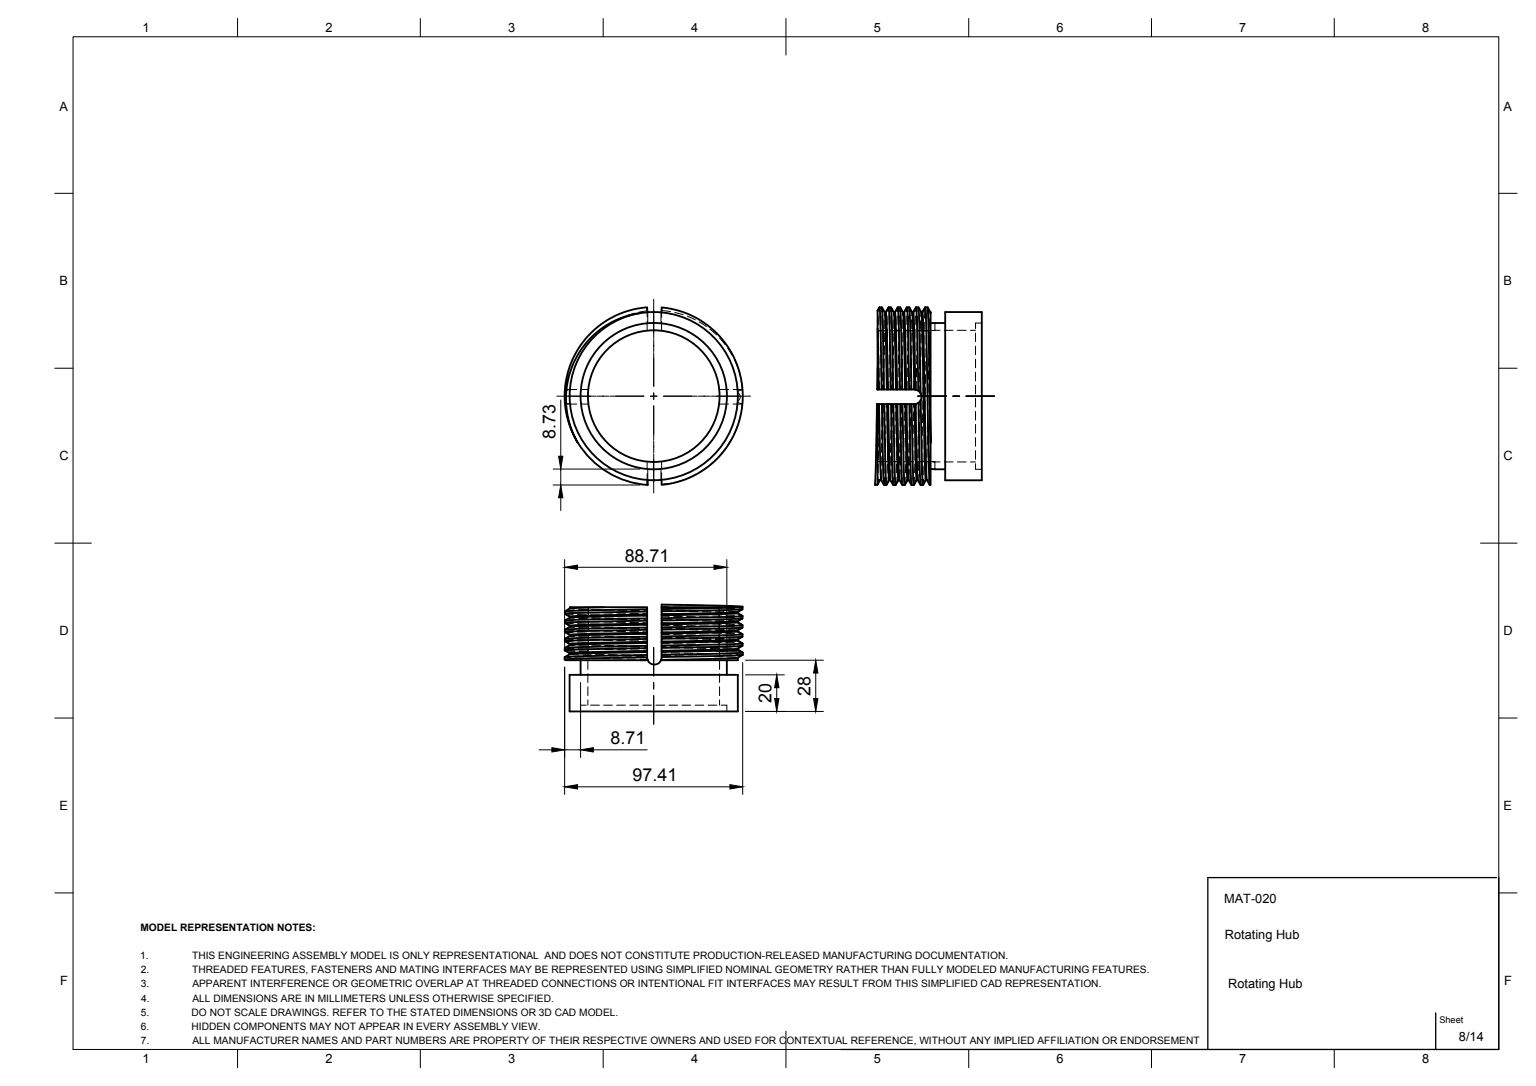
ISO-10303-21;
HEADER;
/* Generated by software containing ST-Developer
 * from STEP Tools, Inc. (www.steptools.com) 
 */

FILE_DESCRIPTION(
/* description */ ('STEP AP214'),
/* implementation_level */ '2;1');

FILE_NAME(
/* name */ 'Rotating Hub.step',
/* time_stamp */ '2026-11-14T06:20:50-08:00',
/* author */ (''),
/* organization */ (''),
/* preprocessor_version */ 'ST-DEVELOPER v20.2',
/* originating_system */ 'Autodesk Translation Framework v15.17.0.0',
/* authorisation */ '');

FILE_SCHEMA (('AUTOMOTIVE_DESIGN { 1 0 10303 214 3 1 1 }'));
ENDSEC;

DATA;
#10=MECHANICAL_DESIGN_GEOMETRIC_PRESENTATION_REPRESENTATION('',(#959),#20658);
#124=FACE_BOUND('',#1300,.T.);
#125=FACE_BOUND('',#1302,.T.);
#126=FACE_BOUND('',#1314,.T.);
#147=ELLIPSE('',#3911,3.97203818895926,3.95968922073708);
#152=(
BOUNDED_SURFACE()
B_SPLINE_SURFACE(1,2,((#5540,#5541,#5542,#5543,#5544,#5545,#5546,#5547,
#5548,#5549,#5550,#5551,#5552,#5553,#5554,#5555,#5556,#5557,#5558,#5559,
#5560,#5561,#5562,#5563,#5564,#5565,#5566,#5567,#5568,#5569,#5570,#5571,
#5572,#5573,#5574,#5575,#5576,#5577,#5578,#5579,#5580,#5581,#5582,#5583,
#5584,#5585,#5586,#5587,#5588,#5589,#5590,#5591,#5592,#5593,#5594,#5595,
#5596,#5597,#5598,#5599,#5600,#5601,#5602,#5603,#5604,#5605,#5606,#5607,
#5608,#5609,#5610,#5611,#5612,#5613,#5614,#5615,#5616,#5617,#5618,#5619,
#5620,#5621,#5622,#5623,#5624,#5625,#5626,#5627,#5628,#5629,#5630,#5631,
#5632,#5633,#5634,#5635,#5636,#5637,#5638,#5639,#5640,#5641,#5642,#5643,
#5644,#5645,#5646,#5647,#5648,#5649,#5650,#5651,#5652,#5653,#5654,#5655,
#5656,#5657,#5658,#5659,#5660,#5661,#5662,#5663,#5664,#5665,#5666,#5667,
#5668,#5669,#5670,#5671,#5672,#5673,#5674,#5675,#5676,#5677,#5678,#5679,
#5680,#5681,#5682,#5683,#5684),(#5685,#5686,#5687,#5688,#5689,#5690,#5691,
#5692,#5693,#5694,#5695,#5696,#5697,#5698,#5699,#5700,#5701,#5702,#5703,
#5704,#5705,#5706,#5707,#5708,#5709,#5710,#5711,#5712,#5713,#5714,#5715,
#5716,#5717,#5718,#5719,#5720,#5721,#5722,#5723,#5724,#5725,#5726,#5727,
#5728,#5729,#5730,#5731,#5732,#5733,#5734,#5735,#5736,#5737,#5738,#5739,
#5740,#5741,#5742,#5743,#5744,#5745,#5746,#5747,#5748,#5749,#5750,#5751,
#5752,#5753,#5754,#5755,#5756,#5757,#5758,#5759,#5760,#5761,#5762,#5763,
#5764,#5765,#5766,#5767,#5768,#5769,#5770,#5771,#5772,#5773,#5774,#5775,
#5776,#5777,#5778,#5779,#5780,#5781,#5782,#5783,#5784,#5785,#5786,#5787,
#5788,#5789,#5790,#5791,#5792,#5793,#5794,#5795,#5796,#5797,#5798,#5799,
#5800,#5801,#5802,#5803,#5804,#5805,#5806,#5807,#5808,#5809,#5810,#5811,
#5812,#5813,#5814,#5815,#5816,#5817,#5818,#5819,#5820,#5821,#5822,#5823,
#5824,#5825,#5826,#5827,#5828,#5829)),.UNSPECIFIED.,.F.,.F.,.F.)
B_SPLINE_SURFACE_WITH_KNOTS((2,2),(3,2,2,2,2,2,2,2,2,2,2,2,2,2,2,2,2,2,
2,2,2,2,2,2,2,2,2,2,2,2,2,2,2,2,2,2,2,2,2,2,2,2,2,2,2,2,2,2,2,2,2,2,2,2,
2,2,2,2,2,2,2,2,2,2,2,2,2,2,2,2,2,2,3),(0.,1.),(0.,0.0138888888888889,0.0277777777777778,
0.0416666666666667,0.0555555555555556,0.0694444444444444,0.0833333333333333,
0.0972222222222222,0.111111111111111,0.125,0.138888888888889,0.152777777777778,
0.166666666666667,0.180555555555556,0.194444444444444,0.208333333333333,
0.222222222222222,0.236111111111111,0.25,0.263888888888889,0.277777777777778,
0.291666666666667,0.305555555555556,0.319444444444444,0.333333333333333,
0.347222222222222,0.361111111111111,0.375,0.388888888888889,0.402777777777778,
0.416666666666667,0.430555555555556,0.444444444444444,0.458333333333333,
0.472222222222222,0.486111111111111,0.5,0.513888888888889,0.527777777777778,
0.541666666666667,0.555555555555556,0.569444444444444,0.583333333333333,
0.597222222222222,0.611111111111111,0.625,0.638888888888889,0.652777777777778,
0.666666666666667,0.680555555555556,0.694444444444444,0.708333333333333,
0.722222222222222,0.736111111111111,0.75,0.763888888888889,0.777777777777778,
0.791666666666667,0.805555555555556,0.819444444444444,0.833333333333333,
0.847222222222222,0.861111111111111,0.875,0.888888888888889,0.902777777777778,
0.916666666666667,0.930555555555556,0.944444444444444,0.958333333333333,
0.972222222222222,0.986111111111111,1.),.UNSPECIFIED.)
GEOMETRIC_REPRESENTATION_ITEM()
RATIONAL_B_SPLINE_SURFACE(((1.,0.965925826289068,1.,0.965925826289068,1.,
0.965925826289068,1.,0.965925826289068,1.,0.965925826289068,1.,0.965925826289068,
1.,0.965925826289068,1.,0.965925826289068,1.,0.965925826289068,1.,0.965925826289068,
1.,0.965925826289068,1.,0.965925826289068,1.,0.965925826289068,1.,0.965925826289068,
1.,0.965925826289068,1.,0.965925826289068,1.,0.965925826289068,1.,0.965925826289068,
1.,0.965925826289068,1.,0.965925826289068,1.,0.965925826289068,1.,0.965925826289068,
1.,0.965925826289068,1.,0.965925826289068,1.,0.965925826289068,1.,0.965925826289068,
1.,0.965925826289068,1.,0.965925826289068,1.,0.965925826289068,1.,0.965925826289068,
1.,0.965925826289068,1.,0.965925826289068,1.,0.965925826289068,1.,0.965925826289068,
1.,0.965925826289068,1.,0.965925826289068,1.,0.965925826289068,1.,0.965925826289068,
1.,0.965925826289068,1.,0.965925826289068,1.,0.965925826289068,1.,0.965925826289068,
1.,0.965925826289068,1.,0.965925826289068,1.,0.965925826289068,1.,0.965925826289068,
1.,0.965925826289068,1.,0.965925826289068,1.,0.965925826289068,1.,0.965925826289068,
1.,0.965925826289068,1.,0.965925826289068,1.,0.965925826289068,1.,0.965925826289068,
1.,0.965925826289068,1.,0.965925826289068,1.,0.965925826289068,1.,0.965925826289068,
1.,0.965925826289068,1.,0.965925826289068,1.,0.965925826289068,1.,0.965925826289068,
1.,0.965925826289068,1.,0.965925826289068,1.,0.965925826289068,1.,0.965925826289068,
1.,0.965925826289068,1.,0.965925826289068,1.,0.965925826289068,1.,0.965925826289068,
1.,0.965925826289068,1.,0.965925826289068,1.),(1.,0.965925826289068,1.,
0.965925826289068,1.,0.965925826289068,1.,0.965925826289068,1.,0.965925826289068,
1.,0.965925826289068,1.,0.965925826289068,1.,0.965925826289068,1.,0.965925826289068,
1.,0.965925826289068,1.,0.965925826289068,1.,0.965925826289068,1.,0.965925826289068,
1.,0.965925826289068,1.,0.965925826289068,1.,0.965925826289068,1.,0.965925826289068,
1.,0.965925826289068,1.,0.965925826289068,1.,0.965925826289068,1.,0.965925826289068,
1.,0.965925826289068,1.,0.965925826289068,1.,0.965925826289068,1.,0.965925826289068,
1.,0.965925826289068,1.,0.965925826289068,1.,0.965925826289068,1.,0.965925826289068,
1.,0.965925826289068,1.,0.965925826289068,1.,0.965925826289068,1.,0.965925826289068,
1.,0.965925826289068,1.,0.965925826289068,1.,0.965925826289068,1.,0.965925826289068,
1.,0.965925826289068,1.,0.965925826289068,1.,0.965925826289068,1.,0.965925826289068,
1.,0.965925826289068,1.,0.965925826289068,1.,0.965925826289068,1.,0.965925826289068,
1.,0.965925826289068,1.,0.965925826289068,1.,0.965925826289068,1.,0.965925826289068,
1.,0.965925826289068,1.,0.965925826289068,1.,0.965925826289068,1.,0.965925826289068,
1.,0.965925826289068,1.,0.965925826289068,1.,0.965925826289068,1.,0.965925826289068,
1.,0.965925826289068,1.,0.965925826289068,1.,0.965925826289068,1.,0.965925826289068,
1.,0.965925826289068,1.,0.965925826289068,1.,0.965925826289068,1.,0.965925826289068,
1.,0.965925826289068,1.,0.965925826289068,1.,0.965925826289068,1.,0.965925826289068,
1.,0.965925826289068,1.,0.965925826289068,1.,0.965925826289068,1.)))
REPRESENTATION_ITEM('')
SURFACE()
);
#153=(
BOUNDED_SURFACE()
B_SPLINE_SURFACE(1,2,((#5847,#5848,#5849,#5850,#5851,#5852,#5853,#5854,
#5855,#5856,#5857,#5858,#5859,#5860,#5861,#5862,#5863,#5864,#5865,#5866,
#5867,#5868,#5869,#5870,#5871,#5872,#5873,#5874,#5875,#5876,#5877,#5878,
#5879,#5880,#5881,#5882,#5883,#5884,#5885,#5886,#5887,#5888,#5889,#5890,
#5891,#5892,#5893,#5894,#5895,#5896,#5897,#5898,#5899,#5900,#5901,#5902,
#5903,#5904,#5905,#5906,#5907,#5908,#5909,#5910,#5911,#5912,#5913,#5914,
#5915,#5916,#5917,#5918,#5919,#5920,#5921,#5922,#5923,#5924,#5925,#5926,
#5927,#5928,#5929,#5930,#5931,#5932,#5933,#5934,#5935,#5936,#5937,#5938,
#5939,#5940,#5941,#5942,#5943,#5944,#5945,#5946,#5947,#5948,#5949,#5950,
#5951,#5952,#5953,#5954,#5955,#5956,#5957,#5958,#5959,#5960,#5961,#5962,
#5963,#5964,#5965,#5966,#5967,#5968,#5969,#5970,#5971,#5972,#5973,#5974,
#5975,#5976,#5977,#5978,#5979,#5980,#5981,#5982,#5983,#5984,#5985,#5986,
#5987,#5988,#5989,#5990,#5991),(#5992,#5993,#5994,#5995,#5996,#5997,#5998,
#5999,#6000,#6001,#6002,#6003,#6004,#6005,#6006,#6007,#6008,#6009,#6010,
#6011,#6012,#6013,#6014,#6015,#6016,#6017,#6018,#6019,#6020,#6021,#6022,
#6023,#6024,#6025,#6026,#6027,#6028,#6029,#6030,#6031,#6032,#6033,#6034,
#6035,#6036,#6037,#6038,#6039,#6040,#6041,#6042,#6043,#6044,#6045,#6046,
#6047,#6048,#6049,#6050,#6051,#6052,#6053,#6054,#6055,#6056,#6057,#6058,
#6059,#6060,#6061,#6062,#6063,#6064,#6065,#6066,#6067,#6068,#6069,#6070,
#6071,#6072,#6073,#6074,#6075,#6076,#6077,#6078,#6079,#6080,#6081,#6082,
#6083,#6084,#6085,#6086,#6087,#6088,#6089,#6090,#6091,#6092,#6093,#6094,
#6095,#6096,#6097,#6098,#6099,#6100,#6101,#6102,#6103,#6104,#6105,#6106,
#6107,#6108,#6109,#6110,#6111,#6112,#6113,#6114,#6115,#6116,#6117,#6118,
#6119,#6120,#6121,#6122,#6123,#6124,#6125,#6126,#6127,#6128,#6129,#6130,
#6131,#6132,#6133,#6134,#6135,#6136)),.UNSPECIFIED.,.F.,.F.,.F.)
B_SPLINE_SURFACE_WITH_KNOTS((2,2),(3,2,2,2,2,2,2,2,2,2,2,2,2,2,2,2,2,2,
2,2,2,2,2,2,2,2,2,2,2,2,2,2,2,2,2,2,2,2,2,2,2,2,2,2,2,2,2,2,2,2,2,2,2,2,
2,2,2,2,2,2,2,2,2,2,2,2,2,2,2,2,2,2,3),(0.,1.),(0.,0.0138888888888889,0.0277777777777778,
0.0416666666666667,0.0555555555555556,0.0694444444444444,0.0833333333333333,
0.0972222222222222,0.111111111111111,0.125,0.138888888888889,0.152777777777778,
0.166666666666667,0.180555555555556,0.194444444444444,0.208333333333333,
0.222222222222222,0.236111111111111,0.25,0.263888888888889,0.277777777777778,
0.291666666666667,0.305555555555556,0.319444444444444,0.333333333333333,
0.347222222222222,0.361111111111111,0.375,0.388888888888889,0.402777777777778,
0.416666666666667,0.430555555555556,0.444444444444444,0.458333333333333,
0.472222222222222,0.486111111111111,0.5,0.513888888888889,0.527777777777778,
0.541666666666667,0.555555555555556,0.569444444444444,0.583333333333333,
0.597222222222222,0.611111111111111,0.625,0.638888888888889,0.652777777777778,
0.666666666666667,0.680555555555556,0.694444444444444,0.708333333333333,
0.722222222222222,0.736111111111111,0.75,0.763888888888889,0.777777777777778,
0.791666666666667,0.805555555555556,0.819444444444444,0.833333333333333,
0.847222222222222,0.861111111111111,0.875,0.888888888888889,0.902777777777778,
0.916666666666667,0.930555555555556,0.944444444444444,0.958333333333333,
0.972222222222222,0.986111111111111,1.),.UNSPECIFIED.)
GEOMETRIC_REPRESENTATION_ITEM()
RATIONAL_B_SPLINE_SURFACE(((1.,0.965925826289068,1.,0.965925826289068,1.,
0.965925826289068,1.,0.965925826289068,1.,0.965925826289068,1.,0.965925826289068,
1.,0.965925826289068,1.,0.965925826289068,1.,0.965925826289068,1.,0.965925826289068,
1.,0.965925826289068,1.,0.965925826289068,1.,0.965925826289068,1.,0.965925826289068,
1.,0.965925826289068,1.,0.965925826289068,1.,0.965925826289068,1.,0.965925826289068,
1.,0.965925826289068,1.,0.965925826289068,1.,0.965925826289068,1.,0.965925826289068,
1.,0.965925826289068,1.,0.965925826289068,1.,0.965925826289068,1.,0.965925826289068,
1.,0.965925826289068,1.,0.965925826289068,1.,0.965925826289068,1.,0.965925826289068,
1.,0.965925826289068,1.,0.965925826289068,1.,0.965925826289068,1.,0.965925826289068,
1.,0.965925826289068,1.,0.965925826289068,1.,0.965925826289068,1.,0.965925826289068,
1.,0.965925826289068,1.,0.965925826289068,1.,0.965925826289068,1.,0.965925826289068,
1.,0.965925826289068,1.,0.965925826289068,1.,0.965925826289068,1.,0.965925826289068,
1.,0.965925826289068,1.,0.965925826289068,1.,0.965925826289068,1.,0.965925826289068,
1.,0.965925826289068,1.,0.965925826289068,1.,0.965925826289068,1.,0.965925826289068,
1.,0.965925826289068,1.,0.965925826289068,1.,0.965925826289068,1.,0.965925826289068,
1.,0.965925826289068,1.,0.965925826289068,1.,0.965925826289068,1.,0.965925826289068,
1.,0.965925826289068,1.,0.965925826289068,1.,0.965925826289068,1.,0.965925826289068,
1.,0.965925826289068,1.,0.965925826289068,1.,0.965925826289068,1.,0.965925826289068,
1.,0.965925826289068,1.,0.965925826289068,1.),(1.,0.965925826289068,1.,
0.965925826289068,1.,0.965925826289068,1.,0.965925826289068,1.,0.965925826289068,
1.,0.965925826289068,1.,0.965925826289068,1.,0.965925826289068,1.,0.965925826289068,
1.,0.965925826289068,1.,0.965925826289068,1.,0.965925826289068,1.,0.965925826289068,
1.,0.965925826289068,1.,0.965925826289068,1.,0.965925826289068,1.,0.965925826289068,
1.,0.965925826289068,1.,0.965925826289068,1.,0.965925826289068,1.,0.965925826289068,
1.,0.965925826289068,1.,0.965925826289068,1.,0.965925826289068,1.,0.965925826289068,
1.,0.965925826289068,1.,0.965925826289068,1.,0.965925826289068,1.,0.965925826289068,
1.,0.965925826289068,1.,0.965925826289068,1.,0.965925826289068,1.,0.965925826289068,
1.,0.965925826289068,1.,0.965925826289068,1.,0.965925826289068,1.,0.965925826289068,
1.,0.965925826289068,1.,0.965925826289068,1.,0.965925826289068,1.,0.965925826289068,
1.,0.965925826289068,1.,0.965925826289068,1.,0.965925826289068,1.,0.965925826289068,
1.,0.965925826289068,1.,0.965925826289068,1.,0.965925826289068,1.,0.965925826289068,
1.,0.965925826289068,1.,0.965925826289068,1.,0.965925826289068,1.,0.965925826289068,
1.,0.965925826289068,1.,0.965925826289068,1.,0.965925826289068,1.,0.965925826289068,
1.,0.965925826289068,1.,0.965925826289068,1.,0.965925826289068,1.,0.965925826289068,
1.,0.965925826289068,1.,0.965925826289068,1.,0.965925826289068,1.,0.965925826289068,
1.,0.965925826289068,1.,0.965925826289068,1.,0.965925826289068,1.,0.965925826289068,
1.,0.965925826289068,1.,0.965925826289068,1.,0.965925826289068,1.)))
REPRESENTATION_ITEM('')
SURFACE()
);
#154=(
BOUNDED_SURFACE()
B_SPLINE_SURFACE(1,2,((#6162,#6163,#6164,#6165,#6166,#6167,#6168,#6169,
#6170,#6171,#6172,#6173,#6174,#6175,#6176,#6177,#6178,#6179,#6180,#6181,
#6182,#6183,#6184,#6185,#6186,#6187,#6188,#6189,#6190,#6191,#6192,#6193,
#6194,#6195,#6196,#6197,#6198,#6199,#6200,#6201,#6202,#6203,#6204,#6205,
#6206,#6207,#6208,#6209,#6210,#6211,#6212,#6213,#6214,#6215,#6216,#6217,
#6218,#6219,#6220,#6221,#6222,#6223,#6224,#6225,#6226,#6227,#6228,#6229,
#6230,#6231,#6232,#6233,#6234,#6235,#6236,#6237,#6238,#6239,#6240,#6241,
#6242,#6243,#6244,#6245,#6246,#6247,#6248,#6249,#6250,#6251,#6252,#6253,
#6254,#6255,#6256,#6257,#6258,#6259,#6260,#6261,#6262,#6263,#6264,#6265,
#6266,#6267,#6268,#6269,#6270,#6271,#6272,#6273,#6274,#6275,#6276,#6277,
#6278,#6279,#6280,#6281,#6282,#6283,#6284,#6285,#6286,#6287,#6288,#6289,
#6290,#6291,#6292,#6293,#6294,#6295,#6296,#6297,#6298,#6299,#6300,#6301,
#6302,#6303,#6304,#6305,#6306),(#6307,#6308,#6309,#6310,#6311,#6312,#6313,
#6314,#6315,#6316,#6317,#6318,#6319,#6320,#6321,#6322,#6323,#6324,#6325,
#6326,#6327,#6328,#6329,#6330,#6331,#6332,#6333,#6334,#6335,#6336,#6337,
#6338,#6339,#6340,#6341,#6342,#6343,#6344,#6345,#6346,#6347,#6348,#6349,
#6350,#6351,#6352,#6353,#6354,#6355,#6356,#6357,#6358,#6359,#6360,#6361,
#6362,#6363,#6364,#6365,#6366,#6367,#6368,#6369,#6370,#6371,#6372,#6373,
#6374,#6375,#6376,#6377,#6378,#6379,#6380,#6381,#6382,#6383,#6384,#6385,
#6386,#6387,#6388,#6389,#6390,#6391,#6392,#6393,#6394,#6395,#6396,#6397,
#6398,#6399,#6400,#6401,#6402,#6403,#6404,#6405,#6406,#6407,#6408,#6409,
#6410,#6411,#6412,#6413,#6414,#6415,#6416,#6417,#6418,#6419,#6420,#6421,
#6422,#6423,#6424,#6425,#6426,#6427,#6428,#6429,#6430,#6431,#6432,#6433,
#6434,#6435,#6436,#6437,#6438,#6439,#6440,#6441,#6442,#6443,#6444,#6445,
#6446,#6447,#6448,#6449,#6450,#6451)),.UNSPECIFIED.,.F.,.F.,.F.)
B_SPLINE_SURFACE_WITH_KNOTS((2,2),(3,2,2,2,2,2,2,2,2,2,2,2,2,2,2,2,2,2,
2,2,2,2,2,2,2,2,2,2,2,2,2,2,2,2,2,2,2,2,2,2,2,2,2,2,2,2,2,2,2,2,2,2,2,2,
2,2,2,2,2,2,2,2,2,2,2,2,2,2,2,2,2,2,3),(0.,1.),(0.,0.0138888888888889,0.0277777777777778,
0.0416666666666667,0.0555555555555556,0.0694444444444444,0.0833333333333333,
0.0972222222222222,0.111111111111111,0.125,0.138888888888889,0.152777777777778,
0.166666666666667,0.180555555555556,0.194444444444444,0.208333333333333,
0.222222222222222,0.236111111111111,0.25,0.263888888888889,0.277777777777778,
0.291666666666667,0.305555555555556,0.319444444444444,0.333333333333333,
0.347222222222222,0.361111111111111,0.375,0.388888888888889,0.402777777777778,
0.416666666666667,0.430555555555556,0.444444444444444,0.458333333333333,
0.472222222222222,0.486111111111111,0.5,0.513888888888889,0.527777777777778,
0.541666666666667,0.555555555555556,0.569444444444444,0.583333333333333,
0.597222222222222,0.611111111111111,0.625,0.638888888888889,0.652777777777778,
0.666666666666667,0.680555555555556,0.694444444444444,0.708333333333333,
0.722222222222222,0.736111111111111,0.75,0.763888888888889,0.777777777777778,
0.791666666666667,0.805555555555556,0.819444444444444,0.833333333333333,
0.847222222222222,0.861111111111111,0.875,0.888888888888889,0.902777777777778,
0.916666666666667,0.930555555555556,0.944444444444444,0.958333333333333,
0.972222222222222,0.986111111111111,1.),.UNSPECIFIED.)
GEOMETRIC_REPRESENTATION_ITEM()
RATIONAL_B_SPLINE_SURFACE(((1.,0.965925826289068,1.,0.965925826289068,1.,
0.965925826289068,1.,0.965925826289068,1.,0.965925826289068,1.,0.965925826289068,
1.,0.965925826289068,1.,0.965925826289068,1.,0.965925826289068,1.,0.965925826289068,
1.,0.965925826289068,1.,0.965925826289068,1.,0.965925826289068,1.,0.965925826289068,
1.,0.965925826289068,1.,0.965925826289068,1.,0.965925826289068,1.,0.965925826289068,
1.,0.965925826289068,1.,0.965925826289068,1.,0.965925826289068,1.,0.965925826289068,
1.,0.965925826289068,1.,0.965925826289068,1.,0.965925826289068,1.,0.965925826289068,
1.,0.965925826289068,1.,0.965925826289068,1.,0.965925826289068,1.,0.965925826289068,
1.,0.965925826289068,1.,0.965925826289068,1.,0.965925826289068,1.,0.965925826289068,
1.,0.965925826289068,1.,0.965925826289068,1.,0.965925826289068,1.,0.965925826289068,
1.,0.965925826289068,1.,0.965925826289068,1.,0.965925826289068,1.,0.965925826289068,
1.,0.965925826289068,1.,0.965925826289068,1.,0.965925826289068,1.,0.965925826289068,
1.,0.965925826289068,1.,0.965925826289068,1.,0.965925826289068,1.,0.965925826289068,
1.,0.965925826289068,1.,0.965925826289068,1.,0.965925826289068,1.,0.965925826289068,
1.,0.965925826289068,1.,0.965925826289068,1.,0.965925826289068,1.,0.965925826289068,
1.,0.965925826289068,1.,0.965925826289068,1.,0.965925826289068,1.,0.965925826289068,
1.,0.965925826289068,1.,0.965925826289068,1.,0.965925826289068,1.,0.965925826289068,
1.,0.965925826289068,1.,0.965925826289068,1.,0.965925826289068,1.,0.965925826289068,
1.,0.965925826289068,1.,0.965925826289068,1.),(1.,0.965925826289068,1.,
0.965925826289068,1.,0.965925826289068,1.,0.965925826289068,1.,0.965925826289068,
1.,0.965925826289068,1.,0.965925826289068,1.,0.965925826289068,1.,0.965925826289068,
1.,0.965925826289068,1.,0.965925826289068,1.,0.965925826289068,1.,0.965925826289068,
1.,0.965925826289068,1.,0.965925826289068,1.,0.965925826289068,1.,0.965925826289068,
1.,0.965925826289068,1.,0.965925826289068,1.,0.965925826289068,1.,0.965925826289068,
1.,0.965925826289068,1.,0.965925826289068,1.,0.965925826289068,1.,0.965925826289068,
1.,0.965925826289068,1.,0.965925826289068,1.,0.965925826289068,1.,0.965925826289068,
1.,0.965925826289068,1.,0.965925826289068,1.,0.965925826289068,1.,0.965925826289068,
1.,0.965925826289068,1.,0.965925826289068,1.,0.965925826289068,1.,0.965925826289068,
1.,0.965925826289068,1.,0.965925826289068,1.,0.965925826289068,1.,0.965925826289068,
1.,0.965925826289068,1.,0.965925826289068,1.,0.965925826289068,1.,0.965925826289068,
1.,0.965925826289068,1.,0.965925826289068,1.,0.965925826289068,1.,0.965925826289068,
1.,0.965925826289068,1.,0.965925826289068,1.,0.965925826289068,1.,0.965925826289068,
1.,0.965925826289068,1.,0.965925826289068,1.,0.965925826289068,1.,0.965925826289068,
1.,0.965925826289068,1.,0.965925826289068,1.,0.965925826289068,1.,0.965925826289068,
1.,0.965925826289068,1.,0.965925826289068,1.,0.965925826289068,1.,0.965925826289068,
1.,0.965925826289068,1.,0.965925826289068,1.,0.965925826289068,1.,0.965925826289068,
1.,0.965925826289068,1.,0.965925826289068,1.,0.965925826289068,1.)))
REPRESENTATION_ITEM('')
SURFACE()
);
#155=(
BOUNDED_SURFACE()
B_SPLINE_SURFACE(1,2,((#6469,#6470,#6471,#6472,#6473,#6474,#6475,#6476,
#6477,#6478,#6479,#6480,#6481,#6482,#6483,#6484,#6485,#6486,#6487,#6488,
#6489,#6490,#6491,#6492,#6493,#6494,#6495,#6496,#6497,#6498,#6499,#6500,
#6501,#6502,#6503,#6504,#6505,#6506,#6507,#6508,#6509,#6510,#6511,#6512,
#6513,#6514,#6515,#6516,#6517,#6518,#6519,#6520,#6521,#6522,#6523,#6524,
#6525,#6526,#6527,#6528,#6529,#6530,#6531,#6532,#6533,#6534,#6535,#6536,
#6537,#6538,#6539,#6540,#6541,#6542,#6543,#6544,#6545,#6546,#6547,#6548,
#6549,#6550,#6551,#6552,#6553,#6554,#6555,#6556,#6557,#6558,#6559,#6560,
#6561,#6562,#6563,#6564,#6565,#6566,#6567,#6568,#6569,#6570,#6571,#6572,
#6573,#6574,#6575,#6576,#6577,#6578,#6579,#6580,#6581,#6582,#6583,#6584,
#6585,#6586,#6587,#6588,#6589,#6590,#6591,#6592,#6593,#6594,#6595,#6596,
#6597,#6598,#6599,#6600,#6601,#6602,#6603,#6604,#6605,#6606,#6607,#6608,
#6609,#6610,#6611,#6612,#6613),(#6614,#6615,#6616,#6617,#6618,#6619,#6620,
#6621,#6622,#6623,#6624,#6625,#6626,#6627,#6628,#6629,#6630,#6631,#6632,
#6633,#6634,#6635,#6636,#6637,#6638,#6639,#6640,#6641,#6642,#6643,#6644,
#6645,#6646,#6647,#6648,#6649,#6650,#6651,#6652,#6653,#6654,#6655,#6656,
#6657,#6658,#6659,#6660,#6661,#6662,#6663,#6664,#6665,#6666,#6667,#6668,
#6669,#6670,#6671,#6672,#6673,#6674,#6675,#6676,#6677,#6678,#6679,#6680,
#6681,#6682,#6683,#6684,#6685,#6686,#6687,#6688,#6689,#6690,#6691,#6692,
#6693,#6694,#6695,#6696,#6697,#6698,#6699,#6700,#6701,#6702,#6703,#6704,
#6705,#6706,#6707,#6708,#6709,#6710,#6711,#6712,#6713,#6714,#6715,#6716,
#6717,#6718,#6719,#6720,#6721,#6722,#6723,#6724,#6725,#6726,#6727,#6728,
#6729,#6730,#6731,#6732,#6733,#6734,#6735,#6736,#6737,#6738,#6739,#6740,
#6741,#6742,#6743,#6744,#6745,#6746,#6747,#6748,#6749,#6750,#6751,#6752,
#6753,#6754,#6755,#6756,#6757,#6758)),.UNSPECIFIED.,.F.,.F.,.F.)
B_SPLINE_SURFACE_WITH_KNOTS((2,2),(3,2,2,2,2,2,2,2,2,2,2,2,2,2,2,2,2,2,
2,2,2,2,2,2,2,2,2,2,2,2,2,2,2,2,2,2,2,2,2,2,2,2,2,2,2,2,2,2,2,2,2,2,2,2,
2,2,2,2,2,2,2,2,2,2,2,2,2,2,2,2,2,2,3),(0.,1.),(0.,0.0138888888888889,0.0277777777777778,
0.0416666666666667,0.0555555555555556,0.0694444444444444,0.0833333333333333,
0.0972222222222222,0.111111111111111,0.125,0.138888888888889,0.152777777777778,
0.166666666666667,0.180555555555556,0.194444444444444,0.208333333333333,
0.222222222222222,0.236111111111111,0.25,0.263888888888889,0.277777777777778,
0.291666666666667,0.305555555555556,0.319444444444444,0.333333333333333,
0.347222222222222,0.361111111111111,0.375,0.388888888888889,0.402777777777778,
0.416666666666667,0.430555555555556,0.444444444444444,0.458333333333333,
0.472222222222222,0.486111111111111,0.5,0.513888888888889,0.527777777777778,
0.541666666666667,0.555555555555556,0.569444444444444,0.583333333333333,
0.597222222222222,0.611111111111111,0.625,0.638888888888889,0.652777777777778,
0.666666666666667,0.680555555555556,0.694444444444444,0.708333333333333,
0.722222222222222,0.736111111111111,0.75,0.763888888888889,0.777777777777778,
0.791666666666667,0.805555555555556,0.819444444444444,0.833333333333333,
0.847222222222222,0.861111111111111,0.875,0.888888888888889,0.902777777777778,
0.916666666666667,0.930555555555556,0.944444444444444,0.958333333333333,
0.972222222222222,0.986111111111111,1.),.UNSPECIFIED.)
GEOMETRIC_REPRESENTATION_ITEM()
RATIONAL_B_SPLINE_SURFACE(((1.,0.965925826289068,1.,0.965925826289068,1.,
0.965925826289068,1.,0.965925826289068,1.,0.965925826289068,1.,0.965925826289068,
1.,0.965925826289068,1.,0.965925826289068,1.,0.965925826289068,1.,0.965925826289068,
1.,0.965925826289068,1.,0.965925826289068,1.,0.965925826289068,1.,0.965925826289068,
1.,0.965925826289068,1.,0.965925826289068,1.,0.965925826289068,1.,0.965925826289068,
1.,0.965925826289068,1.,0.965925826289068,1.,0.965925826289068,1.,0.965925826289068,
1.,0.965925826289068,1.,0.965925826289068,1.,0.965925826289068,1.,0.965925826289068,
1.,0.965925826289068,1.,0.965925826289068,1.,0.965925826289068,1.,0.965925826289068,
1.,0.965925826289068,1.,0.965925826289068,1.,0.965925826289068,1.,0.965925826289068,
1.,0.965925826289068,1.,0.965925826289068,1.,0.965925826289068,1.,0.965925826289068,
1.,0.965925826289068,1.,0.965925826289068,1.,0.965925826289068,1.,0.965925826289068,
1.,0.965925826289068,1.,0.965925826289068,1.,0.965925826289068,1.,0.965925826289068,
1.,0.965925826289068,1.,0.965925826289068,1.,0.965925826289068,1.,0.965925826289068,
1.,0.965925826289068,1.,0.965925826289068,1.,0.965925826289068,1.,0.965925826289068,
1.,0.965925826289068,1.,0.965925826289068,1.,0.965925826289068,1.,0.965925826289068,
1.,0.965925826289068,1.,0.965925826289068,1.,0.965925826289068,1.,0.965925826289068,
1.,0.965925826289068,1.,0.965925826289068,1.,0.965925826289068,1.,0.965925826289068,
1.,0.965925826289068,1.,0.965925826289068,1.,0.965925826289068,1.,0.965925826289068,
1.,0.965925826289068,1.,0.965925826289068,1.),(1.,0.965925826289068,1.,
0.965925826289068,1.,0.965925826289068,1.,0.965925826289068,1.,0.965925826289068,
1.,0.965925826289068,1.,0.965925826289068,1.,0.965925826289068,1.,0.965925826289068,
1.,0.965925826289068,1.,0.965925826289068,1.,0.965925826289068,1.,0.965925826289068,
1.,0.965925826289068,1.,0.965925826289068,1.,0.965925826289068,1.,0.965925826289068,
1.,0.965925826289068,1.,0.965925826289068,1.,0.965925826289068,1.,0.965925826289068,
1.,0.965925826289068,1.,0.965925826289068,1.,0.965925826289068,1.,0.965925826289068,
1.,0.965925826289068,1.,0.965925826289068,1.,0.965925826289068,1.,0.965925826289068,
1.,0.965925826289068,1.,0.965925826289068,1.,0.965925826289068,1.,0.965925826289068,
1.,0.965925826289068,1.,0.965925826289068,1.,0.965925826289068,1.,0.965925826289068,
1.,0.965925826289068,1.,0.965925826289068,1.,0.965925826289068,1.,0.965925826289068,
1.,0.965925826289068,1.,0.965925826289068,1.,0.965925826289068,1.,0.965925826289068,
1.,0.965925826289068,1.,0.965925826289068,1.,0.965925826289068,1.,0.965925826289068,
1.,0.965925826289068,1.,0.965925826289068,1.,0.965925826289068,1.,0.965925826289068,
1.,0.965925826289068,1.,0.965925826289068,1.,0.965925826289068,1.,0.965925826289068,
1.,0.965925826289068,1.,0.965925826289068,1.,0.965925826289068,1.,0.965925826289068,
1.,0.965925826289068,1.,0.965925826289068,1.,0.965925826289068,1.,0.965925826289068,
1.,0.965925826289068,1.,0.965925826289068,1.,0.965925826289068,1.,0.965925826289068,
1.,0.965925826289068,1.,0.965925826289068,1.,0.965925826289068,1.)))
REPRESENTATION_ITEM('')
SURFACE()
);
#156=(
BOUNDED_SURFACE()
B_SPLINE_SURFACE(1,2,((#6784,#6785,#6786,#6787,#6788,#6789,#6790,#6791,
#6792,#6793,#6794,#6795,#6796,#6797,#6798,#6799,#6800,#6801,#6802,#6803,
#6804,#6805,#6806,#6807,#6808,#6809,#6810,#6811,#6812,#6813,#6814,#6815,
#6816,#6817,#6818,#6819,#6820,#6821,#6822,#6823,#6824,#6825,#6826,#6827,
#6828,#6829,#6830,#6831,#6832,#6833,#6834,#6835,#6836,#6837,#6838,#6839,
#6840,#6841,#6842,#6843,#6844,#6845,#6846,#6847,#6848,#6849,#6850,#6851,
#6852,#6853,#6854,#6855,#6856,#6857,#6858,#6859,#6860,#6861,#6862,#6863,
#6864,#6865,#6866,#6867,#6868,#6869,#6870,#6871,#6872,#6873,#6874,#6875,
#6876,#6877,#6878,#6879,#6880,#6881,#6882,#6883,#6884,#6885,#6886,#6887,
#6888,#6889,#6890,#6891,#6892,#6893,#6894,#6895,#6896,#6897,#6898,#6899,
#6900,#6901,#6902,#6903,#6904,#6905,#6906,#6907,#6908,#6909,#6910,#6911,
#6912,#6913,#6914,#6915,#6916,#6917,#6918,#6919,#6920,#6921,#6922,#6923,
#6924,#6925,#6926,#6927,#6928),(#6929,#6930,#6931,#6932,#6933,#6934,#6935,
#6936,#6937,#6938,#6939,#6940,#6941,#6942,#6943,#6944,#6945,#6946,#6947,
#6948,#6949,#6950,#6951,#6952,#6953,#6954,#6955,#6956,#6957,#6958,#6959,
#6960,#6961,#6962,#6963,#6964,#6965,#6966,#6967,#6968,#6969,#6970,#6971,
#6972,#6973,#6974,#6975,#6976,#6977,#6978,#6979,#6980,#6981,#6982,#6983,
#6984,#6985,#6986,#6987,#6988,#6989,#6990,#6991,#6992,#6993,#6994,#6995,
#6996,#6997,#6998,#6999,#7000,#7001,#7002,#7003,#7004,#7005,#7006,#7007,
#7008,#7009,#7010,#7011,#7012,#7013,#7014,#7015,#7016,#7017,#7018,#7019,
#7020,#7021,#7022,#7023,#7024,#7025,#7026,#7027,#7028,#7029,#7030,#7031,
#7032,#7033,#7034,#7035,#7036,#7037,#7038,#7039,#7040,#7041,#7042,#7043,
#7044,#7045,#7046,#7047,#7048,#7049,#7050,#7051,#7052,#7053,#7054,#7055,
#7056,#7057,#7058,#7059,#7060,#7061,#7062,#7063,#7064,#7065,#7066,#7067,
#7068,#7069,#7070,#7071,#7072,#7073)),.UNSPECIFIED.,.F.,.F.,.F.)
B_SPLINE_SURFACE_WITH_KNOTS((2,2),(3,2,2,2,2,2,2,2,2,2,2,2,2,2,2,2,2,2,
2,2,2,2,2,2,2,2,2,2,2,2,2,2,2,2,2,2,2,2,2,2,2,2,2,2,2,2,2,2,2,2,2,2,2,2,
2,2,2,2,2,2,2,2,2,2,2,2,2,2,2,2,2,2,3),(0.,1.),(0.,0.0138888888888889,0.0277777777777778,
0.0416666666666667,0.0555555555555556,0.0694444444444444,0.0833333333333333,
0.0972222222222222,0.111111111111111,0.125,0.138888888888889,0.152777777777778,
0.166666666666667,0.180555555555556,0.194444444444444,0.208333333333333,
0.222222222222222,0.236111111111111,0.25,0.263888888888889,0.277777777777778,
0.291666666666667,0.305555555555556,0.319444444444444,0.333333333333333,
0.347222222222222,0.361111111111111,0.375,0.388888888888889,0.402777777777778,
0.416666666666667,0.430555555555556,0.444444444444444,0.458333333333333,
0.472222222222222,0.486111111111111,0.5,0.513888888888889,0.527777777777778,
0.541666666666667,0.555555555555556,0.569444444444444,0.583333333333333,
0.597222222222222,0.611111111111111,0.625,0.638888888888889,0.652777777777778,
0.666666666666667,0.680555555555556,0.694444444444444,0.708333333333333,
0.722222222222222,0.736111111111111,0.75,0.763888888888889,0.777777777777778,
0.791666666666667,0.805555555555556,0.819444444444444,0.833333333333333,
0.847222222222222,0.861111111111111,0.875,0.888888888888889,0.902777777777778,
0.916666666666667,0.930555555555556,0.944444444444444,0.958333333333333,
0.972222222222222,0.986111111111111,1.),.UNSPECIFIED.)
GEOMETRIC_REPRESENTATION_ITEM()
RATIONAL_B_SPLINE_SURFACE(((1.,0.965925826289068,1.,0.965925826289068,1.,
0.965925826289068,1.,0.965925826289068,1.,0.965925826289068,1.,0.965925826289068,
1.,0.965925826289068,1.,0.965925826289068,1.,0.965925826289068,1.,0.965925826289068,
1.,0.965925826289068,1.,0.965925826289068,1.,0.965925826289068,1.,0.965925826289068,
1.,0.965925826289068,1.,0.965925826289068,1.,0.965925826289068,1.,0.965925826289068,
1.,0.965925826289068,1.,0.965925826289068,1.,0.965925826289068,1.,0.965925826289068,
1.,0.965925826289068,1.,0.965925826289068,1.,0.965925826289068,1.,0.965925826289068,
1.,0.965925826289068,1.,0.965925826289068,1.,0.965925826289068,1.,0.965925826289068,
1.,0.965925826289068,1.,0.965925826289068,1.,0.965925826289068,1.,0.965925826289068,
1.,0.965925826289068,1.,0.965925826289068,1.,0.965925826289068,1.,0.965925826289068,
1.,0.965925826289068,1.,0.965925826289068,1.,0.965925826289068,1.,0.965925826289068,
1.,0.965925826289068,1.,0.965925826289068,1.,0.965925826289068,1.,0.965925826289068,
1.,0.965925826289068,1.,0.965925826289068,1.,0.965925826289068,1.,0.965925826289068,
1.,0.965925826289068,1.,0.965925826289068,1.,0.965925826289068,1.,0.965925826289068,
1.,0.965925826289068,1.,0.965925826289068,1.,0.965925826289068,1.,0.965925826289068,
1.,0.965925826289068,1.,0.965925826289068,1.,0.965925826289068,1.,0.965925826289068,
1.,0.965925826289068,1.,0.965925826289068,1.,0.965925826289068,1.,0.965925826289068,
1.,0.965925826289068,1.,0.965925826289068,1.,0.965925826289068,1.,0.965925826289068,
1.,0.965925826289068,1.,0.965925826289068,1.),(1.,0.965925826289068,1.,
0.965925826289068,1.,0.965925826289068,1.,0.965925826289068,1.,0.965925826289068,
1.,0.965925826289068,1.,0.965925826289068,1.,0.965925826289068,1.,0.965925826289068,
1.,0.965925826289068,1.,0.965925826289068,1.,0.965925826289068,1.,0.965925826289068,
1.,0.965925826289068,1.,0.965925826289068,1.,0.965925826289068,1.,0.965925826289068,
1.,0.965925826289068,1.,0.965925826289068,1.,0.965925826289068,1.,0.965925826289068,
1.,0.965925826289068,1.,0.965925826289068,1.,0.965925826289068,1.,0.965925826289068,
1.,0.965925826289068,1.,0.965925826289068,1.,0.965925826289068,1.,0.965925826289068,
1.,0.965925826289068,1.,0.965925826289068,1.,0.965925826289068,1.,0.965925826289068,
1.,0.965925826289068,1.,0.965925826289068,1.,0.965925826289068,1.,0.965925826289068,
1.,0.965925826289068,1.,0.965925826289068,1.,0.965925826289068,1.,0.965925826289068,
1.,0.965925826289068,1.,0.965925826289068,1.,0.965925826289068,1.,0.965925826289068,
1.,0.965925826289068,1.,0.965925826289068,1.,0.965925826289068,1.,0.965925826289068,
1.,0.965925826289068,1.,0.965925826289068,1.,0.965925826289068,1.,0.965925826289068,
1.,0.965925826289068,1.,0.965925826289068,1.,0.965925826289068,1.,0.965925826289068,
1.,0.965925826289068,1.,0.965925826289068,1.,0.965925826289068,1.,0.965925826289068,
1.,0.965925826289068,1.,0.965925826289068,1.,0.965925826289068,1.,0.965925826289068,
1.,0.965925826289068,1.,0.965925826289068,1.,0.965925826289068,1.,0.965925826289068,
1.,0.965925826289068,1.,0.965925826289068,1.,0.965925826289068,1.)))
REPRESENTATION_ITEM('')
SURFACE()
);
#157=(
BOUNDED_SURFACE()
B_SPLINE_SURFACE(1,2,((#7091,#7092,#7093,#7094,#7095,#7096,#7097,#7098,
#7099,#7100,#7101,#7102,#7103,#7104,#7105,#7106,#7107,#7108,#7109,#7110,
#7111,#7112,#7113,#7114,#7115,#7116,#7117,#7118,#7119,#7120,#7121,#7122,
#7123,#7124,#7125,#7126,#7127,#7128,#7129,#7130,#7131,#7132,#7133,#7134,
#7135,#7136,#7137,#7138,#7139,#7140,#7141,#7142,#7143,#7144,#7145,#7146,
#7147,#7148,#7149,#7150,#7151,#7152,#7153,#7154,#7155,#7156,#7157,#7158,
#7159,#7160,#7161,#7162,#7163,#7164,#7165,#7166,#7167,#7168,#7169,#7170,
#7171,#7172,#7173,#7174,#7175,#7176,#7177,#7178,#7179,#7180,#7181,#7182,
#7183,#7184,#7185,#7186,#7187,#7188,#7189,#7190,#7191,#7192,#7193,#7194,
#7195,#7196,#7197,#7198,#7199,#7200,#7201,#7202,#7203,#7204,#7205,#7206,
#7207,#7208,#7209,#7210,#7211,#7212,#7213,#7214,#7215,#7216,#7217,#7218,
#7219,#7220,#7221,#7222,#7223,#7224,#7225,#7226,#7227,#7228,#7229,#7230,
#7231,#7232,#7233,#7234,#7235),(#7236,#7237,#7238,#7239,#7240,#7241,#7242,
#7243,#7244,#7245,#7246,#7247,#7248,#7249,#7250,#7251,#7252,#7253,#7254,
#7255,#7256,#7257,#7258,#7259,#7260,#7261,#7262,#7263,#7264,#7265,#7266,
#7267,#7268,#7269,#7270,#7271,#7272,#7273,#7274,#7275,#7276,#7277,#7278,
#7279,#7280,#7281,#7282,#7283,#7284,#7285,#7286,#7287,#7288,#7289,#7290,
#7291,#7292,#7293,#7294,#7295,#7296,#7297,#7298,#7299,#7300,#7301,#7302,
#7303,#7304,#7305,#7306,#7307,#7308,#7309,#7310,#7311,#7312,#7313,#7314,
#7315,#7316,#7317,#7318,#7319,#7320,#7321,#7322,#7323,#7324,#7325,#7326,
#7327,#7328,#7329,#7330,#7331,#7332,#7333,#7334,#7335,#7336,#7337,#7338,
#7339,#7340,#7341,#7342,#7343,#7344,#7345,#7346,#7347,#7348,#7349,#7350,
#7351,#7352,#7353,#7354,#7355,#7356,#7357,#7358,#7359,#7360,#7361,#7362,
#7363,#7364,#7365,#7366,#7367,#7368,#7369,#7370,#7371,#7372,#7373,#7374,
#7375,#7376,#7377,#7378,#7379,#7380)),.UNSPECIFIED.,.F.,.F.,.F.)
B_SPLINE_SURFACE_WITH_KNOTS((2,2),(3,2,2,2,2,2,2,2,2,2,2,2,2,2,2,2,2,2,
2,2,2,2,2,2,2,2,2,2,2,2,2,2,2,2,2,2,2,2,2,2,2,2,2,2,2,2,2,2,2,2,2,2,2,2,
2,2,2,2,2,2,2,2,2,2,2,2,2,2,2,2,2,2,3),(0.,1.),(0.,0.0138888888888889,0.0277777777777778,
0.0416666666666667,0.0555555555555556,0.0694444444444444,0.0833333333333333,
0.0972222222222222,0.111111111111111,0.125,0.138888888888889,0.152777777777778,
0.166666666666667,0.180555555555556,0.194444444444444,0.208333333333333,
0.222222222222222,0.236111111111111,0.25,0.263888888888889,0.277777777777778,
0.291666666666667,0.305555555555556,0.319444444444444,0.333333333333333,
0.347222222222222,0.361111111111111,0.375,0.388888888888889,0.402777777777778,
0.416666666666667,0.430555555555556,0.444444444444444,0.458333333333333,
0.472222222222222,0.486111111111111,0.5,0.513888888888889,0.527777777777778,
0.541666666666667,0.555555555555556,0.569444444444444,0.583333333333333,
0.597222222222222,0.611111111111111,0.625,0.638888888888889,0.652777777777778,
0.666666666666667,0.680555555555556,0.694444444444444,0.708333333333333,
0.722222222222222,0.736111111111111,0.75,0.763888888888889,0.777777777777778,
0.791666666666667,0.805555555555556,0.819444444444444,0.833333333333333,
0.847222222222222,0.861111111111111,0.875,0.888888888888889,0.902777777777778,
0.916666666666667,0.930555555555556,0.944444444444444,0.958333333333333,
0.972222222222222,0.986111111111111,1.),.UNSPECIFIED.)
GEOMETRIC_REPRESENTATION_ITEM()
RATIONAL_B_SPLINE_SURFACE(((1.,0.965925826289068,1.,0.965925826289068,1.,
0.965925826289068,1.,0.965925826289068,1.,0.965925826289068,1.,0.965925826289068,
1.,0.965925826289068,1.,0.965925826289068,1.,0.965925826289068,1.,0.965925826289068,
1.,0.965925826289068,1.,0.965925826289068,1.,0.965925826289068,1.,0.965925826289068,
1.,0.965925826289068,1.,0.965925826289068,1.,0.965925826289068,1.,0.965925826289068,
1.,0.965925826289068,1.,0.965925826289068,1.,0.965925826289068,1.,0.965925826289068,
1.,0.965925826289068,1.,0.965925826289068,1.,0.965925826289068,1.,0.965925826289068,
1.,0.965925826289068,1.,0.965925826289068,1.,0.965925826289068,1.,0.965925826289068,
1.,0.965925826289068,1.,0.965925826289068,1.,0.965925826289068,1.,0.965925826289068,
1.,0.965925826289068,1.,0.965925826289068,1.,0.965925826289068,1.,0.965925826289068,
1.,0.965925826289068,1.,0.965925826289068,1.,0.965925826289068,1.,0.965925826289068,
1.,0.965925826289068,1.,0.965925826289068,1.,0.965925826289068,1.,0.965925826289068,
1.,0.965925826289068,1.,0.965925826289068,1.,0.965925826289068,1.,0.965925826289068,
1.,0.965925826289068,1.,0.965925826289068,1.,0.965925826289068,1.,0.965925826289068,
1.,0.965925826289068,1.,0.965925826289068,1.,0.965925826289068,1.,0.965925826289068,
1.,0.965925826289068,1.,0.965925826289068,1.,0.965925826289068,1.,0.965925826289068,
1.,0.965925826289068,1.,0.965925826289068,1.,0.965925826289068,1.,0.965925826289068,
1.,0.965925826289068,1.,0.965925826289068,1.,0.965925826289068,1.,0.965925826289068,
1.,0.965925826289068,1.,0.965925826289068,1.),(1.,0.965925826289068,1.,
0.965925826289068,1.,0.965925826289068,1.,0.965925826289068,1.,0.965925826289068,
1.,0.965925826289068,1.,0.965925826289068,1.,0.965925826289068,1.,0.965925826289068,
1.,0.965925826289068,1.,0.965925826289068,1.,0.965925826289068,1.,0.965925826289068,
1.,0.965925826289068,1.,0.965925826289068,1.,0.965925826289068,1.,0.965925826289068,
1.,0.965925826289068,1.,0.965925826289068,1.,0.965925826289068,1.,0.965925826289068,
1.,0.965925826289068,1.,0.965925826289068,1.,0.965925826289068,1.,0.965925826289068,
1.,0.965925826289068,1.,0.965925826289068,1.,0.965925826289068,1.,0.965925826289068,
1.,0.965925826289068,1.,0.965925826289068,1.,0.965925826289068,1.,0.965925826289068,
1.,0.965925826289068,1.,0.965925826289068,1.,0.965925826289068,1.,0.965925826289068,
1.,0.965925826289068,1.,0.965925826289068,1.,0.965925826289068,1.,0.965925826289068,
1.,0.965925826289068,1.,0.965925826289068,1.,0.965925826289068,1.,0.965925826289068,
1.,0.965925826289068,1.,0.965925826289068,1.,0.965925826289068,1.,0.965925826289068,
1.,0.965925826289068,1.,0.965925826289068,1.,0.965925826289068,1.,0.965925826289068,
1.,0.965925826289068,1.,0.965925826289068,1.,0.965925826289068,1.,0.965925826289068,
1.,0.965925826289068,1.,0.965925826289068,1.,0.965925826289068,1.,0.965925826289068,
1.,0.965925826289068,1.,0.965925826289068,1.,0.965925826289068,1.,0.965925826289068,
1.,0.965925826289068,1.,0.965925826289068,1.,0.965925826289068,1.,0.965925826289068,
1.,0.965925826289068,1.,0.965925826289068,1.,0.965925826289068,1.)))
REPRESENTATION_ITEM('')
SURFACE()
);
#158=(
BOUNDED_SURFACE()
B_SPLINE_SURFACE(1,2,((#7406,#7407,#7408,#7409,#7410,#7411,#7412,#7413,
#7414,#7415,#7416,#7417,#7418,#7419,#7420,#7421,#7422,#7423,#7424,#7425,
#7426,#7427,#7428,#7429,#7430,#7431,#7432,#7433,#7434,#7435,#7436,#7437,
#7438,#7439,#7440,#7441,#7442,#7443,#7444,#7445,#7446,#7447,#7448,#7449,
#7450,#7451,#7452,#7453,#7454,#7455,#7456,#7457,#7458,#7459,#7460,#7461,
#7462,#7463,#7464,#7465,#7466,#7467,#7468,#7469,#7470,#7471,#7472,#7473,
#7474,#7475,#7476,#7477,#7478,#7479,#7480,#7481,#7482,#7483,#7484,#7485,
#7486,#7487,#7488,#7489,#7490,#7491,#7492,#7493,#7494,#7495,#7496,#7497,
#7498,#7499,#7500,#7501,#7502,#7503,#7504,#7505,#7506,#7507,#7508,#7509,
#7510,#7511,#7512,#7513,#7514,#7515,#7516,#7517,#7518,#7519,#7520,#7521,
#7522,#7523,#7524,#7525,#7526,#7527,#7528,#7529,#7530,#7531,#7532,#7533,
#7534,#7535,#7536,#7537,#7538,#7539,#7540,#7541,#7542,#7543,#7544,#7545,
#7546,#7547,#7548,#7549,#7550),(#7551,#7552,#7553,#7554,#7555,#7556,#7557,
#7558,#7559,#7560,#7561,#7562,#7563,#7564,#7565,#7566,#7567,#7568,#7569,
#7570,#7571,#7572,#7573,#7574,#7575,#7576,#7577,#7578,#7579,#7580,#7581,
#7582,#7583,#7584,#7585,#7586,#7587,#7588,#7589,#7590,#7591,#7592,#7593,
#7594,#7595,#7596,#7597,#7598,#7599,#7600,#7601,#7602,#7603,#7604,#7605,
#7606,#7607,#7608,#7609,#7610,#7611,#7612,#7613,#7614,#7615,#7616,#7617,
#7618,#7619,#7620,#7621,#7622,#7623,#7624,#7625,#7626,#7627,#7628,#7629,
#7630,#7631,#7632,#7633,#7634,#7635,#7636,#7637,#7638,#7639,#7640,#7641,
#7642,#7643,#7644,#7645,#7646,#7647,#7648,#7649,#7650,#7651,#7652,#7653,
#7654,#7655,#7656,#7657,#7658,#7659,#7660,#7661,#7662,#7663,#7664,#7665,
#7666,#7667,#7668,#7669,#7670,#7671,#7672,#7673,#7674,#7675,#7676,#7677,
#7678,#7679,#7680,#7681,#7682,#7683,#7684,#7685,#7686,#7687,#7688,#7689,
#7690,#7691,#7692,#7693,#7694,#7695)),.UNSPECIFIED.,.F.,.F.,.F.)
B_SPLINE_SURFACE_WITH_KNOTS((2,2),(3,2,2,2,2,2,2,2,2,2,2,2,2,2,2,2,2,2,
2,2,2,2,2,2,2,2,2,2,2,2,2,2,2,2,2,2,2,2,2,2,2,2,2,2,2,2,2,2,2,2,2,2,2,2,
2,2,2,2,2,2,2,2,2,2,2,2,2,2,2,2,2,2,3),(0.,1.),(0.,0.0138888888888889,0.0277777777777778,
0.0416666666666667,0.0555555555555556,0.0694444444444444,0.0833333333333333,
0.0972222222222222,0.111111111111111,0.125,0.138888888888889,0.152777777777778,
0.166666666666667,0.180555555555556,0.194444444444444,0.208333333333333,
0.222222222222222,0.236111111111111,0.25,0.263888888888889,0.277777777777778,
0.291666666666667,0.305555555555556,0.319444444444444,0.333333333333333,
0.347222222222222,0.361111111111111,0.375,0.388888888888889,0.402777777777778,
0.416666666666667,0.430555555555556,0.444444444444444,0.458333333333333,
0.472222222222222,0.486111111111111,0.5,0.513888888888889,0.527777777777778,
0.541666666666667,0.555555555555556,0.569444444444444,0.583333333333333,
0.597222222222222,0.611111111111111,0.625,0.638888888888889,0.652777777777778,
0.666666666666667,0.680555555555556,0.694444444444444,0.708333333333333,
0.722222222222222,0.736111111111111,0.75,0.763888888888889,0.777777777777778,
0.791666666666667,0.805555555555556,0.819444444444444,0.833333333333333,
0.847222222222222,0.861111111111111,0.875,0.888888888888889,0.902777777777778,
0.916666666666667,0.930555555555556,0.944444444444444,0.958333333333333,
0.972222222222222,0.986111111111111,1.),.UNSPECIFIED.)
GEOMETRIC_REPRESENTATION_ITEM()
RATIONAL_B_SPLINE_SURFACE(((1.,0.965925826289068,1.,0.965925826289068,1.,
0.965925826289068,1.,0.965925826289068,1.,0.965925826289068,1.,0.965925826289068,
1.,0.965925826289068,1.,0.965925826289068,1.,0.965925826289068,1.,0.965925826289068,
1.,0.965925826289068,1.,0.965925826289068,1.,0.965925826289068,1.,0.965925826289068,
1.,0.965925826289068,1.,0.965925826289068,1.,0.965925826289068,1.,0.965925826289068,
1.,0.965925826289068,1.,0.965925826289068,1.,0.965925826289068,1.,0.965925826289068,
1.,0.965925826289068,1.,0.965925826289068,1.,0.965925826289068,1.,0.965925826289068,
1.,0.965925826289068,1.,0.965925826289068,1.,0.965925826289068,1.,0.965925826289068,
1.,0.965925826289068,1.,0.965925826289068,1.,0.965925826289068,1.,0.965925826289068,
1.,0.965925826289068,1.,0.965925826289068,1.,0.965925826289068,1.,0.965925826289068,
1.,0.965925826289068,1.,0.965925826289068,1.,0.965925826289068,1.,0.965925826289068,
1.,0.965925826289068,1.,0.965925826289068,1.,0.965925826289068,1.,0.965925826289068,
1.,0.965925826289068,1.,0.965925826289068,1.,0.965925826289068,1.,0.965925826289068,
1.,0.965925826289068,1.,0.965925826289068,1.,0.965925826289068,1.,0.965925826289068,
1.,0.965925826289068,1.,0.965925826289068,1.,0.965925826289068,1.,0.965925826289068,
1.,0.965925826289068,1.,0.965925826289068,1.,0.965925826289068,1.,0.965925826289068,
1.,0.965925826289068,1.,0.965925826289068,1.,0.965925826289068,1.,0.965925826289068,
1.,0.965925826289068,1.,0.965925826289068,1.,0.965925826289068,1.,0.965925826289068,
1.,0.965925826289068,1.,0.965925826289068,1.),(1.,0.965925826289068,1.,
0.965925826289068,1.,0.965925826289068,1.,0.965925826289068,1.,0.965925826289068,
1.,0.965925826289068,1.,0.965925826289068,1.,0.965925826289068,1.,0.965925826289068,
1.,0.965925826289068,1.,0.965925826289068,1.,0.965925826289068,1.,0.965925826289068,
1.,0.965925826289068,1.,0.965925826289068,1.,0.965925826289068,1.,0.965925826289068,
1.,0.965925826289068,1.,0.965925826289068,1.,0.965925826289068,1.,0.965925826289068,
1.,0.965925826289068,1.,0.965925826289068,1.,0.965925826289068,1.,0.965925826289068,
1.,0.965925826289068,1.,0.965925826289068,1.,0.965925826289068,1.,0.965925826289068,
1.,0.965925826289068,1.,0.965925826289068,1.,0.965925826289068,1.,0.965925826289068,
1.,0.965925826289068,1.,0.965925826289068,1.,0.965925826289068,1.,0.965925826289068,
1.,0.965925826289068,1.,0.965925826289068,1.,0.965925826289068,1.,0.965925826289068,
1.,0.965925826289068,1.,0.965925826289068,1.,0.965925826289068,1.,0.965925826289068,
1.,0.965925826289068,1.,0.965925826289068,1.,0.965925826289068,1.,0.965925826289068,
1.,0.965925826289068,1.,0.965925826289068,1.,0.965925826289068,1.,0.965925826289068,
1.,0.965925826289068,1.,0.965925826289068,1.,0.965925826289068,1.,0.965925826289068,
1.,0.965925826289068,1.,0.965925826289068,1.,0.965925826289068,1.,0.965925826289068,
1.,0.965925826289068,1.,0.965925826289068,1.,0.965925826289068,1.,0.965925826289068,
1.,0.965925826289068,1.,0.965925826289068,1.,0.965925826289068,1.,0.965925826289068,
1.,0.965925826289068,1.,0.965925826289068,1.,0.965925826289068,1.)))
REPRESENTATION_ITEM('')
SURFACE()
);
#159=(
BOUNDED_SURFACE()
B_SPLINE_SURFACE(1,2,((#7713,#7714,#7715,#7716,#7717,#7718,#7719,#7720,
#7721,#7722,#7723,#7724,#7725,#7726,#7727,#7728,#7729,#7730,#7731,#7732,
#7733,#7734,#7735,#7736,#7737,#7738,#7739,#7740,#7741,#7742,#7743,#7744,
#7745,#7746,#7747,#7748,#7749,#7750,#7751,#7752,#7753,#7754,#7755,#7756,
#7757,#7758,#7759,#7760,#7761,#7762,#7763,#7764,#7765,#7766,#7767,#7768,
#7769,#7770,#7771,#7772,#7773,#7774,#7775,#7776,#7777,#7778,#7779,#7780,
#7781,#7782,#7783,#7784,#7785,#7786,#7787,#7788,#7789,#7790,#7791,#7792,
#7793,#7794,#7795,#7796,#7797,#7798,#7799,#7800,#7801,#7802,#7803,#7804,
#7805,#7806,#7807,#7808,#7809,#7810,#7811,#7812,#7813,#7814,#7815,#7816,
#7817,#7818,#7819,#7820,#7821,#7822,#7823,#7824,#7825,#7826,#7827,#7828,
#7829,#7830,#7831,#7832,#7833,#7834,#7835,#7836,#7837,#7838,#7839,#7840,
#7841,#7842,#7843,#7844,#7845,#7846,#7847,#7848,#7849,#7850,#7851,#7852,
#7853,#7854,#7855,#7856,#7857),(#7858,#7859,#7860,#7861,#7862,#7863,#7864,
#7865,#7866,#7867,#7868,#7869,#7870,#7871,#7872,#7873,#7874,#7875,#7876,
#7877,#7878,#7879,#7880,#7881,#7882,#7883,#7884,#7885,#7886,#7887,#7888,
#7889,#7890,#7891,#7892,#7893,#7894,#7895,#7896,#7897,#7898,#7899,#7900,
#7901,#7902,#7903,#7904,#7905,#7906,#7907,#7908,#7909,#7910,#7911,#7912,
#7913,#7914,#7915,#7916,#7917,#7918,#7919,#7920,#7921,#7922,#7923,#7924,
#7925,#7926,#7927,#7928,#7929,#7930,#7931,#7932,#7933,#7934,#7935,#7936,
#7937,#7938,#7939,#7940,#7941,#7942,#7943,#7944,#7945,#7946,#7947,#7948,
#7949,#7950,#7951,#7952,#7953,#7954,#7955,#7956,#7957,#7958,#7959,#7960,
#7961,#7962,#7963,#7964,#7965,#7966,#7967,#7968,#7969,#7970,#7971,#7972,
#7973,#7974,#7975,#7976,#7977,#7978,#7979,#7980,#7981,#7982,#7983,#7984,
#7985,#7986,#7987,#7988,#7989,#7990,#7991,#7992,#7993,#7994,#7995,#7996,
#7997,#7998,#7999,#8000,#8001,#8002)),.UNSPECIFIED.,.F.,.F.,.F.)
B_SPLINE_SURFACE_WITH_KNOTS((2,2),(3,2,2,2,2,2,2,2,2,2,2,2,2,2,2,2,2,2,
2,2,2,2,2,2,2,2,2,2,2,2,2,2,2,2,2,2,2,2,2,2,2,2,2,2,2,2,2,2,2,2,2,2,2,2,
2,2,2,2,2,2,2,2,2,2,2,2,2,2,2,2,2,2,3),(0.,1.),(0.,0.0138888888888889,0.0277777777777778,
0.0416666666666667,0.0555555555555556,0.0694444444444444,0.0833333333333333,
0.0972222222222222,0.111111111111111,0.125,0.138888888888889,0.152777777777778,
0.166666666666667,0.180555555555556,0.194444444444444,0.208333333333333,
0.222222222222222,0.236111111111111,0.25,0.263888888888889,0.277777777777778,
0.291666666666667,0.305555555555556,0.319444444444444,0.333333333333333,
0.347222222222222,0.361111111111111,0.375,0.388888888888889,0.402777777777778,
0.416666666666667,0.430555555555556,0.444444444444444,0.458333333333333,
0.472222222222222,0.486111111111111,0.5,0.513888888888889,0.527777777777778,
0.541666666666667,0.555555555555556,0.569444444444444,0.583333333333333,
0.597222222222222,0.611111111111111,0.625,0.638888888888889,0.652777777777778,
0.666666666666667,0.680555555555556,0.694444444444444,0.708333333333333,
0.722222222222222,0.736111111111111,0.75,0.763888888888889,0.777777777777778,
0.791666666666667,0.805555555555556,0.819444444444444,0.833333333333333,
0.847222222222222,0.861111111111111,0.875,0.888888888888889,0.902777777777778,
0.916666666666667,0.930555555555556,0.944444444444444,0.958333333333333,
0.972222222222222,0.986111111111111,1.),.UNSPECIFIED.)
GEOMETRIC_REPRESENTATION_ITEM()
RATIONAL_B_SPLINE_SURFACE(((1.,0.965925826289068,1.,0.965925826289068,1.,
0.965925826289068,1.,0.965925826289068,1.,0.965925826289068,1.,0.965925826289068,
1.,0.965925826289068,1.,0.965925826289068,1.,0.965925826289068,1.,0.965925826289068,
1.,0.965925826289068,1.,0.965925826289068,1.,0.965925826289068,1.,0.965925826289068,
1.,0.965925826289068,1.,0.965925826289068,1.,0.965925826289068,1.,0.965925826289068,
1.,0.965925826289068,1.,0.965925826289068,1.,0.965925826289068,1.,0.965925826289068,
1.,0.965925826289068,1.,0.965925826289068,1.,0.965925826289068,1.,0.965925826289068,
1.,0.965925826289068,1.,0.965925826289068,1.,0.965925826289068,1.,0.965925826289068,
1.,0.965925826289068,1.,0.965925826289068,1.,0.965925826289068,1.,0.965925826289068,
1.,0.965925826289068,1.,0.965925826289068,1.,0.965925826289068,1.,0.965925826289068,
1.,0.965925826289068,1.,0.965925826289068,1.,0.965925826289068,1.,0.965925826289068,
1.,0.965925826289068,1.,0.965925826289068,1.,0.965925826289068,1.,0.965925826289068,
1.,0.965925826289068,1.,0.965925826289068,1.,0.965925826289068,1.,0.965925826289068,
1.,0.965925826289068,1.,0.965925826289068,1.,0.965925826289068,1.,0.965925826289068,
1.,0.965925826289068,1.,0.965925826289068,1.,0.965925826289068,1.,0.965925826289068,
1.,0.965925826289068,1.,0.965925826289068,1.,0.965925826289068,1.,0.965925826289068,
1.,0.965925826289068,1.,0.965925826289068,1.,0.965925826289068,1.,0.965925826289068,
1.,0.965925826289068,1.,0.965925826289068,1.,0.965925826289068,1.,0.965925826289068,
1.,0.965925826289068,1.,0.965925826289068,1.),(1.,0.965925826289068,1.,
0.965925826289068,1.,0.965925826289068,1.,0.965925826289068,1.,0.965925826289068,
1.,0.965925826289068,1.,0.965925826289068,1.,0.965925826289068,1.,0.965925826289068,
1.,0.965925826289068,1.,0.965925826289068,1.,0.965925826289068,1.,0.965925826289068,
1.,0.965925826289068,1.,0.965925826289068,1.,0.965925826289068,1.,0.965925826289068,
1.,0.965925826289068,1.,0.965925826289068,1.,0.965925826289068,1.,0.965925826289068,
1.,0.965925826289068,1.,0.965925826289068,1.,0.965925826289068,1.,0.965925826289068,
1.,0.965925826289068,1.,0.965925826289068,1.,0.965925826289068,1.,0.965925826289068,
1.,0.965925826289068,1.,0.965925826289068,1.,0.965925826289068,1.,0.965925826289068,
1.,0.965925826289068,1.,0.965925826289068,1.,0.965925826289068,1.,0.965925826289068,
1.,0.965925826289068,1.,0.965925826289068,1.,0.965925826289068,1.,0.965925826289068,
1.,0.965925826289068,1.,0.965925826289068,1.,0.965925826289068,1.,0.965925826289068,
1.,0.965925826289068,1.,0.965925826289068,1.,0.965925826289068,1.,0.965925826289068,
1.,0.965925826289068,1.,0.965925826289068,1.,0.965925826289068,1.,0.965925826289068,
1.,0.965925826289068,1.,0.965925826289068,1.,0.965925826289068,1.,0.965925826289068,
1.,0.965925826289068,1.,0.965925826289068,1.,0.965925826289068,1.,0.965925826289068,
1.,0.965925826289068,1.,0.965925826289068,1.,0.965925826289068,1.,0.965925826289068,
1.,0.965925826289068,1.,0.965925826289068,1.,0.965925826289068,1.,0.965925826289068,
1.,0.965925826289068,1.,0.965925826289068,1.,0.965925826289068,1.)))
REPRESENTATION_ITEM('')
SURFACE()
);
#160=(
BOUNDED_SURFACE()
B_SPLINE_SURFACE(1,2,((#8031,#8032,#8033,#8034,#8035,#8036,#8037,#8038,
#8039,#8040,#8041,#8042,#8043,#8044,#8045,#8046,#8047,#8048,#8049,#8050,
#8051,#8052,#8053,#8054,#8055,#8056,#8057,#8058,#8059,#8060,#8061,#8062,
#8063,#8064,#8065,#8066,#8067,#8068,#8069,#8070,#8071,#8072,#8073,#8074,
#8075,#8076,#8077,#8078,#8079,#8080,#8081,#8082,#8083,#8084,#8085,#8086,
#8087,#8088,#8089,#8090,#8091,#8092,#8093,#8094,#8095,#8096,#8097,#8098,
#8099,#8100,#8101,#8102,#8103,#8104,#8105,#8106,#8107,#8108,#8109,#8110,
#8111,#8112,#8113,#8114,#8115,#8116,#8117,#8118,#8119,#8120,#8121,#8122,
#8123,#8124,#8125,#8126,#8127,#8128,#8129,#8130,#8131,#8132,#8133,#8134,
#8135,#8136,#8137,#8138,#8139,#8140,#8141,#8142,#8143,#8144,#8145,#8146,
#8147,#8148,#8149,#8150,#8151,#8152,#8153,#8154,#8155,#8156,#8157,#8158,
#8159,#8160,#8161,#8162,#8163,#8164,#8165,#8166,#8167,#8168,#8169,#8170,
#8171,#8172,#8173,#8174,#8175),(#8176,#8177,#8178,#8179,#8180,#8181,#8182,
#8183,#8184,#8185,#8186,#8187,#8188,#8189,#8190,#8191,#8192,#8193,#8194,
#8195,#8196,#8197,#8198,#8199,#8200,#8201,#8202,#8203,#8204,#8205,#8206,
#8207,#8208,#8209,#8210,#8211,#8212,#8213,#8214,#8215,#8216,#8217,#8218,
#8219,#8220,#8221,#8222,#8223,#8224,#8225,#8226,#8227,#8228,#8229,#8230,
#8231,#8232,#8233,#8234,#8235,#8236,#8237,#8238,#8239,#8240,#8241,#8242,
#8243,#8244,#8245,#8246,#8247,#8248,#8249,#8250,#8251,#8252,#8253,#8254,
#8255,#8256,#8257,#8258,#8259,#8260,#8261,#8262,#8263,#8264,#8265,#8266,
#8267,#8268,#8269,#8270,#8271,#8272,#8273,#8274,#8275,#8276,#8277,#8278,
#8279,#8280,#8281,#8282,#8283,#8284,#8285,#8286,#8287,#8288,#8289,#8290,
#8291,#8292,#8293,#8294,#8295,#8296,#8297,#8298,#8299,#8300,#8301,#8302,
#8303,#8304,#8305,#8306,#8307,#8308,#8309,#8310,#8311,#8312,#8313,#8314,
#8315,#8316,#8317,#8318,#8319,#8320)),.UNSPECIFIED.,.F.,.F.,.F.)
B_SPLINE_SURFACE_WITH_KNOTS((2,2),(3,2,2,2,2,2,2,2,2,2,2,2,2,2,2,2,2,2,
2,2,2,2,2,2,2,2,2,2,2,2,2,2,2,2,2,2,2,2,2,2,2,2,2,2,2,2,2,2,2,2,2,2,2,2,
2,2,2,2,2,2,2,2,2,2,2,2,2,2,2,2,2,2,3),(0.,1.),(0.,0.0138888888888889,0.0277777777777778,
0.0416666666666667,0.0555555555555556,0.0694444444444444,0.0833333333333333,
0.0972222222222222,0.111111111111111,0.125,0.138888888888889,0.152777777777778,
0.166666666666667,0.180555555555556,0.194444444444444,0.208333333333333,
0.222222222222222,0.236111111111111,0.25,0.263888888888889,0.277777777777778,
0.291666666666667,0.305555555555556,0.319444444444444,0.333333333333333,
0.347222222222222,0.361111111111111,0.375,0.388888888888889,0.402777777777778,
0.416666666666667,0.430555555555556,0.444444444444444,0.458333333333333,
0.472222222222222,0.486111111111111,0.5,0.513888888888889,0.527777777777778,
0.541666666666667,0.555555555555556,0.569444444444444,0.583333333333333,
0.597222222222222,0.611111111111111,0.625,0.638888888888889,0.652777777777778,
0.666666666666667,0.680555555555556,0.694444444444444,0.708333333333333,
0.722222222222222,0.736111111111111,0.75,0.763888888888889,0.777777777777778,
0.791666666666667,0.805555555555556,0.819444444444444,0.833333333333333,
0.847222222222222,0.861111111111111,0.875,0.888888888888889,0.902777777777778,
0.916666666666667,0.930555555555556,0.944444444444444,0.958333333333333,
0.972222222222222,0.986111111111111,1.),.UNSPECIFIED.)
GEOMETRIC_REPRESENTATION_ITEM()
RATIONAL_B_SPLINE_SURFACE(((1.,0.965925826289068,1.,0.965925826289068,1.,
0.965925826289068,1.,0.965925826289068,1.,0.965925826289068,1.,0.965925826289068,
1.,0.965925826289068,1.,0.965925826289068,1.,0.965925826289068,1.,0.965925826289068,
1.,0.965925826289068,1.,0.965925826289068,1.,0.965925826289068,1.,0.965925826289068,
1.,0.965925826289068,1.,0.965925826289068,1.,0.965925826289068,1.,0.965925826289068,
1.,0.965925826289068,1.,0.965925826289068,1.,0.965925826289068,1.,0.965925826289068,
1.,0.965925826289068,1.,0.965925826289068,1.,0.965925826289068,1.,0.965925826289068,
1.,0.965925826289068,1.,0.965925826289068,1.,0.965925826289068,1.,0.965925826289068,
1.,0.965925826289068,1.,0.965925826289068,1.,0.965925826289068,1.,0.965925826289068,
1.,0.965925826289068,1.,0.965925826289068,1.,0.965925826289068,1.,0.965925826289068,
1.,0.965925826289068,1.,0.965925826289068,1.,0.965925826289068,1.,0.965925826289068,
1.,0.965925826289068,1.,0.965925826289068,1.,0.965925826289068,1.,0.965925826289068,
1.,0.965925826289068,1.,0.965925826289068,1.,0.965925826289068,1.,0.965925826289068,
1.,0.965925826289068,1.,0.965925826289068,1.,0.965925826289068,1.,0.965925826289068,
1.,0.965925826289068,1.,0.965925826289068,1.,0.965925826289068,1.,0.965925826289068,
1.,0.965925826289068,1.,0.965925826289068,1.,0.965925826289068,1.,0.965925826289068,
1.,0.965925826289068,1.,0.965925826289068,1.,0.965925826289068,1.,0.965925826289068,
1.,0.965925826289068,1.,0.965925826289068,1.,0.965925826289068,1.,0.965925826289068,
1.,0.965925826289068,1.,0.965925826289068,1.),(1.,0.965925826289068,1.,
0.965925826289068,1.,0.965925826289068,1.,0.965925826289068,1.,0.965925826289068,
1.,0.965925826289068,1.,0.965925826289068,1.,0.965925826289068,1.,0.965925826289068,
1.,0.965925826289068,1.,0.965925826289068,1.,0.965925826289068,1.,0.965925826289068,
1.,0.965925826289068,1.,0.965925826289068,1.,0.965925826289068,1.,0.965925826289068,
1.,0.965925826289068,1.,0.965925826289068,1.,0.965925826289068,1.,0.965925826289068,
1.,0.965925826289068,1.,0.965925826289068,1.,0.965925826289068,1.,0.965925826289068,
1.,0.965925826289068,1.,0.965925826289068,1.,0.965925826289068,1.,0.965925826289068,
1.,0.965925826289068,1.,0.965925826289068,1.,0.965925826289068,1.,0.965925826289068,
1.,0.965925826289068,1.,0.965925826289068,1.,0.965925826289068,1.,0.965925826289068,
1.,0.965925826289068,1.,0.965925826289068,1.,0.965925826289068,1.,0.965925826289068,
1.,0.965925826289068,1.,0.965925826289068,1.,0.965925826289068,1.,0.965925826289068,
1.,0.965925826289068,1.,0.965925826289068,1.,0.965925826289068,1.,0.965925826289068,
1.,0.965925826289068,1.,0.965925826289068,1.,0.965925826289068,1.,0.965925826289068,
1.,0.965925826289068,1.,0.965925826289068,1.,0.965925826289068,1.,0.965925826289068,
1.,0.965925826289068,1.,0.965925826289068,1.,0.965925826289068,1.,0.965925826289068,
1.,0.965925826289068,1.,0.965925826289068,1.,0.965925826289068,1.,0.965925826289068,
1.,0.965925826289068,1.,0.965925826289068,1.,0.965925826289068,1.,0.965925826289068,
1.,0.965925826289068,1.,0.965925826289068,1.,0.965925826289068,1.)))
REPRESENTATION_ITEM('')
SURFACE()
);
#161=(
BOUNDED_SURFACE()
B_SPLINE_SURFACE(1,2,((#8344,#8345,#8346,#8347,#8348,#8349,#8350,#8351,
#8352,#8353,#8354,#8355,#8356,#8357,#8358,#8359,#8360,#8361,#8362,#8363,
#8364,#8365,#8366,#8367,#8368,#8369,#8370,#8371,#8372,#8373,#8374,#8375,
#8376,#8377,#8378,#8379,#8380,#8381,#8382,#8383,#8384,#8385,#8386,#8387,
#8388,#8389,#8390,#8391,#8392,#8393,#8394,#8395,#8396,#8397,#8398,#8399,
#8400,#8401,#8402,#8403,#8404,#8405,#8406,#8407,#8408,#8409,#8410,#8411,
#8412,#8413,#8414,#8415,#8416,#8417,#8418,#8419,#8420,#8421,#8422,#8423,
#8424,#8425,#8426,#8427,#8428,#8429,#8430,#8431,#8432,#8433,#8434,#8435,
#8436,#8437,#8438,#8439,#8440,#8441,#8442,#8443,#8444,#8445,#8446,#8447,
#8448,#8449,#8450,#8451,#8452,#8453,#8454,#8455,#8456,#8457,#8458,#8459,
#8460,#8461,#8462,#8463,#8464,#8465,#8466,#8467,#8468,#8469,#8470,#8471,
#8472,#8473,#8474,#8475,#8476,#8477,#8478,#8479,#8480,#8481,#8482,#8483,
#8484,#8485,#8486,#8487,#8488),(#8489,#8490,#8491,#8492,#8493,#8494,#8495,
#8496,#8497,#8498,#8499,#8500,#8501,#8502,#8503,#8504,#8505,#8506,#8507,
#8508,#8509,#8510,#8511,#8512,#8513,#8514,#8515,#8516,#8517,#8518,#8519,
#8520,#8521,#8522,#8523,#8524,#8525,#8526,#8527,#8528,#8529,#8530,#8531,
#8532,#8533,#8534,#8535,#8536,#8537,#8538,#8539,#8540,#8541,#8542,#8543,
#8544,#8545,#8546,#8547,#8548,#8549,#8550,#8551,#8552,#8553,#8554,#8555,
#8556,#8557,#8558,#8559,#8560,#8561,#8562,#8563,#8564,#8565,#8566,#8567,
#8568,#8569,#8570,#8571,#8572,#8573,#8574,#8575,#8576,#8577,#8578,#8579,
#8580,#8581,#8582,#8583,#8584,#8585,#8586,#8587,#8588,#8589,#8590,#8591,
#8592,#8593,#8594,#8595,#8596,#8597,#8598,#8599,#8600,#8601,#8602,#8603,
#8604,#8605,#8606,#8607,#8608,#8609,#8610,#8611,#8612,#8613,#8614,#8615,
#8616,#8617,#8618,#8619,#8620,#8621,#8622,#8623,#8624,#8625,#8626,#8627,
#8628,#8629,#8630,#8631,#8632,#8633)),.UNSPECIFIED.,.F.,.F.,.F.)
B_SPLINE_SURFACE_WITH_KNOTS((2,2),(3,2,2,2,2,2,2,2,2,2,2,2,2,2,2,2,2,2,
2,2,2,2,2,2,2,2,2,2,2,2,2,2,2,2,2,2,2,2,2,2,2,2,2,2,2,2,2,2,2,2,2,2,2,2,
2,2,2,2,2,2,2,2,2,2,2,2,2,2,2,2,2,2,3),(0.,1.),(0.,0.0138888888888889,0.0277777777777778,
0.0416666666666667,0.0555555555555556,0.0694444444444444,0.0833333333333333,
0.0972222222222222,0.111111111111111,0.125,0.138888888888889,0.152777777777778,
0.166666666666667,0.180555555555556,0.194444444444444,0.208333333333333,
0.222222222222222,0.236111111111111,0.25,0.263888888888889,0.277777777777778,
0.291666666666667,0.305555555555556,0.319444444444444,0.333333333333333,
0.347222222222222,0.361111111111111,0.375,0.388888888888889,0.402777777777778,
0.416666666666667,0.430555555555556,0.444444444444444,0.458333333333333,
0.472222222222222,0.486111111111111,0.5,0.513888888888889,0.527777777777778,
0.541666666666667,0.555555555555556,0.569444444444444,0.583333333333333,
0.597222222222222,0.611111111111111,0.625,0.638888888888889,0.652777777777778,
0.666666666666667,0.680555555555556,0.694444444444444,0.708333333333333,
0.722222222222222,0.736111111111111,0.75,0.763888888888889,0.777777777777778,
0.791666666666667,0.805555555555556,0.819444444444444,0.833333333333333,
0.847222222222222,0.861111111111111,0.875,0.888888888888889,0.902777777777778,
0.916666666666667,0.930555555555556,0.944444444444444,0.958333333333333,
0.972222222222222,0.986111111111111,1.),.UNSPECIFIED.)
GEOMETRIC_REPRESENTATION_ITEM()
RATIONAL_B_SPLINE_SURFACE(((1.,0.965925826289068,1.,0.965925826289068,1.,
0.965925826289068,1.,0.965925826289068,1.,0.965925826289068,1.,0.965925826289068,
1.,0.965925826289068,1.,0.965925826289068,1.,0.965925826289068,1.,0.965925826289068,
1.,0.965925826289068,1.,0.965925826289068,1.,0.965925826289068,1.,0.965925826289068,
1.,0.965925826289068,1.,0.965925826289068,1.,0.965925826289068,1.,0.965925826289068,
1.,0.965925826289068,1.,0.965925826289068,1.,0.965925826289068,1.,0.965925826289068,
1.,0.965925826289068,1.,0.965925826289068,1.,0.965925826289068,1.,0.965925826289068,
1.,0.965925826289068,1.,0.965925826289068,1.,0.965925826289068,1.,0.965925826289068,
1.,0.965925826289068,1.,0.965925826289068,1.,0.965925826289068,1.,0.965925826289068,
1.,0.965925826289068,1.,0.965925826289068,1.,0.965925826289068,1.,0.965925826289068,
1.,0.965925826289068,1.,0.965925826289068,1.,0.965925826289068,1.,0.965925826289068,
1.,0.965925826289068,1.,0.965925826289068,1.,0.965925826289068,1.,0.965925826289068,
1.,0.965925826289068,1.,0.965925826289068,1.,0.965925826289068,1.,0.965925826289068,
1.,0.965925826289068,1.,0.965925826289068,1.,0.965925826289068,1.,0.965925826289068,
1.,0.965925826289068,1.,0.965925826289068,1.,0.965925826289068,1.,0.965925826289068,
1.,0.965925826289068,1.,0.965925826289068,1.,0.965925826289068,1.,0.965925826289068,
1.,0.965925826289068,1.,0.965925826289068,1.,0.965925826289068,1.,0.965925826289068,
1.,0.965925826289068,1.,0.965925826289068,1.,0.965925826289068,1.,0.965925826289068,
1.,0.965925826289068,1.,0.965925826289068,1.),(1.,0.965925826289068,1.,
0.965925826289068,1.,0.965925826289068,1.,0.965925826289068,1.,0.965925826289068,
1.,0.965925826289068,1.,0.965925826289068,1.,0.965925826289068,1.,0.965925826289068,
1.,0.965925826289068,1.,0.965925826289068,1.,0.965925826289068,1.,0.965925826289068,
1.,0.965925826289068,1.,0.965925826289068,1.,0.965925826289068,1.,0.965925826289068,
1.,0.965925826289068,1.,0.965925826289068,1.,0.965925826289068,1.,0.965925826289068,
1.,0.965925826289068,1.,0.965925826289068,1.,0.965925826289068,1.,0.965925826289068,
1.,0.965925826289068,1.,0.965925826289068,1.,0.965925826289068,1.,0.965925826289068,
1.,0.965925826289068,1.,0.965925826289068,1.,0.965925826289068,1.,0.965925826289068,
1.,0.965925826289068,1.,0.965925826289068,1.,0.965925826289068,1.,0.965925826289068,
1.,0.965925826289068,1.,0.965925826289068,1.,0.965925826289068,1.,0.965925826289068,
1.,0.965925826289068,1.,0.965925826289068,1.,0.965925826289068,1.,0.965925826289068,
1.,0.965925826289068,1.,0.965925826289068,1.,0.965925826289068,1.,0.965925826289068,
1.,0.965925826289068,1.,0.965925826289068,1.,0.965925826289068,1.,0.965925826289068,
1.,0.965925826289068,1.,0.965925826289068,1.,0.965925826289068,1.,0.965925826289068,
1.,0.965925826289068,1.,0.965925826289068,1.,0.965925826289068,1.,0.965925826289068,
1.,0.965925826289068,1.,0.965925826289068,1.,0.965925826289068,1.,0.965925826289068,
1.,0.965925826289068,1.,0.965925826289068,1.,0.965925826289068,1.,0.965925826289068,
1.,0.965925826289068,1.,0.965925826289068,1.,0.965925826289068,1.)))
REPRESENTATION_ITEM('')
SURFACE()
);
#162=(
BOUNDED_SURFACE()
B_SPLINE_SURFACE(1,2,((#8651,#8652,#8653,#8654,#8655,#8656,#8657,#8658,
#8659,#8660,#8661,#8662,#8663,#8664,#8665,#8666,#8667,#8668,#8669,#8670,
#8671,#8672,#8673,#8674,#8675,#8676,#8677,#8678,#8679,#8680,#8681,#8682,
#8683,#8684,#8685,#8686,#8687,#8688,#8689,#8690,#8691,#8692,#8693,#8694,
#8695,#8696,#8697,#8698,#8699,#8700,#8701,#8702,#8703,#8704,#8705,#8706,
#8707,#8708,#8709,#8710,#8711,#8712,#8713,#8714,#8715,#8716,#8717,#8718,
#8719,#8720,#8721,#8722,#8723,#8724,#8725,#8726,#8727,#8728,#8729,#8730,
#8731,#8732,#8733,#8734,#8735,#8736,#8737,#8738,#8739,#8740,#8741,#8742,
#8743,#8744,#8745,#8746,#8747,#8748,#8749,#8750,#8751,#8752,#8753,#8754,
#8755,#8756,#8757,#8758,#8759,#8760,#8761,#8762,#8763,#8764,#8765,#8766,
#8767,#8768,#8769,#8770,#8771,#8772,#8773,#8774,#8775,#8776,#8777,#8778,
#8779,#8780,#8781,#8782,#8783,#8784,#8785,#8786,#8787,#8788,#8789,#8790,
#8791,#8792,#8793,#8794,#8795),(#8796,#8797,#8798,#8799,#8800,#8801,#8802,
#8803,#8804,#8805,#8806,#8807,#8808,#8809,#8810,#8811,#8812,#8813,#8814,
#8815,#8816,#8817,#8818,#8819,#8820,#8821,#8822,#8823,#8824,#8825,#8826,
#8827,#8828,#8829,#8830,#8831,#8832,#8833,#8834,#8835,#8836,#8837,#8838,
#8839,#8840,#8841,#8842,#8843,#8844,#8845,#8846,#8847,#8848,#8849,#8850,
#8851,#8852,#8853,#8854,#8855,#8856,#8857,#8858,#8859,#8860,#8861,#8862,
#8863,#8864,#8865,#8866,#8867,#8868,#8869,#8870,#8871,#8872,#8873,#8874,
#8875,#8876,#8877,#8878,#8879,#8880,#8881,#8882,#8883,#8884,#8885,#8886,
#8887,#8888,#8889,#8890,#8891,#8892,#8893,#8894,#8895,#8896,#8897,#8898,
#8899,#8900,#8901,#8902,#8903,#8904,#8905,#8906,#8907,#8908,#8909,#8910,
#8911,#8912,#8913,#8914,#8915,#8916,#8917,#8918,#8919,#8920,#8921,#8922,
#8923,#8924,#8925,#8926,#8927,#8928,#8929,#8930,#8931,#8932,#8933,#8934,
#8935,#8936,#8937,#8938,#8939,#8940)),.UNSPECIFIED.,.F.,.F.,.F.)
B_SPLINE_SURFACE_WITH_KNOTS((2,2),(3,2,2,2,2,2,2,2,2,2,2,2,2,2,2,2,2,2,
2,2,2,2,2,2,2,2,2,2,2,2,2,2,2,2,2,2,2,2,2,2,2,2,2,2,2,2,2,2,2,2,2,2,2,2,
2,2,2,2,2,2,2,2,2,2,2,2,2,2,2,2,2,2,3),(0.,1.),(0.,0.0138888888888889,0.0277777777777778,
0.0416666666666667,0.0555555555555556,0.0694444444444444,0.0833333333333333,
0.0972222222222222,0.111111111111111,0.125,0.138888888888889,0.152777777777778,
0.166666666666667,0.180555555555556,0.194444444444444,0.208333333333333,
0.222222222222222,0.236111111111111,0.25,0.263888888888889,0.277777777777778,
0.291666666666667,0.305555555555556,0.319444444444444,0.333333333333333,
0.347222222222222,0.361111111111111,0.375,0.388888888888889,0.402777777777778,
0.416666666666667,0.430555555555556,0.444444444444444,0.458333333333333,
0.472222222222222,0.486111111111111,0.5,0.513888888888889,0.527777777777778,
0.541666666666667,0.555555555555556,0.569444444444444,0.583333333333333,
0.597222222222222,0.611111111111111,0.625,0.638888888888889,0.652777777777778,
0.666666666666667,0.680555555555556,0.694444444444444,0.708333333333333,
0.722222222222222,0.736111111111111,0.75,0.763888888888889,0.777777777777778,
0.791666666666667,0.805555555555556,0.819444444444444,0.833333333333333,
0.847222222222222,0.861111111111111,0.875,0.888888888888889,0.902777777777778,
0.916666666666667,0.930555555555556,0.944444444444444,0.958333333333333,
0.972222222222222,0.986111111111111,1.),.UNSPECIFIED.)
GEOMETRIC_REPRESENTATION_ITEM()
RATIONAL_B_SPLINE_SURFACE(((1.,0.965925826289068,1.,0.965925826289068,1.,
0.965925826289068,1.,0.965925826289068,1.,0.965925826289068,1.,0.965925826289068,
1.,0.965925826289068,1.,0.965925826289068,1.,0.965925826289068,1.,0.965925826289068,
1.,0.965925826289068,1.,0.965925826289068,1.,0.965925826289068,1.,0.965925826289068,
1.,0.965925826289068,1.,0.965925826289068,1.,0.965925826289068,1.,0.965925826289068,
1.,0.965925826289068,1.,0.965925826289068,1.,0.965925826289068,1.,0.965925826289068,
1.,0.965925826289068,1.,0.965925826289068,1.,0.965925826289068,1.,0.965925826289068,
1.,0.965925826289068,1.,0.965925826289068,1.,0.965925826289068,1.,0.965925826289068,
1.,0.965925826289068,1.,0.965925826289068,1.,0.965925826289068,1.,0.965925826289068,
1.,0.965925826289068,1.,0.965925826289068,1.,0.965925826289068,1.,0.965925826289068,
1.,0.965925826289068,1.,0.965925826289068,1.,0.965925826289068,1.,0.965925826289068,
1.,0.965925826289068,1.,0.965925826289068,1.,0.965925826289068,1.,0.965925826289068,
1.,0.965925826289068,1.,0.965925826289068,1.,0.965925826289068,1.,0.965925826289068,
1.,0.965925826289068,1.,0.965925826289068,1.,0.965925826289068,1.,0.965925826289068,
1.,0.965925826289068,1.,0.965925826289068,1.,0.965925826289068,1.,0.965925826289068,
1.,0.965925826289068,1.,0.965925826289068,1.,0.965925826289068,1.,0.965925826289068,
1.,0.965925826289068,1.,0.965925826289068,1.,0.965925826289068,1.,0.965925826289068,
1.,0.965925826289068,1.,0.965925826289068,1.,0.965925826289068,1.,0.965925826289068,
1.,0.965925826289068,1.,0.965925826289068,1.),(1.,0.965925826289068,1.,
0.965925826289068,1.,0.965925826289068,1.,0.965925826289068,1.,0.965925826289068,
1.,0.965925826289068,1.,0.965925826289068,1.,0.965925826289068,1.,0.965925826289068,
1.,0.965925826289068,1.,0.965925826289068,1.,0.965925826289068,1.,0.965925826289068,
1.,0.965925826289068,1.,0.965925826289068,1.,0.965925826289068,1.,0.965925826289068,
1.,0.965925826289068,1.,0.965925826289068,1.,0.965925826289068,1.,0.965925826289068,
1.,0.965925826289068,1.,0.965925826289068,1.,0.965925826289068,1.,0.965925826289068,
1.,0.965925826289068,1.,0.965925826289068,1.,0.965925826289068,1.,0.965925826289068,
1.,0.965925826289068,1.,0.965925826289068,1.,0.965925826289068,1.,0.965925826289068,
1.,0.965925826289068,1.,0.965925826289068,1.,0.965925826289068,1.,0.965925826289068,
1.,0.965925826289068,1.,0.965925826289068,1.,0.965925826289068,1.,0.965925826289068,
1.,0.965925826289068,1.,0.965925826289068,1.,0.965925826289068,1.,0.965925826289068,
1.,0.965925826289068,1.,0.965925826289068,1.,0.965925826289068,1.,0.965925826289068,
1.,0.965925826289068,1.,0.965925826289068,1.,0.965925826289068,1.,0.965925826289068,
1.,0.965925826289068,1.,0.965925826289068,1.,0.965925826289068,1.,0.965925826289068,
1.,0.965925826289068,1.,0.965925826289068,1.,0.965925826289068,1.,0.965925826289068,
1.,0.965925826289068,1.,0.965925826289068,1.,0.965925826289068,1.,0.965925826289068,
1.,0.965925826289068,1.,0.965925826289068,1.,0.965925826289068,1.,0.965925826289068,
1.,0.965925826289068,1.,0.965925826289068,1.,0.965925826289068,1.)))
REPRESENTATION_ITEM('')
SURFACE()
);
#163=(
BOUNDED_SURFACE()
B_SPLINE_SURFACE(1,2,((#8966,#8967,#8968,#8969,#8970,#8971,#8972,#8973,
#8974,#8975,#8976,#8977,#8978,#8979,#8980,#8981,#8982,#8983,#8984,#8985,
#8986,#8987,#8988,#8989,#8990,#8991,#8992,#8993,#8994,#8995,#8996,#8997,
#8998,#8999,#9000,#9001,#9002,#9003,#9004,#9005,#9006,#9007,#9008,#9009,
#9010,#9011,#9012,#9013,#9014,#9015,#9016,#9017,#9018,#9019,#9020,#9021,
#9022,#9023,#9024,#9025,#9026,#9027,#9028,#9029,#9030,#9031,#9032,#9033,
#9034,#9035,#9036,#9037,#9038,#9039,#9040,#9041,#9042,#9043,#9044,#9045,
#9046,#9047,#9048,#9049,#9050,#9051,#9052,#9053,#9054,#9055,#9056,#9057,
#9058,#9059,#9060,#9061,#9062,#9063,#9064,#9065,#9066,#9067,#9068,#9069,
#9070,#9071,#9072,#9073,#9074,#9075,#9076,#9077,#9078,#9079,#9080,#9081,
#9082,#9083,#9084,#9085,#9086,#9087,#9088,#9089,#9090,#9091,#9092,#9093,
#9094,#9095,#9096,#9097,#9098,#9099,#9100,#9101,#9102,#9103,#9104,#9105,
#9106,#9107,#9108,#9109,#9110),(#9111,#9112,#9113,#9114,#9115,#9116,#9117,
#9118,#9119,#9120,#9121,#9122,#9123,#9124,#9125,#9126,#9127,#9128,#9129,
#9130,#9131,#9132,#9133,#9134,#9135,#9136,#9137,#9138,#9139,#9140,#9141,
#9142,#9143,#9144,#9145,#9146,#9147,#9148,#9149,#9150,#9151,#9152,#9153,
#9154,#9155,#9156,#9157,#9158,#9159,#9160,#9161,#9162,#9163,#9164,#9165,
#9166,#9167,#9168,#9169,#9170,#9171,#9172,#9173,#9174,#9175,#9176,#9177,
#9178,#9179,#9180,#9181,#9182,#9183,#9184,#9185,#9186,#9187,#9188,#9189,
#9190,#9191,#9192,#9193,#9194,#9195,#9196,#9197,#9198,#9199,#9200,#9201,
#9202,#9203,#9204,#9205,#9206,#9207,#9208,#9209,#9210,#9211,#9212,#9213,
#9214,#9215,#9216,#9217,#9218,#9219,#9220,#9221,#9222,#9223,#9224,#9225,
#9226,#9227,#9228,#9229,#9230,#9231,#9232,#9233,#9234,#9235,#9236,#9237,
#9238,#9239,#9240,#9241,#9242,#9243,#9244,#9245,#9246,#9247,#9248,#9249,
#9250,#9251,#9252,#9253,#9254,#9255)),.UNSPECIFIED.,.F.,.F.,.F.)
B_SPLINE_SURFACE_WITH_KNOTS((2,2),(3,2,2,2,2,2,2,2,2,2,2,2,2,2,2,2,2,2,
2,2,2,2,2,2,2,2,2,2,2,2,2,2,2,2,2,2,2,2,2,2,2,2,2,2,2,2,2,2,2,2,2,2,2,2,
2,2,2,2,2,2,2,2,2,2,2,2,2,2,2,2,2,2,3),(0.,1.),(0.,0.0138888888888889,0.0277777777777778,
0.0416666666666667,0.0555555555555556,0.0694444444444444,0.0833333333333333,
0.0972222222222222,0.111111111111111,0.125,0.138888888888889,0.152777777777778,
0.166666666666667,0.180555555555556,0.194444444444444,0.208333333333333,
0.222222222222222,0.236111111111111,0.25,0.263888888888889,0.277777777777778,
0.291666666666667,0.305555555555556,0.319444444444444,0.333333333333333,
0.347222222222222,0.361111111111111,0.375,0.388888888888889,0.402777777777778,
0.416666666666667,0.430555555555556,0.444444444444444,0.458333333333333,
0.472222222222222,0.486111111111111,0.5,0.513888888888889,0.527777777777778,
0.541666666666667,0.555555555555556,0.569444444444444,0.583333333333333,
0.597222222222222,0.611111111111111,0.625,0.638888888888889,0.652777777777778,
0.666666666666667,0.680555555555556,0.694444444444444,0.708333333333333,
0.722222222222222,0.736111111111111,0.75,0.763888888888889,0.777777777777778,
0.791666666666667,0.805555555555556,0.819444444444444,0.833333333333333,
0.847222222222222,0.861111111111111,0.875,0.888888888888889,0.902777777777778,
0.916666666666667,0.930555555555556,0.944444444444444,0.958333333333333,
0.972222222222222,0.986111111111111,1.),.UNSPECIFIED.)
GEOMETRIC_REPRESENTATION_ITEM()
RATIONAL_B_SPLINE_SURFACE(((1.,0.965925826289068,1.,0.965925826289068,1.,
0.965925826289068,1.,0.965925826289068,1.,0.965925826289068,1.,0.965925826289068,
1.,0.965925826289068,1.,0.965925826289068,1.,0.965925826289068,1.,0.965925826289068,
1.,0.965925826289068,1.,0.965925826289068,1.,0.965925826289068,1.,0.965925826289068,
1.,0.965925826289068,1.,0.965925826289068,1.,0.965925826289068,1.,0.965925826289068,
1.,0.965925826289068,1.,0.965925826289068,1.,0.965925826289068,1.,0.965925826289068,
1.,0.965925826289068,1.,0.965925826289068,1.,0.965925826289068,1.,0.965925826289068,
1.,0.965925826289068,1.,0.965925826289068,1.,0.965925826289068,1.,0.965925826289068,
1.,0.965925826289068,1.,0.965925826289068,1.,0.965925826289068,1.,0.965925826289068,
1.,0.965925826289068,1.,0.965925826289068,1.,0.965925826289068,1.,0.965925826289068,
1.,0.965925826289068,1.,0.965925826289068,1.,0.965925826289068,1.,0.965925826289068,
1.,0.965925826289068,1.,0.965925826289068,1.,0.965925826289068,1.,0.965925826289068,
1.,0.965925826289068,1.,0.965925826289068,1.,0.965925826289068,1.,0.965925826289068,
1.,0.965925826289068,1.,0.965925826289068,1.,0.965925826289068,1.,0.965925826289068,
1.,0.965925826289068,1.,0.965925826289068,1.,0.965925826289068,1.,0.965925826289068,
1.,0.965925826289068,1.,0.965925826289068,1.,0.965925826289068,1.,0.965925826289068,
1.,0.965925826289068,1.,0.965925826289068,1.,0.965925826289068,1.,0.965925826289068,
1.,0.965925826289068,1.,0.965925826289068,1.,0.965925826289068,1.,0.965925826289068,
1.,0.965925826289068,1.,0.965925826289068,1.),(1.,0.965925826289068,1.,
0.965925826289068,1.,0.965925826289068,1.,0.965925826289068,1.,0.965925826289068,
1.,0.965925826289068,1.,0.965925826289068,1.,0.965925826289068,1.,0.965925826289068,
1.,0.965925826289068,1.,0.965925826289068,1.,0.965925826289068,1.,0.965925826289068,
1.,0.965925826289068,1.,0.965925826289068,1.,0.965925826289068,1.,0.965925826289068,
1.,0.965925826289068,1.,0.965925826289068,1.,0.965925826289068,1.,0.965925826289068,
1.,0.965925826289068,1.,0.965925826289068,1.,0.965925826289068,1.,0.965925826289068,
1.,0.965925826289068,1.,0.965925826289068,1.,0.965925826289068,1.,0.965925826289068,
1.,0.965925826289068,1.,0.965925826289068,1.,0.965925826289068,1.,0.965925826289068,
1.,0.965925826289068,1.,0.965925826289068,1.,0.965925826289068,1.,0.965925826289068,
1.,0.965925826289068,1.,0.965925826289068,1.,0.965925826289068,1.,0.965925826289068,
1.,0.965925826289068,1.,0.965925826289068,1.,0.965925826289068,1.,0.965925826289068,
1.,0.965925826289068,1.,0.965925826289068,1.,0.965925826289068,1.,0.965925826289068,
1.,0.965925826289068,1.,0.965925826289068,1.,0.965925826289068,1.,0.965925826289068,
1.,0.965925826289068,1.,0.965925826289068,1.,0.965925826289068,1.,0.965925826289068,
1.,0.965925826289068,1.,0.965925826289068,1.,0.965925826289068,1.,0.965925826289068,
1.,0.965925826289068,1.,0.965925826289068,1.,0.965925826289068,1.,0.965925826289068,
1.,0.965925826289068,1.,0.965925826289068,1.,0.965925826289068,1.,0.965925826289068,
1.,0.965925826289068,1.,0.965925826289068,1.,0.965925826289068,1.)))
REPRESENTATION_ITEM('')
SURFACE()
);
#164=(
BOUNDED_SURFACE()
B_SPLINE_SURFACE(1,2,((#9273,#9274,#9275,#9276,#9277,#9278,#9279,#9280,
#9281,#9282,#9283,#9284,#9285,#9286,#9287,#9288,#9289,#9290,#9291,#9292,
#9293,#9294,#9295,#9296,#9297,#9298,#9299,#9300,#9301,#9302,#9303,#9304,
#9305,#9306,#9307,#9308,#9309,#9310,#9311,#9312,#9313,#9314,#9315,#9316,
#9317,#9318,#9319,#9320,#9321,#9322,#9323,#9324,#9325,#9326,#9327,#9328,
#9329,#9330,#9331,#9332,#9333,#9334,#9335,#9336,#9337,#9338,#9339,#9340,
#9341,#9342,#9343,#9344,#9345,#9346,#9347,#9348,#9349,#9350,#9351,#9352,
#9353,#9354,#9355,#9356,#9357,#9358,#9359,#9360,#9361,#9362,#9363,#9364,
#9365,#9366,#9367,#9368,#9369,#9370,#9371,#9372,#9373,#9374,#9375,#9376,
#9377,#9378,#9379,#9380,#9381,#9382,#9383,#9384,#9385,#9386,#9387,#9388,
#9389,#9390,#9391,#9392,#9393,#9394,#9395,#9396,#9397,#9398,#9399,#9400,
#9401,#9402,#9403,#9404,#9405,#9406,#9407,#9408,#9409,#9410,#9411,#9412,
#9413,#9414,#9415,#9416,#9417),(#9418,#9419,#9420,#9421,#9422,#9423,#9424,
#9425,#9426,#9427,#9428,#9429,#9430,#9431,#9432,#9433,#9434,#9435,#9436,
#9437,#9438,#9439,#9440,#9441,#9442,#9443,#9444,#9445,#9446,#9447,#9448,
#9449,#9450,#9451,#9452,#9453,#9454,#9455,#9456,#9457,#9458,#9459,#9460,
#9461,#9462,#9463,#9464,#9465,#9466,#9467,#9468,#9469,#9470,#9471,#9472,
#9473,#9474,#9475,#9476,#9477,#9478,#9479,#9480,#9481,#9482,#9483,#9484,
#9485,#9486,#9487,#9488,#9489,#9490,#9491,#9492,#9493,#9494,#9495,#9496,
#9497,#9498,#9499,#9500,#9501,#9502,#9503,#9504,#9505,#9506,#9507,#9508,
#9509,#9510,#9511,#9512,#9513,#9514,#9515,#9516,#9517,#9518,#9519,#9520,
#9521,#9522,#9523,#9524,#9525,#9526,#9527,#9528,#9529,#9530,#9531,#9532,
#9533,#9534,#9535,#9536,#9537,#9538,#9539,#9540,#9541,#9542,#9543,#9544,
#9545,#9546,#9547,#9548,#9549,#9550,#9551,#9552,#9553,#9554,#9555,#9556,
#9557,#9558,#9559,#9560,#9561,#9562)),.UNSPECIFIED.,.F.,.F.,.F.)
B_SPLINE_SURFACE_WITH_KNOTS((2,2),(3,2,2,2,2,2,2,2,2,2,2,2,2,2,2,2,2,2,
2,2,2,2,2,2,2,2,2,2,2,2,2,2,2,2,2,2,2,2,2,2,2,2,2,2,2,2,2,2,2,2,2,2,2,2,
2,2,2,2,2,2,2,2,2,2,2,2,2,2,2,2,2,2,3),(0.,1.),(0.,0.0138888888888889,0.0277777777777778,
0.0416666666666667,0.0555555555555556,0.0694444444444444,0.0833333333333333,
0.0972222222222222,0.111111111111111,0.125,0.138888888888889,0.152777777777778,
0.166666666666667,0.180555555555556,0.194444444444444,0.208333333333333,
0.222222222222222,0.236111111111111,0.25,0.263888888888889,0.277777777777778,
0.291666666666667,0.305555555555556,0.319444444444444,0.333333333333333,
0.347222222222222,0.361111111111111,0.375,0.388888888888889,0.402777777777778,
0.416666666666667,0.430555555555556,0.444444444444444,0.458333333333333,
0.472222222222222,0.486111111111111,0.5,0.513888888888889,0.527777777777778,
0.541666666666667,0.555555555555556,0.569444444444444,0.583333333333333,
0.597222222222222,0.611111111111111,0.625,0.638888888888889,0.652777777777778,
0.666666666666667,0.680555555555556,0.694444444444444,0.708333333333333,
0.722222222222222,0.736111111111111,0.75,0.763888888888889,0.777777777777778,
0.791666666666667,0.805555555555556,0.819444444444444,0.833333333333333,
0.847222222222222,0.861111111111111,0.875,0.888888888888889,0.902777777777778,
0.916666666666667,0.930555555555556,0.944444444444444,0.958333333333333,
0.972222222222222,0.986111111111111,1.),.UNSPECIFIED.)
GEOMETRIC_REPRESENTATION_ITEM()
RATIONAL_B_SPLINE_SURFACE(((1.,0.965925826289068,1.,0.965925826289068,1.,
0.965925826289068,1.,0.965925826289068,1.,0.965925826289068,1.,0.965925826289068,
1.,0.965925826289068,1.,0.965925826289068,1.,0.965925826289068,1.,0.965925826289068,
1.,0.965925826289068,1.,0.965925826289068,1.,0.965925826289068,1.,0.965925826289068,
1.,0.965925826289068,1.,0.965925826289068,1.,0.965925826289068,1.,0.965925826289068,
1.,0.965925826289068,1.,0.965925826289068,1.,0.965925826289068,1.,0.965925826289068,
1.,0.965925826289068,1.,0.965925826289068,1.,0.965925826289068,1.,0.965925826289068,
1.,0.965925826289068,1.,0.965925826289068,1.,0.965925826289068,1.,0.965925826289068,
1.,0.965925826289068,1.,0.965925826289068,1.,0.965925826289068,1.,0.965925826289068,
1.,0.965925826289068,1.,0.965925826289068,1.,0.965925826289068,1.,0.965925826289068,
1.,0.965925826289068,1.,0.965925826289068,1.,0.965925826289068,1.,0.965925826289068,
1.,0.965925826289068,1.,0.965925826289068,1.,0.965925826289068,1.,0.965925826289068,
1.,0.965925826289068,1.,0.965925826289068,1.,0.965925826289068,1.,0.965925826289068,
1.,0.965925826289068,1.,0.965925826289068,1.,0.965925826289068,1.,0.965925826289068,
1.,0.965925826289068,1.,0.965925826289068,1.,0.965925826289068,1.,0.965925826289068,
1.,0.965925826289068,1.,0.965925826289068,1.,0.965925826289068,1.,0.965925826289068,
1.,0.965925826289068,1.,0.965925826289068,1.,0.965925826289068,1.,0.965925826289068,
1.,0.965925826289068,1.,0.965925826289068,1.,0.965925826289068,1.,0.965925826289068,
1.,0.965925826289068,1.,0.965925826289068,1.),(1.,0.965925826289068,1.,
0.965925826289068,1.,0.965925826289068,1.,0.965925826289068,1.,0.965925826289068,
1.,0.965925826289068,1.,0.965925826289068,1.,0.965925826289068,1.,0.965925826289068,
1.,0.965925826289068,1.,0.965925826289068,1.,0.965925826289068,1.,0.965925826289068,
1.,0.965925826289068,1.,0.965925826289068,1.,0.965925826289068,1.,0.965925826289068,
1.,0.965925826289068,1.,0.965925826289068,1.,0.965925826289068,1.,0.965925826289068,
1.,0.965925826289068,1.,0.965925826289068,1.,0.965925826289068,1.,0.965925826289068,
1.,0.965925826289068,1.,0.965925826289068,1.,0.965925826289068,1.,0.965925826289068,
1.,0.965925826289068,1.,0.965925826289068,1.,0.965925826289068,1.,0.965925826289068,
1.,0.965925826289068,1.,0.965925826289068,1.,0.965925826289068,1.,0.965925826289068,
1.,0.965925826289068,1.,0.965925826289068,1.,0.965925826289068,1.,0.965925826289068,
1.,0.965925826289068,1.,0.965925826289068,1.,0.965925826289068,1.,0.965925826289068,
1.,0.965925826289068,1.,0.965925826289068,1.,0.965925826289068,1.,0.965925826289068,
1.,0.965925826289068,1.,0.965925826289068,1.,0.965925826289068,1.,0.965925826289068,
1.,0.965925826289068,1.,0.965925826289068,1.,0.965925826289068,1.,0.965925826289068,
1.,0.965925826289068,1.,0.965925826289068,1.,0.965925826289068,1.,0.965925826289068,
1.,0.965925826289068,1.,0.965925826289068,1.,0.965925826289068,1.,0.965925826289068,
1.,0.965925826289068,1.,0.965925826289068,1.,0.965925826289068,1.,0.965925826289068,
1.,0.965925826289068,1.,0.965925826289068,1.,0.965925826289068,1.)))
REPRESENTATION_ITEM('')
SURFACE()
);
#165=(
BOUNDED_SURFACE()
B_SPLINE_SURFACE(1,2,((#9588,#9589,#9590,#9591,#9592,#9593,#9594,#9595,
#9596,#9597,#9598,#9599,#9600,#9601,#9602,#9603,#9604,#9605,#9606,#9607,
#9608,#9609,#9610,#9611,#9612,#9613,#9614,#9615,#9616,#9617,#9618,#9619,
#9620,#9621,#9622,#9623,#9624,#9625,#9626,#9627,#9628,#9629,#9630,#9631,
#9632,#9633,#9634,#9635,#9636,#9637,#9638,#9639,#9640,#9641,#9642,#9643,
#9644,#9645,#9646,#9647,#9648,#9649,#9650,#9651,#9652,#9653,#9654,#9655,
#9656,#9657,#9658,#9659,#9660,#9661,#9662,#9663,#9664,#9665,#9666,#9667,
#9668,#9669,#9670,#9671,#9672,#9673,#9674,#9675,#9676,#9677,#9678,#9679,
#9680,#9681,#9682,#9683,#9684,#9685,#9686,#9687,#9688,#9689,#9690,#9691,
#9692,#9693,#9694,#9695,#9696,#9697,#9698,#9699,#9700,#9701,#9702,#9703,
#9704,#9705,#9706,#9707,#9708,#9709,#9710,#9711,#9712,#9713,#9714,#9715,
#9716,#9717,#9718,#9719,#9720,#9721,#9722,#9723,#9724,#9725,#9726,#9727,
#9728,#9729,#9730,#9731,#9732),(#9733,#9734,#9735,#9736,#9737,#9738,#9739,
#9740,#9741,#9742,#9743,#9744,#9745,#9746,#9747,#9748,#9749,#9750,#9751,
#9752,#9753,#9754,#9755,#9756,#9757,#9758,#9759,#9760,#9761,#9762,#9763,
#9764,#9765,#9766,#9767,#9768,#9769,#9770,#9771,#9772,#9773,#9774,#9775,
#9776,#9777,#9778,#9779,#9780,#9781,#9782,#9783,#9784,#9785,#9786,#9787,
#9788,#9789,#9790,#9791,#9792,#9793,#9794,#9795,#9796,#9797,#9798,#9799,
#9800,#9801,#9802,#9803,#9804,#9805,#9806,#9807,#9808,#9809,#9810,#9811,
#9812,#9813,#9814,#9815,#9816,#9817,#9818,#9819,#9820,#9821,#9822,#9823,
#9824,#9825,#9826,#9827,#9828,#9829,#9830,#9831,#9832,#9833,#9834,#9835,
#9836,#9837,#9838,#9839,#9840,#9841,#9842,#9843,#9844,#9845,#9846,#9847,
#9848,#9849,#9850,#9851,#9852,#9853,#9854,#9855,#9856,#9857,#9858,#9859,
#9860,#9861,#9862,#9863,#9864,#9865,#9866,#9867,#9868,#9869,#9870,#9871,
#9872,#9873,#9874,#9875,#9876,#9877)),.UNSPECIFIED.,.F.,.F.,.F.)
B_SPLINE_SURFACE_WITH_KNOTS((2,2),(3,2,2,2,2,2,2,2,2,2,2,2,2,2,2,2,2,2,
2,2,2,2,2,2,2,2,2,2,2,2,2,2,2,2,2,2,2,2,2,2,2,2,2,2,2,2,2,2,2,2,2,2,2,2,
2,2,2,2,2,2,2,2,2,2,2,2,2,2,2,2,2,2,3),(0.,1.),(0.,0.0138888888888889,0.0277777777777778,
0.0416666666666667,0.0555555555555556,0.0694444444444444,0.0833333333333333,
0.0972222222222222,0.111111111111111,0.125,0.138888888888889,0.152777777777778,
0.166666666666667,0.180555555555556,0.194444444444444,0.208333333333333,
0.222222222222222,0.236111111111111,0.25,0.263888888888889,0.277777777777778,
0.291666666666667,0.305555555555556,0.319444444444444,0.333333333333333,
0.347222222222222,0.361111111111111,0.375,0.388888888888889,0.402777777777778,
0.416666666666667,0.430555555555556,0.444444444444444,0.458333333333333,
0.472222222222222,0.486111111111111,0.5,0.513888888888889,0.527777777777778,
0.541666666666667,0.555555555555556,0.569444444444444,0.583333333333333,
0.597222222222222,0.611111111111111,0.625,0.638888888888889,0.652777777777778,
0.666666666666667,0.680555555555556,0.694444444444444,0.708333333333333,
0.722222222222222,0.736111111111111,0.75,0.763888888888889,0.777777777777778,
0.791666666666667,0.805555555555556,0.819444444444444,0.833333333333333,
0.847222222222222,0.861111111111111,0.875,0.888888888888889,0.902777777777778,
0.916666666666667,0.930555555555556,0.944444444444444,0.958333333333333,
0.972222222222222,0.986111111111111,1.),.UNSPECIFIED.)
GEOMETRIC_REPRESENTATION_ITEM()
RATIONAL_B_SPLINE_SURFACE(((1.,0.965925826289068,1.,0.965925826289068,1.,
0.965925826289068,1.,0.965925826289068,1.,0.965925826289068,1.,0.965925826289068,
1.,0.965925826289068,1.,0.965925826289068,1.,0.965925826289068,1.,0.965925826289068,
1.,0.965925826289068,1.,0.965925826289068,1.,0.965925826289068,1.,0.965925826289068,
1.,0.965925826289068,1.,0.965925826289068,1.,0.965925826289068,1.,0.965925826289068,
1.,0.965925826289068,1.,0.965925826289068,1.,0.965925826289068,1.,0.965925826289068,
1.,0.965925826289068,1.,0.965925826289068,1.,0.965925826289068,1.,0.965925826289068,
1.,0.965925826289068,1.,0.965925826289068,1.,0.965925826289068,1.,0.965925826289068,
1.,0.965925826289068,1.,0.965925826289068,1.,0.965925826289068,1.,0.965925826289068,
1.,0.965925826289068,1.,0.965925826289068,1.,0.965925826289068,1.,0.965925826289068,
1.,0.965925826289068,1.,0.965925826289068,1.,0.965925826289068,1.,0.965925826289068,
1.,0.965925826289068,1.,0.965925826289068,1.,0.965925826289068,1.,0.965925826289068,
1.,0.965925826289068,1.,0.965925826289068,1.,0.965925826289068,1.,0.965925826289068,
1.,0.965925826289068,1.,0.965925826289068,1.,0.965925826289068,1.,0.965925826289068,
1.,0.965925826289068,1.,0.965925826289068,1.,0.965925826289068,1.,0.965925826289068,
1.,0.965925826289068,1.,0.965925826289068,1.,0.965925826289068,1.,0.965925826289068,
1.,0.965925826289068,1.,0.965925826289068,1.,0.965925826289068,1.,0.965925826289068,
1.,0.965925826289068,1.,0.965925826289068,1.,0.965925826289068,1.,0.965925826289068,
1.,0.965925826289068,1.,0.965925826289068,1.),(1.,0.965925826289068,1.,
0.965925826289068,1.,0.965925826289068,1.,0.965925826289068,1.,0.965925826289068,
1.,0.965925826289068,1.,0.965925826289068,1.,0.965925826289068,1.,0.965925826289068,
1.,0.965925826289068,1.,0.965925826289068,1.,0.965925826289068,1.,0.965925826289068,
1.,0.965925826289068,1.,0.965925826289068,1.,0.965925826289068,1.,0.965925826289068,
1.,0.965925826289068,1.,0.965925826289068,1.,0.965925826289068,1.,0.965925826289068,
1.,0.965925826289068,1.,0.965925826289068,1.,0.965925826289068,1.,0.965925826289068,
1.,0.965925826289068,1.,0.965925826289068,1.,0.965925826289068,1.,0.965925826289068,
1.,0.965925826289068,1.,0.965925826289068,1.,0.965925826289068,1.,0.965925826289068,
1.,0.965925826289068,1.,0.965925826289068,1.,0.965925826289068,1.,0.965925826289068,
1.,0.965925826289068,1.,0.965925826289068,1.,0.965925826289068,1.,0.965925826289068,
1.,0.965925826289068,1.,0.965925826289068,1.,0.965925826289068,1.,0.965925826289068,
1.,0.965925826289068,1.,0.965925826289068,1.,0.965925826289068,1.,0.965925826289068,
1.,0.965925826289068,1.,0.965925826289068,1.,0.965925826289068,1.,0.965925826289068,
1.,0.965925826289068,1.,0.965925826289068,1.,0.965925826289068,1.,0.965925826289068,
1.,0.965925826289068,1.,0.965925826289068,1.,0.965925826289068,1.,0.965925826289068,
1.,0.965925826289068,1.,0.965925826289068,1.,0.965925826289068,1.,0.965925826289068,
1.,0.965925826289068,1.,0.965925826289068,1.,0.965925826289068,1.,0.965925826289068,
1.,0.965925826289068,1.,0.965925826289068,1.,0.965925826289068,1.)))
REPRESENTATION_ITEM('')
SURFACE()
);
#166=(
BOUNDED_SURFACE()
B_SPLINE_SURFACE(1,2,((#9895,#9896,#9897,#9898,#9899,#9900,#9901,#9902,
#9903,#9904,#9905,#9906,#9907,#9908,#9909,#9910,#9911,#9912,#9913,#9914,
#9915,#9916,#9917,#9918,#9919,#9920,#9921,#9922,#9923,#9924,#9925,#9926,
#9927,#9928,#9929,#9930,#9931,#9932,#9933,#9934,#9935,#9936,#9937,#9938,
#9939,#9940,#9941,#9942,#9943,#9944,#9945,#9946,#9947,#9948,#9949,#9950,
#9951,#9952,#9953,#9954,#9955,#9956,#9957,#9958,#9959,#9960,#9961,#9962,
#9963,#9964,#9965,#9966,#9967,#9968,#9969,#9970,#9971,#9972,#9973,#9974,
#9975,#9976,#9977,#9978,#9979,#9980,#9981,#9982,#9983,#9984,#9985,#9986,
#9987,#9988,#9989,#9990,#9991,#9992,#9993,#9994,#9995,#9996,#9997,#9998,
#9999,#10000,#10001,#10002,#10003,#10004,#10005,#10006,#10007,#10008,#10009,
#10010,#10011,#10012,#10013,#10014,#10015,#10016,#10017,#10018,#10019,#10020,
#10021,#10022,#10023,#10024,#10025,#10026,#10027,#10028,#10029,#10030,#10031,
#10032,#10033,#10034,#10035,#10036,#10037,#10038,#10039),(#10040,#10041,
#10042,#10043,#10044,#10045,#10046,#10047,#10048,#10049,#10050,#10051,#10052,
#10053,#10054,#10055,#10056,#10057,#10058,#10059,#10060,#10061,#10062,#10063,
#10064,#10065,#10066,#10067,#10068,#10069,#10070,#10071,#10072,#10073,#10074,
#10075,#10076,#10077,#10078,#10079,#10080,#10081,#10082,#10083,#10084,#10085,
#10086,#10087,#10088,#10089,#10090,#10091,#10092,#10093,#10094,#10095,#10096,
#10097,#10098,#10099,#10100,#10101,#10102,#10103,#10104,#10105,#10106,#10107,
#10108,#10109,#10110,#10111,#10112,#10113,#10114,#10115,#10116,#10117,#10118,
#10119,#10120,#10121,#10122,#10123,#10124,#10125,#10126,#10127,#10128,#10129,
#10130,#10131,#10132,#10133,#10134,#10135,#10136,#10137,#10138,#10139,#10140,
#10141,#10142,#10143,#10144,#10145,#10146,#10147,#10148,#10149,#10150,#10151,
#10152,#10153,#10154,#10155,#10156,#10157,#10158,#10159,#10160,#10161,#10162,
#10163,#10164,#10165,#10166,#10167,#10168,#10169,#10170,#10171,#10172,#10173,
#10174,#10175,#10176,#10177,#10178,#10179,#10180,#10181,#10182,#10183,#10184)),
 .UNSPECIFIED.,.F.,.F.,.F.)
B_SPLINE_SURFACE_WITH_KNOTS((2,2),(3,2,2,2,2,2,2,2,2,2,2,2,2,2,2,2,2,2,
2,2,2,2,2,2,2,2,2,2,2,2,2,2,2,2,2,2,2,2,2,2,2,2,2,2,2,2,2,2,2,2,2,2,2,2,
2,2,2,2,2,2,2,2,2,2,2,2,2,2,2,2,2,2,3),(0.,1.),(0.,0.0138888888888889,0.0277777777777778,
0.0416666666666667,0.0555555555555556,0.0694444444444444,0.0833333333333333,
0.0972222222222222,0.111111111111111,0.125,0.138888888888889,0.152777777777778,
0.166666666666667,0.180555555555556,0.194444444444444,0.208333333333333,
0.222222222222222,0.236111111111111,0.25,0.263888888888889,0.277777777777778,
0.291666666666667,0.305555555555556,0.319444444444444,0.333333333333333,
0.347222222222222,0.361111111111111,0.375,0.388888888888889,0.402777777777778,
0.416666666666667,0.430555555555556,0.444444444444444,0.458333333333333,
0.472222222222222,0.486111111111111,0.5,0.513888888888889,0.527777777777778,
0.541666666666667,0.555555555555556,0.569444444444444,0.583333333333333,
0.597222222222222,0.611111111111111,0.625,0.638888888888889,0.652777777777778,
0.666666666666667,0.680555555555556,0.694444444444444,0.708333333333333,
0.722222222222222,0.736111111111111,0.75,0.763888888888889,0.777777777777778,
0.791666666666667,0.805555555555556,0.819444444444444,0.833333333333333,
0.847222222222222,0.861111111111111,0.875,0.888888888888889,0.902777777777778,
0.916666666666667,0.930555555555556,0.944444444444444,0.958333333333333,
0.972222222222222,0.986111111111111,1.),.UNSPECIFIED.)
GEOMETRIC_REPRESENTATION_ITEM()
RATIONAL_B_SPLINE_SURFACE(((1.,0.965925826289068,1.,0.965925826289068,1.,
0.965925826289068,1.,0.965925826289068,1.,0.965925826289068,1.,0.965925826289068,
1.,0.965925826289068,1.,0.965925826289068,1.,0.965925826289068,1.,0.965925826289068,
1.,0.965925826289068,1.,0.965925826289068,1.,0.965925826289068,1.,0.965925826289068,
1.,0.965925826289068,1.,0.965925826289068,1.,0.965925826289068,1.,0.965925826289068,
1.,0.965925826289068,1.,0.965925826289068,1.,0.965925826289068,1.,0.965925826289068,
1.,0.965925826289068,1.,0.965925826289068,1.,0.965925826289068,1.,0.965925826289068,
1.,0.965925826289068,1.,0.965925826289068,1.,0.965925826289068,1.,0.965925826289068,
1.,0.965925826289068,1.,0.965925826289068,1.,0.965925826289068,1.,0.965925826289068,
1.,0.965925826289068,1.,0.965925826289068,1.,0.965925826289068,1.,0.965925826289068,
1.,0.965925826289068,1.,0.965925826289068,1.,0.965925826289068,1.,0.965925826289068,
1.,0.965925826289068,1.,0.965925826289068,1.,0.965925826289068,1.,0.965925826289068,
1.,0.965925826289068,1.,0.965925826289068,1.,0.965925826289068,1.,0.965925826289068,
1.,0.965925826289068,1.,0.965925826289068,1.,0.965925826289068,1.,0.965925826289068,
1.,0.965925826289068,1.,0.965925826289068,1.,0.965925826289068,1.,0.965925826289068,
1.,0.965925826289068,1.,0.965925826289068,1.,0.965925826289068,1.,0.965925826289068,
1.,0.965925826289068,1.,0.965925826289068,1.,0.965925826289068,1.,0.965925826289068,
1.,0.965925826289068,1.,0.965925826289068,1.,0.965925826289068,1.,0.965925826289068,
1.,0.965925826289068,1.,0.965925826289068,1.),(1.,0.965925826289068,1.,
0.965925826289068,1.,0.965925826289068,1.,0.965925826289068,1.,0.965925826289068,
1.,0.965925826289068,1.,0.965925826289068,1.,0.965925826289068,1.,0.965925826289068,
1.,0.965925826289068,1.,0.965925826289068,1.,0.965925826289068,1.,0.965925826289068,
1.,0.965925826289068,1.,0.965925826289068,1.,0.965925826289068,1.,0.965925826289068,
1.,0.965925826289068,1.,0.965925826289068,1.,0.965925826289068,1.,0.965925826289068,
1.,0.965925826289068,1.,0.965925826289068,1.,0.965925826289068,1.,0.965925826289068,
1.,0.965925826289068,1.,0.965925826289068,1.,0.965925826289068,1.,0.965925826289068,
1.,0.965925826289068,1.,0.965925826289068,1.,0.965925826289068,1.,0.965925826289068,
1.,0.965925826289068,1.,0.965925826289068,1.,0.965925826289068,1.,0.965925826289068,
1.,0.965925826289068,1.,0.965925826289068,1.,0.965925826289068,1.,0.965925826289068,
1.,0.965925826289068,1.,0.965925826289068,1.,0.965925826289068,1.,0.965925826289068,
1.,0.965925826289068,1.,0.965925826289068,1.,0.965925826289068,1.,0.965925826289068,
1.,0.965925826289068,1.,0.965925826289068,1.,0.965925826289068,1.,0.965925826289068,
1.,0.965925826289068,1.,0.965925826289068,1.,0.965925826289068,1.,0.965925826289068,
1.,0.965925826289068,1.,0.965925826289068,1.,0.965925826289068,1.,0.965925826289068,
1.,0.965925826289068,1.,0.965925826289068,1.,0.965925826289068,1.,0.965925826289068,
1.,0.965925826289068,1.,0.965925826289068,1.,0.965925826289068,1.,0.965925826289068,
1.,0.965925826289068,1.,0.965925826289068,1.,0.965925826289068,1.)))
REPRESENTATION_ITEM('')
SURFACE()
);
#167=(
BOUNDED_SURFACE()
B_SPLINE_SURFACE(1,2,((#10210,#10211,#10212,#10213,#10214,#10215,#10216,
#10217,#10218,#10219,#10220,#10221,#10222,#10223,#10224,#10225,#10226,#10227,
#10228,#10229,#10230,#10231,#10232,#10233,#10234,#10235,#10236,#10237,#10238,
#10239,#10240,#10241,#10242,#10243,#10244,#10245,#10246,#10247,#10248,#10249,
#10250,#10251,#10252,#10253,#10254,#10255,#10256,#10257,#10258,#10259,#10260,
#10261,#10262,#10263,#10264,#10265,#10266,#10267,#10268,#10269,#10270,#10271,
#10272,#10273,#10274,#10275,#10276,#10277,#10278,#10279,#10280,#10281,#10282,
#10283,#10284,#10285,#10286,#10287,#10288,#10289,#10290,#10291,#10292,#10293,
#10294,#10295,#10296,#10297,#10298,#10299,#10300,#10301,#10302,#10303,#10304,
#10305,#10306,#10307,#10308,#10309,#10310,#10311,#10312,#10313,#10314,#10315,
#10316,#10317,#10318,#10319,#10320,#10321,#10322,#10323,#10324,#10325,#10326,
#10327,#10328,#10329,#10330,#10331,#10332,#10333,#10334,#10335,#10336,#10337,
#10338,#10339,#10340,#10341,#10342,#10343,#10344,#10345,#10346,#10347,#10348,
#10349,#10350,#10351,#10352,#10353,#10354),(#10355,#10356,#10357,#10358,
#10359,#10360,#10361,#10362,#10363,#10364,#10365,#10366,#10367,#10368,#10369,
#10370,#10371,#10372,#10373,#10374,#10375,#10376,#10377,#10378,#10379,#10380,
#10381,#10382,#10383,#10384,#10385,#10386,#10387,#10388,#10389,#10390,#10391,
#10392,#10393,#10394,#10395,#10396,#10397,#10398,#10399,#10400,#10401,#10402,
#10403,#10404,#10405,#10406,#10407,#10408,#10409,#10410,#10411,#10412,#10413,
#10414,#10415,#10416,#10417,#10418,#10419,#10420,#10421,#10422,#10423,#10424,
#10425,#10426,#10427,#10428,#10429,#10430,#10431,#10432,#10433,#10434,#10435,
#10436,#10437,#10438,#10439,#10440,#10441,#10442,#10443,#10444,#10445,#10446,
#10447,#10448,#10449,#10450,#10451,#10452,#10453,#10454,#10455,#10456,#10457,
#10458,#10459,#10460,#10461,#10462,#10463,#10464,#10465,#10466,#10467,#10468,
#10469,#10470,#10471,#10472,#10473,#10474,#10475,#10476,#10477,#10478,#10479,
#10480,#10481,#10482,#10483,#10484,#10485,#10486,#10487,#10488,#10489,#10490,
#10491,#10492,#10493,#10494,#10495,#10496,#10497,#10498,#10499)),
 .UNSPECIFIED.,.F.,.F.,.F.)
B_SPLINE_SURFACE_WITH_KNOTS((2,2),(3,2,2,2,2,2,2,2,2,2,2,2,2,2,2,2,2,2,
2,2,2,2,2,2,2,2,2,2,2,2,2,2,2,2,2,2,2,2,2,2,2,2,2,2,2,2,2,2,2,2,2,2,2,2,
2,2,2,2,2,2,2,2,2,2,2,2,2,2,2,2,2,2,3),(0.,1.),(0.,0.0138888888888889,0.0277777777777778,
0.0416666666666667,0.0555555555555556,0.0694444444444444,0.0833333333333333,
0.0972222222222222,0.111111111111111,0.125,0.138888888888889,0.152777777777778,
0.166666666666667,0.180555555555556,0.194444444444444,0.208333333333333,
0.222222222222222,0.236111111111111,0.25,0.263888888888889,0.277777777777778,
0.291666666666667,0.305555555555556,0.319444444444444,0.333333333333333,
0.347222222222222,0.361111111111111,0.375,0.388888888888889,0.402777777777778,
0.416666666666667,0.430555555555556,0.444444444444444,0.458333333333333,
0.472222222222222,0.486111111111111,0.5,0.513888888888889,0.527777777777778,
0.541666666666667,0.555555555555556,0.569444444444444,0.583333333333333,
0.597222222222222,0.611111111111111,0.625,0.638888888888889,0.652777777777778,
0.666666666666667,0.680555555555556,0.694444444444444,0.708333333333333,
0.722222222222222,0.736111111111111,0.75,0.763888888888889,0.777777777777778,
0.791666666666667,0.805555555555556,0.819444444444444,0.833333333333333,
0.847222222222222,0.861111111111111,0.875,0.888888888888889,0.902777777777778,
0.916666666666667,0.930555555555556,0.944444444444444,0.958333333333333,
0.972222222222222,0.986111111111111,1.),.UNSPECIFIED.)
GEOMETRIC_REPRESENTATION_ITEM()
RATIONAL_B_SPLINE_SURFACE(((1.,0.965925826289068,1.,0.965925826289068,1.,
0.965925826289068,1.,0.965925826289068,1.,0.965925826289068,1.,0.965925826289068,
1.,0.965925826289068,1.,0.965925826289068,1.,0.965925826289068,1.,0.965925826289068,
1.,0.965925826289068,1.,0.965925826289068,1.,0.965925826289068,1.,0.965925826289068,
1.,0.965925826289068,1.,0.965925826289068,1.,0.965925826289068,1.,0.965925826289068,
1.,0.965925826289068,1.,0.965925826289068,1.,0.965925826289068,1.,0.965925826289068,
1.,0.965925826289068,1.,0.965925826289068,1.,0.965925826289068,1.,0.965925826289068,
1.,0.965925826289068,1.,0.965925826289068,1.,0.965925826289068,1.,0.965925826289068,
1.,0.965925826289068,1.,0.965925826289068,1.,0.965925826289068,1.,0.965925826289068,
1.,0.965925826289068,1.,0.965925826289068,1.,0.965925826289068,1.,0.965925826289068,
1.,0.965925826289068,1.,0.965925826289068,1.,0.965925826289068,1.,0.965925826289068,
1.,0.965925826289068,1.,0.965925826289068,1.,0.965925826289068,1.,0.965925826289068,
1.,0.965925826289068,1.,0.965925826289068,1.,0.965925826289068,1.,0.965925826289068,
1.,0.965925826289068,1.,0.965925826289068,1.,0.965925826289068,1.,0.965925826289068,
1.,0.965925826289068,1.,0.965925826289068,1.,0.965925826289068,1.,0.965925826289068,
1.,0.965925826289068,1.,0.965925826289068,1.,0.965925826289068,1.,0.965925826289068,
1.,0.965925826289068,1.,0.965925826289068,1.,0.965925826289068,1.,0.965925826289068,
1.,0.965925826289068,1.,0.965925826289068,1.,0.965925826289068,1.,0.965925826289068,
1.,0.965925826289068,1.,0.965925826289068,1.),(1.,0.965925826289068,1.,
0.965925826289068,1.,0.965925826289068,1.,0.965925826289068,1.,0.965925826289068,
1.,0.965925826289068,1.,0.965925826289068,1.,0.965925826289068,1.,0.965925826289068,
1.,0.965925826289068,1.,0.965925826289068,1.,0.965925826289068,1.,0.965925826289068,
1.,0.965925826289068,1.,0.965925826289068,1.,0.965925826289068,1.,0.965925826289068,
1.,0.965925826289068,1.,0.965925826289068,1.,0.965925826289068,1.,0.965925826289068,
1.,0.965925826289068,1.,0.965925826289068,1.,0.965925826289068,1.,0.965925826289068,
1.,0.965925826289068,1.,0.965925826289068,1.,0.965925826289068,1.,0.965925826289068,
1.,0.965925826289068,1.,0.965925826289068,1.,0.965925826289068,1.,0.965925826289068,
1.,0.965925826289068,1.,0.965925826289068,1.,0.965925826289068,1.,0.965925826289068,
1.,0.965925826289068,1.,0.965925826289068,1.,0.965925826289068,1.,0.965925826289068,
1.,0.965925826289068,1.,0.965925826289068,1.,0.965925826289068,1.,0.965925826289068,
1.,0.965925826289068,1.,0.965925826289068,1.,0.965925826289068,1.,0.965925826289068,
1.,0.965925826289068,1.,0.965925826289068,1.,0.965925826289068,1.,0.965925826289068,
1.,0.965925826289068,1.,0.965925826289068,1.,0.965925826289068,1.,0.965925826289068,
1.,0.965925826289068,1.,0.965925826289068,1.,0.965925826289068,1.,0.965925826289068,
1.,0.965925826289068,1.,0.965925826289068,1.,0.965925826289068,1.,0.965925826289068,
1.,0.965925826289068,1.,0.965925826289068,1.,0.965925826289068,1.,0.965925826289068,
1.,0.965925826289068,1.,0.965925826289068,1.,0.965925826289068,1.)))
REPRESENTATION_ITEM('')
SURFACE()
);
#168=(
BOUNDED_SURFACE()
B_SPLINE_SURFACE(1,2,((#10531,#10532,#10533,#10534,#10535,#10536,#10537,
#10538,#10539,#10540,#10541,#10542,#10543,#10544,#10545,#10546,#10547,#10548,
#10549,#10550,#10551,#10552,#10553,#10554,#10555,#10556,#10557,#10558,#10559,
#10560,#10561,#10562,#10563,#10564,#10565,#10566,#10567,#10568,#10569,#10570,
#10571,#10572,#10573,#10574,#10575,#10576,#10577,#10578,#10579,#10580,#10581,
#10582,#10583,#10584,#10585,#10586,#10587,#10588,#10589,#10590,#10591,#10592,
#10593,#10594,#10595,#10596,#10597,#10598,#10599,#10600,#10601,#10602,#10603,
#10604,#10605,#10606,#10607,#10608,#10609,#10610,#10611,#10612,#10613,#10614,
#10615,#10616,#10617,#10618,#10619,#10620,#10621,#10622,#10623,#10624,#10625,
#10626,#10627,#10628,#10629,#10630,#10631,#10632,#10633,#10634,#10635,#10636,
#10637,#10638,#10639,#10640,#10641,#10642,#10643,#10644,#10645,#10646,#10647,
#10648,#10649,#10650,#10651,#10652,#10653,#10654,#10655,#10656,#10657,#10658,
#10659,#10660,#10661,#10662,#10663,#10664,#10665,#10666,#10667,#10668,#10669,
#10670,#10671,#10672,#10673,#10674,#10675),(#10676,#10677,#10678,#10679,
#10680,#10681,#10682,#10683,#10684,#10685,#10686,#10687,#10688,#10689,#10690,
#10691,#10692,#10693,#10694,#10695,#10696,#10697,#10698,#10699,#10700,#10701,
#10702,#10703,#10704,#10705,#10706,#10707,#10708,#10709,#10710,#10711,#10712,
#10713,#10714,#10715,#10716,#10717,#10718,#10719,#10720,#10721,#10722,#10723,
#10724,#10725,#10726,#10727,#10728,#10729,#10730,#10731,#10732,#10733,#10734,
#10735,#10736,#10737,#10738,#10739,#10740,#10741,#10742,#10743,#10744,#10745,
#10746,#10747,#10748,#10749,#10750,#10751,#10752,#10753,#10754,#10755,#10756,
#10757,#10758,#10759,#10760,#10761,#10762,#10763,#10764,#10765,#10766,#10767,
#10768,#10769,#10770,#10771,#10772,#10773,#10774,#10775,#10776,#10777,#10778,
#10779,#10780,#10781,#10782,#10783,#10784,#10785,#10786,#10787,#10788,#10789,
#10790,#10791,#10792,#10793,#10794,#10795,#10796,#10797,#10798,#10799,#10800,
#10801,#10802,#10803,#10804,#10805,#10806,#10807,#10808,#10809,#10810,#10811,
#10812,#10813,#10814,#10815,#10816,#10817,#10818,#10819,#10820)),
 .UNSPECIFIED.,.F.,.F.,.F.)
B_SPLINE_SURFACE_WITH_KNOTS((2,2),(3,2,2,2,2,2,2,2,2,2,2,2,2,2,2,2,2,2,
2,2,2,2,2,2,2,2,2,2,2,2,2,2,2,2,2,2,2,2,2,2,2,2,2,2,2,2,2,2,2,2,2,2,2,2,
2,2,2,2,2,2,2,2,2,2,2,2,2,2,2,2,2,2,3),(0.,1.),(0.,0.0138888888888889,0.0277777777777778,
0.0416666666666667,0.0555555555555556,0.0694444444444444,0.0833333333333333,
0.0972222222222222,0.111111111111111,0.125,0.138888888888889,0.152777777777778,
0.166666666666667,0.180555555555556,0.194444444444444,0.208333333333333,
0.222222222222222,0.236111111111111,0.25,0.263888888888889,0.277777777777778,
0.291666666666667,0.305555555555556,0.319444444444444,0.333333333333333,
0.347222222222222,0.361111111111111,0.375,0.388888888888889,0.402777777777778,
0.416666666666667,0.430555555555556,0.444444444444444,0.458333333333333,
0.472222222222222,0.486111111111111,0.5,0.513888888888889,0.527777777777778,
0.541666666666667,0.555555555555556,0.569444444444444,0.583333333333333,
0.597222222222222,0.611111111111111,0.625,0.638888888888889,0.652777777777778,
0.666666666666667,0.680555555555556,0.694444444444444,0.708333333333333,
0.722222222222222,0.736111111111111,0.75,0.763888888888889,0.777777777777778,
0.791666666666667,0.805555555555556,0.819444444444444,0.833333333333333,
0.847222222222222,0.861111111111111,0.875,0.888888888888889,0.902777777777778,
0.916666666666667,0.930555555555556,0.944444444444444,0.958333333333333,
0.972222222222222,0.986111111111111,1.),.UNSPECIFIED.)
GEOMETRIC_REPRESENTATION_ITEM()
RATIONAL_B_SPLINE_SURFACE(((1.,0.965925826289068,1.,0.965925826289068,1.,
0.965925826289068,1.,0.965925826289068,1.,0.965925826289068,1.,0.965925826289068,
1.,0.965925826289068,1.,0.965925826289068,1.,0.965925826289068,1.,0.965925826289068,
1.,0.965925826289068,1.,0.965925826289068,1.,0.965925826289068,1.,0.965925826289068,
1.,0.965925826289068,1.,0.965925826289068,1.,0.965925826289068,1.,0.965925826289068,
1.,0.965925826289068,1.,0.965925826289068,1.,0.965925826289068,1.,0.965925826289068,
1.,0.965925826289068,1.,0.965925826289068,1.,0.965925826289068,1.,0.965925826289068,
1.,0.965925826289068,1.,0.965925826289068,1.,0.965925826289068,1.,0.965925826289068,
1.,0.965925826289068,1.,0.965925826289068,1.,0.965925826289068,1.,0.965925826289068,
1.,0.965925826289068,1.,0.965925826289068,1.,0.965925826289068,1.,0.965925826289068,
1.,0.965925826289068,1.,0.965925826289068,1.,0.965925826289068,1.,0.965925826289068,
1.,0.965925826289068,1.,0.965925826289068,1.,0.965925826289068,1.,0.965925826289068,
1.,0.965925826289068,1.,0.965925826289068,1.,0.965925826289068,1.,0.965925826289068,
1.,0.965925826289068,1.,0.965925826289068,1.,0.965925826289068,1.,0.965925826289068,
1.,0.965925826289068,1.,0.965925826289068,1.,0.965925826289068,1.,0.965925826289068,
1.,0.965925826289068,1.,0.965925826289068,1.,0.965925826289068,1.,0.965925826289068,
1.,0.965925826289068,1.,0.965925826289068,1.,0.965925826289068,1.,0.965925826289068,
1.,0.965925826289068,1.,0.965925826289068,1.,0.965925826289068,1.,0.965925826289068,
1.,0.965925826289068,1.,0.965925826289068,1.),(1.,0.965925826289068,1.,
0.965925826289068,1.,0.965925826289068,1.,0.965925826289068,1.,0.965925826289068,
1.,0.965925826289068,1.,0.965925826289068,1.,0.965925826289068,1.,0.965925826289068,
1.,0.965925826289068,1.,0.965925826289068,1.,0.965925826289068,1.,0.965925826289068,
1.,0.965925826289068,1.,0.965925826289068,1.,0.965925826289068,1.,0.965925826289068,
1.,0.965925826289068,1.,0.965925826289068,1.,0.965925826289068,1.,0.965925826289068,
1.,0.965925826289068,1.,0.965925826289068,1.,0.965925826289068,1.,0.965925826289068,
1.,0.965925826289068,1.,0.965925826289068,1.,0.965925826289068,1.,0.965925826289068,
1.,0.965925826289068,1.,0.965925826289068,1.,0.965925826289068,1.,0.965925826289068,
1.,0.965925826289068,1.,0.965925826289068,1.,0.965925826289068,1.,0.965925826289068,
1.,0.965925826289068,1.,0.965925826289068,1.,0.965925826289068,1.,0.965925826289068,
1.,0.965925826289068,1.,0.965925826289068,1.,0.965925826289068,1.,0.965925826289068,
1.,0.965925826289068,1.,0.965925826289068,1.,0.965925826289068,1.,0.965925826289068,
1.,0.965925826289068,1.,0.965925826289068,1.,0.965925826289068,1.,0.965925826289068,
1.,0.965925826289068,1.,0.965925826289068,1.,0.965925826289068,1.,0.965925826289068,
1.,0.965925826289068,1.,0.965925826289068,1.,0.965925826289068,1.,0.965925826289068,
1.,0.965925826289068,1.,0.965925826289068,1.,0.965925826289068,1.,0.965925826289068,
1.,0.965925826289068,1.,0.965925826289068,1.,0.965925826289068,1.,0.965925826289068,
1.,0.965925826289068,1.,0.965925826289068,1.,0.965925826289068,1.)))
REPRESENTATION_ITEM('')
SURFACE()
);
#169=(
BOUNDED_SURFACE()
B_SPLINE_SURFACE(1,2,((#11117,#11118,#11119,#11120,#11121,#11122,#11123,
#11124,#11125,#11126,#11127,#11128,#11129,#11130,#11131,#11132,#11133,#11134,
#11135,#11136,#11137,#11138,#11139,#11140,#11141,#11142,#11143,#11144,#11145,
#11146,#11147,#11148,#11149,#11150,#11151,#11152,#11153,#11154,#11155,#11156,
#11157,#11158,#11159,#11160,#11161,#11162,#11163,#11164,#11165,#11166,#11167,
#11168,#11169,#11170,#11171,#11172,#11173,#11174,#11175,#11176,#11177,#11178,
#11179,#11180,#11181,#11182,#11183,#11184,#11185,#11186,#11187,#11188,#11189,
#11190,#11191,#11192,#11193,#11194,#11195,#11196,#11197,#11198,#11199,#11200,
#11201,#11202,#11203,#11204,#11205,#11206,#11207,#11208,#11209,#11210,#11211,
#11212,#11213,#11214,#11215,#11216,#11217,#11218,#11219,#11220,#11221,#11222,
#11223,#11224,#11225,#11226,#11227,#11228,#11229,#11230,#11231,#11232,#11233,
#11234,#11235,#11236,#11237,#11238,#11239,#11240,#11241,#11242,#11243,#11244,
#11245,#11246,#11247,#11248,#11249,#11250,#11251,#11252,#11253,#11254,#11255,
#11256,#11257,#11258,#11259,#11260,#11261),(#11262,#11263,#11264,#11265,
#11266,#11267,#11268,#11269,#11270,#11271,#11272,#11273,#11274,#11275,#11276,
#11277,#11278,#11279,#11280,#11281,#11282,#11283,#11284,#11285,#11286,#11287,
#11288,#11289,#11290,#11291,#11292,#11293,#11294,#11295,#11296,#11297,#11298,
#11299,#11300,#11301,#11302,#11303,#11304,#11305,#11306,#11307,#11308,#11309,
#11310,#11311,#11312,#11313,#11314,#11315,#11316,#11317,#11318,#11319,#11320,
#11321,#11322,#11323,#11324,#11325,#11326,#11327,#11328,#11329,#11330,#11331,
#11332,#11333,#11334,#11335,#11336,#11337,#11338,#11339,#11340,#11341,#11342,
#11343,#11344,#11345,#11346,#11347,#11348,#11349,#11350,#11351,#11352,#11353,
#11354,#11355,#11356,#11357,#11358,#11359,#11360,#11361,#11362,#11363,#11364,
#11365,#11366,#11367,#11368,#11369,#11370,#11371,#11372,#11373,#11374,#11375,
#11376,#11377,#11378,#11379,#11380,#11381,#11382,#11383,#11384,#11385,#11386,
#11387,#11388,#11389,#11390,#11391,#11392,#11393,#11394,#11395,#11396,#11397,
#11398,#11399,#11400,#11401,#11402,#11403,#11404,#11405,#11406)),
 .UNSPECIFIED.,.F.,.F.,.F.)
B_SPLINE_SURFACE_WITH_KNOTS((2,2),(3,2,2,2,2,2,2,2,2,2,2,2,2,2,2,2,2,2,
2,2,2,2,2,2,2,2,2,2,2,2,2,2,2,2,2,2,2,2,2,2,2,2,2,2,2,2,2,2,2,2,2,2,2,2,
2,2,2,2,2,2,2,2,2,2,2,2,2,2,2,2,2,2,3),(0.,1.),(0.,0.0138888888888889,0.0277777777777778,
0.0416666666666667,0.0555555555555556,0.0694444444444444,0.0833333333333333,
0.0972222222222222,0.111111111111111,0.125,0.138888888888889,0.152777777777778,
0.166666666666667,0.180555555555556,0.194444444444444,0.208333333333333,
0.222222222222222,0.236111111111111,0.25,0.263888888888889,0.277777777777778,
0.291666666666667,0.305555555555556,0.319444444444444,0.333333333333333,
0.347222222222222,0.361111111111111,0.375,0.388888888888889,0.402777777777778,
0.416666666666667,0.430555555555556,0.444444444444444,0.458333333333333,
0.472222222222222,0.486111111111111,0.5,0.513888888888889,0.527777777777778,
0.541666666666667,0.555555555555556,0.569444444444444,0.583333333333333,
0.597222222222222,0.611111111111111,0.625,0.638888888888889,0.652777777777778,
0.666666666666667,0.680555555555556,0.694444444444444,0.708333333333333,
0.722222222222222,0.736111111111111,0.75,0.763888888888889,0.777777777777778,
0.791666666666667,0.805555555555556,0.819444444444444,0.833333333333333,
0.847222222222222,0.861111111111111,0.875,0.888888888888889,0.902777777777778,
0.916666666666667,0.930555555555556,0.944444444444444,0.958333333333333,
0.972222222222222,0.986111111111111,1.),.UNSPECIFIED.)
GEOMETRIC_REPRESENTATION_ITEM()
RATIONAL_B_SPLINE_SURFACE(((1.,0.965925826289068,1.,0.965925826289068,1.,
0.965925826289068,1.,0.965925826289068,1.,0.965925826289068,1.,0.965925826289068,
1.,0.965925826289068,1.,0.965925826289068,1.,0.965925826289068,1.,0.965925826289068,
1.,0.965925826289068,1.,0.965925826289068,1.,0.965925826289068,1.,0.965925826289068,
1.,0.965925826289068,1.,0.965925826289068,1.,0.965925826289068,1.,0.965925826289068,
1.,0.965925826289068,1.,0.965925826289068,1.,0.965925826289068,1.,0.965925826289068,
1.,0.965925826289068,1.,0.965925826289068,1.,0.965925826289068,1.,0.965925826289068,
1.,0.965925826289068,1.,0.965925826289068,1.,0.965925826289068,1.,0.965925826289068,
1.,0.965925826289068,1.,0.965925826289068,1.,0.965925826289068,1.,0.965925826289068,
1.,0.965925826289068,1.,0.965925826289068,1.,0.965925826289068,1.,0.965925826289068,
1.,0.965925826289068,1.,0.965925826289068,1.,0.965925826289068,1.,0.965925826289068,
1.,0.965925826289068,1.,0.965925826289068,1.,0.965925826289068,1.,0.965925826289068,
1.,0.965925826289068,1.,0.965925826289068,1.,0.965925826289068,1.,0.965925826289068,
1.,0.965925826289068,1.,0.965925826289068,1.,0.965925826289068,1.,0.965925826289068,
1.,0.965925826289068,1.,0.965925826289068,1.,0.965925826289068,1.,0.965925826289068,
1.,0.965925826289068,1.,0.965925826289068,1.,0.965925826289068,1.,0.965925826289068,
1.,0.965925826289068,1.,0.965925826289068,1.,0.965925826289068,1.,0.965925826289068,
1.,0.965925826289068,1.,0.965925826289068,1.,0.965925826289068,1.,0.965925826289068,
1.,0.965925826289068,1.,0.965925826289068,1.),(1.,0.965925826289068,1.,
0.965925826289068,1.,0.965925826289068,1.,0.965925826289068,1.,0.965925826289068,
1.,0.965925826289068,1.,0.965925826289068,1.,0.965925826289068,1.,0.965925826289068,
1.,0.965925826289068,1.,0.965925826289068,1.,0.965925826289068,1.,0.965925826289068,
1.,0.965925826289068,1.,0.965925826289068,1.,0.965925826289068,1.,0.965925826289068,
1.,0.965925826289068,1.,0.965925826289068,1.,0.965925826289068,1.,0.965925826289068,
1.,0.965925826289068,1.,0.965925826289068,1.,0.965925826289068,1.,0.965925826289068,
1.,0.965925826289068,1.,0.965925826289068,1.,0.965925826289068,1.,0.965925826289068,
1.,0.965925826289068,1.,0.965925826289068,1.,0.965925826289068,1.,0.965925826289068,
1.,0.965925826289068,1.,0.965925826289068,1.,0.965925826289068,1.,0.965925826289068,
1.,0.965925826289068,1.,0.965925826289068,1.,0.965925826289068,1.,0.965925826289068,
1.,0.965925826289068,1.,0.965925826289068,1.,0.965925826289068,1.,0.965925826289068,
1.,0.965925826289068,1.,0.965925826289068,1.,0.965925826289068,1.,0.965925826289068,
1.,0.965925826289068,1.,0.965925826289068,1.,0.965925826289068,1.,0.965925826289068,
1.,0.965925826289068,1.,0.965925826289068,1.,0.965925826289068,1.,0.965925826289068,
1.,0.965925826289068,1.,0.965925826289068,1.,0.965925826289068,1.,0.965925826289068,
1.,0.965925826289068,1.,0.965925826289068,1.,0.965925826289068,1.,0.965925826289068,
1.,0.965925826289068,1.,0.965925826289068,1.,0.965925826289068,1.,0.965925826289068,
1.,0.965925826289068,1.,0.965925826289068,1.,0.965925826289068,1.)))
REPRESENTATION_ITEM('')
SURFACE()
);
#170=(
BOUNDED_SURFACE()
B_SPLINE_SURFACE(1,2,((#11430,#11431,#11432,#11433,#11434,#11435,#11436,
#11437,#11438,#11439,#11440,#11441,#11442,#11443,#11444,#11445,#11446,#11447,
#11448,#11449,#11450,#11451,#11452,#11453,#11454,#11455,#11456,#11457,#11458,
#11459,#11460,#11461,#11462,#11463,#11464,#11465,#11466,#11467,#11468,#11469,
#11470,#11471,#11472,#11473,#11474,#11475,#11476,#11477,#11478,#11479,#11480,
#11481,#11482,#11483,#11484,#11485,#11486,#11487,#11488,#11489,#11490,#11491,
#11492,#11493,#11494,#11495,#11496,#11497,#11498,#11499,#11500,#11501,#11502,
#11503,#11504,#11505,#11506,#11507,#11508,#11509,#11510,#11511,#11512,#11513,
#11514,#11515,#11516,#11517,#11518,#11519,#11520,#11521,#11522,#11523,#11524,
#11525,#11526,#11527,#11528,#11529,#11530,#11531,#11532,#11533,#11534,#11535,
#11536,#11537,#11538,#11539,#11540,#11541,#11542,#11543,#11544,#11545,#11546,
#11547,#11548,#11549,#11550,#11551,#11552,#11553,#11554,#11555,#11556,#11557,
#11558,#11559,#11560,#11561,#11562,#11563,#11564,#11565,#11566,#11567,#11568,
#11569,#11570,#11571,#11572,#11573,#11574),(#11575,#11576,#11577,#11578,
#11579,#11580,#11581,#11582,#11583,#11584,#11585,#11586,#11587,#11588,#11589,
#11590,#11591,#11592,#11593,#11594,#11595,#11596,#11597,#11598,#11599,#11600,
#11601,#11602,#11603,#11604,#11605,#11606,#11607,#11608,#11609,#11610,#11611,
#11612,#11613,#11614,#11615,#11616,#11617,#11618,#11619,#11620,#11621,#11622,
#11623,#11624,#11625,#11626,#11627,#11628,#11629,#11630,#11631,#11632,#11633,
#11634,#11635,#11636,#11637,#11638,#11639,#11640,#11641,#11642,#11643,#11644,
#11645,#11646,#11647,#11648,#11649,#11650,#11651,#11652,#11653,#11654,#11655,
#11656,#11657,#11658,#11659,#11660,#11661,#11662,#11663,#11664,#11665,#11666,
#11667,#11668,#11669,#11670,#11671,#11672,#11673,#11674,#11675,#11676,#11677,
#11678,#11679,#11680,#11681,#11682,#11683,#11684,#11685,#11686,#11687,#11688,
#11689,#11690,#11691,#11692,#11693,#11694,#11695,#11696,#11697,#11698,#11699,
#11700,#11701,#11702,#11703,#11704,#11705,#11706,#11707,#11708,#11709,#11710,
#11711,#11712,#11713,#11714,#11715,#11716,#11717,#11718,#11719)),
 .UNSPECIFIED.,.F.,.F.,.F.)
B_SPLINE_SURFACE_WITH_KNOTS((2,2),(3,2,2,2,2,2,2,2,2,2,2,2,2,2,2,2,2,2,
2,2,2,2,2,2,2,2,2,2,2,2,2,2,2,2,2,2,2,2,2,2,2,2,2,2,2,2,2,2,2,2,2,2,2,2,
2,2,2,2,2,2,2,2,2,2,2,2,2,2,2,2,2,2,3),(0.,1.),(0.,0.0138888888888889,0.0277777777777778,
0.0416666666666667,0.0555555555555556,0.0694444444444444,0.0833333333333333,
0.0972222222222222,0.111111111111111,0.125,0.138888888888889,0.152777777777778,
0.166666666666667,0.180555555555556,0.194444444444444,0.208333333333333,
0.222222222222222,0.236111111111111,0.25,0.263888888888889,0.277777777777778,
0.291666666666667,0.305555555555556,0.319444444444444,0.333333333333333,
0.347222222222222,0.361111111111111,0.375,0.388888888888889,0.402777777777778,
0.416666666666667,0.430555555555556,0.444444444444444,0.458333333333333,
0.472222222222222,0.486111111111111,0.5,0.513888888888889,0.527777777777778,
0.541666666666667,0.555555555555556,0.569444444444444,0.583333333333333,
0.597222222222222,0.611111111111111,0.625,0.638888888888889,0.652777777777778,
0.666666666666667,0.680555555555556,0.694444444444444,0.708333333333333,
0.722222222222222,0.736111111111111,0.75,0.763888888888889,0.777777777777778,
0.791666666666667,0.805555555555556,0.819444444444444,0.833333333333333,
0.847222222222222,0.861111111111111,0.875,0.888888888888889,0.902777777777778,
0.916666666666667,0.930555555555556,0.944444444444444,0.958333333333333,
0.972222222222222,0.986111111111111,1.),.UNSPECIFIED.)
GEOMETRIC_REPRESENTATION_ITEM()
RATIONAL_B_SPLINE_SURFACE(((1.,0.965925826289068,1.,0.965925826289068,1.,
0.965925826289068,1.,0.965925826289068,1.,0.965925826289068,1.,0.965925826289068,
1.,0.965925826289068,1.,0.965925826289068,1.,0.965925826289068,1.,0.965925826289068,
1.,0.965925826289068,1.,0.965925826289068,1.,0.965925826289068,1.,0.965925826289068,
1.,0.965925826289068,1.,0.965925826289068,1.,0.965925826289068,1.,0.965925826289068,
1.,0.965925826289068,1.,0.965925826289068,1.,0.965925826289068,1.,0.965925826289068,
1.,0.965925826289068,1.,0.965925826289068,1.,0.965925826289068,1.,0.965925826289068,
1.,0.965925826289068,1.,0.965925826289068,1.,0.965925826289068,1.,0.965925826289068,
1.,0.965925826289068,1.,0.965925826289068,1.,0.965925826289068,1.,0.965925826289068,
1.,0.965925826289068,1.,0.965925826289068,1.,0.965925826289068,1.,0.965925826289068,
1.,0.965925826289068,1.,0.965925826289068,1.,0.965925826289068,1.,0.965925826289068,
1.,0.965925826289068,1.,0.965925826289068,1.,0.965925826289068,1.,0.965925826289068,
1.,0.965925826289068,1.,0.965925826289068,1.,0.965925826289068,1.,0.965925826289068,
1.,0.965925826289068,1.,0.965925826289068,1.,0.965925826289068,1.,0.965925826289068,
1.,0.965925826289068,1.,0.965925826289068,1.,0.965925826289068,1.,0.965925826289068,
1.,0.965925826289068,1.,0.965925826289068,1.,0.965925826289068,1.,0.965925826289068,
1.,0.965925826289068,1.,0.965925826289068,1.,0.965925826289068,1.,0.965925826289068,
1.,0.965925826289068,1.,0.965925826289068,1.,0.965925826289068,1.,0.965925826289068,
1.,0.965925826289068,1.,0.965925826289068,1.),(1.,0.965925826289068,1.,
0.965925826289068,1.,0.965925826289068,1.,0.965925826289068,1.,0.965925826289068,
1.,0.965925826289068,1.,0.965925826289068,1.,0.965925826289068,1.,0.965925826289068,
1.,0.965925826289068,1.,0.965925826289068,1.,0.965925826289068,1.,0.965925826289068,
1.,0.965925826289068,1.,0.965925826289068,1.,0.965925826289068,1.,0.965925826289068,
1.,0.965925826289068,1.,0.965925826289068,1.,0.965925826289068,1.,0.965925826289068,
1.,0.965925826289068,1.,0.965925826289068,1.,0.965925826289068,1.,0.965925826289068,
1.,0.965925826289068,1.,0.965925826289068,1.,0.965925826289068,1.,0.965925826289068,
1.,0.965925826289068,1.,0.965925826289068,1.,0.965925826289068,1.,0.965925826289068,
1.,0.965925826289068,1.,0.965925826289068,1.,0.965925826289068,1.,0.965925826289068,
1.,0.965925826289068,1.,0.965925826289068,1.,0.965925826289068,1.,0.965925826289068,
1.,0.965925826289068,1.,0.965925826289068,1.,0.965925826289068,1.,0.965925826289068,
1.,0.965925826289068,1.,0.965925826289068,1.,0.965925826289068,1.,0.965925826289068,
1.,0.965925826289068,1.,0.965925826289068,1.,0.965925826289068,1.,0.965925826289068,
1.,0.965925826289068,1.,0.965925826289068,1.,0.965925826289068,1.,0.965925826289068,
1.,0.965925826289068,1.,0.965925826289068,1.,0.965925826289068,1.,0.965925826289068,
1.,0.965925826289068,1.,0.965925826289068,1.,0.965925826289068,1.,0.965925826289068,
1.,0.965925826289068,1.,0.965925826289068,1.,0.965925826289068,1.,0.965925826289068,
1.,0.965925826289068,1.,0.965925826289068,1.,0.965925826289068,1.)))
REPRESENTATION_ITEM('')
SURFACE()
);
#171=(
BOUNDED_SURFACE()
B_SPLINE_SURFACE(1,2,((#11750,#11751,#11752,#11753,#11754,#11755,#11756,
#11757,#11758,#11759,#11760,#11761,#11762,#11763,#11764,#11765,#11766,#11767,
#11768,#11769,#11770,#11771,#11772,#11773,#11774,#11775,#11776,#11777,#11778,
#11779,#11780,#11781,#11782,#11783,#11784,#11785,#11786,#11787,#11788,#11789,
#11790,#11791,#11792,#11793,#11794,#11795,#11796,#11797,#11798,#11799,#11800,
#11801,#11802,#11803,#11804,#11805,#11806,#11807,#11808,#11809,#11810,#11811,
#11812,#11813,#11814,#11815,#11816,#11817,#11818,#11819,#11820,#11821,#11822,
#11823,#11824,#11825,#11826,#11827,#11828,#11829,#11830,#11831,#11832,#11833,
#11834,#11835,#11836,#11837,#11838,#11839,#11840,#11841,#11842,#11843,#11844,
#11845,#11846,#11847,#11848,#11849,#11850,#11851,#11852,#11853,#11854,#11855,
#11856,#11857,#11858,#11859,#11860,#11861,#11862,#11863,#11864,#11865,#11866,
#11867,#11868,#11869,#11870,#11871,#11872,#11873,#11874,#11875,#11876,#11877,
#11878,#11879,#11880,#11881,#11882,#11883,#11884,#11885,#11886,#11887,#11888,
#11889,#11890,#11891,#11892,#11893,#11894),(#11895,#11896,#11897,#11898,
#11899,#11900,#11901,#11902,#11903,#11904,#11905,#11906,#11907,#11908,#11909,
#11910,#11911,#11912,#11913,#11914,#11915,#11916,#11917,#11918,#11919,#11920,
#11921,#11922,#11923,#11924,#11925,#11926,#11927,#11928,#11929,#11930,#11931,
#11932,#11933,#11934,#11935,#11936,#11937,#11938,#11939,#11940,#11941,#11942,
#11943,#11944,#11945,#11946,#11947,#11948,#11949,#11950,#11951,#11952,#11953,
#11954,#11955,#11956,#11957,#11958,#11959,#11960,#11961,#11962,#11963,#11964,
#11965,#11966,#11967,#11968,#11969,#11970,#11971,#11972,#11973,#11974,#11975,
#11976,#11977,#11978,#11979,#11980,#11981,#11982,#11983,#11984,#11985,#11986,
#11987,#11988,#11989,#11990,#11991,#11992,#11993,#11994,#11995,#11996,#11997,
#11998,#11999,#12000,#12001,#12002,#12003,#12004,#12005,#12006,#12007,#12008,
#12009,#12010,#12011,#12012,#12013,#12014,#12015,#12016,#12017,#12018,#12019,
#12020,#12021,#12022,#12023,#12024,#12025,#12026,#12027,#12028,#12029,#12030,
#12031,#12032,#12033,#12034,#12035,#12036,#12037,#12038,#12039)),
 .UNSPECIFIED.,.F.,.F.,.F.)
B_SPLINE_SURFACE_WITH_KNOTS((2,2),(3,2,2,2,2,2,2,2,2,2,2,2,2,2,2,2,2,2,
2,2,2,2,2,2,2,2,2,2,2,2,2,2,2,2,2,2,2,2,2,2,2,2,2,2,2,2,2,2,2,2,2,2,2,2,
2,2,2,2,2,2,2,2,2,2,2,2,2,2,2,2,2,2,3),(0.,1.),(0.,0.0138888888888889,0.0277777777777778,
0.0416666666666667,0.0555555555555556,0.0694444444444444,0.0833333333333333,
0.0972222222222222,0.111111111111111,0.125,0.138888888888889,0.152777777777778,
0.166666666666667,0.180555555555556,0.194444444444444,0.208333333333333,
0.222222222222222,0.236111111111111,0.25,0.263888888888889,0.277777777777778,
0.291666666666667,0.305555555555556,0.319444444444444,0.333333333333333,
0.347222222222222,0.361111111111111,0.375,0.388888888888889,0.402777777777778,
0.416666666666667,0.430555555555556,0.444444444444444,0.458333333333333,
0.472222222222222,0.486111111111111,0.5,0.513888888888889,0.527777777777778,
0.541666666666667,0.555555555555556,0.569444444444444,0.583333333333333,
0.597222222222222,0.611111111111111,0.625,0.638888888888889,0.652777777777778,
0.666666666666667,0.680555555555556,0.694444444444444,0.708333333333333,
0.722222222222222,0.736111111111111,0.75,0.763888888888889,0.777777777777778,
0.791666666666667,0.805555555555556,0.819444444444444,0.833333333333333,
0.847222222222222,0.861111111111111,0.875,0.888888888888889,0.902777777777778,
0.916666666666667,0.930555555555556,0.944444444444444,0.958333333333333,
0.972222222222222,0.986111111111111,1.),.UNSPECIFIED.)
GEOMETRIC_REPRESENTATION_ITEM()
RATIONAL_B_SPLINE_SURFACE(((1.,0.965925826289068,1.,0.965925826289068,1.,
0.965925826289068,1.,0.965925826289068,1.,0.965925826289068,1.,0.965925826289068,
1.,0.965925826289068,1.,0.965925826289068,1.,0.965925826289068,1.,0.965925826289068,
1.,0.965925826289068,1.,0.965925826289068,1.,0.965925826289068,1.,0.965925826289068,
1.,0.965925826289068,1.,0.965925826289068,1.,0.965925826289068,1.,0.965925826289068,
1.,0.965925826289068,1.,0.965925826289068,1.,0.965925826289068,1.,0.965925826289068,
1.,0.965925826289068,1.,0.965925826289068,1.,0.965925826289068,1.,0.965925826289068,
1.,0.965925826289068,1.,0.965925826289068,1.,0.965925826289068,1.,0.965925826289068,
1.,0.965925826289068,1.,0.965925826289068,1.,0.965925826289068,1.,0.965925826289068,
1.,0.965925826289068,1.,0.965925826289068,1.,0.965925826289068,1.,0.965925826289068,
1.,0.965925826289068,1.,0.965925826289068,1.,0.965925826289068,1.,0.965925826289068,
1.,0.965925826289068,1.,0.965925826289068,1.,0.965925826289068,1.,0.965925826289068,
1.,0.965925826289068,1.,0.965925826289068,1.,0.965925826289068,1.,0.965925826289068,
1.,0.965925826289068,1.,0.965925826289068,1.,0.965925826289068,1.,0.965925826289068,
1.,0.965925826289068,1.,0.965925826289068,1.,0.965925826289068,1.,0.965925826289068,
1.,0.965925826289068,1.,0.965925826289068,1.,0.965925826289068,1.,0.965925826289068,
1.,0.965925826289068,1.,0.965925826289068,1.,0.965925826289068,1.,0.965925826289068,
1.,0.965925826289068,1.,0.965925826289068,1.,0.965925826289068,1.,0.965925826289068,
1.,0.965925826289068,1.,0.965925826289068,1.),(1.,0.965925826289068,1.,
0.965925826289068,1.,0.965925826289068,1.,0.965925826289068,1.,0.965925826289068,
1.,0.965925826289068,1.,0.965925826289068,1.,0.965925826289068,1.,0.965925826289068,
1.,0.965925826289068,1.,0.965925826289068,1.,0.965925826289068,1.,0.965925826289068,
1.,0.965925826289068,1.,0.965925826289068,1.,0.965925826289068,1.,0.965925826289068,
1.,0.965925826289068,1.,0.965925826289068,1.,0.965925826289068,1.,0.965925826289068,
1.,0.965925826289068,1.,0.965925826289068,1.,0.965925826289068,1.,0.965925826289068,
1.,0.965925826289068,1.,0.965925826289068,1.,0.965925826289068,1.,0.965925826289068,
1.,0.965925826289068,1.,0.965925826289068,1.,0.965925826289068,1.,0.965925826289068,
1.,0.965925826289068,1.,0.965925826289068,1.,0.965925826289068,1.,0.965925826289068,
1.,0.965925826289068,1.,0.965925826289068,1.,0.965925826289068,1.,0.965925826289068,
1.,0.965925826289068,1.,0.965925826289068,1.,0.965925826289068,1.,0.965925826289068,
1.,0.965925826289068,1.,0.965925826289068,1.,0.965925826289068,1.,0.965925826289068,
1.,0.965925826289068,1.,0.965925826289068,1.,0.965925826289068,1.,0.965925826289068,
1.,0.965925826289068,1.,0.965925826289068,1.,0.965925826289068,1.,0.965925826289068,
1.,0.965925826289068,1.,0.965925826289068,1.,0.965925826289068,1.,0.965925826289068,
1.,0.965925826289068,1.,0.965925826289068,1.,0.965925826289068,1.,0.965925826289068,
1.,0.965925826289068,1.,0.965925826289068,1.,0.965925826289068,1.,0.965925826289068,
1.,0.965925826289068,1.,0.965925826289068,1.,0.965925826289068,1.)))
REPRESENTATION_ITEM('')
SURFACE()
);
#172=(
BOUNDED_SURFACE()
B_SPLINE_SURFACE(1,2,((#12056,#12057,#12058,#12059,#12060,#12061,#12062,
#12063,#12064,#12065,#12066,#12067,#12068,#12069,#12070,#12071,#12072,#12073,
#12074,#12075,#12076,#12077,#12078,#12079,#12080,#12081,#12082,#12083,#12084,
#12085,#12086,#12087,#12088,#12089,#12090,#12091,#12092,#12093,#12094,#12095,
#12096,#12097,#12098,#12099,#12100,#12101,#12102,#12103,#12104,#12105,#12106,
#12107,#12108,#12109,#12110,#12111,#12112,#12113,#12114,#12115,#12116,#12117,
#12118,#12119,#12120,#12121,#12122,#12123,#12124,#12125,#12126,#12127,#12128,
#12129,#12130,#12131,#12132,#12133,#12134,#12135,#12136,#12137,#12138,#12139,
#12140,#12141,#12142,#12143,#12144,#12145,#12146,#12147,#12148,#12149,#12150,
#12151,#12152,#12153,#12154,#12155,#12156,#12157,#12158,#12159,#12160,#12161,
#12162,#12163,#12164,#12165,#12166,#12167,#12168,#12169,#12170,#12171,#12172,
#12173,#12174,#12175,#12176,#12177,#12178,#12179,#12180,#12181,#12182,#12183,
#12184,#12185,#12186,#12187,#12188,#12189,#12190,#12191,#12192,#12193,#12194,
#12195,#12196,#12197,#12198,#12199,#12200),(#12201,#12202,#12203,#12204,
#12205,#12206,#12207,#12208,#12209,#12210,#12211,#12212,#12213,#12214,#12215,
#12216,#12217,#12218,#12219,#12220,#12221,#12222,#12223,#12224,#12225,#12226,
#12227,#12228,#12229,#12230,#12231,#12232,#12233,#12234,#12235,#12236,#12237,
#12238,#12239,#12240,#12241,#12242,#12243,#12244,#12245,#12246,#12247,#12248,
#12249,#12250,#12251,#12252,#12253,#12254,#12255,#12256,#12257,#12258,#12259,
#12260,#12261,#12262,#12263,#12264,#12265,#12266,#12267,#12268,#12269,#12270,
#12271,#12272,#12273,#12274,#12275,#12276,#12277,#12278,#12279,#12280,#12281,
#12282,#12283,#12284,#12285,#12286,#12287,#12288,#12289,#12290,#12291,#12292,
#12293,#12294,#12295,#12296,#12297,#12298,#12299,#12300,#12301,#12302,#12303,
#12304,#12305,#12306,#12307,#12308,#12309,#12310,#12311,#12312,#12313,#12314,
#12315,#12316,#12317,#12318,#12319,#12320,#12321,#12322,#12323,#12324,#12325,
#12326,#12327,#12328,#12329,#12330,#12331,#12332,#12333,#12334,#12335,#12336,
#12337,#12338,#12339,#12340,#12341,#12342,#12343,#12344,#12345)),
 .UNSPECIFIED.,.F.,.F.,.F.)
B_SPLINE_SURFACE_WITH_KNOTS((2,2),(3,2,2,2,2,2,2,2,2,2,2,2,2,2,2,2,2,2,
2,2,2,2,2,2,2,2,2,2,2,2,2,2,2,2,2,2,2,2,2,2,2,2,2,2,2,2,2,2,2,2,2,2,2,2,
2,2,2,2,2,2,2,2,2,2,2,2,2,2,2,2,2,2,3),(0.,1.),(0.,0.0138888888888889,0.0277777777777778,
0.0416666666666667,0.0555555555555556,0.0694444444444444,0.0833333333333333,
0.0972222222222222,0.111111111111111,0.125,0.138888888888889,0.152777777777778,
0.166666666666667,0.180555555555556,0.194444444444444,0.208333333333333,
0.222222222222222,0.236111111111111,0.25,0.263888888888889,0.277777777777778,
0.291666666666667,0.305555555555556,0.319444444444444,0.333333333333333,
0.347222222222222,0.361111111111111,0.375,0.388888888888889,0.402777777777778,
0.416666666666667,0.430555555555556,0.444444444444444,0.458333333333333,
0.472222222222222,0.486111111111111,0.5,0.513888888888889,0.527777777777778,
0.541666666666667,0.555555555555556,0.569444444444444,0.583333333333333,
0.597222222222222,0.611111111111111,0.625,0.638888888888889,0.652777777777778,
0.666666666666667,0.680555555555556,0.694444444444444,0.708333333333333,
0.722222222222222,0.736111111111111,0.75,0.763888888888889,0.777777777777778,
0.791666666666667,0.805555555555556,0.819444444444444,0.833333333333333,
0.847222222222222,0.861111111111111,0.875,0.888888888888889,0.902777777777778,
0.916666666666667,0.930555555555556,0.944444444444444,0.958333333333333,
0.972222222222222,0.986111111111111,1.),.UNSPECIFIED.)
GEOMETRIC_REPRESENTATION_ITEM()
RATIONAL_B_SPLINE_SURFACE(((1.,0.965925826289068,1.,0.965925826289068,1.,
0.965925826289068,1.,0.965925826289068,1.,0.965925826289068,1.,0.965925826289068,
1.,0.965925826289068,1.,0.965925826289068,1.,0.965925826289068,1.,0.965925826289068,
1.,0.965925826289068,1.,0.965925826289068,1.,0.965925826289068,1.,0.965925826289068,
1.,0.965925826289068,1.,0.965925826289068,1.,0.965925826289068,1.,0.965925826289068,
1.,0.965925826289068,1.,0.965925826289068,1.,0.965925826289068,1.,0.965925826289068,
1.,0.965925826289068,1.,0.965925826289068,1.,0.965925826289068,1.,0.965925826289068,
1.,0.965925826289068,1.,0.965925826289068,1.,0.965925826289068,1.,0.965925826289068,
1.,0.965925826289068,1.,0.965925826289068,1.,0.965925826289068,1.,0.965925826289068,
1.,0.965925826289068,1.,0.965925826289068,1.,0.965925826289068,1.,0.965925826289068,
1.,0.965925826289068,1.,0.965925826289068,1.,0.965925826289068,1.,0.965925826289068,
1.,0.965925826289068,1.,0.965925826289068,1.,0.965925826289068,1.,0.965925826289068,
1.,0.965925826289068,1.,0.965925826289068,1.,0.965925826289068,1.,0.965925826289068,
1.,0.965925826289068,1.,0.965925826289068,1.,0.965925826289068,1.,0.965925826289068,
1.,0.965925826289068,1.,0.965925826289068,1.,0.965925826289068,1.,0.965925826289068,
1.,0.965925826289068,1.,0.965925826289068,1.,0.965925826289068,1.,0.965925826289068,
1.,0.965925826289068,1.,0.965925826289068,1.,0.965925826289068,1.,0.965925826289068,
1.,0.965925826289068,1.,0.965925826289068,1.,0.965925826289068,1.,0.965925826289068,
1.,0.965925826289068,1.,0.965925826289068,1.),(1.,0.965925826289068,1.,
0.965925826289068,1.,0.965925826289068,1.,0.965925826289068,1.,0.965925826289068,
1.,0.965925826289068,1.,0.965925826289068,1.,0.965925826289068,1.,0.965925826289068,
1.,0.965925826289068,1.,0.965925826289068,1.,0.965925826289068,1.,0.965925826289068,
1.,0.965925826289068,1.,0.965925826289068,1.,0.965925826289068,1.,0.965925826289068,
1.,0.965925826289068,1.,0.965925826289068,1.,0.965925826289068,1.,0.965925826289068,
1.,0.965925826289068,1.,0.965925826289068,1.,0.965925826289068,1.,0.965925826289068,
1.,0.965925826289068,1.,0.965925826289068,1.,0.965925826289068,1.,0.965925826289068,
1.,0.965925826289068,1.,0.965925826289068,1.,0.965925826289068,1.,0.965925826289068,
1.,0.965925826289068,1.,0.965925826289068,1.,0.965925826289068,1.,0.965925826289068,
1.,0.965925826289068,1.,0.965925826289068,1.,0.965925826289068,1.,0.965925826289068,
1.,0.965925826289068,1.,0.965925826289068,1.,0.965925826289068,1.,0.965925826289068,
1.,0.965925826289068,1.,0.965925826289068,1.,0.965925826289068,1.,0.965925826289068,
1.,0.965925826289068,1.,0.965925826289068,1.,0.965925826289068,1.,0.965925826289068,
1.,0.965925826289068,1.,0.965925826289068,1.,0.965925826289068,1.,0.965925826289068,
1.,0.965925826289068,1.,0.965925826289068,1.,0.965925826289068,1.,0.965925826289068,
1.,0.965925826289068,1.,0.965925826289068,1.,0.965925826289068,1.,0.965925826289068,
1.,0.965925826289068,1.,0.965925826289068,1.,0.965925826289068,1.,0.965925826289068,
1.,0.965925826289068,1.,0.965925826289068,1.,0.965925826289068,1.)))
REPRESENTATION_ITEM('')
SURFACE()
);
#173=(
BOUNDED_SURFACE()
B_SPLINE_SURFACE(1,2,((#12362,#12363,#12364,#12365,#12366,#12367,#12368,
#12369,#12370,#12371,#12372,#12373,#12374,#12375,#12376,#12377,#12378,#12379,
#12380,#12381,#12382,#12383,#12384,#12385,#12386,#12387,#12388,#12389,#12390,
#12391,#12392,#12393,#12394,#12395,#12396,#12397,#12398,#12399,#12400,#12401,
#12402,#12403,#12404,#12405,#12406,#12407,#12408,#12409,#12410,#12411,#12412,
#12413,#12414,#12415,#12416,#12417,#12418,#12419,#12420,#12421,#12422,#12423,
#12424,#12425,#12426,#12427,#12428,#12429,#12430,#12431,#12432,#12433,#12434,
#12435,#12436,#12437,#12438,#12439,#12440,#12441,#12442,#12443,#12444,#12445,
#12446,#12447,#12448,#12449,#12450,#12451,#12452,#12453,#12454,#12455,#12456,
#12457,#12458,#12459,#12460,#12461,#12462,#12463,#12464,#12465,#12466,#12467,
#12468,#12469,#12470,#12471,#12472,#12473,#12474,#12475,#12476,#12477,#12478,
#12479,#12480,#12481,#12482,#12483,#12484,#12485,#12486,#12487,#12488,#12489,
#12490,#12491,#12492,#12493,#12494,#12495,#12496,#12497,#12498,#12499,#12500,
#12501,#12502,#12503,#12504,#12505,#12506),(#12507,#12508,#12509,#12510,
#12511,#12512,#12513,#12514,#12515,#12516,#12517,#12518,#12519,#12520,#12521,
#12522,#12523,#12524,#12525,#12526,#12527,#12528,#12529,#12530,#12531,#12532,
#12533,#12534,#12535,#12536,#12537,#12538,#12539,#12540,#12541,#12542,#12543,
#12544,#12545,#12546,#12547,#12548,#12549,#12550,#12551,#12552,#12553,#12554,
#12555,#12556,#12557,#12558,#12559,#12560,#12561,#12562,#12563,#12564,#12565,
#12566,#12567,#12568,#12569,#12570,#12571,#12572,#12573,#12574,#12575,#12576,
#12577,#12578,#12579,#12580,#12581,#12582,#12583,#12584,#12585,#12586,#12587,
#12588,#12589,#12590,#12591,#12592,#12593,#12594,#12595,#12596,#12597,#12598,
#12599,#12600,#12601,#12602,#12603,#12604,#12605,#12606,#12607,#12608,#12609,
#12610,#12611,#12612,#12613,#12614,#12615,#12616,#12617,#12618,#12619,#12620,
#12621,#12622,#12623,#12624,#12625,#12626,#12627,#12628,#12629,#12630,#12631,
#12632,#12633,#12634,#12635,#12636,#12637,#12638,#12639,#12640,#12641,#12642,
#12643,#12644,#12645,#12646,#12647,#12648,#12649,#12650,#12651)),
 .UNSPECIFIED.,.F.,.F.,.F.)
B_SPLINE_SURFACE_WITH_KNOTS((2,2),(3,2,2,2,2,2,2,2,2,2,2,2,2,2,2,2,2,2,
2,2,2,2,2,2,2,2,2,2,2,2,2,2,2,2,2,2,2,2,2,2,2,2,2,2,2,2,2,2,2,2,2,2,2,2,
2,2,2,2,2,2,2,2,2,2,2,2,2,2,2,2,2,2,3),(0.,1.),(0.,0.0138888888888889,0.0277777777777778,
0.0416666666666667,0.0555555555555556,0.0694444444444444,0.0833333333333333,
0.0972222222222222,0.111111111111111,0.125,0.138888888888889,0.152777777777778,
0.166666666666667,0.180555555555556,0.194444444444444,0.208333333333333,
0.222222222222222,0.236111111111111,0.25,0.263888888888889,0.277777777777778,
0.291666666666667,0.305555555555556,0.319444444444444,0.333333333333333,
0.347222222222222,0.361111111111111,0.375,0.388888888888889,0.402777777777778,
0.416666666666667,0.430555555555556,0.444444444444444,0.458333333333333,
0.472222222222222,0.486111111111111,0.5,0.513888888888889,0.527777777777778,
0.541666666666667,0.555555555555556,0.569444444444444,0.583333333333333,
0.597222222222222,0.611111111111111,0.625,0.638888888888889,0.652777777777778,
0.666666666666667,0.680555555555556,0.694444444444444,0.708333333333333,
0.722222222222222,0.736111111111111,0.75,0.763888888888889,0.777777777777778,
0.791666666666667,0.805555555555556,0.819444444444444,0.833333333333333,
0.847222222222222,0.861111111111111,0.875,0.888888888888889,0.902777777777778,
0.916666666666667,0.930555555555556,0.944444444444444,0.958333333333333,
0.972222222222222,0.986111111111111,1.),.UNSPECIFIED.)
GEOMETRIC_REPRESENTATION_ITEM()
RATIONAL_B_SPLINE_SURFACE(((1.,0.965925826289068,1.,0.965925826289068,1.,
0.965925826289068,1.,0.965925826289068,1.,0.965925826289068,1.,0.965925826289068,
1.,0.965925826289068,1.,0.965925826289068,1.,0.965925826289068,1.,0.965925826289068,
1.,0.965925826289068,1.,0.965925826289068,1.,0.965925826289068,1.,0.965925826289068,
1.,0.965925826289068,1.,0.965925826289068,1.,0.965925826289068,1.,0.965925826289068,
1.,0.965925826289068,1.,0.965925826289068,1.,0.965925826289068,1.,0.965925826289068,
1.,0.965925826289068,1.,0.965925826289068,1.,0.965925826289068,1.,0.965925826289068,
1.,0.965925826289068,1.,0.965925826289068,1.,0.965925826289068,1.,0.965925826289068,
1.,0.965925826289068,1.,0.965925826289068,1.,0.965925826289068,1.,0.965925826289068,
1.,0.965925826289068,1.,0.965925826289068,1.,0.965925826289068,1.,0.965925826289068,
1.,0.965925826289068,1.,0.965925826289068,1.,0.965925826289068,1.,0.965925826289068,
1.,0.965925826289068,1.,0.965925826289068,1.,0.965925826289068,1.,0.965925826289068,
1.,0.965925826289068,1.,0.965925826289068,1.,0.965925826289068,1.,0.965925826289068,
1.,0.965925826289068,1.,0.965925826289068,1.,0.965925826289068,1.,0.965925826289068,
1.,0.965925826289068,1.,0.965925826289068,1.,0.965925826289068,1.,0.965925826289068,
1.,0.965925826289068,1.,0.965925826289068,1.,0.965925826289068,1.,0.965925826289068,
1.,0.965925826289068,1.,0.965925826289068,1.,0.965925826289068,1.,0.965925826289068,
1.,0.965925826289068,1.,0.965925826289068,1.,0.965925826289068,1.,0.965925826289068,
1.,0.965925826289068,1.,0.965925826289068,1.),(1.,0.965925826289068,1.,
0.965925826289068,1.,0.965925826289068,1.,0.965925826289068,1.,0.965925826289068,
1.,0.965925826289068,1.,0.965925826289068,1.,0.965925826289068,1.,0.965925826289068,
1.,0.965925826289068,1.,0.965925826289068,1.,0.965925826289068,1.,0.965925826289068,
1.,0.965925826289068,1.,0.965925826289068,1.,0.965925826289068,1.,0.965925826289068,
1.,0.965925826289068,1.,0.965925826289068,1.,0.965925826289068,1.,0.965925826289068,
1.,0.965925826289068,1.,0.965925826289068,1.,0.965925826289068,1.,0.965925826289068,
1.,0.965925826289068,1.,0.965925826289068,1.,0.965925826289068,1.,0.965925826289068,
1.,0.965925826289068,1.,0.965925826289068,1.,0.965925826289068,1.,0.965925826289068,
1.,0.965925826289068,1.,0.965925826289068,1.,0.965925826289068,1.,0.965925826289068,
1.,0.965925826289068,1.,0.965925826289068,1.,0.965925826289068,1.,0.965925826289068,
1.,0.965925826289068,1.,0.965925826289068,1.,0.965925826289068,1.,0.965925826289068,
1.,0.965925826289068,1.,0.965925826289068,1.,0.965925826289068,1.,0.965925826289068,
1.,0.965925826289068,1.,0.965925826289068,1.,0.965925826289068,1.,0.965925826289068,
1.,0.965925826289068,1.,0.965925826289068,1.,0.965925826289068,1.,0.965925826289068,
1.,0.965925826289068,1.,0.965925826289068,1.,0.965925826289068,1.,0.965925826289068,
1.,0.965925826289068,1.,0.965925826289068,1.,0.965925826289068,1.,0.965925826289068,
1.,0.965925826289068,1.,0.965925826289068,1.,0.965925826289068,1.,0.965925826289068,
1.,0.965925826289068,1.,0.965925826289068,1.,0.965925826289068,1.)))
REPRESENTATION_ITEM('')
SURFACE()
);
#174=(
BOUNDED_SURFACE()
B_SPLINE_SURFACE(1,2,((#12668,#12669,#12670,#12671,#12672,#12673,#12674,
#12675,#12676,#12677,#12678,#12679,#12680,#12681,#12682,#12683,#12684,#12685,
#12686,#12687,#12688,#12689,#12690,#12691,#12692,#12693,#12694,#12695,#12696,
#12697,#12698,#12699,#12700,#12701,#12702,#12703,#12704,#12705,#12706,#12707,
#12708,#12709,#12710,#12711,#12712,#12713,#12714,#12715,#12716,#12717,#12718,
#12719,#12720,#12721,#12722,#12723,#12724,#12725,#12726,#12727,#12728,#12729,
#12730,#12731,#12732,#12733,#12734,#12735,#12736,#12737,#12738,#12739,#12740,
#12741,#12742,#12743,#12744,#12745,#12746,#12747,#12748,#12749,#12750,#12751,
#12752,#12753,#12754,#12755,#12756,#12757,#12758,#12759,#12760,#12761,#12762,
#12763,#12764,#12765,#12766,#12767,#12768,#12769,#12770,#12771,#12772,#12773,
#12774,#12775,#12776,#12777,#12778,#12779,#12780,#12781,#12782,#12783,#12784,
#12785,#12786,#12787,#12788,#12789,#12790,#12791,#12792,#12793,#12794,#12795,
#12796,#12797,#12798,#12799,#12800,#12801,#12802,#12803,#12804,#12805,#12806,
#12807,#12808,#12809,#12810,#12811,#12812),(#12813,#12814,#12815,#12816,
#12817,#12818,#12819,#12820,#12821,#12822,#12823,#12824,#12825,#12826,#12827,
#12828,#12829,#12830,#12831,#12832,#12833,#12834,#12835,#12836,#12837,#12838,
#12839,#12840,#12841,#12842,#12843,#12844,#12845,#12846,#12847,#12848,#12849,
#12850,#12851,#12852,#12853,#12854,#12855,#12856,#12857,#12858,#12859,#12860,
#12861,#12862,#12863,#12864,#12865,#12866,#12867,#12868,#12869,#12870,#12871,
#12872,#12873,#12874,#12875,#12876,#12877,#12878,#12879,#12880,#12881,#12882,
#12883,#12884,#12885,#12886,#12887,#12888,#12889,#12890,#12891,#12892,#12893,
#12894,#12895,#12896,#12897,#12898,#12899,#12900,#12901,#12902,#12903,#12904,
#12905,#12906,#12907,#12908,#12909,#12910,#12911,#12912,#12913,#12914,#12915,
#12916,#12917,#12918,#12919,#12920,#12921,#12922,#12923,#12924,#12925,#12926,
#12927,#12928,#12929,#12930,#12931,#12932,#12933,#12934,#12935,#12936,#12937,
#12938,#12939,#12940,#12941,#12942,#12943,#12944,#12945,#12946,#12947,#12948,
#12949,#12950,#12951,#12952,#12953,#12954,#12955,#12956,#12957)),
 .UNSPECIFIED.,.F.,.F.,.F.)
B_SPLINE_SURFACE_WITH_KNOTS((2,2),(3,2,2,2,2,2,2,2,2,2,2,2,2,2,2,2,2,2,
2,2,2,2,2,2,2,2,2,2,2,2,2,2,2,2,2,2,2,2,2,2,2,2,2,2,2,2,2,2,2,2,2,2,2,2,
2,2,2,2,2,2,2,2,2,2,2,2,2,2,2,2,2,2,3),(0.,1.),(0.,0.0138888888888889,0.0277777777777778,
0.0416666666666667,0.0555555555555556,0.0694444444444444,0.0833333333333333,
0.0972222222222222,0.111111111111111,0.125,0.138888888888889,0.152777777777778,
0.166666666666667,0.180555555555556,0.194444444444444,0.208333333333333,
0.222222222222222,0.236111111111111,0.25,0.263888888888889,0.277777777777778,
0.291666666666667,0.305555555555556,0.319444444444444,0.333333333333333,
0.347222222222222,0.361111111111111,0.375,0.388888888888889,0.402777777777778,
0.416666666666667,0.430555555555556,0.444444444444444,0.458333333333333,
0.472222222222222,0.486111111111111,0.5,0.513888888888889,0.527777777777778,
0.541666666666667,0.555555555555556,0.569444444444444,0.583333333333333,
0.597222222222222,0.611111111111111,0.625,0.638888888888889,0.652777777777778,
0.666666666666667,0.680555555555556,0.694444444444444,0.708333333333333,
0.722222222222222,0.736111111111111,0.75,0.763888888888889,0.777777777777778,
0.791666666666667,0.805555555555556,0.819444444444444,0.833333333333333,
0.847222222222222,0.861111111111111,0.875,0.888888888888889,0.902777777777778,
0.916666666666667,0.930555555555556,0.944444444444444,0.958333333333333,
0.972222222222222,0.986111111111111,1.),.UNSPECIFIED.)
GEOMETRIC_REPRESENTATION_ITEM()
RATIONAL_B_SPLINE_SURFACE(((1.,0.965925826289068,1.,0.965925826289068,1.,
0.965925826289068,1.,0.965925826289068,1.,0.965925826289068,1.,0.965925826289068,
1.,0.965925826289068,1.,0.965925826289068,1.,0.965925826289068,1.,0.965925826289068,
1.,0.965925826289068,1.,0.965925826289068,1.,0.965925826289068,1.,0.965925826289068,
1.,0.965925826289068,1.,0.965925826289068,1.,0.965925826289068,1.,0.965925826289068,
1.,0.965925826289068,1.,0.965925826289068,1.,0.965925826289068,1.,0.965925826289068,
1.,0.965925826289068,1.,0.965925826289068,1.,0.965925826289068,1.,0.965925826289068,
1.,0.965925826289068,1.,0.965925826289068,1.,0.965925826289068,1.,0.965925826289068,
1.,0.965925826289068,1.,0.965925826289068,1.,0.965925826289068,1.,0.965925826289068,
1.,0.965925826289068,1.,0.965925826289068,1.,0.965925826289068,1.,0.965925826289068,
1.,0.965925826289068,1.,0.965925826289068,1.,0.965925826289068,1.,0.965925826289068,
1.,0.965925826289068,1.,0.965925826289068,1.,0.965925826289068,1.,0.965925826289068,
1.,0.965925826289068,1.,0.965925826289068,1.,0.965925826289068,1.,0.965925826289068,
1.,0.965925826289068,1.,0.965925826289068,1.,0.965925826289068,1.,0.965925826289068,
1.,0.965925826289068,1.,0.965925826289068,1.,0.965925826289068,1.,0.965925826289068,
1.,0.965925826289068,1.,0.965925826289068,1.,0.965925826289068,1.,0.965925826289068,
1.,0.965925826289068,1.,0.965925826289068,1.,0.965925826289068,1.,0.965925826289068,
1.,0.965925826289068,1.,0.965925826289068,1.,0.965925826289068,1.,0.965925826289068,
1.,0.965925826289068,1.,0.965925826289068,1.),(1.,0.965925826289068,1.,
0.965925826289068,1.,0.965925826289068,1.,0.965925826289068,1.,0.965925826289068,
1.,0.965925826289068,1.,0.965925826289068,1.,0.965925826289068,1.,0.965925826289068,
1.,0.965925826289068,1.,0.965925826289068,1.,0.965925826289068,1.,0.965925826289068,
1.,0.965925826289068,1.,0.965925826289068,1.,0.965925826289068,1.,0.965925826289068,
1.,0.965925826289068,1.,0.965925826289068,1.,0.965925826289068,1.,0.965925826289068,
1.,0.965925826289068,1.,0.965925826289068,1.,0.965925826289068,1.,0.965925826289068,
1.,0.965925826289068,1.,0.965925826289068,1.,0.965925826289068,1.,0.965925826289068,
1.,0.965925826289068,1.,0.965925826289068,1.,0.965925826289068,1.,0.965925826289068,
1.,0.965925826289068,1.,0.965925826289068,1.,0.965925826289068,1.,0.965925826289068,
1.,0.965925826289068,1.,0.965925826289068,1.,0.965925826289068,1.,0.965925826289068,
1.,0.965925826289068,1.,0.965925826289068,1.,0.965925826289068,1.,0.965925826289068,
1.,0.965925826289068,1.,0.965925826289068,1.,0.965925826289068,1.,0.965925826289068,
1.,0.965925826289068,1.,0.965925826289068,1.,0.965925826289068,1.,0.965925826289068,
1.,0.965925826289068,1.,0.965925826289068,1.,0.965925826289068,1.,0.965925826289068,
1.,0.965925826289068,1.,0.965925826289068,1.,0.965925826289068,1.,0.965925826289068,
1.,0.965925826289068,1.,0.965925826289068,1.,0.965925826289068,1.,0.965925826289068,
1.,0.965925826289068,1.,0.965925826289068,1.,0.965925826289068,1.,0.965925826289068,
1.,0.965925826289068,1.,0.965925826289068,1.,0.965925826289068,1.)))
REPRESENTATION_ITEM('')
SURFACE()
);
#175=(
BOUNDED_SURFACE()
B_SPLINE_SURFACE(1,2,((#12974,#12975,#12976,#12977,#12978,#12979,#12980,
#12981,#12982,#12983,#12984,#12985,#12986,#12987,#12988,#12989,#12990,#12991,
#12992,#12993,#12994,#12995,#12996,#12997,#12998,#12999,#13000,#13001,#13002,
#13003,#13004,#13005,#13006,#13007,#13008,#13009,#13010,#13011,#13012,#13013,
#13014,#13015,#13016,#13017,#13018,#13019,#13020,#13021,#13022,#13023,#13024,
#13025,#13026,#13027,#13028,#13029,#13030,#13031,#13032,#13033,#13034,#13035,
#13036,#13037,#13038,#13039,#13040,#13041,#13042,#13043,#13044,#13045,#13046,
#13047,#13048,#13049,#13050,#13051,#13052,#13053,#13054,#13055,#13056,#13057,
#13058,#13059,#13060,#13061,#13062,#13063,#13064,#13065,#13066,#13067,#13068,
#13069,#13070,#13071,#13072,#13073,#13074,#13075,#13076,#13077,#13078,#13079,
#13080,#13081,#13082,#13083,#13084,#13085,#13086,#13087,#13088,#13089,#13090,
#13091,#13092,#13093,#13094,#13095,#13096,#13097,#13098,#13099,#13100,#13101,
#13102,#13103,#13104,#13105,#13106,#13107,#13108,#13109,#13110,#13111,#13112,
#13113,#13114,#13115,#13116,#13117,#13118),(#13119,#13120,#13121,#13122,
#13123,#13124,#13125,#13126,#13127,#13128,#13129,#13130,#13131,#13132,#13133,
#13134,#13135,#13136,#13137,#13138,#13139,#13140,#13141,#13142,#13143,#13144,
#13145,#13146,#13147,#13148,#13149,#13150,#13151,#13152,#13153,#13154,#13155,
#13156,#13157,#13158,#13159,#13160,#13161,#13162,#13163,#13164,#13165,#13166,
#13167,#13168,#13169,#13170,#13171,#13172,#13173,#13174,#13175,#13176,#13177,
#13178,#13179,#13180,#13181,#13182,#13183,#13184,#13185,#13186,#13187,#13188,
#13189,#13190,#13191,#13192,#13193,#13194,#13195,#13196,#13197,#13198,#13199,
#13200,#13201,#13202,#13203,#13204,#13205,#13206,#13207,#13208,#13209,#13210,
#13211,#13212,#13213,#13214,#13215,#13216,#13217,#13218,#13219,#13220,#13221,
#13222,#13223,#13224,#13225,#13226,#13227,#13228,#13229,#13230,#13231,#13232,
#13233,#13234,#13235,#13236,#13237,#13238,#13239,#13240,#13241,#13242,#13243,
#13244,#13245,#13246,#13247,#13248,#13249,#13250,#13251,#13252,#13253,#13254,
#13255,#13256,#13257,#13258,#13259,#13260,#13261,#13262,#13263)),
 .UNSPECIFIED.,.F.,.F.,.F.)
B_SPLINE_SURFACE_WITH_KNOTS((2,2),(3,2,2,2,2,2,2,2,2,2,2,2,2,2,2,2,2,2,
2,2,2,2,2,2,2,2,2,2,2,2,2,2,2,2,2,2,2,2,2,2,2,2,2,2,2,2,2,2,2,2,2,2,2,2,
2,2,2,2,2,2,2,2,2,2,2,2,2,2,2,2,2,2,3),(0.,1.),(0.,0.0138888888888889,0.0277777777777778,
0.0416666666666667,0.0555555555555556,0.0694444444444444,0.0833333333333333,
0.0972222222222222,0.111111111111111,0.125,0.138888888888889,0.152777777777778,
0.166666666666667,0.180555555555556,0.194444444444444,0.208333333333333,
0.222222222222222,0.236111111111111,0.25,0.263888888888889,0.277777777777778,
0.291666666666667,0.305555555555556,0.319444444444444,0.333333333333333,
0.347222222222222,0.361111111111111,0.375,0.388888888888889,0.402777777777778,
0.416666666666667,0.430555555555556,0.444444444444444,0.458333333333333,
0.472222222222222,0.486111111111111,0.5,0.513888888888889,0.527777777777778,
0.541666666666667,0.555555555555556,0.569444444444444,0.583333333333333,
0.597222222222222,0.611111111111111,0.625,0.638888888888889,0.652777777777778,
0.666666666666667,0.680555555555556,0.694444444444444,0.708333333333333,
0.722222222222222,0.736111111111111,0.75,0.763888888888889,0.777777777777778,
0.791666666666667,0.805555555555556,0.819444444444444,0.833333333333333,
0.847222222222222,0.861111111111111,0.875,0.888888888888889,0.902777777777778,
0.916666666666667,0.930555555555556,0.944444444444444,0.958333333333333,
0.972222222222222,0.986111111111111,1.),.UNSPECIFIED.)
GEOMETRIC_REPRESENTATION_ITEM()
RATIONAL_B_SPLINE_SURFACE(((1.,0.965925826289068,1.,0.965925826289068,1.,
0.965925826289068,1.,0.965925826289068,1.,0.965925826289068,1.,0.965925826289068,
1.,0.965925826289068,1.,0.965925826289068,1.,0.965925826289068,1.,0.965925826289068,
1.,0.965925826289068,1.,0.965925826289068,1.,0.965925826289068,1.,0.965925826289068,
1.,0.965925826289068,1.,0.965925826289068,1.,0.965925826289068,1.,0.965925826289068,
1.,0.965925826289068,1.,0.965925826289068,1.,0.965925826289068,1.,0.965925826289068,
1.,0.965925826289068,1.,0.965925826289068,1.,0.965925826289068,1.,0.965925826289068,
1.,0.965925826289068,1.,0.965925826289068,1.,0.965925826289068,1.,0.965925826289068,
1.,0.965925826289068,1.,0.965925826289068,1.,0.965925826289068,1.,0.965925826289068,
1.,0.965925826289068,1.,0.965925826289068,1.,0.965925826289068,1.,0.965925826289068,
1.,0.965925826289068,1.,0.965925826289068,1.,0.965925826289068,1.,0.965925826289068,
1.,0.965925826289068,1.,0.965925826289068,1.,0.965925826289068,1.,0.965925826289068,
1.,0.965925826289068,1.,0.965925826289068,1.,0.965925826289068,1.,0.965925826289068,
1.,0.965925826289068,1.,0.965925826289068,1.,0.965925826289068,1.,0.965925826289068,
1.,0.965925826289068,1.,0.965925826289068,1.,0.965925826289068,1.,0.965925826289068,
1.,0.965925826289068,1.,0.965925826289068,1.,0.965925826289068,1.,0.965925826289068,
1.,0.965925826289068,1.,0.965925826289068,1.,0.965925826289068,1.,0.965925826289068,
1.,0.965925826289068,1.,0.965925826289068,1.,0.965925826289068,1.,0.965925826289068,
1.,0.965925826289068,1.,0.965925826289068,1.),(1.,0.965925826289068,1.,
0.965925826289068,1.,0.965925826289068,1.,0.965925826289068,1.,0.965925826289068,
1.,0.965925826289068,1.,0.965925826289068,1.,0.965925826289068,1.,0.965925826289068,
1.,0.965925826289068,1.,0.965925826289068,1.,0.965925826289068,1.,0.965925826289068,
1.,0.965925826289068,1.,0.965925826289068,1.,0.965925826289068,1.,0.965925826289068,
1.,0.965925826289068,1.,0.965925826289068,1.,0.965925826289068,1.,0.965925826289068,
1.,0.965925826289068,1.,0.965925826289068,1.,0.965925826289068,1.,0.965925826289068,
1.,0.965925826289068,1.,0.965925826289068,1.,0.965925826289068,1.,0.965925826289068,
1.,0.965925826289068,1.,0.965925826289068,1.,0.965925826289068,1.,0.965925826289068,
1.,0.965925826289068,1.,0.965925826289068,1.,0.965925826289068,1.,0.965925826289068,
1.,0.965925826289068,1.,0.965925826289068,1.,0.965925826289068,1.,0.965925826289068,
1.,0.965925826289068,1.,0.965925826289068,1.,0.965925826289068,1.,0.965925826289068,
1.,0.965925826289068,1.,0.965925826289068,1.,0.965925826289068,1.,0.965925826289068,
1.,0.965925826289068,1.,0.965925826289068,1.,0.965925826289068,1.,0.965925826289068,
1.,0.965925826289068,1.,0.965925826289068,1.,0.965925826289068,1.,0.965925826289068,
1.,0.965925826289068,1.,0.965925826289068,1.,0.965925826289068,1.,0.965925826289068,
1.,0.965925826289068,1.,0.965925826289068,1.,0.965925826289068,1.,0.965925826289068,
1.,0.965925826289068,1.,0.965925826289068,1.,0.965925826289068,1.,0.965925826289068,
1.,0.965925826289068,1.,0.965925826289068,1.,0.965925826289068,1.)))
REPRESENTATION_ITEM('')
SURFACE()
);
#176=(
BOUNDED_SURFACE()
B_SPLINE_SURFACE(1,2,((#13280,#13281,#13282,#13283,#13284,#13285,#13286,
#13287,#13288,#13289,#13290,#13291,#13292,#13293,#13294,#13295,#13296,#13297,
#13298,#13299,#13300,#13301,#13302,#13303,#13304,#13305,#13306,#13307,#13308,
#13309,#13310,#13311,#13312,#13313,#13314,#13315,#13316,#13317,#13318,#13319,
#13320,#13321,#13322,#13323,#13324,#13325,#13326,#13327,#13328,#13329,#13330,
#13331,#13332,#13333,#13334,#13335,#13336,#13337,#13338,#13339,#13340,#13341,
#13342,#13343,#13344,#13345,#13346,#13347,#13348,#13349,#13350,#13351,#13352,
#13353,#13354,#13355,#13356,#13357,#13358,#13359,#13360,#13361,#13362,#13363,
#13364,#13365,#13366,#13367,#13368,#13369,#13370,#13371,#13372,#13373,#13374,
#13375,#13376,#13377,#13378,#13379,#13380,#13381,#13382,#13383,#13384,#13385,
#13386,#13387,#13388,#13389,#13390,#13391,#13392,#13393,#13394,#13395,#13396,
#13397,#13398,#13399,#13400,#13401,#13402,#13403,#13404,#13405,#13406,#13407,
#13408,#13409,#13410,#13411,#13412,#13413,#13414,#13415,#13416,#13417,#13418,
#13419,#13420,#13421,#13422,#13423,#13424),(#13425,#13426,#13427,#13428,
#13429,#13430,#13431,#13432,#13433,#13434,#13435,#13436,#13437,#13438,#13439,
#13440,#13441,#13442,#13443,#13444,#13445,#13446,#13447,#13448,#13449,#13450,
#13451,#13452,#13453,#13454,#13455,#13456,#13457,#13458,#13459,#13460,#13461,
#13462,#13463,#13464,#13465,#13466,#13467,#13468,#13469,#13470,#13471,#13472,
#13473,#13474,#13475,#13476,#13477,#13478,#13479,#13480,#13481,#13482,#13483,
#13484,#13485,#13486,#13487,#13488,#13489,#13490,#13491,#13492,#13493,#13494,
#13495,#13496,#13497,#13498,#13499,#13500,#13501,#13502,#13503,#13504,#13505,
#13506,#13507,#13508,#13509,#13510,#13511,#13512,#13513,#13514,#13515,#13516,
#13517,#13518,#13519,#13520,#13521,#13522,#13523,#13524,#13525,#13526,#13527,
#13528,#13529,#13530,#13531,#13532,#13533,#13534,#13535,#13536,#13537,#13538,
#13539,#13540,#13541,#13542,#13543,#13544,#13545,#13546,#13547,#13548,#13549,
#13550,#13551,#13552,#13553,#13554,#13555,#13556,#13557,#13558,#13559,#13560,
#13561,#13562,#13563,#13564,#13565,#13566,#13567,#13568,#13569)),
 .UNSPECIFIED.,.F.,.F.,.F.)
B_SPLINE_SURFACE_WITH_KNOTS((2,2),(3,2,2,2,2,2,2,2,2,2,2,2,2,2,2,2,2,2,
2,2,2,2,2,2,2,2,2,2,2,2,2,2,2,2,2,2,2,2,2,2,2,2,2,2,2,2,2,2,2,2,2,2,2,2,
2,2,2,2,2,2,2,2,2,2,2,2,2,2,2,2,2,2,3),(0.,1.),(0.,0.0138888888888889,0.0277777777777778,
0.0416666666666667,0.0555555555555556,0.0694444444444444,0.0833333333333333,
0.0972222222222222,0.111111111111111,0.125,0.138888888888889,0.152777777777778,
0.166666666666667,0.180555555555556,0.194444444444444,0.208333333333333,
0.222222222222222,0.236111111111111,0.25,0.263888888888889,0.277777777777778,
0.291666666666667,0.305555555555556,0.319444444444444,0.333333333333333,
0.347222222222222,0.361111111111111,0.375,0.388888888888889,0.402777777777778,
0.416666666666667,0.430555555555556,0.444444444444444,0.458333333333333,
0.472222222222222,0.486111111111111,0.5,0.513888888888889,0.527777777777778,
0.541666666666667,0.555555555555556,0.569444444444444,0.583333333333333,
0.597222222222222,0.611111111111111,0.625,0.638888888888889,0.652777777777778,
0.666666666666667,0.680555555555556,0.694444444444444,0.708333333333333,
0.722222222222222,0.736111111111111,0.75,0.763888888888889,0.777777777777778,
0.791666666666667,0.805555555555556,0.819444444444444,0.833333333333333,
0.847222222222222,0.861111111111111,0.875,0.888888888888889,0.902777777777778,
0.916666666666667,0.930555555555556,0.944444444444444,0.958333333333333,
0.972222222222222,0.986111111111111,1.),.UNSPECIFIED.)
GEOMETRIC_REPRESENTATION_ITEM()
RATIONAL_B_SPLINE_SURFACE(((1.,0.965925826289068,1.,0.965925826289068,1.,
0.965925826289068,1.,0.965925826289068,1.,0.965925826289068,1.,0.965925826289068,
1.,0.965925826289068,1.,0.965925826289068,1.,0.965925826289068,1.,0.965925826289068,
1.,0.965925826289068,1.,0.965925826289068,1.,0.965925826289068,1.,0.965925826289068,
1.,0.965925826289068,1.,0.965925826289068,1.,0.965925826289068,1.,0.965925826289068,
1.,0.965925826289068,1.,0.965925826289068,1.,0.965925826289068,1.,0.965925826289068,
1.,0.965925826289068,1.,0.965925826289068,1.,0.965925826289068,1.,0.965925826289068,
1.,0.965925826289068,1.,0.965925826289068,1.,0.965925826289068,1.,0.965925826289068,
1.,0.965925826289068,1.,0.965925826289068,1.,0.965925826289068,1.,0.965925826289068,
1.,0.965925826289068,1.,0.965925826289068,1.,0.965925826289068,1.,0.965925826289068,
1.,0.965925826289068,1.,0.965925826289068,1.,0.965925826289068,1.,0.965925826289068,
1.,0.965925826289068,1.,0.965925826289068,1.,0.965925826289068,1.,0.965925826289068,
1.,0.965925826289068,1.,0.965925826289068,1.,0.965925826289068,1.,0.965925826289068,
1.,0.965925826289068,1.,0.965925826289068,1.,0.965925826289068,1.,0.965925826289068,
1.,0.965925826289068,1.,0.965925826289068,1.,0.965925826289068,1.,0.965925826289068,
1.,0.965925826289068,1.,0.965925826289068,1.,0.965925826289068,1.,0.965925826289068,
1.,0.965925826289068,1.,0.965925826289068,1.,0.965925826289068,1.,0.965925826289068,
1.,0.965925826289068,1.,0.965925826289068,1.,0.965925826289068,1.,0.965925826289068,
1.,0.965925826289068,1.,0.965925826289068,1.),(1.,0.965925826289068,1.,
0.965925826289068,1.,0.965925826289068,1.,0.965925826289068,1.,0.965925826289068,
1.,0.965925826289068,1.,0.965925826289068,1.,0.965925826289068,1.,0.965925826289068,
1.,0.965925826289068,1.,0.965925826289068,1.,0.965925826289068,1.,0.965925826289068,
1.,0.965925826289068,1.,0.965925826289068,1.,0.965925826289068,1.,0.965925826289068,
1.,0.965925826289068,1.,0.965925826289068,1.,0.965925826289068,1.,0.965925826289068,
1.,0.965925826289068,1.,0.965925826289068,1.,0.965925826289068,1.,0.965925826289068,
1.,0.965925826289068,1.,0.965925826289068,1.,0.965925826289068,1.,0.965925826289068,
1.,0.965925826289068,1.,0.965925826289068,1.,0.965925826289068,1.,0.965925826289068,
1.,0.965925826289068,1.,0.965925826289068,1.,0.965925826289068,1.,0.965925826289068,
1.,0.965925826289068,1.,0.965925826289068,1.,0.965925826289068,1.,0.965925826289068,
1.,0.965925826289068,1.,0.965925826289068,1.,0.965925826289068,1.,0.965925826289068,
1.,0.965925826289068,1.,0.965925826289068,1.,0.965925826289068,1.,0.965925826289068,
1.,0.965925826289068,1.,0.965925826289068,1.,0.965925826289068,1.,0.965925826289068,
1.,0.965925826289068,1.,0.965925826289068,1.,0.965925826289068,1.,0.965925826289068,
1.,0.965925826289068,1.,0.965925826289068,1.,0.965925826289068,1.,0.965925826289068,
1.,0.965925826289068,1.,0.965925826289068,1.,0.965925826289068,1.,0.965925826289068,
1.,0.965925826289068,1.,0.965925826289068,1.,0.965925826289068,1.,0.965925826289068,
1.,0.965925826289068,1.,0.965925826289068,1.,0.965925826289068,1.)))
REPRESENTATION_ITEM('')
SURFACE()
);
#177=(
BOUNDED_SURFACE()
B_SPLINE_SURFACE(1,2,((#13586,#13587,#13588,#13589,#13590,#13591,#13592,
#13593,#13594,#13595,#13596,#13597,#13598,#13599,#13600,#13601,#13602,#13603,
#13604,#13605,#13606,#13607,#13608,#13609,#13610,#13611,#13612,#13613,#13614,
#13615,#13616,#13617,#13618,#13619,#13620,#13621,#13622,#13623,#13624,#13625,
#13626,#13627,#13628,#13629,#13630,#13631,#13632,#13633,#13634,#13635,#13636,
#13637,#13638,#13639,#13640,#13641,#13642,#13643,#13644,#13645,#13646,#13647,
#13648,#13649,#13650,#13651,#13652,#13653,#13654,#13655,#13656,#13657,#13658,
#13659,#13660,#13661,#13662,#13663,#13664,#13665,#13666,#13667,#13668,#13669,
#13670,#13671,#13672,#13673,#13674,#13675,#13676,#13677,#13678,#13679,#13680,
#13681,#13682,#13683,#13684,#13685,#13686,#13687,#13688,#13689,#13690,#13691,
#13692,#13693,#13694,#13695,#13696,#13697,#13698,#13699,#13700,#13701,#13702,
#13703,#13704,#13705,#13706,#13707,#13708,#13709,#13710,#13711,#13712,#13713,
#13714,#13715,#13716,#13717,#13718,#13719,#13720,#13721,#13722,#13723,#13724,
#13725,#13726,#13727,#13728,#13729,#13730),(#13731,#13732,#13733,#13734,
#13735,#13736,#13737,#13738,#13739,#13740,#13741,#13742,#13743,#13744,#13745,
#13746,#13747,#13748,#13749,#13750,#13751,#13752,#13753,#13754,#13755,#13756,
#13757,#13758,#13759,#13760,#13761,#13762,#13763,#13764,#13765,#13766,#13767,
#13768,#13769,#13770,#13771,#13772,#13773,#13774,#13775,#13776,#13777,#13778,
#13779,#13780,#13781,#13782,#13783,#13784,#13785,#13786,#13787,#13788,#13789,
#13790,#13791,#13792,#13793,#13794,#13795,#13796,#13797,#13798,#13799,#13800,
#13801,#13802,#13803,#13804,#13805,#13806,#13807,#13808,#13809,#13810,#13811,
#13812,#13813,#13814,#13815,#13816,#13817,#13818,#13819,#13820,#13821,#13822,
#13823,#13824,#13825,#13826,#13827,#13828,#13829,#13830,#13831,#13832,#13833,
#13834,#13835,#13836,#13837,#13838,#13839,#13840,#13841,#13842,#13843,#13844,
#13845,#13846,#13847,#13848,#13849,#13850,#13851,#13852,#13853,#13854,#13855,
#13856,#13857,#13858,#13859,#13860,#13861,#13862,#13863,#13864,#13865,#13866,
#13867,#13868,#13869,#13870,#13871,#13872,#13873,#13874,#13875)),
 .UNSPECIFIED.,.F.,.F.,.F.)
B_SPLINE_SURFACE_WITH_KNOTS((2,2),(3,2,2,2,2,2,2,2,2,2,2,2,2,2,2,2,2,2,
2,2,2,2,2,2,2,2,2,2,2,2,2,2,2,2,2,2,2,2,2,2,2,2,2,2,2,2,2,2,2,2,2,2,2,2,
2,2,2,2,2,2,2,2,2,2,2,2,2,2,2,2,2,2,3),(0.,1.),(0.,0.0138888888888889,0.0277777777777778,
0.0416666666666667,0.0555555555555556,0.0694444444444444,0.0833333333333333,
0.0972222222222222,0.111111111111111,0.125,0.138888888888889,0.152777777777778,
0.166666666666667,0.180555555555556,0.194444444444444,0.208333333333333,
0.222222222222222,0.236111111111111,0.25,0.263888888888889,0.277777777777778,
0.291666666666667,0.305555555555556,0.319444444444444,0.333333333333333,
0.347222222222222,0.361111111111111,0.375,0.388888888888889,0.402777777777778,
0.416666666666667,0.430555555555556,0.444444444444444,0.458333333333333,
0.472222222222222,0.486111111111111,0.5,0.513888888888889,0.527777777777778,
0.541666666666667,0.555555555555556,0.569444444444444,0.583333333333333,
0.597222222222222,0.611111111111111,0.625,0.638888888888889,0.652777777777778,
0.666666666666667,0.680555555555556,0.694444444444444,0.708333333333333,
0.722222222222222,0.736111111111111,0.75,0.763888888888889,0.777777777777778,
0.791666666666667,0.805555555555556,0.819444444444444,0.833333333333333,
0.847222222222222,0.861111111111111,0.875,0.888888888888889,0.902777777777778,
0.916666666666667,0.930555555555556,0.944444444444444,0.958333333333333,
0.972222222222222,0.986111111111111,1.),.UNSPECIFIED.)
GEOMETRIC_REPRESENTATION_ITEM()
RATIONAL_B_SPLINE_SURFACE(((1.,0.965925826289068,1.,0.965925826289068,1.,
0.965925826289068,1.,0.965925826289068,1.,0.965925826289068,1.,0.965925826289068,
1.,0.965925826289068,1.,0.965925826289068,1.,0.965925826289068,1.,0.965925826289068,
1.,0.965925826289068,1.,0.965925826289068,1.,0.965925826289068,1.,0.965925826289068,
1.,0.965925826289068,1.,0.965925826289068,1.,0.965925826289068,1.,0.965925826289068,
1.,0.965925826289068,1.,0.965925826289068,1.,0.965925826289068,1.,0.965925826289068,
1.,0.965925826289068,1.,0.965925826289068,1.,0.965925826289068,1.,0.965925826289068,
1.,0.965925826289068,1.,0.965925826289068,1.,0.965925826289068,1.,0.965925826289068,
1.,0.965925826289068,1.,0.965925826289068,1.,0.965925826289068,1.,0.965925826289068,
1.,0.965925826289068,1.,0.965925826289068,1.,0.965925826289068,1.,0.965925826289068,
1.,0.965925826289068,1.,0.965925826289068,1.,0.965925826289068,1.,0.965925826289068,
1.,0.965925826289068,1.,0.965925826289068,1.,0.965925826289068,1.,0.965925826289068,
1.,0.965925826289068,1.,0.965925826289068,1.,0.965925826289068,1.,0.965925826289068,
1.,0.965925826289068,1.,0.965925826289068,1.,0.965925826289068,1.,0.965925826289068,
1.,0.965925826289068,1.,0.965925826289068,1.,0.965925826289068,1.,0.965925826289068,
1.,0.965925826289068,1.,0.965925826289068,1.,0.965925826289068,1.,0.965925826289068,
1.,0.965925826289068,1.,0.965925826289068,1.,0.965925826289068,1.,0.965925826289068,
1.,0.965925826289068,1.,0.965925826289068,1.,0.965925826289068,1.,0.965925826289068,
1.,0.965925826289068,1.,0.965925826289068,1.),(1.,0.965925826289068,1.,
0.965925826289068,1.,0.965925826289068,1.,0.965925826289068,1.,0.965925826289068,
1.,0.965925826289068,1.,0.965925826289068,1.,0.965925826289068,1.,0.965925826289068,
1.,0.965925826289068,1.,0.965925826289068,1.,0.965925826289068,1.,0.965925826289068,
1.,0.965925826289068,1.,0.965925826289068,1.,0.965925826289068,1.,0.965925826289068,
1.,0.965925826289068,1.,0.965925826289068,1.,0.965925826289068,1.,0.965925826289068,
1.,0.965925826289068,1.,0.965925826289068,1.,0.965925826289068,1.,0.965925826289068,
1.,0.965925826289068,1.,0.965925826289068,1.,0.965925826289068,1.,0.965925826289068,
1.,0.965925826289068,1.,0.965925826289068,1.,0.965925826289068,1.,0.965925826289068,
1.,0.965925826289068,1.,0.965925826289068,1.,0.965925826289068,1.,0.965925826289068,
1.,0.965925826289068,1.,0.965925826289068,1.,0.965925826289068,1.,0.965925826289068,
1.,0.965925826289068,1.,0.965925826289068,1.,0.965925826289068,1.,0.965925826289068,
1.,0.965925826289068,1.,0.965925826289068,1.,0.965925826289068,1.,0.965925826289068,
1.,0.965925826289068,1.,0.965925826289068,1.,0.965925826289068,1.,0.965925826289068,
1.,0.965925826289068,1.,0.965925826289068,1.,0.965925826289068,1.,0.965925826289068,
1.,0.965925826289068,1.,0.965925826289068,1.,0.965925826289068,1.,0.965925826289068,
1.,0.965925826289068,1.,0.965925826289068,1.,0.965925826289068,1.,0.965925826289068,
1.,0.965925826289068,1.,0.965925826289068,1.,0.965925826289068,1.,0.965925826289068,
1.,0.965925826289068,1.,0.965925826289068,1.,0.965925826289068,1.)))
REPRESENTATION_ITEM('')
SURFACE()
);
#178=(
BOUNDED_SURFACE()
B_SPLINE_SURFACE(1,2,((#13887,#13888,#13889,#13890,#13891,#13892,#13893,
#13894,#13895,#13896,#13897,#13898,#13899,#13900,#13901,#13902,#13903,#13904,
#13905,#13906,#13907,#13908,#13909,#13910,#13911,#13912,#13913,#13914,#13915,
#13916,#13917,#13918,#13919,#13920,#13921,#13922,#13923,#13924,#13925,#13926,
#13927,#13928,#13929,#13930,#13931,#13932,#13933,#13934,#13935,#13936,#13937,
#13938,#13939,#13940,#13941,#13942,#13943,#13944,#13945,#13946,#13947,#13948,
#13949,#13950,#13951,#13952,#13953,#13954,#13955,#13956,#13957,#13958,#13959,
#13960,#13961,#13962,#13963,#13964,#13965,#13966,#13967,#13968,#13969,#13970,
#13971,#13972,#13973,#13974,#13975,#13976,#13977,#13978,#13979,#13980,#13981,
#13982,#13983,#13984,#13985,#13986,#13987,#13988,#13989,#13990,#13991,#13992,
#13993,#13994,#13995,#13996,#13997,#13998,#13999,#14000,#14001,#14002,#14003,
#14004,#14005,#14006,#14007,#14008,#14009,#14010,#14011,#14012,#14013,#14014,
#14015,#14016,#14017,#14018,#14019,#14020,#14021,#14022,#14023,#14024,#14025,
#14026,#14027,#14028,#14029,#14030,#14031),(#14032,#14033,#14034,#14035,
#14036,#14037,#14038,#14039,#14040,#14041,#14042,#14043,#14044,#14045,#14046,
#14047,#14048,#14049,#14050,#14051,#14052,#14053,#14054,#14055,#14056,#14057,
#14058,#14059,#14060,#14061,#14062,#14063,#14064,#14065,#14066,#14067,#14068,
#14069,#14070,#14071,#14072,#14073,#14074,#14075,#14076,#14077,#14078,#14079,
#14080,#14081,#14082,#14083,#14084,#14085,#14086,#14087,#14088,#14089,#14090,
#14091,#14092,#14093,#14094,#14095,#14096,#14097,#14098,#14099,#14100,#14101,
#14102,#14103,#14104,#14105,#14106,#14107,#14108,#14109,#14110,#14111,#14112,
#14113,#14114,#14115,#14116,#14117,#14118,#14119,#14120,#14121,#14122,#14123,
#14124,#14125,#14126,#14127,#14128,#14129,#14130,#14131,#14132,#14133,#14134,
#14135,#14136,#14137,#14138,#14139,#14140,#14141,#14142,#14143,#14144,#14145,
#14146,#14147,#14148,#14149,#14150,#14151,#14152,#14153,#14154,#14155,#14156,
#14157,#14158,#14159,#14160,#14161,#14162,#14163,#14164,#14165,#14166,#14167,
#14168,#14169,#14170,#14171,#14172,#14173,#14174,#14175,#14176)),
 .UNSPECIFIED.,.F.,.F.,.F.)
B_SPLINE_SURFACE_WITH_KNOTS((2,2),(3,2,2,2,2,2,2,2,2,2,2,2,2,2,2,2,2,2,
2,2,2,2,2,2,2,2,2,2,2,2,2,2,2,2,2,2,2,2,2,2,2,2,2,2,2,2,2,2,2,2,2,2,2,2,
2,2,2,2,2,2,2,2,2,2,2,2,2,2,2,2,2,2,3),(0.,1.),(0.,0.0138888888888889,0.0277777777777778,
0.0416666666666667,0.0555555555555556,0.0694444444444444,0.0833333333333333,
0.0972222222222222,0.111111111111111,0.125,0.138888888888889,0.152777777777778,
0.166666666666667,0.180555555555556,0.194444444444444,0.208333333333333,
0.222222222222222,0.236111111111111,0.25,0.263888888888889,0.277777777777778,
0.291666666666667,0.305555555555556,0.319444444444444,0.333333333333333,
0.347222222222222,0.361111111111111,0.375,0.388888888888889,0.402777777777778,
0.416666666666667,0.430555555555556,0.444444444444444,0.458333333333333,
0.472222222222222,0.486111111111111,0.5,0.513888888888889,0.527777777777778,
0.541666666666667,0.555555555555556,0.569444444444444,0.583333333333333,
0.597222222222222,0.611111111111111,0.625,0.638888888888889,0.652777777777778,
0.666666666666667,0.680555555555556,0.694444444444444,0.708333333333333,
0.722222222222222,0.736111111111111,0.75,0.763888888888889,0.777777777777778,
0.791666666666667,0.805555555555556,0.819444444444444,0.833333333333333,
0.847222222222222,0.861111111111111,0.875,0.888888888888889,0.902777777777778,
0.916666666666667,0.930555555555556,0.944444444444444,0.958333333333333,
0.972222222222222,0.986111111111111,1.),.UNSPECIFIED.)
GEOMETRIC_REPRESENTATION_ITEM()
RATIONAL_B_SPLINE_SURFACE(((1.,0.965925826289068,1.,0.965925826289068,1.,
0.965925826289068,1.,0.965925826289068,1.,0.965925826289068,1.,0.965925826289068,
1.,0.965925826289068,1.,0.965925826289068,1.,0.965925826289068,1.,0.965925826289068,
1.,0.965925826289068,1.,0.965925826289068,1.,0.965925826289068,1.,0.965925826289068,
1.,0.965925826289068,1.,0.965925826289068,1.,0.965925826289068,1.,0.965925826289068,
1.,0.965925826289068,1.,0.965925826289068,1.,0.965925826289068,1.,0.965925826289068,
1.,0.965925826289068,1.,0.965925826289068,1.,0.965925826289068,1.,0.965925826289068,
1.,0.965925826289068,1.,0.965925826289068,1.,0.965925826289068,1.,0.965925826289068,
1.,0.965925826289068,1.,0.965925826289068,1.,0.965925826289068,1.,0.965925826289068,
1.,0.965925826289068,1.,0.965925826289068,1.,0.965925826289068,1.,0.965925826289068,
1.,0.965925826289068,1.,0.965925826289068,1.,0.965925826289068,1.,0.965925826289068,
1.,0.965925826289068,1.,0.965925826289068,1.,0.965925826289068,1.,0.965925826289068,
1.,0.965925826289068,1.,0.965925826289068,1.,0.965925826289068,1.,0.965925826289068,
1.,0.965925826289068,1.,0.965925826289068,1.,0.965925826289068,1.,0.965925826289068,
1.,0.965925826289068,1.,0.965925826289068,1.,0.965925826289068,1.,0.965925826289068,
1.,0.965925826289068,1.,0.965925826289068,1.,0.965925826289068,1.,0.965925826289068,
1.,0.965925826289068,1.,0.965925826289068,1.,0.965925826289068,1.,0.965925826289068,
1.,0.965925826289068,1.,0.965925826289068,1.,0.965925826289068,1.,0.965925826289068,
1.,0.965925826289068,1.,0.965925826289068,1.),(1.,0.965925826289068,1.,
0.965925826289068,1.,0.965925826289068,1.,0.965925826289068,1.,0.965925826289068,
1.,0.965925826289068,1.,0.965925826289068,1.,0.965925826289068,1.,0.965925826289068,
1.,0.965925826289068,1.,0.965925826289068,1.,0.965925826289068,1.,0.965925826289068,
1.,0.965925826289068,1.,0.965925826289068,1.,0.965925826289068,1.,0.965925826289068,
1.,0.965925826289068,1.,0.965925826289068,1.,0.965925826289068,1.,0.965925826289068,
1.,0.965925826289068,1.,0.965925826289068,1.,0.965925826289068,1.,0.965925826289068,
1.,0.965925826289068,1.,0.965925826289068,1.,0.965925826289068,1.,0.965925826289068,
1.,0.965925826289068,1.,0.965925826289068,1.,0.965925826289068,1.,0.965925826289068,
1.,0.965925826289068,1.,0.965925826289068,1.,0.965925826289068,1.,0.965925826289068,
1.,0.965925826289068,1.,0.965925826289068,1.,0.965925826289068,1.,0.965925826289068,
1.,0.965925826289068,1.,0.965925826289068,1.,0.965925826289068,1.,0.965925826289068,
1.,0.965925826289068,1.,0.965925826289068,1.,0.965925826289068,1.,0.965925826289068,
1.,0.965925826289068,1.,0.965925826289068,1.,0.965925826289068,1.,0.965925826289068,
1.,0.965925826289068,1.,0.965925826289068,1.,0.965925826289068,1.,0.965925826289068,
1.,0.965925826289068,1.,0.965925826289068,1.,0.965925826289068,1.,0.965925826289068,
1.,0.965925826289068,1.,0.965925826289068,1.,0.965925826289068,1.,0.965925826289068,
1.,0.965925826289068,1.,0.965925826289068,1.,0.965925826289068,1.,0.965925826289068,
1.,0.965925826289068,1.,0.965925826289068,1.,0.965925826289068,1.)))
REPRESENTATION_ITEM('')
SURFACE()
);
#179=(
BOUNDED_SURFACE()
B_SPLINE_SURFACE(1,2,((#14185,#14186,#14187,#14188,#14189,#14190,#14191,
#14192,#14193,#14194,#14195,#14196,#14197,#14198,#14199,#14200,#14201,#14202,
#14203,#14204,#14205,#14206,#14207,#14208,#14209,#14210,#14211,#14212,#14213,
#14214,#14215,#14216,#14217,#14218,#14219,#14220,#14221,#14222,#14223,#14224,
#14225,#14226,#14227,#14228,#14229,#14230,#14231,#14232,#14233,#14234,#14235,
#14236,#14237,#14238,#14239,#14240,#14241,#14242,#14243,#14244,#14245,#14246,
#14247,#14248,#14249,#14250,#14251,#14252,#14253,#14254,#14255,#14256,#14257,
#14258,#14259,#14260,#14261,#14262,#14263,#14264,#14265,#14266,#14267,#14268,
#14269,#14270,#14271,#14272,#14273,#14274,#14275,#14276,#14277,#14278,#14279,
#14280,#14281,#14282,#14283,#14284,#14285,#14286,#14287,#14288,#14289,#14290,
#14291,#14292,#14293,#14294,#14295,#14296,#14297,#14298,#14299,#14300,#14301,
#14302,#14303,#14304,#14305,#14306,#14307,#14308,#14309,#14310,#14311,#14312,
#14313,#14314,#14315,#14316,#14317,#14318,#14319,#14320,#14321,#14322,#14323,
#14324,#14325,#14326,#14327,#14328,#14329),(#14330,#14331,#14332,#14333,
#14334,#14335,#14336,#14337,#14338,#14339,#14340,#14341,#14342,#14343,#14344,
#14345,#14346,#14347,#14348,#14349,#14350,#14351,#14352,#14353,#14354,#14355,
#14356,#14357,#14358,#14359,#14360,#14361,#14362,#14363,#14364,#14365,#14366,
#14367,#14368,#14369,#14370,#14371,#14372,#14373,#14374,#14375,#14376,#14377,
#14378,#14379,#14380,#14381,#14382,#14383,#14384,#14385,#14386,#14387,#14388,
#14389,#14390,#14391,#14392,#14393,#14394,#14395,#14396,#14397,#14398,#14399,
#14400,#14401,#14402,#14403,#14404,#14405,#14406,#14407,#14408,#14409,#14410,
#14411,#14412,#14413,#14414,#14415,#14416,#14417,#14418,#14419,#14420,#14421,
#14422,#14423,#14424,#14425,#14426,#14427,#14428,#14429,#14430,#14431,#14432,
#14433,#14434,#14435,#14436,#14437,#14438,#14439,#14440,#14441,#14442,#14443,
#14444,#14445,#14446,#14447,#14448,#14449,#14450,#14451,#14452,#14453,#14454,
#14455,#14456,#14457,#14458,#14459,#14460,#14461,#14462,#14463,#14464,#14465,
#14466,#14467,#14468,#14469,#14470,#14471,#14472,#14473,#14474)),
 .UNSPECIFIED.,.F.,.F.,.F.)
B_SPLINE_SURFACE_WITH_KNOTS((2,2),(3,2,2,2,2,2,2,2,2,2,2,2,2,2,2,2,2,2,
2,2,2,2,2,2,2,2,2,2,2,2,2,2,2,2,2,2,2,2,2,2,2,2,2,2,2,2,2,2,2,2,2,2,2,2,
2,2,2,2,2,2,2,2,2,2,2,2,2,2,2,2,2,2,3),(0.,1.),(0.,0.0138888888888889,0.0277777777777778,
0.0416666666666667,0.0555555555555556,0.0694444444444444,0.0833333333333333,
0.0972222222222222,0.111111111111111,0.125,0.138888888888889,0.152777777777778,
0.166666666666667,0.180555555555556,0.194444444444444,0.208333333333333,
0.222222222222222,0.236111111111111,0.25,0.263888888888889,0.277777777777778,
0.291666666666667,0.305555555555556,0.319444444444444,0.333333333333333,
0.347222222222222,0.361111111111111,0.375,0.388888888888889,0.402777777777778,
0.416666666666667,0.430555555555556,0.444444444444444,0.458333333333333,
0.472222222222222,0.486111111111111,0.5,0.513888888888889,0.527777777777778,
0.541666666666667,0.555555555555556,0.569444444444444,0.583333333333333,
0.597222222222222,0.611111111111111,0.625,0.638888888888889,0.652777777777778,
0.666666666666667,0.680555555555556,0.694444444444444,0.708333333333333,
0.722222222222222,0.736111111111111,0.75,0.763888888888889,0.777777777777778,
0.791666666666667,0.805555555555556,0.819444444444444,0.833333333333333,
0.847222222222222,0.861111111111111,0.875,0.888888888888889,0.902777777777778,
0.916666666666667,0.930555555555556,0.944444444444444,0.958333333333333,
0.972222222222222,0.986111111111111,1.),.UNSPECIFIED.)
GEOMETRIC_REPRESENTATION_ITEM()
RATIONAL_B_SPLINE_SURFACE(((1.,0.965925826289068,1.,0.965925826289068,1.,
0.965925826289068,1.,0.965925826289068,1.,0.965925826289068,1.,0.965925826289068,
1.,0.965925826289068,1.,0.965925826289068,1.,0.965925826289068,1.,0.965925826289068,
1.,0.965925826289068,1.,0.965925826289068,1.,0.965925826289068,1.,0.965925826289068,
1.,0.965925826289068,1.,0.965925826289068,1.,0.965925826289068,1.,0.965925826289068,
1.,0.965925826289068,1.,0.965925826289068,1.,0.965925826289068,1.,0.965925826289068,
1.,0.965925826289068,1.,0.965925826289068,1.,0.965925826289068,1.,0.965925826289068,
1.,0.965925826289068,1.,0.965925826289068,1.,0.965925826289068,1.,0.965925826289068,
1.,0.965925826289068,1.,0.965925826289068,1.,0.965925826289068,1.,0.965925826289068,
1.,0.965925826289068,1.,0.965925826289068,1.,0.965925826289068,1.,0.965925826289068,
1.,0.965925826289068,1.,0.965925826289068,1.,0.965925826289068,1.,0.965925826289068,
1.,0.965925826289068,1.,0.965925826289068,1.,0.965925826289068,1.,0.965925826289068,
1.,0.965925826289068,1.,0.965925826289068,1.,0.965925826289068,1.,0.965925826289068,
1.,0.965925826289068,1.,0.965925826289068,1.,0.965925826289068,1.,0.965925826289068,
1.,0.965925826289068,1.,0.965925826289068,1.,0.965925826289068,1.,0.965925826289068,
1.,0.965925826289068,1.,0.965925826289068,1.,0.965925826289068,1.,0.965925826289068,
1.,0.965925826289068,1.,0.965925826289068,1.,0.965925826289068,1.,0.965925826289068,
1.,0.965925826289068,1.,0.965925826289068,1.,0.965925826289068,1.,0.965925826289068,
1.,0.965925826289068,1.,0.965925826289068,1.),(1.,0.965925826289068,1.,
0.965925826289068,1.,0.965925826289068,1.,0.965925826289068,1.,0.965925826289068,
1.,0.965925826289068,1.,0.965925826289068,1.,0.965925826289068,1.,0.965925826289068,
1.,0.965925826289068,1.,0.965925826289068,1.,0.965925826289068,1.,0.965925826289068,
1.,0.965925826289068,1.,0.965925826289068,1.,0.965925826289068,1.,0.965925826289068,
1.,0.965925826289068,1.,0.965925826289068,1.,0.965925826289068,1.,0.965925826289068,
1.,0.965925826289068,1.,0.965925826289068,1.,0.965925826289068,1.,0.965925826289068,
1.,0.965925826289068,1.,0.965925826289068,1.,0.965925826289068,1.,0.965925826289068,
1.,0.965925826289068,1.,0.965925826289068,1.,0.965925826289068,1.,0.965925826289068,
1.,0.965925826289068,1.,0.965925826289068,1.,0.965925826289068,1.,0.965925826289068,
1.,0.965925826289068,1.,0.965925826289068,1.,0.965925826289068,1.,0.965925826289068,
1.,0.965925826289068,1.,0.965925826289068,1.,0.965925826289068,1.,0.965925826289068,
1.,0.965925826289068,1.,0.965925826289068,1.,0.965925826289068,1.,0.965925826289068,
1.,0.965925826289068,1.,0.965925826289068,1.,0.965925826289068,1.,0.965925826289068,
1.,0.965925826289068,1.,0.965925826289068,1.,0.965925826289068,1.,0.965925826289068,
1.,0.965925826289068,1.,0.965925826289068,1.,0.965925826289068,1.,0.965925826289068,
1.,0.965925826289068,1.,0.965925826289068,1.,0.965925826289068,1.,0.965925826289068,
1.,0.965925826289068,1.,0.965925826289068,1.,0.965925826289068,1.,0.965925826289068,
1.,0.965925826289068,1.,0.965925826289068,1.,0.965925826289068,1.)))
REPRESENTATION_ITEM('')
SURFACE()
);
#180=(
BOUNDED_SURFACE()
B_SPLINE_SURFACE(1,2,((#14483,#14484,#14485,#14486,#14487,#14488,#14489,
#14490,#14491,#14492,#14493,#14494,#14495,#14496,#14497,#14498,#14499,#14500,
#14501,#14502,#14503,#14504,#14505,#14506,#14507,#14508,#14509,#14510,#14511,
#14512,#14513,#14514,#14515,#14516,#14517,#14518,#14519,#14520,#14521,#14522,
#14523,#14524,#14525,#14526,#14527,#14528,#14529,#14530,#14531,#14532,#14533,
#14534,#14535,#14536,#14537,#14538,#14539,#14540,#14541,#14542,#14543,#14544,
#14545,#14546,#14547,#14548,#14549,#14550,#14551,#14552,#14553,#14554,#14555,
#14556,#14557,#14558,#14559,#14560,#14561,#14562,#14563,#14564,#14565,#14566,
#14567,#14568,#14569,#14570,#14571,#14572,#14573,#14574,#14575,#14576,#14577,
#14578,#14579,#14580,#14581,#14582,#14583,#14584,#14585,#14586,#14587,#14588,
#14589,#14590,#14591,#14592,#14593,#14594,#14595,#14596,#14597,#14598,#14599,
#14600,#14601,#14602,#14603,#14604,#14605,#14606,#14607,#14608,#14609,#14610,
#14611,#14612,#14613,#14614,#14615,#14616,#14617,#14618,#14619,#14620,#14621,
#14622,#14623,#14624,#14625,#14626,#14627),(#14628,#14629,#14630,#14631,
#14632,#14633,#14634,#14635,#14636,#14637,#14638,#14639,#14640,#14641,#14642,
#14643,#14644,#14645,#14646,#14647,#14648,#14649,#14650,#14651,#14652,#14653,
#14654,#14655,#14656,#14657,#14658,#14659,#14660,#14661,#14662,#14663,#14664,
#14665,#14666,#14667,#14668,#14669,#14670,#14671,#14672,#14673,#14674,#14675,
#14676,#14677,#14678,#14679,#14680,#14681,#14682,#14683,#14684,#14685,#14686,
#14687,#14688,#14689,#14690,#14691,#14692,#14693,#14694,#14695,#14696,#14697,
#14698,#14699,#14700,#14701,#14702,#14703,#14704,#14705,#14706,#14707,#14708,
#14709,#14710,#14711,#14712,#14713,#14714,#14715,#14716,#14717,#14718,#14719,
#14720,#14721,#14722,#14723,#14724,#14725,#14726,#14727,#14728,#14729,#14730,
#14731,#14732,#14733,#14734,#14735,#14736,#14737,#14738,#14739,#14740,#14741,
#14742,#14743,#14744,#14745,#14746,#14747,#14748,#14749,#14750,#14751,#14752,
#14753,#14754,#14755,#14756,#14757,#14758,#14759,#14760,#14761,#14762,#14763,
#14764,#14765,#14766,#14767,#14768,#14769,#14770,#14771,#14772)),
 .UNSPECIFIED.,.F.,.F.,.F.)
B_SPLINE_SURFACE_WITH_KNOTS((2,2),(3,2,2,2,2,2,2,2,2,2,2,2,2,2,2,2,2,2,
2,2,2,2,2,2,2,2,2,2,2,2,2,2,2,2,2,2,2,2,2,2,2,2,2,2,2,2,2,2,2,2,2,2,2,2,
2,2,2,2,2,2,2,2,2,2,2,2,2,2,2,2,2,2,3),(0.,1.),(0.,0.0138888888888889,0.0277777777777778,
0.0416666666666667,0.0555555555555556,0.0694444444444444,0.0833333333333333,
0.0972222222222222,0.111111111111111,0.125,0.138888888888889,0.152777777777778,
0.166666666666667,0.180555555555556,0.194444444444444,0.208333333333333,
0.222222222222222,0.236111111111111,0.25,0.263888888888889,0.277777777777778,
0.291666666666667,0.305555555555556,0.319444444444444,0.333333333333333,
0.347222222222222,0.361111111111111,0.375,0.388888888888889,0.402777777777778,
0.416666666666667,0.430555555555556,0.444444444444444,0.458333333333333,
0.472222222222222,0.486111111111111,0.5,0.513888888888889,0.527777777777778,
0.541666666666667,0.555555555555556,0.569444444444444,0.583333333333333,
0.597222222222222,0.611111111111111,0.625,0.638888888888889,0.652777777777778,
0.666666666666667,0.680555555555556,0.694444444444444,0.708333333333333,
0.722222222222222,0.736111111111111,0.75,0.763888888888889,0.777777777777778,
0.791666666666667,0.805555555555556,0.819444444444444,0.833333333333333,
0.847222222222222,0.861111111111111,0.875,0.888888888888889,0.902777777777778,
0.916666666666667,0.930555555555556,0.944444444444444,0.958333333333333,
0.972222222222222,0.986111111111111,1.),.UNSPECIFIED.)
GEOMETRIC_REPRESENTATION_ITEM()
RATIONAL_B_SPLINE_SURFACE(((1.,0.965925826289068,1.,0.965925826289068,1.,
0.965925826289068,1.,0.965925826289068,1.,0.965925826289068,1.,0.965925826289068,
1.,0.965925826289068,1.,0.965925826289068,1.,0.965925826289068,1.,0.965925826289068,
1.,0.965925826289068,1.,0.965925826289068,1.,0.965925826289068,1.,0.965925826289068,
1.,0.965925826289068,1.,0.965925826289068,1.,0.965925826289068,1.,0.965925826289068,
1.,0.965925826289068,1.,0.965925826289068,1.,0.965925826289068,1.,0.965925826289068,
1.,0.965925826289068,1.,0.965925826289068,1.,0.965925826289068,1.,0.965925826289068,
1.,0.965925826289068,1.,0.965925826289068,1.,0.965925826289068,1.,0.965925826289068,
1.,0.965925826289068,1.,0.965925826289068,1.,0.965925826289068,1.,0.965925826289068,
1.,0.965925826289068,1.,0.965925826289068,1.,0.965925826289068,1.,0.965925826289068,
1.,0.965925826289068,1.,0.965925826289068,1.,0.965925826289068,1.,0.965925826289068,
1.,0.965925826289068,1.,0.965925826289068,1.,0.965925826289068,1.,0.965925826289068,
1.,0.965925826289068,1.,0.965925826289068,1.,0.965925826289068,1.,0.965925826289068,
1.,0.965925826289068,1.,0.965925826289068,1.,0.965925826289068,1.,0.965925826289068,
1.,0.965925826289068,1.,0.965925826289068,1.,0.965925826289068,1.,0.965925826289068,
1.,0.965925826289068,1.,0.965925826289068,1.,0.965925826289068,1.,0.965925826289068,
1.,0.965925826289068,1.,0.965925826289068,1.,0.965925826289068,1.,0.965925826289068,
1.,0.965925826289068,1.,0.965925826289068,1.,0.965925826289068,1.,0.965925826289068,
1.,0.965925826289068,1.,0.965925826289068,1.),(1.,0.965925826289068,1.,
0.965925826289068,1.,0.965925826289068,1.,0.965925826289068,1.,0.965925826289068,
1.,0.965925826289068,1.,0.965925826289068,1.,0.965925826289068,1.,0.965925826289068,
1.,0.965925826289068,1.,0.965925826289068,1.,0.965925826289068,1.,0.965925826289068,
1.,0.965925826289068,1.,0.965925826289068,1.,0.965925826289068,1.,0.965925826289068,
1.,0.965925826289068,1.,0.965925826289068,1.,0.965925826289068,1.,0.965925826289068,
1.,0.965925826289068,1.,0.965925826289068,1.,0.965925826289068,1.,0.965925826289068,
1.,0.965925826289068,1.,0.965925826289068,1.,0.965925826289068,1.,0.965925826289068,
1.,0.965925826289068,1.,0.965925826289068,1.,0.965925826289068,1.,0.965925826289068,
1.,0.965925826289068,1.,0.965925826289068,1.,0.965925826289068,1.,0.965925826289068,
1.,0.965925826289068,1.,0.965925826289068,1.,0.965925826289068,1.,0.965925826289068,
1.,0.965925826289068,1.,0.965925826289068,1.,0.965925826289068,1.,0.965925826289068,
1.,0.965925826289068,1.,0.965925826289068,1.,0.965925826289068,1.,0.965925826289068,
1.,0.965925826289068,1.,0.965925826289068,1.,0.965925826289068,1.,0.965925826289068,
1.,0.965925826289068,1.,0.965925826289068,1.,0.965925826289068,1.,0.965925826289068,
1.,0.965925826289068,1.,0.965925826289068,1.,0.965925826289068,1.,0.965925826289068,
1.,0.965925826289068,1.,0.965925826289068,1.,0.965925826289068,1.,0.965925826289068,
1.,0.965925826289068,1.,0.965925826289068,1.,0.965925826289068,1.,0.965925826289068,
1.,0.965925826289068,1.,0.965925826289068,1.,0.965925826289068,1.)))
REPRESENTATION_ITEM('')
SURFACE()
);
#181=(
BOUNDED_SURFACE()
B_SPLINE_SURFACE(1,2,((#14781,#14782,#14783,#14784,#14785,#14786,#14787,
#14788,#14789,#14790,#14791,#14792,#14793,#14794,#14795,#14796,#14797,#14798,
#14799,#14800,#14801,#14802,#14803,#14804,#14805,#14806,#14807,#14808,#14809,
#14810,#14811,#14812,#14813,#14814,#14815,#14816,#14817,#14818,#14819,#14820,
#14821,#14822,#14823,#14824,#14825,#14826,#14827,#14828,#14829,#14830,#14831,
#14832,#14833,#14834,#14835,#14836,#14837,#14838,#14839,#14840,#14841,#14842,
#14843,#14844,#14845,#14846,#14847,#14848,#14849,#14850,#14851,#14852,#14853,
#14854,#14855,#14856,#14857,#14858,#14859,#14860,#14861,#14862,#14863,#14864,
#14865,#14866,#14867,#14868,#14869,#14870,#14871,#14872,#14873,#14874,#14875,
#14876,#14877,#14878,#14879,#14880,#14881,#14882,#14883,#14884,#14885,#14886,
#14887,#14888,#14889,#14890,#14891,#14892,#14893,#14894,#14895,#14896,#14897,
#14898,#14899,#14900,#14901,#14902,#14903,#14904,#14905,#14906,#14907,#14908,
#14909,#14910,#14911,#14912,#14913,#14914,#14915,#14916,#14917,#14918,#14919,
#14920,#14921,#14922,#14923,#14924,#14925),(#14926,#14927,#14928,#14929,
#14930,#14931,#14932,#14933,#14934,#14935,#14936,#14937,#14938,#14939,#14940,
#14941,#14942,#14943,#14944,#14945,#14946,#14947,#14948,#14949,#14950,#14951,
#14952,#14953,#14954,#14955,#14956,#14957,#14958,#14959,#14960,#14961,#14962,
#14963,#14964,#14965,#14966,#14967,#14968,#14969,#14970,#14971,#14972,#14973,
#14974,#14975,#14976,#14977,#14978,#14979,#14980,#14981,#14982,#14983,#14984,
#14985,#14986,#14987,#14988,#14989,#14990,#14991,#14992,#14993,#14994,#14995,
#14996,#14997,#14998,#14999,#15000,#15001,#15002,#15003,#15004,#15005,#15006,
#15007,#15008,#15009,#15010,#15011,#15012,#15013,#15014,#15015,#15016,#15017,
#15018,#15019,#15020,#15021,#15022,#15023,#15024,#15025,#15026,#15027,#15028,
#15029,#15030,#15031,#15032,#15033,#15034,#15035,#15036,#15037,#15038,#15039,
#15040,#15041,#15042,#15043,#15044,#15045,#15046,#15047,#15048,#15049,#15050,
#15051,#15052,#15053,#15054,#15055,#15056,#15057,#15058,#15059,#15060,#15061,
#15062,#15063,#15064,#15065,#15066,#15067,#15068,#15069,#15070)),
 .UNSPECIFIED.,.F.,.F.,.F.)
B_SPLINE_SURFACE_WITH_KNOTS((2,2),(3,2,2,2,2,2,2,2,2,2,2,2,2,2,2,2,2,2,
2,2,2,2,2,2,2,2,2,2,2,2,2,2,2,2,2,2,2,2,2,2,2,2,2,2,2,2,2,2,2,2,2,2,2,2,
2,2,2,2,2,2,2,2,2,2,2,2,2,2,2,2,2,2,3),(0.,1.),(0.,0.0138888888888889,0.0277777777777778,
0.0416666666666667,0.0555555555555556,0.0694444444444444,0.0833333333333333,
0.0972222222222222,0.111111111111111,0.125,0.138888888888889,0.152777777777778,
0.166666666666667,0.180555555555556,0.194444444444444,0.208333333333333,
0.222222222222222,0.236111111111111,0.25,0.263888888888889,0.277777777777778,
0.291666666666667,0.305555555555556,0.319444444444444,0.333333333333333,
0.347222222222222,0.361111111111111,0.375,0.388888888888889,0.402777777777778,
0.416666666666667,0.430555555555556,0.444444444444444,0.458333333333333,
0.472222222222222,0.486111111111111,0.5,0.513888888888889,0.527777777777778,
0.541666666666667,0.555555555555556,0.569444444444444,0.583333333333333,
0.597222222222222,0.611111111111111,0.625,0.638888888888889,0.652777777777778,
0.666666666666667,0.680555555555556,0.694444444444444,0.708333333333333,
0.722222222222222,0.736111111111111,0.75,0.763888888888889,0.777777777777778,
0.791666666666667,0.805555555555556,0.819444444444444,0.833333333333333,
0.847222222222222,0.861111111111111,0.875,0.888888888888889,0.902777777777778,
0.916666666666667,0.930555555555556,0.944444444444444,0.958333333333333,
0.972222222222222,0.986111111111111,1.),.UNSPECIFIED.)
GEOMETRIC_REPRESENTATION_ITEM()
RATIONAL_B_SPLINE_SURFACE(((1.,0.965925826289068,1.,0.965925826289068,1.,
0.965925826289068,1.,0.965925826289068,1.,0.965925826289068,1.,0.965925826289068,
1.,0.965925826289068,1.,0.965925826289068,1.,0.965925826289068,1.,0.965925826289068,
1.,0.965925826289068,1.,0.965925826289068,1.,0.965925826289068,1.,0.965925826289068,
1.,0.965925826289068,1.,0.965925826289068,1.,0.965925826289068,1.,0.965925826289068,
1.,0.965925826289068,1.,0.965925826289068,1.,0.965925826289068,1.,0.965925826289068,
1.,0.965925826289068,1.,0.965925826289068,1.,0.965925826289068,1.,0.965925826289068,
1.,0.965925826289068,1.,0.965925826289068,1.,0.965925826289068,1.,0.965925826289068,
1.,0.965925826289068,1.,0.965925826289068,1.,0.965925826289068,1.,0.965925826289068,
1.,0.965925826289068,1.,0.965925826289068,1.,0.965925826289068,1.,0.965925826289068,
1.,0.965925826289068,1.,0.965925826289068,1.,0.965925826289068,1.,0.965925826289068,
1.,0.965925826289068,1.,0.965925826289068,1.,0.965925826289068,1.,0.965925826289068,
1.,0.965925826289068,1.,0.965925826289068,1.,0.965925826289068,1.,0.965925826289068,
1.,0.965925826289068,1.,0.965925826289068,1.,0.965925826289068,1.,0.965925826289068,
1.,0.965925826289068,1.,0.965925826289068,1.,0.965925826289068,1.,0.965925826289068,
1.,0.965925826289068,1.,0.965925826289068,1.,0.965925826289068,1.,0.965925826289068,
1.,0.965925826289068,1.,0.965925826289068,1.,0.965925826289068,1.,0.965925826289068,
1.,0.965925826289068,1.,0.965925826289068,1.,0.965925826289068,1.,0.965925826289068,
1.,0.965925826289068,1.,0.965925826289068,1.),(1.,0.965925826289068,1.,
0.965925826289068,1.,0.965925826289068,1.,0.965925826289068,1.,0.965925826289068,
1.,0.965925826289068,1.,0.965925826289068,1.,0.965925826289068,1.,0.965925826289068,
1.,0.965925826289068,1.,0.965925826289068,1.,0.965925826289068,1.,0.965925826289068,
1.,0.965925826289068,1.,0.965925826289068,1.,0.965925826289068,1.,0.965925826289068,
1.,0.965925826289068,1.,0.965925826289068,1.,0.965925826289068,1.,0.965925826289068,
1.,0.965925826289068,1.,0.965925826289068,1.,0.965925826289068,1.,0.965925826289068,
1.,0.965925826289068,1.,0.965925826289068,1.,0.965925826289068,1.,0.965925826289068,
1.,0.965925826289068,1.,0.965925826289068,1.,0.965925826289068,1.,0.965925826289068,
1.,0.965925826289068,1.,0.965925826289068,1.,0.965925826289068,1.,0.965925826289068,
1.,0.965925826289068,1.,0.965925826289068,1.,0.965925826289068,1.,0.965925826289068,
1.,0.965925826289068,1.,0.965925826289068,1.,0.965925826289068,1.,0.965925826289068,
1.,0.965925826289068,1.,0.965925826289068,1.,0.965925826289068,1.,0.965925826289068,
1.,0.965925826289068,1.,0.965925826289068,1.,0.965925826289068,1.,0.965925826289068,
1.,0.965925826289068,1.,0.965925826289068,1.,0.965925826289068,1.,0.965925826289068,
1.,0.965925826289068,1.,0.965925826289068,1.,0.965925826289068,1.,0.965925826289068,
1.,0.965925826289068,1.,0.965925826289068,1.,0.965925826289068,1.,0.965925826289068,
1.,0.965925826289068,1.,0.965925826289068,1.,0.965925826289068,1.,0.965925826289068,
1.,0.965925826289068,1.,0.965925826289068,1.,0.965925826289068,1.)))
REPRESENTATION_ITEM('')
SURFACE()
);
#182=(
BOUNDED_SURFACE()
B_SPLINE_SURFACE(1,2,((#15079,#15080,#15081,#15082,#15083,#15084,#15085,
#15086,#15087,#15088,#15089,#15090,#15091,#15092,#15093,#15094,#15095,#15096,
#15097,#15098,#15099,#15100,#15101,#15102,#15103,#15104,#15105,#15106,#15107,
#15108,#15109,#15110,#15111,#15112,#15113,#15114,#15115,#15116,#15117,#15118,
#15119,#15120,#15121,#15122,#15123,#15124,#15125,#15126,#15127,#15128,#15129,
#15130,#15131,#15132,#15133,#15134,#15135,#15136,#15137,#15138,#15139,#15140,
#15141,#15142,#15143,#15144,#15145,#15146,#15147,#15148,#15149,#15150,#15151,
#15152,#15153,#15154,#15155,#15156,#15157,#15158,#15159,#15160,#15161,#15162,
#15163,#15164,#15165,#15166,#15167,#15168,#15169,#15170,#15171,#15172,#15173,
#15174,#15175,#15176,#15177,#15178,#15179,#15180,#15181,#15182,#15183,#15184,
#15185,#15186,#15187,#15188,#15189,#15190,#15191,#15192,#15193,#15194,#15195,
#15196,#15197,#15198,#15199,#15200,#15201,#15202,#15203,#15204,#15205,#15206,
#15207,#15208,#15209,#15210,#15211,#15212,#15213,#15214,#15215,#15216,#15217,
#15218,#15219,#15220,#15221,#15222,#15223),(#15224,#15225,#15226,#15227,
#15228,#15229,#15230,#15231,#15232,#15233,#15234,#15235,#15236,#15237,#15238,
#15239,#15240,#15241,#15242,#15243,#15244,#15245,#15246,#15247,#15248,#15249,
#15250,#15251,#15252,#15253,#15254,#15255,#15256,#15257,#15258,#15259,#15260,
#15261,#15262,#15263,#15264,#15265,#15266,#15267,#15268,#15269,#15270,#15271,
#15272,#15273,#15274,#15275,#15276,#15277,#15278,#15279,#15280,#15281,#15282,
#15283,#15284,#15285,#15286,#15287,#15288,#15289,#15290,#15291,#15292,#15293,
#15294,#15295,#15296,#15297,#15298,#15299,#15300,#15301,#15302,#15303,#15304,
#15305,#15306,#15307,#15308,#15309,#15310,#15311,#15312,#15313,#15314,#15315,
#15316,#15317,#15318,#15319,#15320,#15321,#15322,#15323,#15324,#15325,#15326,
#15327,#15328,#15329,#15330,#15331,#15332,#15333,#15334,#15335,#15336,#15337,
#15338,#15339,#15340,#15341,#15342,#15343,#15344,#15345,#15346,#15347,#15348,
#15349,#15350,#15351,#15352,#15353,#15354,#15355,#15356,#15357,#15358,#15359,
#15360,#15361,#15362,#15363,#15364,#15365,#15366,#15367,#15368)),
 .UNSPECIFIED.,.F.,.F.,.F.)
B_SPLINE_SURFACE_WITH_KNOTS((2,2),(3,2,2,2,2,2,2,2,2,2,2,2,2,2,2,2,2,2,
2,2,2,2,2,2,2,2,2,2,2,2,2,2,2,2,2,2,2,2,2,2,2,2,2,2,2,2,2,2,2,2,2,2,2,2,
2,2,2,2,2,2,2,2,2,2,2,2,2,2,2,2,2,2,3),(0.,1.),(0.,0.0138888888888889,0.0277777777777778,
0.0416666666666667,0.0555555555555556,0.0694444444444444,0.0833333333333333,
0.0972222222222222,0.111111111111111,0.125,0.138888888888889,0.152777777777778,
0.166666666666667,0.180555555555556,0.194444444444444,0.208333333333333,
0.222222222222222,0.236111111111111,0.25,0.263888888888889,0.277777777777778,
0.291666666666667,0.305555555555556,0.319444444444444,0.333333333333333,
0.347222222222222,0.361111111111111,0.375,0.388888888888889,0.402777777777778,
0.416666666666667,0.430555555555556,0.444444444444444,0.458333333333333,
0.472222222222222,0.486111111111111,0.5,0.513888888888889,0.527777777777778,
0.541666666666667,0.555555555555556,0.569444444444444,0.583333333333333,
0.597222222222222,0.611111111111111,0.625,0.638888888888889,0.652777777777778,
0.666666666666667,0.680555555555556,0.694444444444444,0.708333333333333,
0.722222222222222,0.736111111111111,0.75,0.763888888888889,0.777777777777778,
0.791666666666667,0.805555555555556,0.819444444444444,0.833333333333333,
0.847222222222222,0.861111111111111,0.875,0.888888888888889,0.902777777777778,
0.916666666666667,0.930555555555556,0.944444444444444,0.958333333333333,
0.972222222222222,0.986111111111111,1.),.UNSPECIFIED.)
GEOMETRIC_REPRESENTATION_ITEM()
RATIONAL_B_SPLINE_SURFACE(((1.,0.965925826289068,1.,0.965925826289068,1.,
0.965925826289068,1.,0.965925826289068,1.,0.965925826289068,1.,0.965925826289068,
1.,0.965925826289068,1.,0.965925826289068,1.,0.965925826289068,1.,0.965925826289068,
1.,0.965925826289068,1.,0.965925826289068,1.,0.965925826289068,1.,0.965925826289068,
1.,0.965925826289068,1.,0.965925826289068,1.,0.965925826289068,1.,0.965925826289068,
1.,0.965925826289068,1.,0.965925826289068,1.,0.965925826289068,1.,0.965925826289068,
1.,0.965925826289068,1.,0.965925826289068,1.,0.965925826289068,1.,0.965925826289068,
1.,0.965925826289068,1.,0.965925826289068,1.,0.965925826289068,1.,0.965925826289068,
1.,0.965925826289068,1.,0.965925826289068,1.,0.965925826289068,1.,0.965925826289068,
1.,0.965925826289068,1.,0.965925826289068,1.,0.965925826289068,1.,0.965925826289068,
1.,0.965925826289068,1.,0.965925826289068,1.,0.965925826289068,1.,0.965925826289068,
1.,0.965925826289068,1.,0.965925826289068,1.,0.965925826289068,1.,0.965925826289068,
1.,0.965925826289068,1.,0.965925826289068,1.,0.965925826289068,1.,0.965925826289068,
1.,0.965925826289068,1.,0.965925826289068,1.,0.965925826289068,1.,0.965925826289068,
1.,0.965925826289068,1.,0.965925826289068,1.,0.965925826289068,1.,0.965925826289068,
1.,0.965925826289068,1.,0.965925826289068,1.,0.965925826289068,1.,0.965925826289068,
1.,0.965925826289068,1.,0.965925826289068,1.,0.965925826289068,1.,0.965925826289068,
1.,0.965925826289068,1.,0.965925826289068,1.,0.965925826289068,1.,0.965925826289068,
1.,0.965925826289068,1.,0.965925826289068,1.),(1.,0.965925826289068,1.,
0.965925826289068,1.,0.965925826289068,1.,0.965925826289068,1.,0.965925826289068,
1.,0.965925826289068,1.,0.965925826289068,1.,0.965925826289068,1.,0.965925826289068,
1.,0.965925826289068,1.,0.965925826289068,1.,0.965925826289068,1.,0.965925826289068,
1.,0.965925826289068,1.,0.965925826289068,1.,0.965925826289068,1.,0.965925826289068,
1.,0.965925826289068,1.,0.965925826289068,1.,0.965925826289068,1.,0.965925826289068,
1.,0.965925826289068,1.,0.965925826289068,1.,0.965925826289068,1.,0.965925826289068,
1.,0.965925826289068,1.,0.965925826289068,1.,0.965925826289068,1.,0.965925826289068,
1.,0.965925826289068,1.,0.965925826289068,1.,0.965925826289068,1.,0.965925826289068,
1.,0.965925826289068,1.,0.965925826289068,1.,0.965925826289068,1.,0.965925826289068,
1.,0.965925826289068,1.,0.965925826289068,1.,0.965925826289068,1.,0.965925826289068,
1.,0.965925826289068,1.,0.965925826289068,1.,0.965925826289068,1.,0.965925826289068,
1.,0.965925826289068,1.,0.965925826289068,1.,0.965925826289068,1.,0.965925826289068,
1.,0.965925826289068,1.,0.965925826289068,1.,0.965925826289068,1.,0.965925826289068,
1.,0.965925826289068,1.,0.965925826289068,1.,0.965925826289068,1.,0.965925826289068,
1.,0.965925826289068,1.,0.965925826289068,1.,0.965925826289068,1.,0.965925826289068,
1.,0.965925826289068,1.,0.965925826289068,1.,0.965925826289068,1.,0.965925826289068,
1.,0.965925826289068,1.,0.965925826289068,1.,0.965925826289068,1.,0.965925826289068,
1.,0.965925826289068,1.,0.965925826289068,1.,0.965925826289068,1.)))
REPRESENTATION_ITEM('')
SURFACE()
);
#183=(
BOUNDED_SURFACE()
B_SPLINE_SURFACE(1,2,((#15377,#15378,#15379,#15380,#15381,#15382,#15383,
#15384,#15385,#15386,#15387,#15388,#15389,#15390,#15391,#15392,#15393,#15394,
#15395,#15396,#15397,#15398,#15399,#15400,#15401,#15402,#15403,#15404,#15405,
#15406,#15407,#15408,#15409,#15410,#15411,#15412,#15413,#15414,#15415,#15416,
#15417,#15418,#15419,#15420,#15421,#15422,#15423,#15424,#15425,#15426,#15427,
#15428,#15429,#15430,#15431,#15432,#15433,#15434,#15435,#15436,#15437,#15438,
#15439,#15440,#15441,#15442,#15443,#15444,#15445,#15446,#15447,#15448,#15449,
#15450,#15451,#15452,#15453,#15454,#15455,#15456,#15457,#15458,#15459,#15460,
#15461,#15462,#15463,#15464,#15465,#15466,#15467,#15468,#15469,#15470,#15471,
#15472,#15473,#15474,#15475,#15476,#15477,#15478,#15479,#15480,#15481,#15482,
#15483,#15484,#15485,#15486,#15487,#15488,#15489,#15490,#15491,#15492,#15493,
#15494,#15495,#15496,#15497,#15498,#15499,#15500,#15501,#15502,#15503,#15504,
#15505,#15506,#15507,#15508,#15509,#15510,#15511,#15512,#15513,#15514,#15515,
#15516,#15517,#15518,#15519,#15520,#15521),(#15522,#15523,#15524,#15525,
#15526,#15527,#15528,#15529,#15530,#15531,#15532,#15533,#15534,#15535,#15536,
#15537,#15538,#15539,#15540,#15541,#15542,#15543,#15544,#15545,#15546,#15547,
#15548,#15549,#15550,#15551,#15552,#15553,#15554,#15555,#15556,#15557,#15558,
#15559,#15560,#15561,#15562,#15563,#15564,#15565,#15566,#15567,#15568,#15569,
#15570,#15571,#15572,#15573,#15574,#15575,#15576,#15577,#15578,#15579,#15580,
#15581,#15582,#15583,#15584,#15585,#15586,#15587,#15588,#15589,#15590,#15591,
#15592,#15593,#15594,#15595,#15596,#15597,#15598,#15599,#15600,#15601,#15602,
#15603,#15604,#15605,#15606,#15607,#15608,#15609,#15610,#15611,#15612,#15613,
#15614,#15615,#15616,#15617,#15618,#15619,#15620,#15621,#15622,#15623,#15624,
#15625,#15626,#15627,#15628,#15629,#15630,#15631,#15632,#15633,#15634,#15635,
#15636,#15637,#15638,#15639,#15640,#15641,#15642,#15643,#15644,#15645,#15646,
#15647,#15648,#15649,#15650,#15651,#15652,#15653,#15654,#15655,#15656,#15657,
#15658,#15659,#15660,#15661,#15662,#15663,#15664,#15665,#15666)),
 .UNSPECIFIED.,.F.,.F.,.F.)
B_SPLINE_SURFACE_WITH_KNOTS((2,2),(3,2,2,2,2,2,2,2,2,2,2,2,2,2,2,2,2,2,
2,2,2,2,2,2,2,2,2,2,2,2,2,2,2,2,2,2,2,2,2,2,2,2,2,2,2,2,2,2,2,2,2,2,2,2,
2,2,2,2,2,2,2,2,2,2,2,2,2,2,2,2,2,2,3),(0.,1.),(0.,0.0138888888888889,0.0277777777777778,
0.0416666666666667,0.0555555555555556,0.0694444444444444,0.0833333333333333,
0.0972222222222222,0.111111111111111,0.125,0.138888888888889,0.152777777777778,
0.166666666666667,0.180555555555556,0.194444444444444,0.208333333333333,
0.222222222222222,0.236111111111111,0.25,0.263888888888889,0.277777777777778,
0.291666666666667,0.305555555555556,0.319444444444444,0.333333333333333,
0.347222222222222,0.361111111111111,0.375,0.388888888888889,0.402777777777778,
0.416666666666667,0.430555555555556,0.444444444444444,0.458333333333333,
0.472222222222222,0.486111111111111,0.5,0.513888888888889,0.527777777777778,
0.541666666666667,0.555555555555556,0.569444444444444,0.583333333333333,
0.597222222222222,0.611111111111111,0.625,0.638888888888889,0.652777777777778,
0.666666666666667,0.680555555555556,0.694444444444444,0.708333333333333,
0.722222222222222,0.736111111111111,0.75,0.763888888888889,0.777777777777778,
0.791666666666667,0.805555555555556,0.819444444444444,0.833333333333333,
0.847222222222222,0.861111111111111,0.875,0.888888888888889,0.902777777777778,
0.916666666666667,0.930555555555556,0.944444444444444,0.958333333333333,
0.972222222222222,0.986111111111111,1.),.UNSPECIFIED.)
GEOMETRIC_REPRESENTATION_ITEM()
RATIONAL_B_SPLINE_SURFACE(((1.,0.965925826289068,1.,0.965925826289068,1.,
0.965925826289068,1.,0.965925826289068,1.,0.965925826289068,1.,0.965925826289068,
1.,0.965925826289068,1.,0.965925826289068,1.,0.965925826289068,1.,0.965925826289068,
1.,0.965925826289068,1.,0.965925826289068,1.,0.965925826289068,1.,0.965925826289068,
1.,0.965925826289068,1.,0.965925826289068,1.,0.965925826289068,1.,0.965925826289068,
1.,0.965925826289068,1.,0.965925826289068,1.,0.965925826289068,1.,0.965925826289068,
1.,0.965925826289068,1.,0.965925826289068,1.,0.965925826289068,1.,0.965925826289068,
1.,0.965925826289068,1.,0.965925826289068,1.,0.965925826289068,1.,0.965925826289068,
1.,0.965925826289068,1.,0.965925826289068,1.,0.965925826289068,1.,0.965925826289068,
1.,0.965925826289068,1.,0.965925826289068,1.,0.965925826289068,1.,0.965925826289068,
1.,0.965925826289068,1.,0.965925826289068,1.,0.965925826289068,1.,0.965925826289068,
1.,0.965925826289068,1.,0.965925826289068,1.,0.965925826289068,1.,0.965925826289068,
1.,0.965925826289068,1.,0.965925826289068,1.,0.965925826289068,1.,0.965925826289068,
1.,0.965925826289068,1.,0.965925826289068,1.,0.965925826289068,1.,0.965925826289068,
1.,0.965925826289068,1.,0.965925826289068,1.,0.965925826289068,1.,0.965925826289068,
1.,0.965925826289068,1.,0.965925826289068,1.,0.965925826289068,1.,0.965925826289068,
1.,0.965925826289068,1.,0.965925826289068,1.,0.965925826289068,1.,0.965925826289068,
1.,0.965925826289068,1.,0.965925826289068,1.,0.965925826289068,1.,0.965925826289068,
1.,0.965925826289068,1.,0.965925826289068,1.),(1.,0.965925826289068,1.,
0.965925826289068,1.,0.965925826289068,1.,0.965925826289068,1.,0.965925826289068,
1.,0.965925826289068,1.,0.965925826289068,1.,0.965925826289068,1.,0.965925826289068,
1.,0.965925826289068,1.,0.965925826289068,1.,0.965925826289068,1.,0.965925826289068,
1.,0.965925826289068,1.,0.965925826289068,1.,0.965925826289068,1.,0.965925826289068,
1.,0.965925826289068,1.,0.965925826289068,1.,0.965925826289068,1.,0.965925826289068,
1.,0.965925826289068,1.,0.965925826289068,1.,0.965925826289068,1.,0.965925826289068,
1.,0.965925826289068,1.,0.965925826289068,1.,0.965925826289068,1.,0.965925826289068,
1.,0.965925826289068,1.,0.965925826289068,1.,0.965925826289068,1.,0.965925826289068,
1.,0.965925826289068,1.,0.965925826289068,1.,0.965925826289068,1.,0.965925826289068,
1.,0.965925826289068,1.,0.965925826289068,1.,0.965925826289068,1.,0.965925826289068,
1.,0.965925826289068,1.,0.965925826289068,1.,0.965925826289068,1.,0.965925826289068,
1.,0.965925826289068,1.,0.965925826289068,1.,0.965925826289068,1.,0.965925826289068,
1.,0.965925826289068,1.,0.965925826289068,1.,0.965925826289068,1.,0.965925826289068,
1.,0.965925826289068,1.,0.965925826289068,1.,0.965925826289068,1.,0.965925826289068,
1.,0.965925826289068,1.,0.965925826289068,1.,0.965925826289068,1.,0.965925826289068,
1.,0.965925826289068,1.,0.965925826289068,1.,0.965925826289068,1.,0.965925826289068,
1.,0.965925826289068,1.,0.965925826289068,1.,0.965925826289068,1.,0.965925826289068,
1.,0.965925826289068,1.,0.965925826289068,1.,0.965925826289068,1.)))
REPRESENTATION_ITEM('')
SURFACE()
);
#184=(
BOUNDED_SURFACE()
B_SPLINE_SURFACE(1,2,((#15675,#15676,#15677,#15678,#15679,#15680,#15681,
#15682,#15683,#15684,#15685,#15686,#15687,#15688,#15689,#15690,#15691,#15692,
#15693,#15694,#15695,#15696,#15697,#15698,#15699,#15700,#15701,#15702,#15703,
#15704,#15705,#15706,#15707,#15708,#15709,#15710,#15711,#15712,#15713,#15714,
#15715,#15716,#15717,#15718,#15719,#15720,#15721,#15722,#15723,#15724,#15725,
#15726,#15727,#15728,#15729,#15730,#15731,#15732,#15733,#15734,#15735,#15736,
#15737,#15738,#15739,#15740,#15741,#15742,#15743,#15744,#15745,#15746,#15747,
#15748,#15749,#15750,#15751,#15752,#15753,#15754,#15755,#15756,#15757,#15758,
#15759,#15760,#15761,#15762,#15763,#15764,#15765,#15766,#15767,#15768,#15769,
#15770,#15771,#15772,#15773,#15774,#15775,#15776,#15777,#15778,#15779,#15780,
#15781,#15782,#15783,#15784,#15785,#15786,#15787,#15788,#15789,#15790,#15791,
#15792,#15793,#15794,#15795,#15796,#15797,#15798,#15799,#15800,#15801,#15802,
#15803,#15804,#15805,#15806,#15807,#15808,#15809,#15810,#15811,#15812,#15813,
#15814,#15815,#15816,#15817,#15818,#15819),(#15820,#15821,#15822,#15823,
#15824,#15825,#15826,#15827,#15828,#15829,#15830,#15831,#15832,#15833,#15834,
#15835,#15836,#15837,#15838,#15839,#15840,#15841,#15842,#15843,#15844,#15845,
#15846,#15847,#15848,#15849,#15850,#15851,#15852,#15853,#15854,#15855,#15856,
#15857,#15858,#15859,#15860,#15861,#15862,#15863,#15864,#15865,#15866,#15867,
#15868,#15869,#15870,#15871,#15872,#15873,#15874,#15875,#15876,#15877,#15878,
#15879,#15880,#15881,#15882,#15883,#15884,#15885,#15886,#15887,#15888,#15889,
#15890,#15891,#15892,#15893,#15894,#15895,#15896,#15897,#15898,#15899,#15900,
#15901,#15902,#15903,#15904,#15905,#15906,#15907,#15908,#15909,#15910,#15911,
#15912,#15913,#15914,#15915,#15916,#15917,#15918,#15919,#15920,#15921,#15922,
#15923,#15924,#15925,#15926,#15927,#15928,#15929,#15930,#15931,#15932,#15933,
#15934,#15935,#15936,#15937,#15938,#15939,#15940,#15941,#15942,#15943,#15944,
#15945,#15946,#15947,#15948,#15949,#15950,#15951,#15952,#15953,#15954,#15955,
#15956,#15957,#15958,#15959,#15960,#15961,#15962,#15963,#15964)),
 .UNSPECIFIED.,.F.,.F.,.F.)
B_SPLINE_SURFACE_WITH_KNOTS((2,2),(3,2,2,2,2,2,2,2,2,2,2,2,2,2,2,2,2,2,
2,2,2,2,2,2,2,2,2,2,2,2,2,2,2,2,2,2,2,2,2,2,2,2,2,2,2,2,2,2,2,2,2,2,2,2,
2,2,2,2,2,2,2,2,2,2,2,2,2,2,2,2,2,2,3),(0.,1.),(0.,0.0138888888888889,0.0277777777777778,
0.0416666666666667,0.0555555555555556,0.0694444444444444,0.0833333333333333,
0.0972222222222222,0.111111111111111,0.125,0.138888888888889,0.152777777777778,
0.166666666666667,0.180555555555556,0.194444444444444,0.208333333333333,
0.222222222222222,0.236111111111111,0.25,0.263888888888889,0.277777777777778,
0.291666666666667,0.305555555555556,0.319444444444444,0.333333333333333,
0.347222222222222,0.361111111111111,0.375,0.388888888888889,0.402777777777778,
0.416666666666667,0.430555555555556,0.444444444444444,0.458333333333333,
0.472222222222222,0.486111111111111,0.5,0.513888888888889,0.527777777777778,
0.541666666666667,0.555555555555556,0.569444444444444,0.583333333333333,
0.597222222222222,0.611111111111111,0.625,0.638888888888889,0.652777777777778,
0.666666666666667,0.680555555555556,0.694444444444444,0.708333333333333,
0.722222222222222,0.736111111111111,0.75,0.763888888888889,0.777777777777778,
0.791666666666667,0.805555555555556,0.819444444444444,0.833333333333333,
0.847222222222222,0.861111111111111,0.875,0.888888888888889,0.902777777777778,
0.916666666666667,0.930555555555556,0.944444444444444,0.958333333333333,
0.972222222222222,0.986111111111111,1.),.UNSPECIFIED.)
GEOMETRIC_REPRESENTATION_ITEM()
RATIONAL_B_SPLINE_SURFACE(((1.,0.965925826289068,1.,0.965925826289068,1.,
0.965925826289068,1.,0.965925826289068,1.,0.965925826289068,1.,0.965925826289068,
1.,0.965925826289068,1.,0.965925826289068,1.,0.965925826289068,1.,0.965925826289068,
1.,0.965925826289068,1.,0.965925826289068,1.,0.965925826289068,1.,0.965925826289068,
1.,0.965925826289068,1.,0.965925826289068,1.,0.965925826289068,1.,0.965925826289068,
1.,0.965925826289068,1.,0.965925826289068,1.,0.965925826289068,1.,0.965925826289068,
1.,0.965925826289068,1.,0.965925826289068,1.,0.965925826289068,1.,0.965925826289068,
1.,0.965925826289068,1.,0.965925826289068,1.,0.965925826289068,1.,0.965925826289068,
1.,0.965925826289068,1.,0.965925826289068,1.,0.965925826289068,1.,0.965925826289068,
1.,0.965925826289068,1.,0.965925826289068,1.,0.965925826289068,1.,0.965925826289068,
1.,0.965925826289068,1.,0.965925826289068,1.,0.965925826289068,1.,0.965925826289068,
1.,0.965925826289068,1.,0.965925826289068,1.,0.965925826289068,1.,0.965925826289068,
1.,0.965925826289068,1.,0.965925826289068,1.,0.965925826289068,1.,0.965925826289068,
1.,0.965925826289068,1.,0.965925826289068,1.,0.965925826289068,1.,0.965925826289068,
1.,0.965925826289068,1.,0.965925826289068,1.,0.965925826289068,1.,0.965925826289068,
1.,0.965925826289068,1.,0.965925826289068,1.,0.965925826289068,1.,0.965925826289068,
1.,0.965925826289068,1.,0.965925826289068,1.,0.965925826289068,1.,0.965925826289068,
1.,0.965925826289068,1.,0.965925826289068,1.,0.965925826289068,1.,0.965925826289068,
1.,0.965925826289068,1.,0.965925826289068,1.),(1.,0.965925826289068,1.,
0.965925826289068,1.,0.965925826289068,1.,0.965925826289068,1.,0.965925826289068,
1.,0.965925826289068,1.,0.965925826289068,1.,0.965925826289068,1.,0.965925826289068,
1.,0.965925826289068,1.,0.965925826289068,1.,0.965925826289068,1.,0.965925826289068,
1.,0.965925826289068,1.,0.965925826289068,1.,0.965925826289068,1.,0.965925826289068,
1.,0.965925826289068,1.,0.965925826289068,1.,0.965925826289068,1.,0.965925826289068,
1.,0.965925826289068,1.,0.965925826289068,1.,0.965925826289068,1.,0.965925826289068,
1.,0.965925826289068,1.,0.965925826289068,1.,0.965925826289068,1.,0.965925826289068,
1.,0.965925826289068,1.,0.965925826289068,1.,0.965925826289068,1.,0.965925826289068,
1.,0.965925826289068,1.,0.965925826289068,1.,0.965925826289068,1.,0.965925826289068,
1.,0.965925826289068,1.,0.965925826289068,1.,0.965925826289068,1.,0.965925826289068,
1.,0.965925826289068,1.,0.965925826289068,1.,0.965925826289068,1.,0.965925826289068,
1.,0.965925826289068,1.,0.965925826289068,1.,0.965925826289068,1.,0.965925826289068,
1.,0.965925826289068,1.,0.965925826289068,1.,0.965925826289068,1.,0.965925826289068,
1.,0.965925826289068,1.,0.965925826289068,1.,0.965925826289068,1.,0.965925826289068,
1.,0.965925826289068,1.,0.965925826289068,1.,0.965925826289068,1.,0.965925826289068,
1.,0.965925826289068,1.,0.965925826289068,1.,0.965925826289068,1.,0.965925826289068,
1.,0.965925826289068,1.,0.965925826289068,1.,0.965925826289068,1.,0.965925826289068,
1.,0.965925826289068,1.,0.965925826289068,1.,0.965925826289068,1.)))
REPRESENTATION_ITEM('')
SURFACE()
);
#185=(
BOUNDED_SURFACE()
B_SPLINE_SURFACE(1,2,((#15973,#15974,#15975,#15976,#15977,#15978,#15979,
#15980,#15981,#15982,#15983,#15984,#15985,#15986,#15987,#15988,#15989,#15990,
#15991,#15992,#15993,#15994,#15995,#15996,#15997,#15998,#15999,#16000,#16001,
#16002,#16003,#16004,#16005,#16006,#16007,#16008,#16009,#16010,#16011,#16012,
#16013,#16014,#16015,#16016,#16017,#16018,#16019,#16020,#16021,#16022,#16023,
#16024,#16025,#16026,#16027,#16028,#16029,#16030,#16031,#16032,#16033,#16034,
#16035,#16036,#16037,#16038,#16039,#16040,#16041,#16042,#16043,#16044,#16045,
#16046,#16047,#16048,#16049,#16050,#16051,#16052,#16053,#16054,#16055,#16056,
#16057,#16058,#16059,#16060,#16061,#16062,#16063,#16064,#16065,#16066,#16067,
#16068,#16069,#16070,#16071,#16072,#16073,#16074,#16075,#16076,#16077,#16078,
#16079,#16080,#16081,#16082,#16083,#16084,#16085,#16086,#16087,#16088,#16089,
#16090,#16091,#16092,#16093,#16094,#16095,#16096,#16097,#16098,#16099,#16100,
#16101,#16102,#16103,#16104,#16105,#16106,#16107,#16108,#16109,#16110,#16111,
#16112,#16113,#16114,#16115,#16116,#16117),(#16118,#16119,#16120,#16121,
#16122,#16123,#16124,#16125,#16126,#16127,#16128,#16129,#16130,#16131,#16132,
#16133,#16134,#16135,#16136,#16137,#16138,#16139,#16140,#16141,#16142,#16143,
#16144,#16145,#16146,#16147,#16148,#16149,#16150,#16151,#16152,#16153,#16154,
#16155,#16156,#16157,#16158,#16159,#16160,#16161,#16162,#16163,#16164,#16165,
#16166,#16167,#16168,#16169,#16170,#16171,#16172,#16173,#16174,#16175,#16176,
#16177,#16178,#16179,#16180,#16181,#16182,#16183,#16184,#16185,#16186,#16187,
#16188,#16189,#16190,#16191,#16192,#16193,#16194,#16195,#16196,#16197,#16198,
#16199,#16200,#16201,#16202,#16203,#16204,#16205,#16206,#16207,#16208,#16209,
#16210,#16211,#16212,#16213,#16214,#16215,#16216,#16217,#16218,#16219,#16220,
#16221,#16222,#16223,#16224,#16225,#16226,#16227,#16228,#16229,#16230,#16231,
#16232,#16233,#16234,#16235,#16236,#16237,#16238,#16239,#16240,#16241,#16242,
#16243,#16244,#16245,#16246,#16247,#16248,#16249,#16250,#16251,#16252,#16253,
#16254,#16255,#16256,#16257,#16258,#16259,#16260,#16261,#16262)),
 .UNSPECIFIED.,.F.,.F.,.F.)
B_SPLINE_SURFACE_WITH_KNOTS((2,2),(3,2,2,2,2,2,2,2,2,2,2,2,2,2,2,2,2,2,
2,2,2,2,2,2,2,2,2,2,2,2,2,2,2,2,2,2,2,2,2,2,2,2,2,2,2,2,2,2,2,2,2,2,2,2,
2,2,2,2,2,2,2,2,2,2,2,2,2,2,2,2,2,2,3),(0.,1.),(0.,0.0138888888888889,0.0277777777777778,
0.0416666666666667,0.0555555555555556,0.0694444444444444,0.0833333333333333,
0.0972222222222222,0.111111111111111,0.125,0.138888888888889,0.152777777777778,
0.166666666666667,0.180555555555556,0.194444444444444,0.208333333333333,
0.222222222222222,0.236111111111111,0.25,0.263888888888889,0.277777777777778,
0.291666666666667,0.305555555555556,0.319444444444444,0.333333333333333,
0.347222222222222,0.361111111111111,0.375,0.388888888888889,0.402777777777778,
0.416666666666667,0.430555555555556,0.444444444444444,0.458333333333333,
0.472222222222222,0.486111111111111,0.5,0.513888888888889,0.527777777777778,
0.541666666666667,0.555555555555556,0.569444444444444,0.583333333333333,
0.597222222222222,0.611111111111111,0.625,0.638888888888889,0.652777777777778,
0.666666666666667,0.680555555555556,0.694444444444444,0.708333333333333,
0.722222222222222,0.736111111111111,0.75,0.763888888888889,0.777777777777778,
0.791666666666667,0.805555555555556,0.819444444444444,0.833333333333333,
0.847222222222222,0.861111111111111,0.875,0.888888888888889,0.902777777777778,
0.916666666666667,0.930555555555556,0.944444444444444,0.958333333333333,
0.972222222222222,0.986111111111111,1.),.UNSPECIFIED.)
GEOMETRIC_REPRESENTATION_ITEM()
RATIONAL_B_SPLINE_SURFACE(((1.,0.965925826289068,1.,0.965925826289068,1.,
0.965925826289068,1.,0.965925826289068,1.,0.965925826289068,1.,0.965925826289068,
1.,0.965925826289068,1.,0.965925826289068,1.,0.965925826289068,1.,0.965925826289068,
1.,0.965925826289068,1.,0.965925826289068,1.,0.965925826289068,1.,0.965925826289068,
1.,0.965925826289068,1.,0.965925826289068,1.,0.965925826289068,1.,0.965925826289068,
1.,0.965925826289068,1.,0.965925826289068,1.,0.965925826289068,1.,0.965925826289068,
1.,0.965925826289068,1.,0.965925826289068,1.,0.965925826289068,1.,0.965925826289068,
1.,0.965925826289068,1.,0.965925826289068,1.,0.965925826289068,1.,0.965925826289068,
1.,0.965925826289068,1.,0.965925826289068,1.,0.965925826289068,1.,0.965925826289068,
1.,0.965925826289068,1.,0.965925826289068,1.,0.965925826289068,1.,0.965925826289068,
1.,0.965925826289068,1.,0.965925826289068,1.,0.965925826289068,1.,0.965925826289068,
1.,0.965925826289068,1.,0.965925826289068,1.,0.965925826289068,1.,0.965925826289068,
1.,0.965925826289068,1.,0.965925826289068,1.,0.965925826289068,1.,0.965925826289068,
1.,0.965925826289068,1.,0.965925826289068,1.,0.965925826289068,1.,0.965925826289068,
1.,0.965925826289068,1.,0.965925826289068,1.,0.965925826289068,1.,0.965925826289068,
1.,0.965925826289068,1.,0.965925826289068,1.,0.965925826289068,1.,0.965925826289068,
1.,0.965925826289068,1.,0.965925826289068,1.,0.965925826289068,1.,0.965925826289068,
1.,0.965925826289068,1.,0.965925826289068,1.,0.965925826289068,1.,0.965925826289068,
1.,0.965925826289068,1.,0.965925826289068,1.),(1.,0.965925826289068,1.,
0.965925826289068,1.,0.965925826289068,1.,0.965925826289068,1.,0.965925826289068,
1.,0.965925826289068,1.,0.965925826289068,1.,0.965925826289068,1.,0.965925826289068,
1.,0.965925826289068,1.,0.965925826289068,1.,0.965925826289068,1.,0.965925826289068,
1.,0.965925826289068,1.,0.965925826289068,1.,0.965925826289068,1.,0.965925826289068,
1.,0.965925826289068,1.,0.965925826289068,1.,0.965925826289068,1.,0.965925826289068,
1.,0.965925826289068,1.,0.965925826289068,1.,0.965925826289068,1.,0.965925826289068,
1.,0.965925826289068,1.,0.965925826289068,1.,0.965925826289068,1.,0.965925826289068,
1.,0.965925826289068,1.,0.965925826289068,1.,0.965925826289068,1.,0.965925826289068,
1.,0.965925826289068,1.,0.965925826289068,1.,0.965925826289068,1.,0.965925826289068,
1.,0.965925826289068,1.,0.965925826289068,1.,0.965925826289068,1.,0.965925826289068,
1.,0.965925826289068,1.,0.965925826289068,1.,0.965925826289068,1.,0.965925826289068,
1.,0.965925826289068,1.,0.965925826289068,1.,0.965925826289068,1.,0.965925826289068,
1.,0.965925826289068,1.,0.965925826289068,1.,0.965925826289068,1.,0.965925826289068,
1.,0.965925826289068,1.,0.965925826289068,1.,0.965925826289068,1.,0.965925826289068,
1.,0.965925826289068,1.,0.965925826289068,1.,0.965925826289068,1.,0.965925826289068,
1.,0.965925826289068,1.,0.965925826289068,1.,0.965925826289068,1.,0.965925826289068,
1.,0.965925826289068,1.,0.965925826289068,1.,0.965925826289068,1.,0.965925826289068,
1.,0.965925826289068,1.,0.965925826289068,1.,0.965925826289068,1.)))
REPRESENTATION_ITEM('')
SURFACE()
);
#186=(
BOUNDED_SURFACE()
B_SPLINE_SURFACE(1,2,((#16271,#16272,#16273,#16274,#16275,#16276,#16277,
#16278,#16279,#16280,#16281,#16282,#16283,#16284,#16285,#16286,#16287,#16288,
#16289,#16290,#16291,#16292,#16293,#16294,#16295,#16296,#16297,#16298,#16299,
#16300,#16301,#16302,#16303,#16304,#16305,#16306,#16307,#16308,#16309,#16310,
#16311,#16312,#16313,#16314,#16315,#16316,#16317,#16318,#16319,#16320,#16321,
#16322,#16323,#16324,#16325,#16326,#16327,#16328,#16329,#16330,#16331,#16332,
#16333,#16334,#16335,#16336,#16337,#16338,#16339,#16340,#16341,#16342,#16343,
#16344,#16345,#16346,#16347,#16348,#16349,#16350,#16351,#16352,#16353,#16354,
#16355,#16356,#16357,#16358,#16359,#16360,#16361,#16362,#16363,#16364,#16365,
#16366,#16367,#16368,#16369,#16370,#16371,#16372,#16373,#16374,#16375,#16376,
#16377,#16378,#16379,#16380,#16381,#16382,#16383,#16384,#16385,#16386,#16387,
#16388,#16389,#16390,#16391,#16392,#16393,#16394,#16395,#16396,#16397,#16398,
#16399,#16400,#16401,#16402,#16403,#16404,#16405,#16406,#16407,#16408,#16409,
#16410,#16411,#16412,#16413,#16414,#16415),(#16416,#16417,#16418,#16419,
#16420,#16421,#16422,#16423,#16424,#16425,#16426,#16427,#16428,#16429,#16430,
#16431,#16432,#16433,#16434,#16435,#16436,#16437,#16438,#16439,#16440,#16441,
#16442,#16443,#16444,#16445,#16446,#16447,#16448,#16449,#16450,#16451,#16452,
#16453,#16454,#16455,#16456,#16457,#16458,#16459,#16460,#16461,#16462,#16463,
#16464,#16465,#16466,#16467,#16468,#16469,#16470,#16471,#16472,#16473,#16474,
#16475,#16476,#16477,#16478,#16479,#16480,#16481,#16482,#16483,#16484,#16485,
#16486,#16487,#16488,#16489,#16490,#16491,#16492,#16493,#16494,#16495,#16496,
#16497,#16498,#16499,#16500,#16501,#16502,#16503,#16504,#16505,#16506,#16507,
#16508,#16509,#16510,#16511,#16512,#16513,#16514,#16515,#16516,#16517,#16518,
#16519,#16520,#16521,#16522,#16523,#16524,#16525,#16526,#16527,#16528,#16529,
#16530,#16531,#16532,#16533,#16534,#16535,#16536,#16537,#16538,#16539,#16540,
#16541,#16542,#16543,#16544,#16545,#16546,#16547,#16548,#16549,#16550,#16551,
#16552,#16553,#16554,#16555,#16556,#16557,#16558,#16559,#16560)),
 .UNSPECIFIED.,.F.,.F.,.F.)
B_SPLINE_SURFACE_WITH_KNOTS((2,2),(3,2,2,2,2,2,2,2,2,2,2,2,2,2,2,2,2,2,
2,2,2,2,2,2,2,2,2,2,2,2,2,2,2,2,2,2,2,2,2,2,2,2,2,2,2,2,2,2,2,2,2,2,2,2,
2,2,2,2,2,2,2,2,2,2,2,2,2,2,2,2,2,2,3),(0.,1.),(0.,0.0138888888888889,0.0277777777777778,
0.0416666666666667,0.0555555555555556,0.0694444444444444,0.0833333333333333,
0.0972222222222222,0.111111111111111,0.125,0.138888888888889,0.152777777777778,
0.166666666666667,0.180555555555556,0.194444444444444,0.208333333333333,
0.222222222222222,0.236111111111111,0.25,0.263888888888889,0.277777777777778,
0.291666666666667,0.305555555555556,0.319444444444444,0.333333333333333,
0.347222222222222,0.361111111111111,0.375,0.388888888888889,0.402777777777778,
0.416666666666667,0.430555555555556,0.444444444444444,0.458333333333333,
0.472222222222222,0.486111111111111,0.5,0.513888888888889,0.527777777777778,
0.541666666666667,0.555555555555556,0.569444444444444,0.583333333333333,
0.597222222222222,0.611111111111111,0.625,0.638888888888889,0.652777777777778,
0.666666666666667,0.680555555555556,0.694444444444444,0.708333333333333,
0.722222222222222,0.736111111111111,0.75,0.763888888888889,0.777777777777778,
0.791666666666667,0.805555555555556,0.819444444444444,0.833333333333333,
0.847222222222222,0.861111111111111,0.875,0.888888888888889,0.902777777777778,
0.916666666666667,0.930555555555556,0.944444444444444,0.958333333333333,
0.972222222222222,0.986111111111111,1.),.UNSPECIFIED.)
GEOMETRIC_REPRESENTATION_ITEM()
RATIONAL_B_SPLINE_SURFACE(((1.,0.965925826289068,1.,0.965925826289068,1.,
0.965925826289068,1.,0.965925826289068,1.,0.965925826289068,1.,0.965925826289068,
1.,0.965925826289068,1.,0.965925826289068,1.,0.965925826289068,1.,0.965925826289068,
1.,0.965925826289068,1.,0.965925826289068,1.,0.965925826289068,1.,0.965925826289068,
1.,0.965925826289068,1.,0.965925826289068,1.,0.965925826289068,1.,0.965925826289068,
1.,0.965925826289068,1.,0.965925826289068,1.,0.965925826289068,1.,0.965925826289068,
1.,0.965925826289068,1.,0.965925826289068,1.,0.965925826289068,1.,0.965925826289068,
1.,0.965925826289068,1.,0.965925826289068,1.,0.965925826289068,1.,0.965925826289068,
1.,0.965925826289068,1.,0.965925826289068,1.,0.965925826289068,1.,0.965925826289068,
1.,0.965925826289068,1.,0.965925826289068,1.,0.965925826289068,1.,0.965925826289068,
1.,0.965925826289068,1.,0.965925826289068,1.,0.965925826289068,1.,0.965925826289068,
1.,0.965925826289068,1.,0.965925826289068,1.,0.965925826289068,1.,0.965925826289068,
1.,0.965925826289068,1.,0.965925826289068,1.,0.965925826289068,1.,0.965925826289068,
1.,0.965925826289068,1.,0.965925826289068,1.,0.965925826289068,1.,0.965925826289068,
1.,0.965925826289068,1.,0.965925826289068,1.,0.965925826289068,1.,0.965925826289068,
1.,0.965925826289068,1.,0.965925826289068,1.,0.965925826289068,1.,0.965925826289068,
1.,0.965925826289068,1.,0.965925826289068,1.,0.965925826289068,1.,0.965925826289068,
1.,0.965925826289068,1.,0.965925826289068,1.,0.965925826289068,1.,0.965925826289068,
1.,0.965925826289068,1.,0.965925826289068,1.),(1.,0.965925826289068,1.,
0.965925826289068,1.,0.965925826289068,1.,0.965925826289068,1.,0.965925826289068,
1.,0.965925826289068,1.,0.965925826289068,1.,0.965925826289068,1.,0.965925826289068,
1.,0.965925826289068,1.,0.965925826289068,1.,0.965925826289068,1.,0.965925826289068,
1.,0.965925826289068,1.,0.965925826289068,1.,0.965925826289068,1.,0.965925826289068,
1.,0.965925826289068,1.,0.965925826289068,1.,0.965925826289068,1.,0.965925826289068,
1.,0.965925826289068,1.,0.965925826289068,1.,0.965925826289068,1.,0.965925826289068,
1.,0.965925826289068,1.,0.965925826289068,1.,0.965925826289068,1.,0.965925826289068,
1.,0.965925826289068,1.,0.965925826289068,1.,0.965925826289068,1.,0.965925826289068,
1.,0.965925826289068,1.,0.965925826289068,1.,0.965925826289068,1.,0.965925826289068,
1.,0.965925826289068,1.,0.965925826289068,1.,0.965925826289068,1.,0.965925826289068,
1.,0.965925826289068,1.,0.965925826289068,1.,0.965925826289068,1.,0.965925826289068,
1.,0.965925826289068,1.,0.965925826289068,1.,0.965925826289068,1.,0.965925826289068,
1.,0.965925826289068,1.,0.965925826289068,1.,0.965925826289068,1.,0.965925826289068,
1.,0.965925826289068,1.,0.965925826289068,1.,0.965925826289068,1.,0.965925826289068,
1.,0.965925826289068,1.,0.965925826289068,1.,0.965925826289068,1.,0.965925826289068,
1.,0.965925826289068,1.,0.965925826289068,1.,0.965925826289068,1.,0.965925826289068,
1.,0.965925826289068,1.,0.965925826289068,1.,0.965925826289068,1.,0.965925826289068,
1.,0.965925826289068,1.,0.965925826289068,1.,0.965925826289068,1.)))
REPRESENTATION_ITEM('')
SURFACE()
);
#187=(
BOUNDED_SURFACE()
B_SPLINE_SURFACE(1,2,((#16577,#16578,#16579,#16580,#16581,#16582,#16583,
#16584,#16585,#16586,#16587,#16588,#16589,#16590,#16591,#16592,#16593,#16594,
#16595,#16596,#16597,#16598,#16599,#16600,#16601,#16602,#16603,#16604,#16605,
#16606,#16607,#16608,#16609,#16610,#16611,#16612,#16613,#16614,#16615,#16616,
#16617,#16618,#16619,#16620,#16621,#16622,#16623,#16624,#16625,#16626,#16627,
#16628,#16629,#16630,#16631,#16632,#16633,#16634,#16635,#16636,#16637,#16638,
#16639,#16640,#16641,#16642,#16643,#16644,#16645,#16646,#16647,#16648,#16649,
#16650,#16651,#16652,#16653,#16654,#16655,#16656,#16657,#16658,#16659,#16660,
#16661,#16662,#16663,#16664,#16665,#16666,#16667,#16668,#16669,#16670,#16671,
#16672,#16673,#16674,#16675,#16676,#16677,#16678,#16679,#16680,#16681,#16682,
#16683,#16684,#16685,#16686,#16687,#16688,#16689,#16690,#16691,#16692,#16693,
#16694,#16695,#16696,#16697,#16698,#16699,#16700,#16701,#16702,#16703,#16704,
#16705,#16706,#16707,#16708,#16709,#16710,#16711,#16712,#16713,#16714,#16715,
#16716,#16717,#16718,#16719,#16720,#16721),(#16722,#16723,#16724,#16725,
#16726,#16727,#16728,#16729,#16730,#16731,#16732,#16733,#16734,#16735,#16736,
#16737,#16738,#16739,#16740,#16741,#16742,#16743,#16744,#16745,#16746,#16747,
#16748,#16749,#16750,#16751,#16752,#16753,#16754,#16755,#16756,#16757,#16758,
#16759,#16760,#16761,#16762,#16763,#16764,#16765,#16766,#16767,#16768,#16769,
#16770,#16771,#16772,#16773,#16774,#16775,#16776,#16777,#16778,#16779,#16780,
#16781,#16782,#16783,#16784,#16785,#16786,#16787,#16788,#16789,#16790,#16791,
#16792,#16793,#16794,#16795,#16796,#16797,#16798,#16799,#16800,#16801,#16802,
#16803,#16804,#16805,#16806,#16807,#16808,#16809,#16810,#16811,#16812,#16813,
#16814,#16815,#16816,#16817,#16818,#16819,#16820,#16821,#16822,#16823,#16824,
#16825,#16826,#16827,#16828,#16829,#16830,#16831,#16832,#16833,#16834,#16835,
#16836,#16837,#16838,#16839,#16840,#16841,#16842,#16843,#16844,#16845,#16846,
#16847,#16848,#16849,#16850,#16851,#16852,#16853,#16854,#16855,#16856,#16857,
#16858,#16859,#16860,#16861,#16862,#16863,#16864,#16865,#16866)),
 .UNSPECIFIED.,.F.,.F.,.F.)
B_SPLINE_SURFACE_WITH_KNOTS((2,2),(3,2,2,2,2,2,2,2,2,2,2,2,2,2,2,2,2,2,
2,2,2,2,2,2,2,2,2,2,2,2,2,2,2,2,2,2,2,2,2,2,2,2,2,2,2,2,2,2,2,2,2,2,2,2,
2,2,2,2,2,2,2,2,2,2,2,2,2,2,2,2,2,2,3),(0.,1.),(0.,0.0138888888888889,0.0277777777777778,
0.0416666666666667,0.0555555555555556,0.0694444444444444,0.0833333333333333,
0.0972222222222222,0.111111111111111,0.125,0.138888888888889,0.152777777777778,
0.166666666666667,0.180555555555556,0.194444444444444,0.208333333333333,
0.222222222222222,0.236111111111111,0.25,0.263888888888889,0.277777777777778,
0.291666666666667,0.305555555555556,0.319444444444444,0.333333333333333,
0.347222222222222,0.361111111111111,0.375,0.388888888888889,0.402777777777778,
0.416666666666667,0.430555555555556,0.444444444444444,0.458333333333333,
0.472222222222222,0.486111111111111,0.5,0.513888888888889,0.527777777777778,
0.541666666666667,0.555555555555556,0.569444444444444,0.583333333333333,
0.597222222222222,0.611111111111111,0.625,0.638888888888889,0.652777777777778,
0.666666666666667,0.680555555555556,0.694444444444444,0.708333333333333,
0.722222222222222,0.736111111111111,0.75,0.763888888888889,0.777777777777778,
0.791666666666667,0.805555555555556,0.819444444444444,0.833333333333333,
0.847222222222222,0.861111111111111,0.875,0.888888888888889,0.902777777777778,
0.916666666666667,0.930555555555556,0.944444444444444,0.958333333333333,
0.972222222222222,0.986111111111111,1.),.UNSPECIFIED.)
GEOMETRIC_REPRESENTATION_ITEM()
RATIONAL_B_SPLINE_SURFACE(((1.,0.965925826289068,1.,0.965925826289068,1.,
0.965925826289068,1.,0.965925826289068,1.,0.965925826289068,1.,0.965925826289068,
1.,0.965925826289068,1.,0.965925826289068,1.,0.965925826289068,1.,0.965925826289068,
1.,0.965925826289068,1.,0.965925826289068,1.,0.965925826289068,1.,0.965925826289068,
1.,0.965925826289068,1.,0.965925826289068,1.,0.965925826289068,1.,0.965925826289068,
1.,0.965925826289068,1.,0.965925826289068,1.,0.965925826289068,1.,0.965925826289068,
1.,0.965925826289068,1.,0.965925826289068,1.,0.965925826289068,1.,0.965925826289068,
1.,0.965925826289068,1.,0.965925826289068,1.,0.965925826289068,1.,0.965925826289068,
1.,0.965925826289068,1.,0.965925826289068,1.,0.965925826289068,1.,0.965925826289068,
1.,0.965925826289068,1.,0.965925826289068,1.,0.965925826289068,1.,0.965925826289068,
1.,0.965925826289068,1.,0.965925826289068,1.,0.965925826289068,1.,0.965925826289068,
1.,0.965925826289068,1.,0.965925826289068,1.,0.965925826289068,1.,0.965925826289068,
1.,0.965925826289068,1.,0.965925826289068,1.,0.965925826289068,1.,0.965925826289068,
1.,0.965925826289068,1.,0.965925826289068,1.,0.965925826289068,1.,0.965925826289068,
1.,0.965925826289068,1.,0.965925826289068,1.,0.965925826289068,1.,0.965925826289068,
1.,0.965925826289068,1.,0.965925826289068,1.,0.965925826289068,1.,0.965925826289068,
1.,0.965925826289068,1.,0.965925826289068,1.,0.965925826289068,1.,0.965925826289068,
1.,0.965925826289068,1.,0.965925826289068,1.,0.965925826289068,1.,0.965925826289068,
1.,0.965925826289068,1.,0.965925826289068,1.),(1.,0.965925826289068,1.,
0.965925826289068,1.,0.965925826289068,1.,0.965925826289068,1.,0.965925826289068,
1.,0.965925826289068,1.,0.965925826289068,1.,0.965925826289068,1.,0.965925826289068,
1.,0.965925826289068,1.,0.965925826289068,1.,0.965925826289068,1.,0.965925826289068,
1.,0.965925826289068,1.,0.965925826289068,1.,0.965925826289068,1.,0.965925826289068,
1.,0.965925826289068,1.,0.965925826289068,1.,0.965925826289068,1.,0.965925826289068,
1.,0.965925826289068,1.,0.965925826289068,1.,0.965925826289068,1.,0.965925826289068,
1.,0.965925826289068,1.,0.965925826289068,1.,0.965925826289068,1.,0.965925826289068,
1.,0.965925826289068,1.,0.965925826289068,1.,0.965925826289068,1.,0.965925826289068,
1.,0.965925826289068,1.,0.965925826289068,1.,0.965925826289068,1.,0.965925826289068,
1.,0.965925826289068,1.,0.965925826289068,1.,0.965925826289068,1.,0.965925826289068,
1.,0.965925826289068,1.,0.965925826289068,1.,0.965925826289068,1.,0.965925826289068,
1.,0.965925826289068,1.,0.965925826289068,1.,0.965925826289068,1.,0.965925826289068,
1.,0.965925826289068,1.,0.965925826289068,1.,0.965925826289068,1.,0.965925826289068,
1.,0.965925826289068,1.,0.965925826289068,1.,0.965925826289068,1.,0.965925826289068,
1.,0.965925826289068,1.,0.965925826289068,1.,0.965925826289068,1.,0.965925826289068,
1.,0.965925826289068,1.,0.965925826289068,1.,0.965925826289068,1.,0.965925826289068,
1.,0.965925826289068,1.,0.965925826289068,1.,0.965925826289068,1.,0.965925826289068,
1.,0.965925826289068,1.,0.965925826289068,1.,0.965925826289068,1.)))
REPRESENTATION_ITEM('')
SURFACE()
);
#188=(
BOUNDED_SURFACE()
B_SPLINE_SURFACE(1,2,((#17011,#17012,#17013,#17014,#17015,#17016,#17017,
#17018,#17019,#17020,#17021,#17022,#17023,#17024,#17025,#17026,#17027,#17028,
#17029,#17030,#17031,#17032,#17033,#17034,#17035,#17036,#17037,#17038,#17039,
#17040,#17041,#17042,#17043,#17044,#17045,#17046,#17047,#17048,#17049,#17050,
#17051,#17052,#17053,#17054,#17055,#17056,#17057,#17058,#17059,#17060,#17061,
#17062,#17063,#17064,#17065,#17066,#17067,#17068,#17069,#17070,#17071,#17072,
#17073,#17074,#17075,#17076,#17077,#17078,#17079,#17080,#17081,#17082,#17083,
#17084,#17085,#17086,#17087,#17088,#17089,#17090,#17091,#17092,#17093,#17094,
#17095,#17096,#17097,#17098,#17099,#17100,#17101,#17102,#17103,#17104,#17105,
#17106,#17107,#17108,#17109,#17110,#17111,#17112,#17113,#17114,#17115,#17116,
#17117,#17118,#17119,#17120,#17121,#17122,#17123,#17124,#17125,#17126,#17127,
#17128,#17129,#17130,#17131,#17132,#17133,#17134,#17135,#17136,#17137,#17138,
#17139,#17140,#17141,#17142,#17143,#17144,#17145,#17146,#17147,#17148,#17149,
#17150,#17151,#17152,#17153,#17154,#17155),(#17156,#17157,#17158,#17159,
#17160,#17161,#17162,#17163,#17164,#17165,#17166,#17167,#17168,#17169,#17170,
#17171,#17172,#17173,#17174,#17175,#17176,#17177,#17178,#17179,#17180,#17181,
#17182,#17183,#17184,#17185,#17186,#17187,#17188,#17189,#17190,#17191,#17192,
#17193,#17194,#17195,#17196,#17197,#17198,#17199,#17200,#17201,#17202,#17203,
#17204,#17205,#17206,#17207,#17208,#17209,#17210,#17211,#17212,#17213,#17214,
#17215,#17216,#17217,#17218,#17219,#17220,#17221,#17222,#17223,#17224,#17225,
#17226,#17227,#17228,#17229,#17230,#17231,#17232,#17233,#17234,#17235,#17236,
#17237,#17238,#17239,#17240,#17241,#17242,#17243,#17244,#17245,#17246,#17247,
#17248,#17249,#17250,#17251,#17252,#17253,#17254,#17255,#17256,#17257,#17258,
#17259,#17260,#17261,#17262,#17263,#17264,#17265,#17266,#17267,#17268,#17269,
#17270,#17271,#17272,#17273,#17274,#17275,#17276,#17277,#17278,#17279,#17280,
#17281,#17282,#17283,#17284,#17285,#17286,#17287,#17288,#17289,#17290,#17291,
#17292,#17293,#17294,#17295,#17296,#17297,#17298,#17299,#17300)),
 .UNSPECIFIED.,.F.,.F.,.F.)
B_SPLINE_SURFACE_WITH_KNOTS((2,2),(3,2,2,2,2,2,2,2,2,2,2,2,2,2,2,2,2,2,
2,2,2,2,2,2,2,2,2,2,2,2,2,2,2,2,2,2,2,2,2,2,2,2,2,2,2,2,2,2,2,2,2,2,2,2,
2,2,2,2,2,2,2,2,2,2,2,2,2,2,2,2,2,2,3),(0.,1.),(0.,0.0138888888888889,0.0277777777777778,
0.0416666666666667,0.0555555555555556,0.0694444444444444,0.0833333333333333,
0.0972222222222222,0.111111111111111,0.125,0.138888888888889,0.152777777777778,
0.166666666666667,0.180555555555556,0.194444444444444,0.208333333333333,
0.222222222222222,0.236111111111111,0.25,0.263888888888889,0.277777777777778,
0.291666666666667,0.305555555555556,0.319444444444444,0.333333333333333,
0.347222222222222,0.361111111111111,0.375,0.388888888888889,0.402777777777778,
0.416666666666667,0.430555555555556,0.444444444444444,0.458333333333333,
0.472222222222222,0.486111111111111,0.5,0.513888888888889,0.527777777777778,
0.541666666666667,0.555555555555556,0.569444444444444,0.583333333333333,
0.597222222222222,0.611111111111111,0.625,0.638888888888889,0.652777777777778,
0.666666666666667,0.680555555555556,0.694444444444444,0.708333333333333,
0.722222222222222,0.736111111111111,0.75,0.763888888888889,0.777777777777778,
0.791666666666667,0.805555555555556,0.819444444444444,0.833333333333333,
0.847222222222222,0.861111111111111,0.875,0.888888888888889,0.902777777777778,
0.916666666666667,0.930555555555556,0.944444444444444,0.958333333333333,
0.972222222222222,0.986111111111111,1.),.UNSPECIFIED.)
GEOMETRIC_REPRESENTATION_ITEM()
RATIONAL_B_SPLINE_SURFACE(((1.,0.965925826289068,1.,0.965925826289068,1.,
0.965925826289068,1.,0.965925826289068,1.,0.965925826289068,1.,0.965925826289068,
1.,0.965925826289068,1.,0.965925826289068,1.,0.965925826289068,1.,0.965925826289068,
1.,0.965925826289068,1.,0.965925826289068,1.,0.965925826289068,1.,0.965925826289068,
1.,0.965925826289068,1.,0.965925826289068,1.,0.965925826289068,1.,0.965925826289068,
1.,0.965925826289068,1.,0.965925826289068,1.,0.965925826289068,1.,0.965925826289068,
1.,0.965925826289068,1.,0.965925826289068,1.,0.965925826289068,1.,0.965925826289068,
1.,0.965925826289068,1.,0.965925826289068,1.,0.965925826289068,1.,0.965925826289068,
1.,0.965925826289068,1.,0.965925826289068,1.,0.965925826289068,1.,0.965925826289068,
1.,0.965925826289068,1.,0.965925826289068,1.,0.965925826289068,1.,0.965925826289068,
1.,0.965925826289068,1.,0.965925826289068,1.,0.965925826289068,1.,0.965925826289068,
1.,0.965925826289068,1.,0.965925826289068,1.,0.965925826289068,1.,0.965925826289068,
1.,0.965925826289068,1.,0.965925826289068,1.,0.965925826289068,1.,0.965925826289068,
1.,0.965925826289068,1.,0.965925826289068,1.,0.965925826289068,1.,0.965925826289068,
1.,0.965925826289068,1.,0.965925826289068,1.,0.965925826289068,1.,0.965925826289068,
1.,0.965925826289068,1.,0.965925826289068,1.,0.965925826289068,1.,0.965925826289068,
1.,0.965925826289068,1.,0.965925826289068,1.,0.965925826289068,1.,0.965925826289068,
1.,0.965925826289068,1.,0.965925826289068,1.,0.965925826289068,1.,0.965925826289068,
1.,0.965925826289068,1.,0.965925826289068,1.),(1.,0.965925826289068,1.,
0.965925826289068,1.,0.965925826289068,1.,0.965925826289068,1.,0.965925826289068,
1.,0.965925826289068,1.,0.965925826289068,1.,0.965925826289068,1.,0.965925826289068,
1.,0.965925826289068,1.,0.965925826289068,1.,0.965925826289068,1.,0.965925826289068,
1.,0.965925826289068,1.,0.965925826289068,1.,0.965925826289068,1.,0.965925826289068,
1.,0.965925826289068,1.,0.965925826289068,1.,0.965925826289068,1.,0.965925826289068,
1.,0.965925826289068,1.,0.965925826289068,1.,0.965925826289068,1.,0.965925826289068,
1.,0.965925826289068,1.,0.965925826289068,1.,0.965925826289068,1.,0.965925826289068,
1.,0.965925826289068,1.,0.965925826289068,1.,0.965925826289068,1.,0.965925826289068,
1.,0.965925826289068,1.,0.965925826289068,1.,0.965925826289068,1.,0.965925826289068,
1.,0.965925826289068,1.,0.965925826289068,1.,0.965925826289068,1.,0.965925826289068,
1.,0.965925826289068,1.,0.965925826289068,1.,0.965925826289068,1.,0.965925826289068,
1.,0.965925826289068,1.,0.965925826289068,1.,0.965925826289068,1.,0.965925826289068,
1.,0.965925826289068,1.,0.965925826289068,1.,0.965925826289068,1.,0.965925826289068,
1.,0.965925826289068,1.,0.965925826289068,1.,0.965925826289068,1.,0.965925826289068,
1.,0.965925826289068,1.,0.965925826289068,1.,0.965925826289068,1.,0.965925826289068,
1.,0.965925826289068,1.,0.965925826289068,1.,0.965925826289068,1.,0.965925826289068,
1.,0.965925826289068,1.,0.965925826289068,1.,0.965925826289068,1.,0.965925826289068,
1.,0.965925826289068,1.,0.965925826289068,1.,0.965925826289068,1.)))
REPRESENTATION_ITEM('')
SURFACE()
);
#189=(
BOUNDED_SURFACE()
B_SPLINE_SURFACE(1,2,((#17308,#17309,#17310,#17311,#17312,#17313,#17314,
#17315,#17316,#17317,#17318,#17319,#17320,#17321,#17322,#17323,#17324,#17325,
#17326,#17327,#17328,#17329,#17330,#17331,#17332,#17333,#17334,#17335,#17336,
#17337,#17338,#17339,#17340,#17341,#17342,#17343,#17344,#17345,#17346,#17347,
#17348,#17349,#17350,#17351,#17352,#17353,#17354,#17355,#17356,#17357,#17358,
#17359,#17360,#17361,#17362,#17363,#17364,#17365,#17366,#17367,#17368,#17369,
#17370,#17371,#17372,#17373,#17374,#17375,#17376,#17377,#17378,#17379,#17380,
#17381,#17382,#17383,#17384,#17385,#17386,#17387,#17388,#17389,#17390,#17391,
#17392,#17393,#17394,#17395,#17396,#17397,#17398,#17399,#17400,#17401,#17402,
#17403,#17404,#17405,#17406,#17407,#17408,#17409,#17410,#17411,#17412,#17413,
#17414,#17415,#17416,#17417,#17418,#17419,#17420,#17421,#17422,#17423,#17424,
#17425,#17426,#17427,#17428,#17429,#17430,#17431,#17432,#17433,#17434,#17435,
#17436,#17437,#17438,#17439,#17440,#17441,#17442,#17443,#17444,#17445,#17446,
#17447,#17448,#17449,#17450,#17451,#17452),(#17453,#17454,#17455,#17456,
#17457,#17458,#17459,#17460,#17461,#17462,#17463,#17464,#17465,#17466,#17467,
#17468,#17469,#17470,#17471,#17472,#17473,#17474,#17475,#17476,#17477,#17478,
#17479,#17480,#17481,#17482,#17483,#17484,#17485,#17486,#17487,#17488,#17489,
#17490,#17491,#17492,#17493,#17494,#17495,#17496,#17497,#17498,#17499,#17500,
#17501,#17502,#17503,#17504,#17505,#17506,#17507,#17508,#17509,#17510,#17511,
#17512,#17513,#17514,#17515,#17516,#17517,#17518,#17519,#17520,#17521,#17522,
#17523,#17524,#17525,#17526,#17527,#17528,#17529,#17530,#17531,#17532,#17533,
#17534,#17535,#17536,#17537,#17538,#17539,#17540,#17541,#17542,#17543,#17544,
#17545,#17546,#17547,#17548,#17549,#17550,#17551,#17552,#17553,#17554,#17555,
#17556,#17557,#17558,#17559,#17560,#17561,#17562,#17563,#17564,#17565,#17566,
#17567,#17568,#17569,#17570,#17571,#17572,#17573,#17574,#17575,#17576,#17577,
#17578,#17579,#17580,#17581,#17582,#17583,#17584,#17585,#17586,#17587,#17588,
#17589,#17590,#17591,#17592,#17593,#17594,#17595,#17596,#17597)),
 .UNSPECIFIED.,.F.,.F.,.F.)
B_SPLINE_SURFACE_WITH_KNOTS((2,2),(3,2,2,2,2,2,2,2,2,2,2,2,2,2,2,2,2,2,
2,2,2,2,2,2,2,2,2,2,2,2,2,2,2,2,2,2,2,2,2,2,2,2,2,2,2,2,2,2,2,2,2,2,2,2,
2,2,2,2,2,2,2,2,2,2,2,2,2,2,2,2,2,2,3),(0.,1.),(0.,0.0138888888888889,0.0277777777777778,
0.0416666666666667,0.0555555555555556,0.0694444444444444,0.0833333333333333,
0.0972222222222222,0.111111111111111,0.125,0.138888888888889,0.152777777777778,
0.166666666666667,0.180555555555556,0.194444444444444,0.208333333333333,
0.222222222222222,0.236111111111111,0.25,0.263888888888889,0.277777777777778,
0.291666666666667,0.305555555555556,0.319444444444444,0.333333333333333,
0.347222222222222,0.361111111111111,0.375,0.388888888888889,0.402777777777778,
0.416666666666667,0.430555555555556,0.444444444444444,0.458333333333333,
0.472222222222222,0.486111111111111,0.5,0.513888888888889,0.527777777777778,
0.541666666666667,0.555555555555556,0.569444444444444,0.583333333333333,
0.597222222222222,0.611111111111111,0.625,0.638888888888889,0.652777777777778,
0.666666666666667,0.680555555555556,0.694444444444444,0.708333333333333,
0.722222222222222,0.736111111111111,0.75,0.763888888888889,0.777777777777778,
0.791666666666667,0.805555555555556,0.819444444444444,0.833333333333333,
0.847222222222222,0.861111111111111,0.875,0.888888888888889,0.902777777777778,
0.916666666666667,0.930555555555556,0.944444444444444,0.958333333333333,
0.972222222222222,0.986111111111111,1.),.UNSPECIFIED.)
GEOMETRIC_REPRESENTATION_ITEM()
RATIONAL_B_SPLINE_SURFACE(((1.,0.965925826289068,1.,0.965925826289068,1.,
0.965925826289068,1.,0.965925826289068,1.,0.965925826289068,1.,0.965925826289068,
1.,0.965925826289068,1.,0.965925826289068,1.,0.965925826289068,1.,0.965925826289068,
1.,0.965925826289068,1.,0.965925826289068,1.,0.965925826289068,1.,0.965925826289068,
1.,0.965925826289068,1.,0.965925826289068,1.,0.965925826289068,1.,0.965925826289068,
1.,0.965925826289068,1.,0.965925826289068,1.,0.965925826289068,1.,0.965925826289068,
1.,0.965925826289068,1.,0.965925826289068,1.,0.965925826289068,1.,0.965925826289068,
1.,0.965925826289068,1.,0.965925826289068,1.,0.965925826289068,1.,0.965925826289068,
1.,0.965925826289068,1.,0.965925826289068,1.,0.965925826289068,1.,0.965925826289068,
1.,0.965925826289068,1.,0.965925826289068,1.,0.965925826289068,1.,0.965925826289068,
1.,0.965925826289068,1.,0.965925826289068,1.,0.965925826289068,1.,0.965925826289068,
1.,0.965925826289068,1.,0.965925826289068,1.,0.965925826289068,1.,0.965925826289068,
1.,0.965925826289068,1.,0.965925826289068,1.,0.965925826289068,1.,0.965925826289068,
1.,0.965925826289068,1.,0.965925826289068,1.,0.965925826289068,1.,0.965925826289068,
1.,0.965925826289068,1.,0.965925826289068,1.,0.965925826289068,1.,0.965925826289068,
1.,0.965925826289068,1.,0.965925826289068,1.,0.965925826289068,1.,0.965925826289068,
1.,0.965925826289068,1.,0.965925826289068,1.,0.965925826289068,1.,0.965925826289068,
1.,0.965925826289068,1.,0.965925826289068,1.,0.965925826289068,1.,0.965925826289068,
1.,0.965925826289068,1.,0.965925826289068,1.),(1.,0.965925826289068,1.,
0.965925826289068,1.,0.965925826289068,1.,0.965925826289068,1.,0.965925826289068,
1.,0.965925826289068,1.,0.965925826289068,1.,0.965925826289068,1.,0.965925826289068,
1.,0.965925826289068,1.,0.965925826289068,1.,0.965925826289068,1.,0.965925826289068,
1.,0.965925826289068,1.,0.965925826289068,1.,0.965925826289068,1.,0.965925826289068,
1.,0.965925826289068,1.,0.965925826289068,1.,0.965925826289068,1.,0.965925826289068,
1.,0.965925826289068,1.,0.965925826289068,1.,0.965925826289068,1.,0.965925826289068,
1.,0.965925826289068,1.,0.965925826289068,1.,0.965925826289068,1.,0.965925826289068,
1.,0.965925826289068,1.,0.965925826289068,1.,0.965925826289068,1.,0.965925826289068,
1.,0.965925826289068,1.,0.965925826289068,1.,0.965925826289068,1.,0.965925826289068,
1.,0.965925826289068,1.,0.965925826289068,1.,0.965925826289068,1.,0.965925826289068,
1.,0.965925826289068,1.,0.965925826289068,1.,0.965925826289068,1.,0.965925826289068,
1.,0.965925826289068,1.,0.965925826289068,1.,0.965925826289068,1.,0.965925826289068,
1.,0.965925826289068,1.,0.965925826289068,1.,0.965925826289068,1.,0.965925826289068,
1.,0.965925826289068,1.,0.965925826289068,1.,0.965925826289068,1.,0.965925826289068,
1.,0.965925826289068,1.,0.965925826289068,1.,0.965925826289068,1.,0.965925826289068,
1.,0.965925826289068,1.,0.965925826289068,1.,0.965925826289068,1.,0.965925826289068,
1.,0.965925826289068,1.,0.965925826289068,1.,0.965925826289068,1.,0.965925826289068,
1.,0.965925826289068,1.,0.965925826289068,1.,0.965925826289068,1.)))
REPRESENTATION_ITEM('')
SURFACE()
);
#190=(
BOUNDED_SURFACE()
B_SPLINE_SURFACE(1,2,((#17653,#17654,#17655,#17656,#17657,#17658,#17659,
#17660,#17661,#17662,#17663,#17664,#17665,#17666,#17667,#17668,#17669,#17670,
#17671,#17672,#17673,#17674,#17675,#17676,#17677,#17678,#17679,#17680,#17681,
#17682,#17683,#17684,#17685,#17686,#17687,#17688,#17689,#17690,#17691,#17692,
#17693,#17694,#17695,#17696,#17697,#17698,#17699,#17700,#17701,#17702,#17703,
#17704,#17705,#17706,#17707,#17708,#17709,#17710,#17711,#17712,#17713,#17714,
#17715,#17716,#17717,#17718,#17719,#17720,#17721,#17722,#17723,#17724,#17725,
#17726,#17727,#17728,#17729,#17730,#17731,#17732,#17733,#17734,#17735,#17736,
#17737,#17738,#17739,#17740,#17741,#17742,#17743,#17744,#17745,#17746,#17747,
#17748,#17749,#17750,#17751,#17752,#17753,#17754,#17755,#17756,#17757,#17758,
#17759,#17760,#17761,#17762,#17763,#17764,#17765,#17766,#17767,#17768,#17769,
#17770,#17771,#17772,#17773,#17774,#17775,#17776,#17777,#17778,#17779,#17780,
#17781,#17782,#17783,#17784,#17785,#17786,#17787,#17788,#17789,#17790,#17791,
#17792,#17793,#17794,#17795,#17796,#17797),(#17798,#17799,#17800,#17801,
#17802,#17803,#17804,#17805,#17806,#17807,#17808,#17809,#17810,#17811,#17812,
#17813,#17814,#17815,#17816,#17817,#17818,#17819,#17820,#17821,#17822,#17823,
#17824,#17825,#17826,#17827,#17828,#17829,#17830,#17831,#17832,#17833,#17834,
#17835,#17836,#17837,#17838,#17839,#17840,#17841,#17842,#17843,#17844,#17845,
#17846,#17847,#17848,#17849,#17850,#17851,#17852,#17853,#17854,#17855,#17856,
#17857,#17858,#17859,#17860,#17861,#17862,#17863,#17864,#17865,#17866,#17867,
#17868,#17869,#17870,#17871,#17872,#17873,#17874,#17875,#17876,#17877,#17878,
#17879,#17880,#17881,#17882,#17883,#17884,#17885,#17886,#17887,#17888,#17889,
#17890,#17891,#17892,#17893,#17894,#17895,#17896,#17897,#17898,#17899,#17900,
#17901,#17902,#17903,#17904,#17905,#17906,#17907,#17908,#17909,#17910,#17911,
#17912,#17913,#17914,#17915,#17916,#17917,#17918,#17919,#17920,#17921,#17922,
#17923,#17924,#17925,#17926,#17927,#17928,#17929,#17930,#17931,#17932,#17933,
#17934,#17935,#17936,#17937,#17938,#17939,#17940,#17941,#17942)),
 .UNSPECIFIED.,.F.,.F.,.F.)
B_SPLINE_SURFACE_WITH_KNOTS((2,2),(3,2,2,2,2,2,2,2,2,2,2,2,2,2,2,2,2,2,
2,2,2,2,2,2,2,2,2,2,2,2,2,2,2,2,2,2,2,2,2,2,2,2,2,2,2,2,2,2,2,2,2,2,2,2,
2,2,2,2,2,2,2,2,2,2,2,2,2,2,2,2,2,2,3),(0.,1.),(0.,0.0138888888888889,0.0277777777777778,
0.0416666666666667,0.0555555555555556,0.0694444444444444,0.0833333333333333,
0.0972222222222222,0.111111111111111,0.125,0.138888888888889,0.152777777777778,
0.166666666666667,0.180555555555556,0.194444444444444,0.208333333333333,
0.222222222222222,0.236111111111111,0.25,0.263888888888889,0.277777777777778,
0.291666666666667,0.305555555555556,0.319444444444444,0.333333333333333,
0.347222222222222,0.361111111111111,0.375,0.388888888888889,0.402777777777778,
0.416666666666667,0.430555555555556,0.444444444444444,0.458333333333333,
0.472222222222222,0.486111111111111,0.5,0.513888888888889,0.527777777777778,
0.541666666666667,0.555555555555556,0.569444444444444,0.583333333333333,
0.597222222222222,0.611111111111111,0.625,0.638888888888889,0.652777777777778,
0.666666666666667,0.680555555555556,0.694444444444444,0.708333333333333,
0.722222222222222,0.736111111111111,0.75,0.763888888888889,0.777777777777778,
0.791666666666667,0.805555555555556,0.819444444444444,0.833333333333333,
0.847222222222222,0.861111111111111,0.875,0.888888888888889,0.902777777777778,
0.916666666666667,0.930555555555556,0.944444444444444,0.958333333333333,
0.972222222222222,0.986111111111111,1.),.UNSPECIFIED.)
GEOMETRIC_REPRESENTATION_ITEM()
RATIONAL_B_SPLINE_SURFACE(((1.,0.965925826289068,1.,0.965925826289068,1.,
0.965925826289068,1.,0.965925826289068,1.,0.965925826289068,1.,0.965925826289068,
1.,0.965925826289068,1.,0.965925826289068,1.,0.965925826289068,1.,0.965925826289068,
1.,0.965925826289068,1.,0.965925826289068,1.,0.965925826289068,1.,0.965925826289068,
1.,0.965925826289068,1.,0.965925826289068,1.,0.965925826289068,1.,0.965925826289068,
1.,0.965925826289068,1.,0.965925826289068,1.,0.965925826289068,1.,0.965925826289068,
1.,0.965925826289068,1.,0.965925826289068,1.,0.965925826289068,1.,0.965925826289068,
1.,0.965925826289068,1.,0.965925826289068,1.,0.965925826289068,1.,0.965925826289068,
1.,0.965925826289068,1.,0.965925826289068,1.,0.965925826289068,1.,0.965925826289068,
1.,0.965925826289068,1.,0.965925826289068,1.,0.965925826289068,1.,0.965925826289068,
1.,0.965925826289068,1.,0.965925826289068,1.,0.965925826289068,1.,0.965925826289068,
1.,0.965925826289068,1.,0.965925826289068,1.,0.965925826289068,1.,0.965925826289068,
1.,0.965925826289068,1.,0.965925826289068,1.,0.965925826289068,1.,0.965925826289068,
1.,0.965925826289068,1.,0.965925826289068,1.,0.965925826289068,1.,0.965925826289068,
1.,0.965925826289068,1.,0.965925826289068,1.,0.965925826289068,1.,0.965925826289068,
1.,0.965925826289068,1.,0.965925826289068,1.,0.965925826289068,1.,0.965925826289068,
1.,0.965925826289068,1.,0.965925826289068,1.,0.965925826289068,1.,0.965925826289068,
1.,0.965925826289068,1.,0.965925826289068,1.,0.965925826289068,1.,0.965925826289068,
1.,0.965925826289068,1.,0.965925826289068,1.),(1.,0.965925826289068,1.,
0.965925826289068,1.,0.965925826289068,1.,0.965925826289068,1.,0.965925826289068,
1.,0.965925826289068,1.,0.965925826289068,1.,0.965925826289068,1.,0.965925826289068,
1.,0.965925826289068,1.,0.965925826289068,1.,0.965925826289068,1.,0.965925826289068,
1.,0.965925826289068,1.,0.965925826289068,1.,0.965925826289068,1.,0.965925826289068,
1.,0.965925826289068,1.,0.965925826289068,1.,0.965925826289068,1.,0.965925826289068,
1.,0.965925826289068,1.,0.965925826289068,1.,0.965925826289068,1.,0.965925826289068,
1.,0.965925826289068,1.,0.965925826289068,1.,0.965925826289068,1.,0.965925826289068,
1.,0.965925826289068,1.,0.965925826289068,1.,0.965925826289068,1.,0.965925826289068,
1.,0.965925826289068,1.,0.965925826289068,1.,0.965925826289068,1.,0.965925826289068,
1.,0.965925826289068,1.,0.965925826289068,1.,0.965925826289068,1.,0.965925826289068,
1.,0.965925826289068,1.,0.965925826289068,1.,0.965925826289068,1.,0.965925826289068,
1.,0.965925826289068,1.,0.965925826289068,1.,0.965925826289068,1.,0.965925826289068,
1.,0.965925826289068,1.,0.965925826289068,1.,0.965925826289068,1.,0.965925826289068,
1.,0.965925826289068,1.,0.965925826289068,1.,0.965925826289068,1.,0.965925826289068,
1.,0.965925826289068,1.,0.965925826289068,1.,0.965925826289068,1.,0.965925826289068,
1.,0.965925826289068,1.,0.965925826289068,1.,0.965925826289068,1.,0.965925826289068,
1.,0.965925826289068,1.,0.965925826289068,1.,0.965925826289068,1.,0.965925826289068,
1.,0.965925826289068,1.,0.965925826289068,1.,0.965925826289068,1.)))
REPRESENTATION_ITEM('')
SURFACE()
);
#191=(
BOUNDED_SURFACE()
B_SPLINE_SURFACE(1,2,((#17973,#17974,#17975,#17976,#17977,#17978,#17979,
#17980,#17981,#17982,#17983,#17984,#17985,#17986,#17987,#17988,#17989,#17990,
#17991,#17992,#17993,#17994,#17995,#17996,#17997,#17998,#17999,#18000,#18001,
#18002,#18003,#18004,#18005,#18006,#18007,#18008,#18009,#18010,#18011,#18012,
#18013,#18014,#18015,#18016,#18017,#18018,#18019,#18020,#18021,#18022,#18023,
#18024,#18025,#18026,#18027,#18028,#18029,#18030,#18031,#18032,#18033,#18034,
#18035,#18036,#18037,#18038,#18039,#18040,#18041,#18042,#18043,#18044,#18045,
#18046,#18047,#18048,#18049,#18050,#18051,#18052,#18053,#18054,#18055,#18056,
#18057,#18058,#18059,#18060,#18061,#18062,#18063,#18064,#18065,#18066,#18067,
#18068,#18069,#18070,#18071,#18072,#18073,#18074,#18075,#18076,#18077,#18078,
#18079,#18080,#18081,#18082,#18083,#18084,#18085,#18086,#18087,#18088,#18089,
#18090,#18091,#18092,#18093,#18094,#18095,#18096,#18097,#18098,#18099,#18100,
#18101,#18102,#18103,#18104,#18105,#18106,#18107,#18108,#18109,#18110,#18111,
#18112,#18113,#18114,#18115,#18116,#18117),(#18118,#18119,#18120,#18121,
#18122,#18123,#18124,#18125,#18126,#18127,#18128,#18129,#18130,#18131,#18132,
#18133,#18134,#18135,#18136,#18137,#18138,#18139,#18140,#18141,#18142,#18143,
#18144,#18145,#18146,#18147,#18148,#18149,#18150,#18151,#18152,#18153,#18154,
#18155,#18156,#18157,#18158,#18159,#18160,#18161,#18162,#18163,#18164,#18165,
#18166,#18167,#18168,#18169,#18170,#18171,#18172,#18173,#18174,#18175,#18176,
#18177,#18178,#18179,#18180,#18181,#18182,#18183,#18184,#18185,#18186,#18187,
#18188,#18189,#18190,#18191,#18192,#18193,#18194,#18195,#18196,#18197,#18198,
#18199,#18200,#18201,#18202,#18203,#18204,#18205,#18206,#18207,#18208,#18209,
#18210,#18211,#18212,#18213,#18214,#18215,#18216,#18217,#18218,#18219,#18220,
#18221,#18222,#18223,#18224,#18225,#18226,#18227,#18228,#18229,#18230,#18231,
#18232,#18233,#18234,#18235,#18236,#18237,#18238,#18239,#18240,#18241,#18242,
#18243,#18244,#18245,#18246,#18247,#18248,#18249,#18250,#18251,#18252,#18253,
#18254,#18255,#18256,#18257,#18258,#18259,#18260,#18261,#18262)),
 .UNSPECIFIED.,.F.,.F.,.F.)
B_SPLINE_SURFACE_WITH_KNOTS((2,2),(3,2,2,2,2,2,2,2,2,2,2,2,2,2,2,2,2,2,
2,2,2,2,2,2,2,2,2,2,2,2,2,2,2,2,2,2,2,2,2,2,2,2,2,2,2,2,2,2,2,2,2,2,2,2,
2,2,2,2,2,2,2,2,2,2,2,2,2,2,2,2,2,2,3),(0.,1.),(0.,0.0138888888888889,0.0277777777777778,
0.0416666666666667,0.0555555555555556,0.0694444444444444,0.0833333333333333,
0.0972222222222222,0.111111111111111,0.125,0.138888888888889,0.152777777777778,
0.166666666666667,0.180555555555556,0.194444444444444,0.208333333333333,
0.222222222222222,0.236111111111111,0.25,0.263888888888889,0.277777777777778,
0.291666666666667,0.305555555555556,0.319444444444444,0.333333333333333,
0.347222222222222,0.361111111111111,0.375,0.388888888888889,0.402777777777778,
0.416666666666667,0.430555555555556,0.444444444444444,0.458333333333333,
0.472222222222222,0.486111111111111,0.5,0.513888888888889,0.527777777777778,
0.541666666666667,0.555555555555556,0.569444444444444,0.583333333333333,
0.597222222222222,0.611111111111111,0.625,0.638888888888889,0.652777777777778,
0.666666666666667,0.680555555555556,0.694444444444444,0.708333333333333,
0.722222222222222,0.736111111111111,0.75,0.763888888888889,0.777777777777778,
0.791666666666667,0.805555555555556,0.819444444444444,0.833333333333333,
0.847222222222222,0.861111111111111,0.875,0.888888888888889,0.902777777777778,
0.916666666666667,0.930555555555556,0.944444444444444,0.958333333333333,
0.972222222222222,0.986111111111111,1.),.UNSPECIFIED.)
GEOMETRIC_REPRESENTATION_ITEM()
RATIONAL_B_SPLINE_SURFACE(((1.,0.965925826289068,1.,0.965925826289068,1.,
0.965925826289068,1.,0.965925826289068,1.,0.965925826289068,1.,0.965925826289068,
1.,0.965925826289068,1.,0.965925826289068,1.,0.965925826289068,1.,0.965925826289068,
1.,0.965925826289068,1.,0.965925826289068,1.,0.965925826289068,1.,0.965925826289068,
1.,0.965925826289068,1.,0.965925826289068,1.,0.965925826289068,1.,0.965925826289068,
1.,0.965925826289068,1.,0.965925826289068,1.,0.965925826289068,1.,0.965925826289068,
1.,0.965925826289068,1.,0.965925826289068,1.,0.965925826289068,1.,0.965925826289068,
1.,0.965925826289068,1.,0.965925826289068,1.,0.965925826289068,1.,0.965925826289068,
1.,0.965925826289068,1.,0.965925826289068,1.,0.965925826289068,1.,0.965925826289068,
1.,0.965925826289068,1.,0.965925826289068,1.,0.965925826289068,1.,0.965925826289068,
1.,0.965925826289068,1.,0.965925826289068,1.,0.965925826289068,1.,0.965925826289068,
1.,0.965925826289068,1.,0.965925826289068,1.,0.965925826289068,1.,0.965925826289068,
1.,0.965925826289068,1.,0.965925826289068,1.,0.965925826289068,1.,0.965925826289068,
1.,0.965925826289068,1.,0.965925826289068,1.,0.965925826289068,1.,0.965925826289068,
1.,0.965925826289068,1.,0.965925826289068,1.,0.965925826289068,1.,0.965925826289068,
1.,0.965925826289068,1.,0.965925826289068,1.,0.965925826289068,1.,0.965925826289068,
1.,0.965925826289068,1.,0.965925826289068,1.,0.965925826289068,1.,0.965925826289068,
1.,0.965925826289068,1.,0.965925826289068,1.,0.965925826289068,1.,0.965925826289068,
1.,0.965925826289068,1.,0.965925826289068,1.),(1.,0.965925826289068,1.,
0.965925826289068,1.,0.965925826289068,1.,0.965925826289068,1.,0.965925826289068,
1.,0.965925826289068,1.,0.965925826289068,1.,0.965925826289068,1.,0.965925826289068,
1.,0.965925826289068,1.,0.965925826289068,1.,0.965925826289068,1.,0.965925826289068,
1.,0.965925826289068,1.,0.965925826289068,1.,0.965925826289068,1.,0.965925826289068,
1.,0.965925826289068,1.,0.965925826289068,1.,0.965925826289068,1.,0.965925826289068,
1.,0.965925826289068,1.,0.965925826289068,1.,0.965925826289068,1.,0.965925826289068,
1.,0.965925826289068,1.,0.965925826289068,1.,0.965925826289068,1.,0.965925826289068,
1.,0.965925826289068,1.,0.965925826289068,1.,0.965925826289068,1.,0.965925826289068,
1.,0.965925826289068,1.,0.965925826289068,1.,0.965925826289068,1.,0.965925826289068,
1.,0.965925826289068,1.,0.965925826289068,1.,0.965925826289068,1.,0.965925826289068,
1.,0.965925826289068,1.,0.965925826289068,1.,0.965925826289068,1.,0.965925826289068,
1.,0.965925826289068,1.,0.965925826289068,1.,0.965925826289068,1.,0.965925826289068,
1.,0.965925826289068,1.,0.965925826289068,1.,0.965925826289068,1.,0.965925826289068,
1.,0.965925826289068,1.,0.965925826289068,1.,0.965925826289068,1.,0.965925826289068,
1.,0.965925826289068,1.,0.965925826289068,1.,0.965925826289068,1.,0.965925826289068,
1.,0.965925826289068,1.,0.965925826289068,1.,0.965925826289068,1.,0.965925826289068,
1.,0.965925826289068,1.,0.965925826289068,1.,0.965925826289068,1.,0.965925826289068,
1.,0.965925826289068,1.,0.965925826289068,1.,0.965925826289068,1.)))
REPRESENTATION_ITEM('')
SURFACE()
);
#192=(
BOUNDED_SURFACE()
B_SPLINE_SURFACE(1,2,((#18367,#18368,#18369,#18370,#18371,#18372,#18373,
#18374,#18375,#18376,#18377,#18378,#18379,#18380,#18381,#18382,#18383,#18384,
#18385,#18386,#18387,#18388,#18389,#18390,#18391,#18392,#18393,#18394,#18395,
#18396,#18397,#18398,#18399,#18400,#18401,#18402,#18403,#18404,#18405,#18406,
#18407,#18408,#18409,#18410,#18411,#18412,#18413,#18414,#18415,#18416,#18417,
#18418,#18419,#18420,#18421,#18422,#18423,#18424,#18425,#18426,#18427,#18428,
#18429,#18430,#18431,#18432,#18433,#18434,#18435,#18436,#18437,#18438,#18439,
#18440,#18441,#18442,#18443,#18444,#18445,#18446,#18447,#18448,#18449,#18450,
#18451,#18452,#18453,#18454,#18455,#18456,#18457,#18458,#18459,#18460,#18461,
#18462,#18463,#18464,#18465,#18466,#18467,#18468,#18469,#18470,#18471,#18472,
#18473,#18474,#18475,#18476,#18477,#18478,#18479,#18480,#18481,#18482,#18483,
#18484,#18485,#18486,#18487,#18488,#18489,#18490,#18491,#18492,#18493,#18494,
#18495,#18496,#18497,#18498,#18499,#18500,#18501,#18502,#18503,#18504,#18505,
#18506,#18507,#18508,#18509,#18510,#18511),(#18512,#18513,#18514,#18515,
#18516,#18517,#18518,#18519,#18520,#18521,#18522,#18523,#18524,#18525,#18526,
#18527,#18528,#18529,#18530,#18531,#18532,#18533,#18534,#18535,#18536,#18537,
#18538,#18539,#18540,#18541,#18542,#18543,#18544,#18545,#18546,#18547,#18548,
#18549,#18550,#18551,#18552,#18553,#18554,#18555,#18556,#18557,#18558,#18559,
#18560,#18561,#18562,#18563,#18564,#18565,#18566,#18567,#18568,#18569,#18570,
#18571,#18572,#18573,#18574,#18575,#18576,#18577,#18578,#18579,#18580,#18581,
#18582,#18583,#18584,#18585,#18586,#18587,#18588,#18589,#18590,#18591,#18592,
#18593,#18594,#18595,#18596,#18597,#18598,#18599,#18600,#18601,#18602,#18603,
#18604,#18605,#18606,#18607,#18608,#18609,#18610,#18611,#18612,#18613,#18614,
#18615,#18616,#18617,#18618,#18619,#18620,#18621,#18622,#18623,#18624,#18625,
#18626,#18627,#18628,#18629,#18630,#18631,#18632,#18633,#18634,#18635,#18636,
#18637,#18638,#18639,#18640,#18641,#18642,#18643,#18644,#18645,#18646,#18647,
#18648,#18649,#18650,#18651,#18652,#18653,#18654,#18655,#18656)),
 .UNSPECIFIED.,.F.,.F.,.F.)
B_SPLINE_SURFACE_WITH_KNOTS((2,2),(3,2,2,2,2,2,2,2,2,2,2,2,2,2,2,2,2,2,
2,2,2,2,2,2,2,2,2,2,2,2,2,2,2,2,2,2,2,2,2,2,2,2,2,2,2,2,2,2,2,2,2,2,2,2,
2,2,2,2,2,2,2,2,2,2,2,2,2,2,2,2,2,2,3),(0.,1.00000000985537),(0.,0.0138888888888889,
0.0277777777777778,0.0416666666666667,0.0555555555555556,0.0694444444444444,
0.0833333333333333,0.0972222222222222,0.111111111111111,0.125,0.138888888888889,
0.152777777777778,0.166666666666667,0.180555555555556,0.194444444444444,
0.208333333333333,0.222222222222222,0.236111111111111,0.25,0.263888888888889,
0.277777777777778,0.291666666666667,0.305555555555556,0.319444444444444,
0.333333333333333,0.347222222222222,0.361111111111111,0.375,0.388888888888889,
0.402777777777778,0.416666666666667,0.430555555555556,0.444444444444444,
0.458333333333333,0.472222222222222,0.486111111111111,0.5,0.513888888888889,
0.527777777777778,0.541666666666667,0.555555555555556,0.569444444444444,
0.583333333333333,0.597222222222222,0.611111111111111,0.625,0.638888888888889,
0.652777777777778,0.666666666666667,0.680555555555556,0.694444444444444,
0.708333333333333,0.722222222222222,0.736111111111111,0.75,0.763888888888889,
0.777777777777778,0.791666666666667,0.805555555555556,0.819444444444444,
0.833333333333333,0.847222222222222,0.861111111111111,0.875,0.888888888888889,
0.902777777777778,0.916666666666667,0.930555555555556,0.944444444444444,
0.958333333333333,0.972222222222222,0.986111111111111,1.),.UNSPECIFIED.)
GEOMETRIC_REPRESENTATION_ITEM()
RATIONAL_B_SPLINE_SURFACE(((1.,0.965925826289068,1.,0.965925826289068,1.,
0.965925826289068,1.,0.965925826289068,1.,0.965925826289068,1.,0.965925826289068,
1.,0.965925826289068,1.,0.965925826289068,1.,0.965925826289068,1.,0.965925826289068,
1.,0.965925826289068,1.,0.965925826289068,1.,0.965925826289068,1.,0.965925826289068,
1.,0.965925826289068,1.,0.965925826289068,1.,0.965925826289068,1.,0.965925826289068,
1.,0.965925826289068,1.,0.965925826289068,1.,0.965925826289068,1.,0.965925826289068,
1.,0.965925826289068,1.,0.965925826289068,1.,0.965925826289068,1.,0.965925826289068,
1.,0.965925826289068,1.,0.965925826289068,1.,0.965925826289068,1.,0.965925826289068,
1.,0.965925826289068,1.,0.965925826289068,1.,0.965925826289068,1.,0.965925826289068,
1.,0.965925826289068,1.,0.965925826289068,1.,0.965925826289068,1.,0.965925826289068,
1.,0.965925826289068,1.,0.965925826289068,1.,0.965925826289068,1.,0.965925826289068,
1.,0.965925826289068,1.,0.965925826289068,1.,0.965925826289068,1.,0.965925826289068,
1.,0.965925826289068,1.,0.965925826289068,1.,0.965925826289068,1.,0.965925826289068,
1.,0.965925826289068,1.,0.965925826289068,1.,0.965925826289068,1.,0.965925826289068,
1.,0.965925826289068,1.,0.965925826289068,1.,0.965925826289068,1.,0.965925826289068,
1.,0.965925826289068,1.,0.965925826289068,1.,0.965925826289068,1.,0.965925826289068,
1.,0.965925826289068,1.,0.965925826289068,1.,0.965925826289068,1.,0.965925826289068,
1.,0.965925826289068,1.,0.965925826289068,1.,0.965925826289068,1.,0.965925826289068,
1.,0.965925826289068,1.,0.965925826289068,1.),(1.,0.965925826289068,1.,
0.965925826289068,1.,0.965925826289068,1.,0.965925826289068,1.,0.965925826289068,
1.,0.965925826289068,1.,0.965925826289068,1.,0.965925826289068,1.,0.965925826289068,
1.,0.965925826289068,1.,0.965925826289068,1.,0.965925826289068,1.,0.965925826289068,
1.,0.965925826289068,1.,0.965925826289068,1.,0.965925826289068,1.,0.965925826289068,
1.,0.965925826289068,1.,0.965925826289068,1.,0.965925826289068,1.,0.965925826289068,
1.,0.965925826289068,1.,0.965925826289068,1.,0.965925826289068,1.,0.965925826289068,
1.,0.965925826289068,1.,0.965925826289068,1.,0.965925826289068,1.,0.965925826289068,
1.,0.965925826289068,1.,0.965925826289068,1.,0.965925826289068,1.,0.965925826289068,
1.,0.965925826289068,1.,0.965925826289068,1.,0.965925826289068,1.,0.965925826289068,
1.,0.965925826289068,1.,0.965925826289068,1.,0.965925826289068,1.,0.965925826289068,
1.,0.965925826289068,1.,0.965925826289068,1.,0.965925826289068,1.,0.965925826289068,
1.,0.965925826289068,1.,0.965925826289068,1.,0.965925826289068,1.,0.965925826289068,
1.,0.965925826289068,1.,0.965925826289068,1.,0.965925826289068,1.,0.965925826289068,
1.,0.965925826289068,1.,0.965925826289068,1.,0.965925826289068,1.,0.965925826289068,
1.,0.965925826289068,1.,0.965925826289068,1.,0.965925826289068,1.,0.965925826289068,
1.,0.965925826289068,1.,0.965925826289068,1.,0.965925826289068,1.,0.965925826289068,
1.,0.965925826289068,1.,0.965925826289068,1.,0.965925826289068,1.,0.965925826289068,
1.,0.965925826289068,1.,0.965925826289068,1.,0.965925826289068,1.)))
REPRESENTATION_ITEM('')
SURFACE()
);
#193=(
BOUNDED_SURFACE()
B_SPLINE_SURFACE(1,2,((#18703,#18704,#18705,#18706,#18707,#18708,#18709,
#18710,#18711,#18712,#18713,#18714,#18715,#18716,#18717,#18718,#18719,#18720,
#18721,#18722,#18723,#18724,#18725,#18726,#18727,#18728,#18729,#18730,#18731,
#18732,#18733,#18734,#18735,#18736,#18737,#18738,#18739,#18740,#18741,#18742,
#18743,#18744,#18745,#18746,#18747,#18748,#18749,#18750,#18751,#18752,#18753,
#18754,#18755,#18756,#18757,#18758,#18759,#18760,#18761,#18762,#18763,#18764,
#18765,#18766,#18767,#18768,#18769,#18770,#18771,#18772,#18773,#18774,#18775,
#18776,#18777,#18778,#18779,#18780,#18781,#18782,#18783,#18784,#18785,#18786,
#18787,#18788,#18789,#18790,#18791,#18792,#18793,#18794,#18795,#18796,#18797,
#18798,#18799,#18800,#18801,#18802,#18803,#18804,#18805,#18806,#18807,#18808,
#18809,#18810,#18811,#18812,#18813,#18814,#18815,#18816,#18817,#18818,#18819,
#18820,#18821,#18822,#18823,#18824,#18825,#18826,#18827,#18828,#18829,#18830,
#18831,#18832,#18833,#18834,#18835,#18836,#18837,#18838,#18839,#18840,#18841,
#18842,#18843,#18844,#18845,#18846,#18847),(#18848,#18849,#18850,#18851,
#18852,#18853,#18854,#18855,#18856,#18857,#18858,#18859,#18860,#18861,#18862,
#18863,#18864,#18865,#18866,#18867,#18868,#18869,#18870,#18871,#18872,#18873,
#18874,#18875,#18876,#18877,#18878,#18879,#18880,#18881,#18882,#18883,#18884,
#18885,#18886,#18887,#18888,#18889,#18890,#18891,#18892,#18893,#18894,#18895,
#18896,#18897,#18898,#18899,#18900,#18901,#18902,#18903,#18904,#18905,#18906,
#18907,#18908,#18909,#18910,#18911,#18912,#18913,#18914,#18915,#18916,#18917,
#18918,#18919,#18920,#18921,#18922,#18923,#18924,#18925,#18926,#18927,#18928,
#18929,#18930,#18931,#18932,#18933,#18934,#18935,#18936,#18937,#18938,#18939,
#18940,#18941,#18942,#18943,#18944,#18945,#18946,#18947,#18948,#18949,#18950,
#18951,#18952,#18953,#18954,#18955,#18956,#18957,#18958,#18959,#18960,#18961,
#18962,#18963,#18964,#18965,#18966,#18967,#18968,#18969,#18970,#18971,#18972,
#18973,#18974,#18975,#18976,#18977,#18978,#18979,#18980,#18981,#18982,#18983,
#18984,#18985,#18986,#18987,#18988,#18989,#18990,#18991,#18992)),
 .UNSPECIFIED.,.F.,.F.,.F.)
B_SPLINE_SURFACE_WITH_KNOTS((2,2),(3,2,2,2,2,2,2,2,2,2,2,2,2,2,2,2,2,2,
2,2,2,2,2,2,2,2,2,2,2,2,2,2,2,2,2,2,2,2,2,2,2,2,2,2,2,2,2,2,2,2,2,2,2,2,
2,2,2,2,2,2,2,2,2,2,2,2,2,2,2,2,2,2,3),(0.,1.),(0.,0.0138888888888889,0.0277777777777778,
0.0416666666666667,0.0555555555555556,0.0694444444444444,0.0833333333333333,
0.0972222222222222,0.111111111111111,0.125,0.138888888888889,0.152777777777778,
0.166666666666667,0.180555555555556,0.194444444444444,0.208333333333333,
0.222222222222222,0.236111111111111,0.25,0.263888888888889,0.277777777777778,
0.291666666666667,0.305555555555556,0.319444444444444,0.333333333333333,
0.347222222222222,0.361111111111111,0.375,0.388888888888889,0.402777777777778,
0.416666666666667,0.430555555555556,0.444444444444444,0.458333333333333,
0.472222222222222,0.486111111111111,0.5,0.513888888888889,0.527777777777778,
0.541666666666667,0.555555555555556,0.569444444444444,0.583333333333333,
0.597222222222222,0.611111111111111,0.625,0.638888888888889,0.652777777777778,
0.666666666666667,0.680555555555556,0.694444444444444,0.708333333333333,
0.722222222222222,0.736111111111111,0.75,0.763888888888889,0.777777777777778,
0.791666666666667,0.805555555555556,0.819444444444444,0.833333333333333,
0.847222222222222,0.861111111111111,0.875,0.888888888888889,0.902777777777778,
0.916666666666667,0.930555555555556,0.944444444444444,0.958333333333333,
0.972222222222222,0.986111111111111,1.),.UNSPECIFIED.)
GEOMETRIC_REPRESENTATION_ITEM()
RATIONAL_B_SPLINE_SURFACE(((1.,0.965925826289068,1.,0.965925826289068,1.,
0.965925826289068,1.,0.965925826289068,1.,0.965925826289068,1.,0.965925826289068,
1.,0.965925826289068,1.,0.965925826289068,1.,0.965925826289068,1.,0.965925826289068,
1.,0.965925826289068,1.,0.965925826289068,1.,0.965925826289068,1.,0.965925826289068,
1.,0.965925826289068,1.,0.965925826289068,1.,0.965925826289068,1.,0.965925826289068,
1.,0.965925826289068,1.,0.965925826289068,1.,0.965925826289068,1.,0.965925826289068,
1.,0.965925826289068,1.,0.965925826289068,1.,0.965925826289068,1.,0.965925826289068,
1.,0.965925826289068,1.,0.965925826289068,1.,0.965925826289068,1.,0.965925826289068,
1.,0.965925826289068,1.,0.965925826289068,1.,0.965925826289068,1.,0.965925826289068,
1.,0.965925826289068,1.,0.965925826289068,1.,0.965925826289068,1.,0.965925826289068,
1.,0.965925826289068,1.,0.965925826289068,1.,0.965925826289068,1.,0.965925826289068,
1.,0.965925826289068,1.,0.965925826289068,1.,0.965925826289068,1.,0.965925826289068,
1.,0.965925826289068,1.,0.965925826289068,1.,0.965925826289068,1.,0.965925826289068,
1.,0.965925826289068,1.,0.965925826289068,1.,0.965925826289068,1.,0.965925826289068,
1.,0.965925826289068,1.,0.965925826289068,1.,0.965925826289068,1.,0.965925826289068,
1.,0.965925826289068,1.,0.965925826289068,1.,0.965925826289068,1.,0.965925826289068,
1.,0.965925826289068,1.,0.965925826289068,1.,0.965925826289068,1.,0.965925826289068,
1.,0.965925826289068,1.,0.965925826289068,1.,0.965925826289068,1.,0.965925826289068,
1.,0.965925826289068,1.,0.965925826289068,1.),(1.,0.965925826289068,1.,
0.965925826289068,1.,0.965925826289068,1.,0.965925826289068,1.,0.965925826289068,
1.,0.965925826289068,1.,0.965925826289068,1.,0.965925826289068,1.,0.965925826289068,
1.,0.965925826289068,1.,0.965925826289068,1.,0.965925826289068,1.,0.965925826289068,
1.,0.965925826289068,1.,0.965925826289068,1.,0.965925826289068,1.,0.965925826289068,
1.,0.965925826289068,1.,0.965925826289068,1.,0.965925826289068,1.,0.965925826289068,
1.,0.965925826289068,1.,0.965925826289068,1.,0.965925826289068,1.,0.965925826289068,
1.,0.965925826289068,1.,0.965925826289068,1.,0.965925826289068,1.,0.965925826289068,
1.,0.965925826289068,1.,0.965925826289068,1.,0.965925826289068,1.,0.965925826289068,
1.,0.965925826289068,1.,0.965925826289068,1.,0.965925826289068,1.,0.965925826289068,
1.,0.965925826289068,1.,0.965925826289068,1.,0.965925826289068,1.,0.965925826289068,
1.,0.965925826289068,1.,0.965925826289068,1.,0.965925826289068,1.,0.965925826289068,
1.,0.965925826289068,1.,0.965925826289068,1.,0.965925826289068,1.,0.965925826289068,
1.,0.965925826289068,1.,0.965925826289068,1.,0.965925826289068,1.,0.965925826289068,
1.,0.965925826289068,1.,0.965925826289068,1.,0.965925826289068,1.,0.965925826289068,
1.,0.965925826289068,1.,0.965925826289068,1.,0.965925826289068,1.,0.965925826289068,
1.,0.965925826289068,1.,0.965925826289068,1.,0.965925826289068,1.,0.965925826289068,
1.,0.965925826289068,1.,0.965925826289068,1.,0.965925826289068,1.,0.965925826289068,
1.,0.965925826289068,1.,0.965925826289068,1.,0.965925826289068,1.)))
REPRESENTATION_ITEM('')
SURFACE()
);
#194=(
BOUNDED_SURFACE()
B_SPLINE_SURFACE(1,2,((#19006,#19007,#19008,#19009,#19010,#19011,#19012,
#19013,#19014,#19015,#19016,#19017,#19018,#19019,#19020,#19021,#19022,#19023,
#19024,#19025,#19026,#19027,#19028,#19029,#19030,#19031,#19032,#19033,#19034,
#19035,#19036,#19037,#19038,#19039,#19040,#19041,#19042,#19043,#19044,#19045,
#19046,#19047,#19048,#19049,#19050,#19051,#19052,#19053,#19054,#19055,#19056,
#19057,#19058,#19059,#19060,#19061,#19062,#19063,#19064,#19065,#19066,#19067,
#19068,#19069,#19070,#19071,#19072,#19073,#19074,#19075,#19076,#19077,#19078,
#19079,#19080,#19081,#19082,#19083,#19084,#19085,#19086,#19087,#19088,#19089,
#19090,#19091,#19092,#19093,#19094,#19095,#19096,#19097,#19098,#19099,#19100,
#19101,#19102,#19103,#19104,#19105,#19106,#19107,#19108,#19109,#19110,#19111,
#19112,#19113,#19114,#19115,#19116,#19117,#19118,#19119,#19120,#19121,#19122,
#19123,#19124,#19125,#19126,#19127,#19128,#19129,#19130,#19131,#19132,#19133,
#19134,#19135,#19136,#19137,#19138,#19139,#19140,#19141,#19142,#19143,#19144,
#19145,#19146,#19147,#19148,#19149,#19150),(#19151,#19152,#19153,#19154,
#19155,#19156,#19157,#19158,#19159,#19160,#19161,#19162,#19163,#19164,#19165,
#19166,#19167,#19168,#19169,#19170,#19171,#19172,#19173,#19174,#19175,#19176,
#19177,#19178,#19179,#19180,#19181,#19182,#19183,#19184,#19185,#19186,#19187,
#19188,#19189,#19190,#19191,#19192,#19193,#19194,#19195,#19196,#19197,#19198,
#19199,#19200,#19201,#19202,#19203,#19204,#19205,#19206,#19207,#19208,#19209,
#19210,#19211,#19212,#19213,#19214,#19215,#19216,#19217,#19218,#19219,#19220,
#19221,#19222,#19223,#19224,#19225,#19226,#19227,#19228,#19229,#19230,#19231,
#19232,#19233,#19234,#19235,#19236,#19237,#19238,#19239,#19240,#19241,#19242,
#19243,#19244,#19245,#19246,#19247,#19248,#19249,#19250,#19251,#19252,#19253,
#19254,#19255,#19256,#19257,#19258,#19259,#19260,#19261,#19262,#19263,#19264,
#19265,#19266,#19267,#19268,#19269,#19270,#19271,#19272,#19273,#19274,#19275,
#19276,#19277,#19278,#19279,#19280,#19281,#19282,#19283,#19284,#19285,#19286,
#19287,#19288,#19289,#19290,#19291,#19292,#19293,#19294,#19295)),
 .UNSPECIFIED.,.F.,.F.,.F.)
B_SPLINE_SURFACE_WITH_KNOTS((2,2),(3,2,2,2,2,2,2,2,2,2,2,2,2,2,2,2,2,2,
2,2,2,2,2,2,2,2,2,2,2,2,2,2,2,2,2,2,2,2,2,2,2,2,2,2,2,2,2,2,2,2,2,2,2,2,
2,2,2,2,2,2,2,2,2,2,2,2,2,2,2,2,2,2,3),(0.,1.),(0.,0.0138888888888889,0.0277777777777778,
0.0416666666666667,0.0555555555555556,0.0694444444444444,0.0833333333333333,
0.0972222222222222,0.111111111111111,0.125,0.138888888888889,0.152777777777778,
0.166666666666667,0.180555555555556,0.194444444444444,0.208333333333333,
0.222222222222222,0.236111111111111,0.25,0.263888888888889,0.277777777777778,
0.291666666666667,0.305555555555556,0.319444444444444,0.333333333333333,
0.347222222222222,0.361111111111111,0.375,0.388888888888889,0.402777777777778,
0.416666666666667,0.430555555555556,0.444444444444444,0.458333333333333,
0.472222222222222,0.486111111111111,0.5,0.513888888888889,0.527777777777778,
0.541666666666667,0.555555555555556,0.569444444444444,0.583333333333333,
0.597222222222222,0.611111111111111,0.625,0.638888888888889,0.652777777777778,
0.666666666666667,0.680555555555556,0.694444444444444,0.708333333333333,
0.722222222222222,0.736111111111111,0.75,0.763888888888889,0.777777777777778,
0.791666666666667,0.805555555555556,0.819444444444444,0.833333333333333,
0.847222222222222,0.861111111111111,0.875,0.888888888888889,0.902777777777778,
0.916666666666667,0.930555555555556,0.944444444444444,0.958333333333333,
0.972222222222222,0.986111111111111,1.),.UNSPECIFIED.)
GEOMETRIC_REPRESENTATION_ITEM()
RATIONAL_B_SPLINE_SURFACE(((1.,0.965925826289068,1.,0.965925826289068,1.,
0.965925826289068,1.,0.965925826289068,1.,0.965925826289068,1.,0.965925826289068,
1.,0.965925826289068,1.,0.965925826289068,1.,0.965925826289068,1.,0.965925826289068,
1.,0.965925826289068,1.,0.965925826289068,1.,0.965925826289068,1.,0.965925826289068,
1.,0.965925826289068,1.,0.965925826289068,1.,0.965925826289068,1.,0.965925826289068,
1.,0.965925826289068,1.,0.965925826289068,1.,0.965925826289068,1.,0.965925826289068,
1.,0.965925826289068,1.,0.965925826289068,1.,0.965925826289068,1.,0.965925826289068,
1.,0.965925826289068,1.,0.965925826289068,1.,0.965925826289068,1.,0.965925826289068,
1.,0.965925826289068,1.,0.965925826289068,1.,0.965925826289068,1.,0.965925826289068,
1.,0.965925826289068,1.,0.965925826289068,1.,0.965925826289068,1.,0.965925826289068,
1.,0.965925826289068,1.,0.965925826289068,1.,0.965925826289068,1.,0.965925826289068,
1.,0.965925826289068,1.,0.965925826289068,1.,0.965925826289068,1.,0.965925826289068,
1.,0.965925826289068,1.,0.965925826289068,1.,0.965925826289068,1.,0.965925826289068,
1.,0.965925826289068,1.,0.965925826289068,1.,0.965925826289068,1.,0.965925826289068,
1.,0.965925826289068,1.,0.965925826289068,1.,0.965925826289068,1.,0.965925826289068,
1.,0.965925826289068,1.,0.965925826289068,1.,0.965925826289068,1.,0.965925826289068,
1.,0.965925826289068,1.,0.965925826289068,1.,0.965925826289068,1.,0.965925826289068,
1.,0.965925826289068,1.,0.965925826289068,1.,0.965925826289068,1.,0.965925826289068,
1.,0.965925826289068,1.,0.965925826289068,1.),(1.,0.965925826289068,1.,
0.965925826289068,1.,0.965925826289068,1.,0.965925826289068,1.,0.965925826289068,
1.,0.965925826289068,1.,0.965925826289068,1.,0.965925826289068,1.,0.965925826289068,
1.,0.965925826289068,1.,0.965925826289068,1.,0.965925826289068,1.,0.965925826289068,
1.,0.965925826289068,1.,0.965925826289068,1.,0.965925826289068,1.,0.965925826289068,
1.,0.965925826289068,1.,0.965925826289068,1.,0.965925826289068,1.,0.965925826289068,
1.,0.965925826289068,1.,0.965925826289068,1.,0.965925826289068,1.,0.965925826289068,
1.,0.965925826289068,1.,0.965925826289068,1.,0.965925826289068,1.,0.965925826289068,
1.,0.965925826289068,1.,0.965925826289068,1.,0.965925826289068,1.,0.965925826289068,
1.,0.965925826289068,1.,0.965925826289068,1.,0.965925826289068,1.,0.965925826289068,
1.,0.965925826289068,1.,0.965925826289068,1.,0.965925826289068,1.,0.965925826289068,
1.,0.965925826289068,1.,0.965925826289068,1.,0.965925826289068,1.,0.965925826289068,
1.,0.965925826289068,1.,0.965925826289068,1.,0.965925826289068,1.,0.965925826289068,
1.,0.965925826289068,1.,0.965925826289068,1.,0.965925826289068,1.,0.965925826289068,
1.,0.965925826289068,1.,0.965925826289068,1.,0.965925826289068,1.,0.965925826289068,
1.,0.965925826289068,1.,0.965925826289068,1.,0.965925826289068,1.,0.965925826289068,
1.,0.965925826289068,1.,0.965925826289068,1.,0.965925826289068,1.,0.965925826289068,
1.,0.965925826289068,1.,0.965925826289068,1.,0.965925826289068,1.,0.965925826289068,
1.,0.965925826289068,1.,0.965925826289068,1.,0.965925826289068,1.)))
REPRESENTATION_ITEM('')
SURFACE()
);
#197=(
BOUNDED_CURVE()
B_SPLINE_CURVE(2,(#5212,#5213,#5214,#5215,#5216,#5217,#5218),
 .UNSPECIFIED.,.F.,.F.)
B_SPLINE_CURVE_WITH_KNOTS((3,2,2,3),(0.710433099667006,0.722222222222222,
0.736111111111111,0.747484081398396),.UNSPECIFIED.)
CURVE()
GEOMETRIC_REPRESENTATION_ITEM()
RATIONAL_B_SPLINE_CURVE((0.991254739061418,0.971077268091095,1.,0.965925826289068,
1.,0.97209823130717,0.989891404642439))
REPRESENTATION_ITEM('')
);
#198=(
BOUNDED_CURVE()
B_SPLINE_CURVE(2,(#5221,#5222,#5223,#5224,#5225,#5226,#5227),
 .UNSPECIFIED.,.F.,.F.)
B_SPLINE_CURVE_WITH_KNOTS((3,2,2,3),(0.543766433000339,0.555555555555556,
0.569444444444444,0.580817414731729),.UNSPECIFIED.)
CURVE()
GEOMETRIC_REPRESENTATION_ITEM()
RATIONAL_B_SPLINE_CURVE((0.991254739061418,0.971077268091095,1.,0.965925826289068,
1.,0.97209823130717,0.989891404642439))
REPRESENTATION_ITEM('')
);
#199=(
BOUNDED_CURVE()
B_SPLINE_CURVE(2,(#5233,#5234,#5235,#5236,#5237,#5238,#5239),
 .UNSPECIFIED.,.F.,.F.)
B_SPLINE_CURVE_WITH_KNOTS((3,2,2,3),(0.585429670084067,0.597222222222222,
0.611111111111111,0.622900233666328),.UNSPECIFIED.)
CURVE()
GEOMETRIC_REPRESENTATION_ITEM()
RATIONAL_B_SPLINE_CURVE((0.991266482904706,0.971068854156347,1.,0.965925826289068,
1.,0.971077268091093,0.99125473906142))
REPRESENTATION_ITEM('')
);
#200=(
BOUNDED_CURVE()
B_SPLINE_CURVE(2,(#5245,#5246,#5247,#5248,#5249,#5250,#5251),
 .UNSPECIFIED.,.F.,.F.)
B_SPLINE_CURVE_WITH_KNOTS((3,2,2,3),(0.752096336750733,0.763888888888889,
0.777777777777778,0.78959636025962),.UNSPECIFIED.)
CURVE()
GEOMETRIC_REPRESENTATION_ITEM()
RATIONAL_B_SPLINE_CURVE((0.991266482904706,0.971068854156347,1.,0.965925826289068,
1.,0.971004992859764,0.991355888936111))
REPRESENTATION_ITEM('')
);
#201=(
BOUNDED_CURVE()
B_SPLINE_CURVE(2,(#5257,#5258,#5259,#5260,#5261,#5262,#5263),
 .UNSPECIFIED.,.F.,.F.)
B_SPLINE_CURVE_WITH_KNOTS((3,2,2,3),(0.210433099667006,0.222222222222222,
0.236111111111111,0.247484081398396),.UNSPECIFIED.)
CURVE()
GEOMETRIC_REPRESENTATION_ITEM()
RATIONAL_B_SPLINE_CURVE((0.991254739061418,0.971077268091095,1.,0.965925826289068,
1.,0.97209823130717,0.989891404642439))
REPRESENTATION_ITEM('')
);
#202=(
BOUNDED_CURVE()
B_SPLINE_CURVE(2,(#5266,#5267,#5268,#5269,#5270,#5271,#5272),
 .UNSPECIFIED.,.F.,.F.)
B_SPLINE_CURVE_WITH_KNOTS((3,2,2,3),(0.0437664330003391,0.0555555555555556,
0.0694444444444444,0.080817414731729),.UNSPECIFIED.)
CURVE()
GEOMETRIC_REPRESENTATION_ITEM()
RATIONAL_B_SPLINE_CURVE((0.991254739061418,0.971077268091094,1.,0.965925826289068,
1.,0.97209823130717,0.989891404642439))
REPRESENTATION_ITEM('')
);
#203=(
BOUNDED_CURVE()
B_SPLINE_CURVE(2,(#5278,#5279,#5280,#5281,#5282,#5283,#5284),
 .UNSPECIFIED.,.F.,.F.)
B_SPLINE_CURVE_WITH_KNOTS((3,2,2,3),(0.0854296700840668,0.0972222222222222,
0.111111111111111,0.122900233666328),.UNSPECIFIED.)
CURVE()
GEOMETRIC_REPRESENTATION_ITEM()
RATIONAL_B_SPLINE_CURVE((0.991266482904706,0.971068854156348,1.,0.965925826289068,
1.,0.971077268091095,0.991254739061418))
REPRESENTATION_ITEM('')
);
#204=(
BOUNDED_CURVE()
B_SPLINE_CURVE(2,(#5287,#5288,#5289,#5290,#5291,#5292,#5293),
 .UNSPECIFIED.,.F.,.F.)
B_SPLINE_CURVE_WITH_KNOTS((3,2,2,3),(0.252096336750733,0.263888888888889,
0.277777777777778,0.289566900332994),.UNSPECIFIED.)
CURVE()
GEOMETRIC_REPRESENTATION_ITEM()
RATIONAL_B_SPLINE_CURVE((0.991266482904706,0.971068854156347,1.,0.965925826289068,
1.,0.971077268091095,0.991254739061418))
REPRESENTATION_ITEM('')
);
#205=(
BOUNDED_CURVE()
B_SPLINE_CURVE(2,(#5299,#5300,#5301,#5302,#5303,#5304,#5305),
 .UNSPECIFIED.,.F.,.F.)
B_SPLINE_CURVE_WITH_KNOTS((3,2,2,3),(0.377099766333672,0.388888888888889,
0.402777777777778,0.414150748065062),.UNSPECIFIED.)
CURVE()
GEOMETRIC_REPRESENTATION_ITEM()
RATIONAL_B_SPLINE_CURVE((0.991254739061418,0.971077268091095,1.,0.965925826289068,
1.,0.97209823130717,0.989891404642439))
REPRESENTATION_ITEM('')
);
#206=(
BOUNDED_CURVE()
B_SPLINE_CURVE(2,(#5308,#5309,#5310,#5311,#5312,#5313,#5314),
 .UNSPECIFIED.,.F.,.F.)
B_SPLINE_CURVE_WITH_KNOTS((3,2,2,3),(0.210433099667006,0.222222222222222,
0.236111111111111,0.247484081398396),.UNSPECIFIED.)
CURVE()
GEOMETRIC_REPRESENTATION_ITEM()
RATIONAL_B_SPLINE_CURVE((0.991254739061418,0.971077268091095,1.,0.965925826289068,
1.,0.97209823130717,0.989891404642439))
REPRESENTATION_ITEM('')
);
#207=(
BOUNDED_CURVE()
B_SPLINE_CURVE(2,(#5320,#5321,#5322,#5323,#5324,#5325,#5326),
 .UNSPECIFIED.,.F.,.F.)
B_SPLINE_CURVE_WITH_KNOTS((3,2,2,3),(0.252096336750733,0.263888888888889,
0.277777777777778,0.289566900332994),.UNSPECIFIED.)
CURVE()
GEOMETRIC_REPRESENTATION_ITEM()
RATIONAL_B_SPLINE_CURVE((0.991266482904706,0.971068854156347,1.,0.965925826289068,
1.,0.971077268091095,0.991254739061418))
REPRESENTATION_ITEM('')
);
#208=(
BOUNDED_CURVE()
B_SPLINE_CURVE(2,(#5329,#5330,#5331,#5332,#5333,#5334,#5335),
 .UNSPECIFIED.,.F.,.F.)
B_SPLINE_CURVE_WITH_KNOTS((3,2,2,3),(0.4187630034174,0.430555555555556,
0.444444444444444,0.456233566999661),.UNSPECIFIED.)
CURVE()
GEOMETRIC_REPRESENTATION_ITEM()
RATIONAL_B_SPLINE_CURVE((0.991266482904706,0.971068854156347,1.,0.965925826289068,
1.,0.971077268091095,0.991254739061418))
REPRESENTATION_ITEM('')
);
#209=(
BOUNDED_CURVE()
B_SPLINE_CURVE(2,(#5341,#5342,#5343,#5344,#5345,#5346,#5347),
 .UNSPECIFIED.,.F.,.F.)
B_SPLINE_CURVE_WITH_KNOTS((3,2,2,3),(0.543766433000339,0.555555555555556,
0.569444444444444,0.580817414731729),.UNSPECIFIED.)
CURVE()
GEOMETRIC_REPRESENTATION_ITEM()
RATIONAL_B_SPLINE_CURVE((0.991254739061418,0.971077268091094,1.,0.965925826289068,
1.,0.97209823130717,0.989891404642439))
REPRESENTATION_ITEM('')
);
#210=(
BOUNDED_CURVE()
B_SPLINE_CURVE(2,(#5350,#5351,#5352,#5353,#5354,#5355,#5356),
 .UNSPECIFIED.,.F.,.F.)
B_SPLINE_CURVE_WITH_KNOTS((3,2,2,3),(0.377099766333672,0.388888888888889,
0.402777777777778,0.414150748065062),.UNSPECIFIED.)
CURVE()
GEOMETRIC_REPRESENTATION_ITEM()
RATIONAL_B_SPLINE_CURVE((0.991254739061418,0.971077268091095,1.,0.965925826289068,
1.,0.97209823130717,0.989891404642439))
REPRESENTATION_ITEM('')
);
#211=(
BOUNDED_CURVE()
B_SPLINE_CURVE(2,(#5362,#5363,#5364,#5365,#5366,#5367,#5368),
 .UNSPECIFIED.,.F.,.F.)
B_SPLINE_CURVE_WITH_KNOTS((3,2,2,3),(0.4187630034174,0.430555555555556,
0.444444444444444,0.456233566999661),.UNSPECIFIED.)
CURVE()
GEOMETRIC_REPRESENTATION_ITEM()
RATIONAL_B_SPLINE_CURVE((0.991266482904706,0.971068854156347,1.,0.965925826289068,
1.,0.971077268091095,0.991254739061418))
REPRESENTATION_ITEM('')
);
#212=(
BOUNDED_CURVE()
B_SPLINE_CURVE(2,(#5371,#5372,#5373,#5374,#5375,#5376,#5377),
 .UNSPECIFIED.,.F.,.F.)
B_SPLINE_CURVE_WITH_KNOTS((3,2,2,3),(0.585429670084067,0.597222222222222,
0.611111111111111,0.622900233666328),.UNSPECIFIED.)
CURVE()
GEOMETRIC_REPRESENTATION_ITEM()
RATIONAL_B_SPLINE_CURVE((0.991266482904706,0.971068854156347,1.,0.965925826289068,
1.,0.971077268091095,0.991254739061418))
REPRESENTATION_ITEM('')
);
#213=(
BOUNDED_CURVE()
B_SPLINE_CURVE(2,(#5383,#5384,#5385,#5386,#5387,#5388,#5389),
 .UNSPECIFIED.,.F.,.F.)
B_SPLINE_CURVE_WITH_KNOTS((3,2,2,3),(0.00251591860160435,0.0138888888888889,
0.0277777777777778,0.039154184928472),.UNSPECIFIED.)
CURVE()
GEOMETRIC_REPRESENTATION_ITEM()
RATIONAL_B_SPLINE_CURVE((0.989891404642439,0.97209823130717,1.,0.965925826289068,
1.,0.972089799510949,0.989902162858515))
REPRESENTATION_ITEM('')
);
#214=(
BOUNDED_CURVE()
B_SPLINE_CURVE(2,(#5392,#5393,#5394,#5395,#5396,#5397,#5398),
 .UNSPECIFIED.,.F.,.F.)
B_SPLINE_CURVE_WITH_KNOTS((3,2,2,3),(0.169182585268271,0.180555555555556,
0.194444444444444,0.205820851595139),.UNSPECIFIED.)
CURVE()
GEOMETRIC_REPRESENTATION_ITEM()
RATIONAL_B_SPLINE_CURVE((0.989891404642439,0.97209823130717,1.,0.965925826289068,
1.,0.972089799510949,0.989902162858515))
REPRESENTATION_ITEM('')
);
#215=(
BOUNDED_CURVE()
B_SPLINE_CURVE(2,(#5404,#5405,#5406,#5407,#5408,#5409,#5410),
 .UNSPECIFIED.,.F.,.F.)
B_SPLINE_CURVE_WITH_KNOTS((3,2,2,3),(0.127512481738195,0.138888888888889,
0.152777777777778,0.164570329915933),.UNSPECIFIED.)
CURVE()
GEOMETRIC_REPRESENTATION_ITEM()
RATIONAL_B_SPLINE_CURVE((0.989902162858515,0.972089799510949,1.,0.965925826289068,
1.,0.971068854156348,0.991266482904706))
REPRESENTATION_ITEM('')
);
#216=(
BOUNDED_CURVE()
B_SPLINE_CURVE(2,(#5419,#5420,#5421,#5422,#5423,#5424,#5425),
 .UNSPECIFIED.,.F.,.F.)
B_SPLINE_CURVE_WITH_KNOTS((3,2,2,3),(0.169182585268271,0.180555555555556,
0.194444444444444,0.205820851595139),.UNSPECIFIED.)
CURVE()
GEOMETRIC_REPRESENTATION_ITEM()
RATIONAL_B_SPLINE_CURVE((0.989891404642439,0.97209823130717,1.,0.965925826289068,
1.,0.972089799510949,0.989902162858515))
REPRESENTATION_ITEM('')
);
#217=(
BOUNDED_CURVE()
B_SPLINE_CURVE(2,(#5428,#5429,#5430,#5431,#5432,#5433,#5434),
 .UNSPECIFIED.,.F.,.F.)
B_SPLINE_CURVE_WITH_KNOTS((3,2,2,3),(0.335849251934938,0.347222222222222,
0.361111111111111,0.372487518261805),.UNSPECIFIED.)
CURVE()
GEOMETRIC_REPRESENTATION_ITEM()
RATIONAL_B_SPLINE_CURVE((0.989891404642439,0.97209823130717,1.,0.965925826289068,
1.,0.972089799510949,0.989902162858515))
REPRESENTATION_ITEM('')
);
#218=(
BOUNDED_CURVE()
B_SPLINE_CURVE(2,(#5440,#5441,#5442,#5443,#5444,#5445,#5446),
 .UNSPECIFIED.,.F.,.F.)
B_SPLINE_CURVE_WITH_KNOTS((3,2,2,3),(0.294179148404861,0.305555555555556,
0.319444444444444,0.3312369965826),.UNSPECIFIED.)
CURVE()
GEOMETRIC_REPRESENTATION_ITEM()
RATIONAL_B_SPLINE_CURVE((0.989902162858515,0.972089799510949,1.,0.965925826289068,
1.,0.971068854156348,0.991266482904706))
REPRESENTATION_ITEM('')
);
#219=(
BOUNDED_CURVE()
B_SPLINE_CURVE(2,(#5449,#5450,#5451,#5452,#5453,#5454,#5455),
 .UNSPECIFIED.,.F.,.F.)
B_SPLINE_CURVE_WITH_KNOTS((3,2,2,3),(0.127512481738195,0.138888888888889,
0.152777777777778,0.164570329915933),.UNSPECIFIED.)
CURVE()
GEOMETRIC_REPRESENTATION_ITEM()
RATIONAL_B_SPLINE_CURVE((0.989902162858515,0.972089799510949,1.,0.965925826289068,
1.,0.971068854156348,0.991266482904706))
REPRESENTATION_ITEM('')
);
#220=(
BOUNDED_CURVE()
B_SPLINE_CURVE(2,(#5461,#5462,#5463,#5464,#5465,#5466,#5467),
 .UNSPECIFIED.,.F.,.F.)
B_SPLINE_CURVE_WITH_KNOTS((3,2,2,3),(0.335849251934938,0.347222222222222,
0.361111111111111,0.372487518261805),.UNSPECIFIED.)
CURVE()
GEOMETRIC_REPRESENTATION_ITEM()
RATIONAL_B_SPLINE_CURVE((0.989891404642439,0.97209823130717,1.,0.965925826289068,
1.,0.972089799510949,0.989902162858515))
REPRESENTATION_ITEM('')
);
#221=(
BOUNDED_CURVE()
B_SPLINE_CURVE(2,(#5470,#5471,#5472,#5473,#5474,#5475,#5476),
 .UNSPECIFIED.,.F.,.F.)
B_SPLINE_CURVE_WITH_KNOTS((3,2,2,3),(0.502515918601604,0.513888888888889,
0.527777777777778,0.539154184928472),.UNSPECIFIED.)
CURVE()
GEOMETRIC_REPRESENTATION_ITEM()
RATIONAL_B_SPLINE_CURVE((0.989891404642439,0.97209823130717,1.,0.965925826289068,
1.,0.972089799510949,0.989902162858515))
REPRESENTATION_ITEM('')
);
#222=(
BOUNDED_CURVE()
B_SPLINE_CURVE(2,(#5482,#5483,#5484,#5485,#5486,#5487,#5488),
 .UNSPECIFIED.,.F.,.F.)
B_SPLINE_CURVE_WITH_KNOTS((3,2,2,3),(0.460845815071528,0.472222222222222,
0.486111111111111,0.497903663249267),.UNSPECIFIED.)
CURVE()
GEOMETRIC_REPRESENTATION_ITEM()
RATIONAL_B_SPLINE_CURVE((0.989902162858515,0.972089799510949,1.,0.965925826289068,
1.,0.971068854156348,0.991266482904706))
REPRESENTATION_ITEM('')
);
#223=(
BOUNDED_CURVE()
B_SPLINE_CURVE(2,(#5491,#5492,#5493,#5494,#5495,#5496,#5497),
 .UNSPECIFIED.,.F.,.F.)
B_SPLINE_CURVE_WITH_KNOTS((3,2,2,3),(0.294179148404861,0.305555555555556,
0.319444444444444,0.3312369965826),.UNSPECIFIED.)
CURVE()
GEOMETRIC_REPRESENTATION_ITEM()
RATIONAL_B_SPLINE_CURVE((0.989902162858515,0.972089799510949,1.,0.965925826289068,
1.,0.971068854156348,0.991266482904706))
REPRESENTATION_ITEM('')
);
#224=(
BOUNDED_CURVE()
B_SPLINE_CURVE(2,(#5503,#5504,#5505,#5506,#5507,#5508,#5509),
 .UNSPECIFIED.,.F.,.F.)
B_SPLINE_CURVE_WITH_KNOTS((3,2,2,3),(0.502515918601604,0.513888888888889,
0.527777777777778,0.539154184928472),.UNSPECIFIED.)
CURVE()
GEOMETRIC_REPRESENTATION_ITEM()
RATIONAL_B_SPLINE_CURVE((0.989891404642439,0.97209823130717,1.,0.965925826289068,
1.,0.972089799510949,0.989902162858515))
REPRESENTATION_ITEM('')
);
#225=(
BOUNDED_CURVE()
B_SPLINE_CURVE(2,(#5512,#5513,#5514,#5515,#5516,#5517,#5518),
 .UNSPECIFIED.,.F.,.F.)
B_SPLINE_CURVE_WITH_KNOTS((3,2,2,3),(0.669182585268271,0.680555555555556,
0.694444444444444,0.705820851595139),.UNSPECIFIED.)
CURVE()
GEOMETRIC_REPRESENTATION_ITEM()
RATIONAL_B_SPLINE_CURVE((0.989891404642439,0.97209823130717,1.,0.965925826289068,
1.,0.972089799510949,0.989902162858515))
REPRESENTATION_ITEM('')
);
#226=(
BOUNDED_CURVE()
B_SPLINE_CURVE(2,(#5524,#5525,#5526,#5527,#5528,#5529,#5530),
 .UNSPECIFIED.,.F.,.F.)
B_SPLINE_CURVE_WITH_KNOTS((3,2,2,3),(0.627512481738195,0.638888888888889,
0.652777777777778,0.664570329915933),.UNSPECIFIED.)
CURVE()
GEOMETRIC_REPRESENTATION_ITEM()
RATIONAL_B_SPLINE_CURVE((0.989902162858515,0.972089799510949,1.,0.965925826289068,
1.,0.971068854156347,0.991266482904706))
REPRESENTATION_ITEM('')
);
#227=(
BOUNDED_CURVE()
B_SPLINE_CURVE(2,(#5533,#5534,#5535,#5536,#5537,#5538,#5539),
 .UNSPECIFIED.,.F.,.F.)
B_SPLINE_CURVE_WITH_KNOTS((3,2,2,3),(0.460845815071528,0.472222222222222,
0.486111111111111,0.497903663249267),.UNSPECIFIED.)
CURVE()
GEOMETRIC_REPRESENTATION_ITEM()
RATIONAL_B_SPLINE_CURVE((0.989902162858515,0.972089799510949,1.,0.965925826289068,
1.,0.971068854156348,0.991266482904706))
REPRESENTATION_ITEM('')
);
#228=(
BOUNDED_CURVE()
B_SPLINE_CURVE(2,(#5832,#5833,#5834,#5835,#5836,#5837,#5838),
 .UNSPECIFIED.,.F.,.F.)
B_SPLINE_CURVE_WITH_KNOTS((3,2,2,3),(0.0436499985776507,0.0555555555555556,
0.0694444444444444,0.0809569637747658),.UNSPECIFIED.)
CURVE()
GEOMETRIC_REPRESENTATION_ITEM()
RATIONAL_B_SPLINE_CURVE((0.991658091170858,0.970791614805482,1.,0.965925826289068,
1.,0.971755869987148,0.99033493732901))
REPRESENTATION_ITEM('')
);
#229=(
BOUNDED_CURVE()
B_SPLINE_CURVE(2,(#6146,#6147,#6148,#6149,#6150,#6151,#6152),
 .UNSPECIFIED.,.F.,.F.)
B_SPLINE_CURVE_WITH_KNOTS((3,2,2,3),(0.0853134259903282,0.0972222222222222,
0.111111111111111,0.123016668089016),.UNSPECIFIED.)
CURVE()
GEOMETRIC_REPRESENTATION_ITEM()
RATIONAL_B_SPLINE_CURVE((0.991669449544642,0.970783667812458,1.,0.965925826289068,
1.,0.970791614805482,0.991658091170858))
REPRESENTATION_ITEM('')
);
#230=(
BOUNDED_CURVE()
B_SPLINE_CURVE(2,(#6454,#6455,#6456,#6457,#6458,#6459,#6460),
 .UNSPECIFIED.,.F.,.F.)
B_SPLINE_CURVE_WITH_KNOTS((3,2,2,3),(0.210316665244317,0.222222222222222,
0.236111111111111,0.247623630441432),.UNSPECIFIED.)
CURVE()
GEOMETRIC_REPRESENTATION_ITEM()
RATIONAL_B_SPLINE_CURVE((0.991658091170858,0.970791614805482,1.,0.965925826289068,
1.,0.971755869987148,0.99033493732901))
REPRESENTATION_ITEM('')
);
#231=(
BOUNDED_CURVE()
B_SPLINE_CURVE(2,(#6768,#6769,#6770,#6771,#6772,#6773,#6774),
 .UNSPECIFIED.,.F.,.F.)
B_SPLINE_CURVE_WITH_KNOTS((3,2,2,3),(0.251980092656995,0.263888888888889,
0.277777777777778,0.289683334755683),.UNSPECIFIED.)
CURVE()
GEOMETRIC_REPRESENTATION_ITEM()
RATIONAL_B_SPLINE_CURVE((0.991669449544642,0.970783667812457,1.,0.965925826289068,
1.,0.970791614805482,0.991658091170858))
REPRESENTATION_ITEM('')
);
#232=(
BOUNDED_CURVE()
B_SPLINE_CURVE(2,(#7076,#7077,#7078,#7079,#7080,#7081,#7082),
 .UNSPECIFIED.,.F.,.F.)
B_SPLINE_CURVE_WITH_KNOTS((3,2,2,3),(0.376983331910984,0.388888888888889,
0.402777777777778,0.414290297108099),.UNSPECIFIED.)
CURVE()
GEOMETRIC_REPRESENTATION_ITEM()
RATIONAL_B_SPLINE_CURVE((0.991658091170857,0.970791614805482,1.,0.965925826289068,
1.,0.971755869987148,0.99033493732901))
REPRESENTATION_ITEM('')
);
#233=(
BOUNDED_CURVE()
B_SPLINE_CURVE(2,(#7390,#7391,#7392,#7393,#7394,#7395,#7396),
 .UNSPECIFIED.,.F.,.F.)
B_SPLINE_CURVE_WITH_KNOTS((3,2,2,3),(0.418646759323662,0.430555555555556,
0.444444444444444,0.456350001422349),.UNSPECIFIED.)
CURVE()
GEOMETRIC_REPRESENTATION_ITEM()
RATIONAL_B_SPLINE_CURVE((0.991669449544642,0.970783667812457,1.,0.965925826289068,
1.,0.970791614805482,0.991658091170858))
REPRESENTATION_ITEM('')
);
#234=(
BOUNDED_CURVE()
B_SPLINE_CURVE(2,(#7698,#7699,#7700,#7701,#7702,#7703,#7704),
 .UNSPECIFIED.,.F.,.F.)
B_SPLINE_CURVE_WITH_KNOTS((3,2,2,3),(0.543649998577651,0.555555555555556,
0.569444444444444,0.580956963774766),.UNSPECIFIED.)
CURVE()
GEOMETRIC_REPRESENTATION_ITEM()
RATIONAL_B_SPLINE_CURVE((0.991658091170858,0.970791614805482,1.,0.965925826289068,
1.,0.971755869987148,0.99033493732901))
REPRESENTATION_ITEM('')
);
#235=(
BOUNDED_CURVE()
B_SPLINE_CURVE(2,(#8012,#8013,#8014,#8015,#8016,#8017,#8018),
 .UNSPECIFIED.,.F.,.F.)
B_SPLINE_CURVE_WITH_KNOTS((3,2,2,3),(0.585313425990328,0.597222222222222,
0.611111111111111,0.623016668089016),.UNSPECIFIED.)
CURVE()
GEOMETRIC_REPRESENTATION_ITEM()
RATIONAL_B_SPLINE_CURVE((0.991669449544642,0.970783667812458,1.,0.965925826289068,
1.,0.970791614805482,0.991658091170858))
REPRESENTATION_ITEM('')
);
#236=(
BOUNDED_CURVE()
B_SPLINE_CURVE(2,(#8336,#8337,#8338,#8339,#8340,#8341,#8342),
 .UNSPECIFIED.,.F.,.F.)
B_SPLINE_CURVE_WITH_KNOTS((3,2,2,3),(0.00237636955856754,0.0138888888888889,
0.0277777777777778,0.0392935428934596),.UNSPECIFIED.)
CURVE()
GEOMETRIC_REPRESENTATION_ITEM()
RATIONAL_B_SPLINE_CURVE((0.99033493732901,0.971755869987148,1.,0.965925826289068,
1.,0.971747906970446,0.990345417239974))
REPRESENTATION_ITEM('')
);
#237=(
BOUNDED_CURVE()
B_SPLINE_CURVE(2,(#8643,#8644,#8645,#8646,#8647,#8648,#8649),
 .UNSPECIFIED.,.F.,.F.)
B_SPLINE_CURVE_WITH_KNOTS((3,2,2,3),(0.169043036225234,0.180555555555556,
0.194444444444444,0.205960209560126),.UNSPECIFIED.)
CURVE()
GEOMETRIC_REPRESENTATION_ITEM()
RATIONAL_B_SPLINE_CURVE((0.99033493732901,0.971755869987148,1.,0.965925826289068,
1.,0.971747906970446,0.990345417239974))
REPRESENTATION_ITEM('')
);
#238=(
BOUNDED_CURVE()
B_SPLINE_CURVE(2,(#8943,#8944,#8945,#8946,#8947,#8948,#8949),
 .UNSPECIFIED.,.F.,.F.)
B_SPLINE_CURVE_WITH_KNOTS((3,2,2,3),(0.127373123773207,0.138888888888889,
0.152777777777778,0.164686574009672),.UNSPECIFIED.)
CURVE()
GEOMETRIC_REPRESENTATION_ITEM()
RATIONAL_B_SPLINE_CURVE((0.990345417239974,0.971747906970446,1.,0.965925826289068,
1.,0.970783667812458,0.991669449544642))
REPRESENTATION_ITEM('')
);
#239=(
BOUNDED_CURVE()
B_SPLINE_CURVE(2,(#9265,#9266,#9267,#9268,#9269,#9270,#9271),
 .UNSPECIFIED.,.F.,.F.)
B_SPLINE_CURVE_WITH_KNOTS((3,2,2,3),(0.335709702891901,0.347222222222222,
0.361111111111111,0.372626876226793),.UNSPECIFIED.)
CURVE()
GEOMETRIC_REPRESENTATION_ITEM()
RATIONAL_B_SPLINE_CURVE((0.99033493732901,0.971755869987148,1.,0.965925826289068,
1.,0.971747906970446,0.990345417239974))
REPRESENTATION_ITEM('')
);
#240=(
BOUNDED_CURVE()
B_SPLINE_CURVE(2,(#9565,#9566,#9567,#9568,#9569,#9570,#9571),
 .UNSPECIFIED.,.F.,.F.)
B_SPLINE_CURVE_WITH_KNOTS((3,2,2,3),(0.294039790439874,0.305555555555556,
0.319444444444444,0.331353240676338),.UNSPECIFIED.)
CURVE()
GEOMETRIC_REPRESENTATION_ITEM()
RATIONAL_B_SPLINE_CURVE((0.990345417239974,0.971747906970446,1.,0.965925826289068,
1.,0.970783667812457,0.991669449544642))
REPRESENTATION_ITEM('')
);
#241=(
BOUNDED_CURVE()
B_SPLINE_CURVE(2,(#9887,#9888,#9889,#9890,#9891,#9892,#9893),
 .UNSPECIFIED.,.F.,.F.)
B_SPLINE_CURVE_WITH_KNOTS((3,2,2,3),(0.502376369558567,0.513888888888889,
0.527777777777778,0.53929354289346),.UNSPECIFIED.)
CURVE()
GEOMETRIC_REPRESENTATION_ITEM()
RATIONAL_B_SPLINE_CURVE((0.99033493732901,0.971755869987148,1.,0.965925826289068,
1.,0.971747906970446,0.990345417239974))
REPRESENTATION_ITEM('')
);
#242=(
BOUNDED_CURVE()
B_SPLINE_CURVE(2,(#10187,#10188,#10189,#10190,#10191,#10192,#10193),
 .UNSPECIFIED.,.F.,.F.)
B_SPLINE_CURVE_WITH_KNOTS((3,2,2,3),(0.46070645710654,0.472222222222222,
0.486111111111111,0.498019907343005),.UNSPECIFIED.)
CURVE()
GEOMETRIC_REPRESENTATION_ITEM()
RATIONAL_B_SPLINE_CURVE((0.990345417239974,0.971747906970446,1.,0.965925826289068,
1.,0.970783667812457,0.991669449544642))
REPRESENTATION_ITEM('')
);
#243=(
BOUNDED_CURVE()
B_SPLINE_CURVE(2,(#10502,#10503,#10504,#10505,#10506,#10507,#10508),
 .UNSPECIFIED.,.F.,.F.)
B_SPLINE_CURVE_WITH_KNOTS((3,2,2,3),(0.669182585268271,0.680555555555556,
0.694444444444444,0.706339757525137),.UNSPECIFIED.)
CURVE()
GEOMETRIC_REPRESENTATION_ITEM()
RATIONAL_B_SPLINE_CURVE((0.989891404642439,0.97209823130717,1.,0.965925826289068,
1.,0.970816746573466,0.991622219962871))
REPRESENTATION_ITEM('')
);
#244=(
BOUNDED_CURVE()
B_SPLINE_CURVE(2,(#10518,#10519,#10520,#10521,#10522,#10523,#10524),
 .UNSPECIFIED.,.F.,.F.)
B_SPLINE_CURVE_WITH_KNOTS((3,2,2,3),(0.669043036225234,0.680555555555556,
0.694444444444444,0.706021829576019),.UNSPECIFIED.)
CURVE()
GEOMETRIC_REPRESENTATION_ITEM()
RATIONAL_B_SPLINE_CURVE((0.99033493732901,0.971755869987148,1.,0.965925826289068,
1.,0.971596732089403,0.990545786488669))
REPRESENTATION_ITEM('')
);
#245=(
BOUNDED_CURVE()
B_SPLINE_CURVE(2,(#10823,#10824,#10825,#10826,#10827,#10828,#10829),
 .UNSPECIFIED.,.F.,.F.)
B_SPLINE_CURVE_WITH_KNOTS((3,2,2,3),(0.627373123773207,0.638888888888889,
0.652777777777778,0.664686574009672),.UNSPECIFIED.)
CURVE()
GEOMETRIC_REPRESENTATION_ITEM()
RATIONAL_B_SPLINE_CURVE((0.990345417239974,0.971747906970446,1.,0.965925826289068,
1.,0.970783667812458,0.991669449544642))
REPRESENTATION_ITEM('')
);
#246=(
BOUNDED_CURVE()
B_SPLINE_CURVE(2,(#10841,#10842,#10843,#10844,#10845,#10846,#10847),
 .UNSPECIFIED.,.F.,.F.)
B_SPLINE_CURVE_WITH_KNOTS((3,2,2,3),(0.62751099544001,0.638888888888889,
0.652777777777778,0.664570329915933),.UNSPECIFIED.)
CURVE()
GEOMETRIC_REPRESENTATION_ITEM()
RATIONAL_B_SPLINE_CURVE((0.989906817917388,0.972086153115408,1.,0.965925826289068,
1.,0.971068854156347,0.991266482904706))
REPRESENTATION_ITEM('')
);
#247=(
BOUNDED_CURVE()
B_SPLINE_CURVE(2,(#10859,#10860,#10861,#10862,#10863,#10864,#10865),
 .UNSPECIFIED.,.F.,.F.)
B_SPLINE_CURVE_WITH_KNOTS((3,2,2,3),(0.0436499985776507,0.0555555555555556,
0.0694444444444444,0.0809569637747658),.UNSPECIFIED.)
CURVE()
GEOMETRIC_REPRESENTATION_ITEM()
RATIONAL_B_SPLINE_CURVE((0.991658091170858,0.970791614805482,1.,0.965925826289068,
1.,0.971755869987148,0.99033493732901))
REPRESENTATION_ITEM('')
);
#248=(
BOUNDED_CURVE()
B_SPLINE_CURVE(2,(#10872,#10873,#10874,#10875,#10876,#10877,#10878),
 .UNSPECIFIED.,.F.,.F.)
B_SPLINE_CURVE_WITH_KNOTS((3,2,2,3),(0.0853134259903282,0.0972222222222222,
0.111111111111111,0.123016668089016),.UNSPECIFIED.)
CURVE()
GEOMETRIC_REPRESENTATION_ITEM()
RATIONAL_B_SPLINE_CURVE((0.991669449544642,0.970783667812458,1.,0.965925826289068,
1.,0.970791614805482,0.991658091170858))
REPRESENTATION_ITEM('')
);
#249=(
BOUNDED_CURVE()
B_SPLINE_CURVE(2,(#10883,#10884,#10885,#10886,#10887,#10888,#10889),
 .UNSPECIFIED.,.F.,.F.)
B_SPLINE_CURVE_WITH_KNOTS((3,2,2,3),(0.210316665244317,0.222222222222222,
0.236111111111111,0.247623630441432),.UNSPECIFIED.)
CURVE()
GEOMETRIC_REPRESENTATION_ITEM()
RATIONAL_B_SPLINE_CURVE((0.991658091170858,0.970791614805482,1.,0.965925826289068,
1.,0.971755869987148,0.99033493732901))
REPRESENTATION_ITEM('')
);
#250=(
BOUNDED_CURVE()
B_SPLINE_CURVE(2,(#10896,#10897,#10898,#10899,#10900,#10901,#10902),
 .UNSPECIFIED.,.F.,.F.)
B_SPLINE_CURVE_WITH_KNOTS((3,2,2,3),(0.251980092656995,0.263888888888889,
0.277777777777778,0.289683334755683),.UNSPECIFIED.)
CURVE()
GEOMETRIC_REPRESENTATION_ITEM()
RATIONAL_B_SPLINE_CURVE((0.991669449544642,0.970783667812457,1.,0.965925826289068,
1.,0.970791614805482,0.991658091170858))
REPRESENTATION_ITEM('')
);
#251=(
BOUNDED_CURVE()
B_SPLINE_CURVE(2,(#10907,#10908,#10909,#10910,#10911,#10912,#10913),
 .UNSPECIFIED.,.F.,.F.)
B_SPLINE_CURVE_WITH_KNOTS((3,2,2,3),(0.376983331910984,0.388888888888889,
0.402777777777778,0.414290297108099),.UNSPECIFIED.)
CURVE()
GEOMETRIC_REPRESENTATION_ITEM()
RATIONAL_B_SPLINE_CURVE((0.991658091170857,0.970791614805482,1.,0.965925826289068,
1.,0.971755869987148,0.99033493732901))
REPRESENTATION_ITEM('')
);
#252=(
BOUNDED_CURVE()
B_SPLINE_CURVE(2,(#10920,#10921,#10922,#10923,#10924,#10925,#10926),
 .UNSPECIFIED.,.F.,.F.)
B_SPLINE_CURVE_WITH_KNOTS((3,2,2,3),(0.418646759323662,0.430555555555556,
0.444444444444444,0.456350001422349),.UNSPECIFIED.)
CURVE()
GEOMETRIC_REPRESENTATION_ITEM()
RATIONAL_B_SPLINE_CURVE((0.991669449544642,0.970783667812457,1.,0.965925826289068,
1.,0.970791614805482,0.991658091170858))
REPRESENTATION_ITEM('')
);
#253=(
BOUNDED_CURVE()
B_SPLINE_CURVE(2,(#10931,#10932,#10933,#10934,#10935,#10936,#10937),
 .UNSPECIFIED.,.F.,.F.)
B_SPLINE_CURVE_WITH_KNOTS((3,2,2,3),(0.543649998577651,0.555555555555556,
0.569444444444444,0.580956963774766),.UNSPECIFIED.)
CURVE()
GEOMETRIC_REPRESENTATION_ITEM()
RATIONAL_B_SPLINE_CURVE((0.991658091170858,0.970791614805482,1.,0.965925826289068,
1.,0.971755869987148,0.99033493732901))
REPRESENTATION_ITEM('')
);
#254=(
BOUNDED_CURVE()
B_SPLINE_CURVE(2,(#10944,#10945,#10946,#10947,#10948,#10949,#10950),
 .UNSPECIFIED.,.F.,.F.)
B_SPLINE_CURVE_WITH_KNOTS((3,2,2,3),(0.585313425990328,0.597222222222222,
0.611111111111111,0.623016668089016),.UNSPECIFIED.)
CURVE()
GEOMETRIC_REPRESENTATION_ITEM()
RATIONAL_B_SPLINE_CURVE((0.991669449544642,0.970783667812458,1.,0.965925826289068,
1.,0.970791614805482,0.991658091170858))
REPRESENTATION_ITEM('')
);
#255=(
BOUNDED_CURVE()
B_SPLINE_CURVE(2,(#10956,#10957,#10958,#10959,#10960,#10961,#10962),
 .UNSPECIFIED.,.F.,.F.)
B_SPLINE_CURVE_WITH_KNOTS((3,2,2,3),(0.00237636955856754,0.0138888888888889,
0.0277777777777778,0.0392935428934596),.UNSPECIFIED.)
CURVE()
GEOMETRIC_REPRESENTATION_ITEM()
RATIONAL_B_SPLINE_CURVE((0.99033493732901,0.971755869987148,1.,0.965925826289068,
1.,0.971747906970446,0.990345417239974))
REPRESENTATION_ITEM('')
);
#256=(
BOUNDED_CURVE()
B_SPLINE_CURVE(2,(#10968,#10969,#10970,#10971,#10972,#10973,#10974),
 .UNSPECIFIED.,.F.,.F.)
B_SPLINE_CURVE_WITH_KNOTS((3,2,2,3),(0.169043036225234,0.180555555555556,
0.194444444444444,0.205960209560126),.UNSPECIFIED.)
CURVE()
GEOMETRIC_REPRESENTATION_ITEM()
RATIONAL_B_SPLINE_CURVE((0.99033493732901,0.971755869987148,1.,0.965925826289068,
1.,0.971747906970446,0.990345417239974))
REPRESENTATION_ITEM('')
);
#257=(
BOUNDED_CURVE()
B_SPLINE_CURVE(2,(#10979,#10980,#10981,#10982,#10983,#10984,#10985),
 .UNSPECIFIED.,.F.,.F.)
B_SPLINE_CURVE_WITH_KNOTS((3,2,2,3),(0.127373123773207,0.138888888888889,
0.152777777777778,0.164686574009672),.UNSPECIFIED.)
CURVE()
GEOMETRIC_REPRESENTATION_ITEM()
RATIONAL_B_SPLINE_CURVE((0.990345417239974,0.971747906970446,1.,0.965925826289068,
1.,0.970783667812458,0.991669449544642))
REPRESENTATION_ITEM('')
);
#258=(
BOUNDED_CURVE()
B_SPLINE_CURVE(2,(#10992,#10993,#10994,#10995,#10996,#10997,#10998),
 .UNSPECIFIED.,.F.,.F.)
B_SPLINE_CURVE_WITH_KNOTS((3,2,2,3),(0.335709702891901,0.347222222222222,
0.361111111111111,0.372626876226793),.UNSPECIFIED.)
CURVE()
GEOMETRIC_REPRESENTATION_ITEM()
RATIONAL_B_SPLINE_CURVE((0.99033493732901,0.971755869987148,1.,0.965925826289068,
1.,0.971747906970446,0.990345417239974))
REPRESENTATION_ITEM('')
);
#259=(
BOUNDED_CURVE()
B_SPLINE_CURVE(2,(#11003,#11004,#11005,#11006,#11007,#11008,#11009),
 .UNSPECIFIED.,.F.,.F.)
B_SPLINE_CURVE_WITH_KNOTS((3,2,2,3),(0.294039790439874,0.305555555555556,
0.319444444444444,0.331353240676338),.UNSPECIFIED.)
CURVE()
GEOMETRIC_REPRESENTATION_ITEM()
RATIONAL_B_SPLINE_CURVE((0.990345417239974,0.971747906970446,1.,0.965925826289068,
1.,0.970783667812457,0.991669449544642))
REPRESENTATION_ITEM('')
);
#260=(
BOUNDED_CURVE()
B_SPLINE_CURVE(2,(#11016,#11017,#11018,#11019,#11020,#11021,#11022),
 .UNSPECIFIED.,.F.,.F.)
B_SPLINE_CURVE_WITH_KNOTS((3,2,2,3),(0.502376369558567,0.513888888888889,
0.527777777777778,0.53929354289346),.UNSPECIFIED.)
CURVE()
GEOMETRIC_REPRESENTATION_ITEM()
RATIONAL_B_SPLINE_CURVE((0.99033493732901,0.971755869987148,1.,0.965925826289068,
1.,0.971747906970446,0.990345417239974))
REPRESENTATION_ITEM('')
);
#261=(
BOUNDED_CURVE()
B_SPLINE_CURVE(2,(#11027,#11028,#11029,#11030,#11031,#11032,#11033),
 .UNSPECIFIED.,.F.,.F.)
B_SPLINE_CURVE_WITH_KNOTS((3,2,2,3),(0.46070645710654,0.472222222222222,
0.486111111111111,0.498019907343005),.UNSPECIFIED.)
CURVE()
GEOMETRIC_REPRESENTATION_ITEM()
RATIONAL_B_SPLINE_CURVE((0.990345417239974,0.971747906970446,1.,0.965925826289068,
1.,0.970783667812457,0.991669449544642))
REPRESENTATION_ITEM('')
);
#262=(
BOUNDED_CURVE()
B_SPLINE_CURVE(2,(#11040,#11041,#11042,#11043,#11044,#11045,#11046),
 .UNSPECIFIED.,.F.,.F.)
B_SPLINE_CURVE_WITH_KNOTS((3,2,2,3),(0.669043036225234,0.680555555555556,
0.694444444444444,0.705960209560126),.UNSPECIFIED.)
CURVE()
GEOMETRIC_REPRESENTATION_ITEM()
RATIONAL_B_SPLINE_CURVE((0.99033493732901,0.971755869987148,1.,0.965925826289068,
1.,0.971747906970446,0.990345417239974))
REPRESENTATION_ITEM('')
);
#263=(
BOUNDED_CURVE()
B_SPLINE_CURVE(2,(#11056,#11057,#11058,#11059,#11060,#11061,#11062),
 .UNSPECIFIED.,.F.,.F.)
B_SPLINE_CURVE_WITH_KNOTS((3,2,2,3),(0.627373123773207,0.638888888888889,
0.652777777777778,0.664686574009672),.UNSPECIFIED.)
CURVE()
GEOMETRIC_REPRESENTATION_ITEM()
RATIONAL_B_SPLINE_CURVE((0.990345417239974,0.971747906970446,1.,0.965925826289068,
1.,0.970783667812458,0.991669449544642))
REPRESENTATION_ITEM('')
);
#264=(
BOUNDED_CURVE()
B_SPLINE_CURVE(2,(#11068,#11069,#11070,#11071,#11072,#11073,#11074),
 .UNSPECIFIED.,.F.,.F.)
B_SPLINE_CURVE_WITH_KNOTS((3,2,2,3),(0.710316665244317,0.722222222222222,
0.736111111111111,0.747623630441432),.UNSPECIFIED.)
CURVE()
GEOMETRIC_REPRESENTATION_ITEM()
RATIONAL_B_SPLINE_CURVE((0.991658091170858,0.970791614805482,1.,0.965925826289068,
1.,0.971755869987148,0.99033493732901))
REPRESENTATION_ITEM('')
);
#265=(
BOUNDED_CURVE()
B_SPLINE_CURVE(2,(#11078,#11079,#11080,#11081,#11082,#11083,#11084),
 .UNSPECIFIED.,.F.,.F.)
B_SPLINE_CURVE_WITH_KNOTS((3,2,2,3),(0.710237354772895,0.722222222222222,
0.736111111111111,0.747623630441432),.UNSPECIFIED.)
CURVE()
GEOMETRIC_REPRESENTATION_ITEM()
RATIONAL_B_SPLINE_CURVE((0.991938323047677,0.970597039213297,1.,0.965925826289068,
1.,0.971755869987148,0.99033493732901))
REPRESENTATION_ITEM('')
);
#266=(
BOUNDED_CURVE()
B_SPLINE_CURVE(2,(#11094,#11095,#11096,#11097,#11098,#11099,#11100),
 .UNSPECIFIED.,.F.,.F.)
B_SPLINE_CURVE_WITH_KNOTS((3,2,2,3),(0.751980092656995,0.763888888888889,
0.777777777777778,0.790814625085749),.UNSPECIFIED.)
CURVE()
GEOMETRIC_REPRESENTATION_ITEM()
RATIONAL_B_SPLINE_CURVE((0.991669449544642,0.970783667812458,1.,0.965925826289068,
1.,0.968016174413341,0.996075776898402))
REPRESENTATION_ITEM('')
);
#267=(
BOUNDED_CURVE()
B_SPLINE_CURVE(2,(#11104,#11105,#11106,#11107,#11108,#11109,#11110),
 .UNSPECIFIED.,.F.,.F.)
B_SPLINE_CURVE_WITH_KNOTS((3,2,2,3),(0.751980092656995,0.763888888888889,
0.777777777777778,0.790051277060462),.UNSPECIFIED.)
CURVE()
GEOMETRIC_REPRESENTATION_ITEM()
RATIONAL_B_SPLINE_CURVE((0.991669449544642,0.970783667812458,1.,0.965925826289068,
1.,0.969888927044859,0.99299567954319))
REPRESENTATION_ITEM('')
);
#268=(
BOUNDED_CURVE()
B_SPLINE_CURVE(2,(#11738,#11739,#11740,#11741,#11742),.UNSPECIFIED.,.F.,
 .F.)
B_SPLINE_CURVE_WITH_KNOTS((3,2,3),(0.100045993303939,0.111111111111111,
0.122900233666328),.UNSPECIFIED.)
CURVE()
GEOMETRIC_REPRESENTATION_ITEM()
RATIONAL_B_SPLINE_CURVE((0.988961607054814,0.972853498266867,1.,0.971077268091095,
0.991254739061418))
REPRESENTATION_ITEM('')
);
#269=(
BOUNDED_CURVE()
B_SPLINE_CURVE(2,(#13879,#13880,#13881,#13882,#13883,#13884,#13885),
 .UNSPECIFIED.,.F.,.F.)
B_SPLINE_CURVE_WITH_KNOTS((3,2,2,3),(0.00238251257661542,0.0138888888888889,
0.0277777777777778,0.0392874082837476),.UNSPECIFIED.)
CURVE()
GEOMETRIC_REPRESENTATION_ITEM()
RATIONAL_B_SPLINE_CURVE((0.990315123280967,0.971770940902162,1.,0.965925826289068,
1.,0.971762957256948,0.990325616225644))
REPRESENTATION_ITEM('')
);
#270=(
BOUNDED_CURVE()
B_SPLINE_CURVE(2,(#16908,#16909,#16910,#16911,#16912,#16913,#16914,#16915,
#16916,#16917,#16918,#16919,#16920),.UNSPECIFIED.,.F.,.F.)
B_SPLINE_CURVE_WITH_KNOTS((3,2,2,2,2,2,3),(0.752096336750733,0.763888888888889,
0.777777777777778,0.791666666666667,0.805555555555556,0.819444444444444,
0.8312369965826),.UNSPECIFIED.)
CURVE()
GEOMETRIC_REPRESENTATION_ITEM()
RATIONAL_B_SPLINE_CURVE((0.991266482904706,0.971068854156347,1.,0.965925826289068,
1.,0.965925826289068,1.,0.965925826289068,1.,0.965925826289068,1.,0.971068854156347,
0.991266482904706))
REPRESENTATION_ITEM('')
);
#271=(
BOUNDED_CURVE()
B_SPLINE_CURVE(2,(#16923,#16924,#16925,#16926,#16927,#16928,#16929,#16930,
#16931,#16932,#16933,#16934,#16935),.UNSPECIFIED.,.F.,.F.)
B_SPLINE_CURVE_WITH_KNOTS((3,2,2,2,2,2,3),(0.9187630034174,0.930555555555556,
0.944444444444444,0.958333333333333,0.972222222222222,0.986111111111111,
0.997903663249267),.UNSPECIFIED.)
CURVE()
GEOMETRIC_REPRESENTATION_ITEM()
RATIONAL_B_SPLINE_CURVE((0.991266482904706,0.971068854156347,1.,0.965925826289068,
1.,0.965925826289068,1.,0.965925826289068,1.,0.965925826289068,1.,0.971068854156347,
0.991266482904706))
REPRESENTATION_ITEM('')
);
#272=(
BOUNDED_CURVE()
B_SPLINE_CURVE(2,(#16941,#16942,#16943,#16944,#16945,#16946,#16947),
 .UNSPECIFIED.,.F.,.F.)
B_SPLINE_CURVE_WITH_KNOTS((3,2,2,3),(0.876137334108343,0.888888888888889,
0.902777777777778,0.914150748065062),.UNSPECIFIED.)
CURVE()
GEOMETRIC_REPRESENTATION_ITEM()
RATIONAL_B_SPLINE_CURVE((0.994876443540461,0.968716094127271,1.,0.965925826289068,
1.,0.97209823130717,0.989891404642439))
REPRESENTATION_ITEM('')
);
#273=(
BOUNDED_CURVE()
B_SPLINE_CURVE(2,(#16965,#16966,#16967,#16968,#16969,#16970,#16971),
 .UNSPECIFIED.,.F.,.F.)
B_SPLINE_CURVE_WITH_KNOTS((3,2,2,3),(0.70986335383276,0.722222222222222,
0.736111111111111,0.747484081398396),.UNSPECIFIED.)
CURVE()
GEOMETRIC_REPRESENTATION_ITEM()
RATIONAL_B_SPLINE_CURVE((0.993319695194941,0.969679487557137,1.,0.965925826289068,
1.,0.97209823130717,0.989891404642439))
REPRESENTATION_ITEM('')
);
#274=(
BOUNDED_CURVE()
B_SPLINE_CURVE(2,(#16989,#16990,#16991,#16992,#16993,#16994,#16995),
 .UNSPECIFIED.,.F.,.F.)
B_SPLINE_CURVE_WITH_KNOTS((3,2,2,3),(0.835849251934938,0.847222222222222,
0.861111111111111,0.87338656566107),.UNSPECIFIED.)
CURVE()
GEOMETRIC_REPRESENTATION_ITEM()
RATIONAL_B_SPLINE_CURVE((0.989891404642439,0.97209823130717,1.,0.965925826289068,
1.,0.969884130108453,0.993003043077312))
REPRESENTATION_ITEM('')
);
#275=(
BOUNDED_CURVE()
B_SPLINE_CURVE(2,(#17000,#17001,#17002,#17003,#17004,#17005,#17006),
 .UNSPECIFIED.,.F.,.F.)
B_SPLINE_CURVE_WITH_KNOTS((3,2,2,3),(0.794135813030579,0.805555555555556,
0.819444444444444,0.8312369965826),.UNSPECIFIED.)
CURVE()
GEOMETRIC_REPRESENTATION_ITEM()
RATIONAL_B_SPLINE_CURVE((0.990038529153568,0.971983483081829,1.,0.965925826289068,
1.,0.971068854156347,0.991266482904706))
REPRESENTATION_ITEM('')
);
#276=(
BOUNDED_CURVE()
B_SPLINE_CURVE(2,(#17600,#17601,#17602,#17603,#17604,#17605,#17606),
 .UNSPECIFIED.,.F.,.F.)
B_SPLINE_CURVE_WITH_KNOTS((3,2,2,3),(0.792847371553036,0.805555555555556,
0.819444444444444,0.831353240676339),.UNSPECIFIED.)
CURVE()
GEOMETRIC_REPRESENTATION_ITEM()
RATIONAL_B_SPLINE_CURVE((0.994699154130647,0.968822497413832,1.,0.965925826289068,
1.,0.970783667812457,0.991669449544642))
REPRESENTATION_ITEM('')
);
#277=(
BOUNDED_CURVE()
B_SPLINE_CURVE(2,(#17945,#17946,#17947,#17948,#17949,#17950,#17951,#17952,
#17953,#17954,#17955,#17956,#17957),.UNSPECIFIED.,.F.,.F.)
B_SPLINE_CURVE_WITH_KNOTS((3,2,2,2,2,2,3),(0.835709702891901,0.847222222222222,
0.861111111111111,0.875,0.888888888888889,0.902777777777778,0.914290297108099),
 .UNSPECIFIED.)
CURVE()
GEOMETRIC_REPRESENTATION_ITEM()
RATIONAL_B_SPLINE_CURVE((0.99033493732901,0.971755869987148,1.,0.965925826289068,
1.,0.965925826289068,1.,0.965925826289068,1.,0.965925826289068,1.,0.971755869987148,
0.99033493732901))
REPRESENTATION_ITEM('')
);
#278=(
BOUNDED_CURVE()
B_SPLINE_CURVE(2,(#18274,#18275,#18276,#18277,#18278,#18279,#18280,#18281,
#18282,#18283,#18284),.UNSPECIFIED.,.F.,.F.)
B_SPLINE_CURVE_WITH_KNOTS((3,2,2,2,2,3),(0.918646759323661,0.930555555555556,
0.944444444444444,0.958333333333333,0.972222222222222,0.972937471698986),
 .UNSPECIFIED.)
CURVE()
GEOMETRIC_REPRESENTATION_ITEM()
RATIONAL_B_SPLINE_CURVE((0.991669449544642,0.970783667812457,1.,0.965925826289068,
1.,0.965925826289068,1.,0.965925826289068,1.,0.998245249485912,0.996671231123559))
REPRESENTATION_ITEM('')
);
#279=(
BOUNDED_CURVE()
B_SPLINE_CURVE(2,(#18310,#18311,#18312,#18313,#18314,#18315,#18316),
 .UNSPECIFIED.,.F.,.F.)
B_SPLINE_CURVE_WITH_KNOTS((3,2,2,3),(0.793632040812071,0.805555555555556,
0.819444444444444,0.831353240676339),.UNSPECIFIED.)
CURVE()
GEOMETRIC_REPRESENTATION_ITEM()
RATIONAL_B_SPLINE_CURVE((0.991721153062242,0.970747558291768,1.,0.965925826289068,
1.,0.970783667812457,0.991669449544642))
REPRESENTATION_ITEM('')
);
#280=(
BOUNDED_CURVE()
B_SPLINE_CURVE(2,(#18327,#18328,#18329,#18330,#18331,#18332,#18333,#18334,
#18335,#18336,#18337,#18338,#18339),.UNSPECIFIED.,.F.,.F.)
B_SPLINE_CURVE_WITH_KNOTS((3,2,2,2,2,2,3),(0.835709702891901,0.847222222222222,
0.861111111111111,0.875,0.888888888888889,0.902777777777778,0.914290297108099),
 .UNSPECIFIED.)
CURVE()
GEOMETRIC_REPRESENTATION_ITEM()
RATIONAL_B_SPLINE_CURVE((0.99033493732901,0.971755869987148,1.,0.965925826289068,
1.,0.965925826289068,1.,0.965925826289068,1.,0.965925826289068,1.,0.971755869987148,
0.99033493732901))
REPRESENTATION_ITEM('')
);
#281=(
BOUNDED_CURVE()
B_SPLINE_CURVE(2,(#18346,#18347,#18348,#18349,#18350,#18351,#18352,#18353,
#18354,#18355,#18356,#18357,#18358),.UNSPECIFIED.,.F.,.F.)
B_SPLINE_CURVE_WITH_KNOTS((3,2,2,2,2,2,3),(0.918646759323661,0.930555555555556,
0.944444444444444,0.958333333333333,0.972222222222222,0.986111111111111,
0.998105847682342),.UNSPECIFIED.)
CURVE()
GEOMETRIC_REPRESENTATION_ITEM()
RATIONAL_B_SPLINE_CURVE((0.991669449544642,0.970783667812457,1.,0.965925826289068,
1.,0.965925826289068,1.,0.965925826289068,1.,0.965925826289068,1.,0.970572826896762,
0.991973505068469))
REPRESENTATION_ITEM('')
);
#294=B_SPLINE_CURVE_WITH_KNOTS('',3,(#5030,#5031,#5032,#5033,#5034,#5035,
#5036,#5037,#5038,#5039,#5040,#5041,#5042,#5043),.UNSPECIFIED.,.F.,.F.,
(4,2,2,2,2,2,4),(-1.03917131396603,-0.897633242543498,-0.747971508363487,
-0.598309774183476,-0.448752618812303,-0.299195463441129,-0.15765582292854),
 .UNSPECIFIED.);
#295=B_SPLINE_CURVE_WITH_KNOTS('',3,(#5051,#5052,#5053,#5054,#5055,#5056,
#5057,#5058,#5059,#5060,#5061,#5062,#5063,#5064),.UNSPECIFIED.,.F.,.F.,
(4,2,2,2,2,2,4),(0.15765582292854,0.299195463441129,0.448752618812303,0.598309774183476,
0.747971508363487,0.897633242543498,1.03917131396603),.UNSPECIFIED.);
#296=B_SPLINE_CURVE_WITH_KNOTS('',3,(#5068,#5069,#5070,#5071,#5072,#5073,
#5074,#5075,#5076,#5077,#5078,#5079,#5080,#5081,#5082,#5083,#5084,#5085),
 .UNSPECIFIED.,.F.,.F.,(4,2,2,2,2,2,2,2,4),(9.99999990605937E-7,1.61032997746592,
3.21316436538662,5.0051599487382,6.82527051959712,8.64573442526924,10.4385724656072,
12.0409045434925,13.6509631821543),.UNSPECIFIED.);
#297=B_SPLINE_CURVE_WITH_KNOTS('',3,(#5091,#5092,#5093,#5094,#5095,#5096),
 .UNSPECIFIED.,.F.,.F.,(4,2,4),(0.,0.149581313593702,0.157659940647757),
 .UNSPECIFIED.);
#298=B_SPLINE_CURVE_WITH_KNOTS('',3,(#5101,#5102,#5103,#5104,#5105,#5106,
#5107,#5108,#5109,#5110,#5111,#5112,#5113,#5114,#5115,#5116,#5117,#5118),
 .UNSPECIFIED.,.F.,.F.,(4,2,2,2,2,2,2,2,4),(-1.19705479780107,-1.04741995877816,
-0.89778511975524,-0.748086035420359,-0.598386951085478,-0.448814985396906,
-0.299243019708333,-0.149621509854167,0.),.UNSPECIFIED.);
#299=B_SPLINE_CURVE_WITH_KNOTS('',3,(#5126,#5127,#5128,#5129,#5130,#5131,
#5132,#5133,#5134,#5135,#5136,#5137,#5138,#5139,#5140,#5141,#5142,#5143),
 .UNSPECIFIED.,.F.,.F.,(4,2,2,2,2,2,2,2,4),(0.,0.149634938642595,0.299269877285189,
0.448970279983913,0.598670682682636,0.748241851215363,0.897813019748089,
1.04743440734167,1.19705579493525),.UNSPECIFIED.);
#300=B_SPLINE_CURVE_WITH_KNOTS('',3,(#5151,#5152,#5153,#5154,#5155,#5156,
#5157,#5158,#5159,#5160,#5161,#5162),.UNSPECIFIED.,.F.,.F.,(4,2,2,2,2,4),
(1.19705479780107,1.34668963682399,1.4963244758469,1.64602356018178,1.79572264451666,
1.83085170358366),.UNSPECIFIED.);
#301=B_SPLINE_CURVE_WITH_KNOTS('',3,(#5167,#5168,#5169,#5170,#5171,#5172,
#5173,#5174,#5175,#5176),.UNSPECIFIED.,.F.,.F.,(4,2,2,2,4),(1.83085170358366,
1.94529461020524,2.09486657589381,2.24448808574798,2.39410959560214),
 .UNSPECIFIED.);
#302=B_SPLINE_CURVE_WITH_KNOTS('',3,(#5184,#5185,#5186,#5187,#5188,#5189,
#5190,#5191,#5192,#5193,#5194,#5195,#5196,#5197,#5198,#5199,#5200,#5201),
 .UNSPECIFIED.,.F.,.F.,(4,2,2,2,2,2,2,2,4),(1.19705579493525,1.34667718252883,
1.49629857012241,1.64586973865514,1.79544090718787,1.94514130988659,2.09484171258531,
2.24447665122791,2.3941115898705),.UNSPECIFIED.);
#303=B_SPLINE_CURVE_WITH_KNOTS('',3,(#5241,#5242,#5243,#5244),
 .UNSPECIFIED.,.F.,.F.,(4,4),(-0.0621119208606391,-0.00070906240656004),
 .UNSPECIFIED.);
#304=B_SPLINE_CURVE_WITH_KNOTS('',3,(#5840,#5841,#5842,#5843,#5844,#5845,
#5846),.UNSPECIFIED.,.F.,.F.,(4,1,2,4),(6.93889390390723E-18,0.000802008422543448,
0.00160401684508564,0.00313358895216332),.UNSPECIFIED.);
#305=B_SPLINE_CURVE_WITH_KNOTS('',3,(#6138,#6139,#6140,#6141,#6142,#6143,
#6144),.UNSPECIFIED.,.F.,.F.,(4,1,2,4),(6.93889390390723E-18,0.000802008422543318,
0.00160401684508542,0.00313356353166787),.UNSPECIFIED.);
#306=B_SPLINE_CURVE_WITH_KNOTS('',3,(#6153,#6154,#6155,#6156,#6157,#6158,
#6159,#6160,#6161),.UNSPECIFIED.,.F.,.F.,(4,2,3,4),(0.,0.000802008422906776,
0.00160401684587021,0.00313013376960514),.UNSPECIFIED.);
#307=B_SPLINE_CURVE_WITH_KNOTS('',3,(#6462,#6463,#6464,#6465,#6466,#6467,
#6468),.UNSPECIFIED.,.F.,.F.,(4,1,2,4),(0.,0.000802008422543473,0.00160401684508569,
0.0031335889521633),.UNSPECIFIED.);
#308=B_SPLINE_CURVE_WITH_KNOTS('',3,(#6760,#6761,#6762,#6763,#6764,#6765,
#6766),.UNSPECIFIED.,.F.,.F.,(4,1,2,4),(1.55158384577955E-17,0.000802008422543312,
0.0016040168450854,0.00313356353166786),.UNSPECIFIED.);
#309=B_SPLINE_CURVE_WITH_KNOTS('',3,(#6775,#6776,#6777,#6778,#6779,#6780,
#6781,#6782,#6783),.UNSPECIFIED.,.F.,.F.,(4,2,3,4),(0.,0.000802008422906776,
0.0016040168458702,0.00313013376960513),.UNSPECIFIED.);
#310=B_SPLINE_CURVE_WITH_KNOTS('',3,(#7084,#7085,#7086,#7087,#7088,#7089,
#7090),.UNSPECIFIED.,.F.,.F.,(4,1,2,4),(0.,0.000802008422543476,0.00160401684508569,
0.00313358895216332),.UNSPECIFIED.);
#311=B_SPLINE_CURVE_WITH_KNOTS('',3,(#7382,#7383,#7384,#7385,#7386,#7387,
#7388),.UNSPECIFIED.,.F.,.F.,(4,1,2,4),(1.55158384577955E-17,0.000802008422543312,
0.0016040168450854,0.00313356353166786),.UNSPECIFIED.);
#312=B_SPLINE_CURVE_WITH_KNOTS('',3,(#7397,#7398,#7399,#7400,#7401,#7402,
#7403,#7404,#7405),.UNSPECIFIED.,.F.,.F.,(4,2,3,4),(0.,0.000802008422906761,
0.0016040168458702,0.00313013376960514),.UNSPECIFIED.);
#313=B_SPLINE_CURVE_WITH_KNOTS('',3,(#7706,#7707,#7708,#7709,#7710,#7711,
#7712),.UNSPECIFIED.,.F.,.F.,(4,1,2,4),(6.93889390390723E-18,0.000802008422543454,
0.00160401684508567,0.00313358895216332),.UNSPECIFIED.);
#314=B_SPLINE_CURVE_WITH_KNOTS('',3,(#8004,#8005,#8006,#8007,#8008,#8009,
#8010),.UNSPECIFIED.,.F.,.F.,(4,1,2,4),(6.93889390390723E-18,0.000802008422543302,
0.00160401684508539,0.00313356353166788),.UNSPECIFIED.);
#315=B_SPLINE_CURVE_WITH_KNOTS('',3,(#8020,#8021,#8022,#8023,#8024,#8025,
#8026,#8027,#8028,#8029),.UNSPECIFIED.,.F.,.F.,(4,3,3,4),(0.,0.00080200842290677,
0.00160401684587019,0.00311589056383513),.UNSPECIFIED.);
#316=B_SPLINE_CURVE_WITH_KNOTS('',3,(#8322,#8323,#8324,#8325,#8326,#8327,
#8328),.UNSPECIFIED.,.F.,.F.,(4,1,2,4),(9.81307786677359E-18,0.000802008422577623,
0.00160401684514919,0.00290160460940762),.UNSPECIFIED.);
#317=B_SPLINE_CURVE_WITH_KNOTS('',3,(#8635,#8636,#8637,#8638,#8639,#8640,
#8641),.UNSPECIFIED.,.F.,.F.,(4,1,2,4),(6.93889390390723E-18,0.000802008422577624,
0.00160401684514921,0.00313695506663807),.UNSPECIFIED.);
#318=B_SPLINE_CURVE_WITH_KNOTS('',3,(#8950,#8951,#8952,#8953,#8954,#8955,
#8956,#8957,#8958),.UNSPECIFIED.,.F.,.F.,(4,2,3,4),(0.,0.000802008422904874,
0.00160401684586611,0.00313011409353478),.UNSPECIFIED.);
#319=B_SPLINE_CURVE_WITH_KNOTS('',3,(#8959,#8960,#8961,#8962,#8963,#8964,
#8965),.UNSPECIFIED.,.F.,.F.,(4,1,2,4),(0.,0.000802008422577178,0.00160401684514837,
0.00313692497239048),.UNSPECIFIED.);
#320=B_SPLINE_CURVE_WITH_KNOTS('',3,(#9257,#9258,#9259,#9260,#9261,#9262,
#9263),.UNSPECIFIED.,.F.,.F.,(4,1,2,4),(6.93889390390723E-18,0.000802008422577621,
0.00160401684514922,0.00313695506663807),.UNSPECIFIED.);
#321=B_SPLINE_CURVE_WITH_KNOTS('',3,(#9572,#9573,#9574,#9575,#9576,#9577,
#9578,#9579,#9580),.UNSPECIFIED.,.F.,.F.,(4,2,3,4),(0.,0.000802008422904867,
0.00160401684586611,0.00313011409353478),.UNSPECIFIED.);
#322=B_SPLINE_CURVE_WITH_KNOTS('',3,(#9581,#9582,#9583,#9584,#9585,#9586,
#9587),.UNSPECIFIED.,.F.,.F.,(4,1,2,4),(0.,0.000802008422577179,0.00160401684514836,
0.0031369249723905),.UNSPECIFIED.);
#323=B_SPLINE_CURVE_WITH_KNOTS('',3,(#9879,#9880,#9881,#9882,#9883,#9884,
#9885),.UNSPECIFIED.,.F.,.F.,(4,1,2,4),(0.,0.000802008422577639,0.00160401684514923,
0.00313695506663809),.UNSPECIFIED.);
#324=B_SPLINE_CURVE_WITH_KNOTS('',3,(#10194,#10195,#10196,#10197,#10198,
#10199,#10200,#10201,#10202),.UNSPECIFIED.,.F.,.F.,(4,2,3,4),(0.,0.000802008422904871,
0.0016040168458661,0.00313011409353478),.UNSPECIFIED.);
#325=B_SPLINE_CURVE_WITH_KNOTS('',3,(#10203,#10204,#10205,#10206,#10207,
#10208,#10209),.UNSPECIFIED.,.F.,.F.,(4,1,2,4),(0.,0.000802008422577185,
0.00160401684514837,0.00313692497239049),.UNSPECIFIED.);
#326=B_SPLINE_CURVE_WITH_KNOTS('',3,(#10510,#10511,#10512,#10513,#10514,
#10515,#10516),.UNSPECIFIED.,.F.,.F.,(4,1,2,4),(0.,0.000802008422577623,
0.0016040168451492,0.00313695506663806),.UNSPECIFIED.);
#327=B_SPLINE_CURVE_WITH_KNOTS('',3,(#10525,#10526,#10527,#10528,#10529,
#10530),.UNSPECIFIED.,.F.,.F.,(4,2,4),(-0.317506811553133,-0.158581801084095,
0.),.UNSPECIFIED.);
#328=B_SPLINE_CURVE_WITH_KNOTS('',3,(#10831,#10832,#10833,#10834,#10835,
#10836,#10837,#10838,#10839),.UNSPECIFIED.,.F.,.F.,(4,2,3,4),(0.,0.000802008422904858,
0.00160401684586608,0.00313011409353478),.UNSPECIFIED.);
#329=B_SPLINE_CURVE_WITH_KNOTS('',3,(#10850,#10851,#10852,#10853,#10854,
#10855),.UNSPECIFIED.,.F.,.F.,(4,2,4),(1.31690409731013E-6,0.127022192229024,
0.28504745144389),.UNSPECIFIED.);
#330=B_SPLINE_CURVE_WITH_KNOTS('',3,(#11049,#11050,#11051,#11052),
 .UNSPECIFIED.,.F.,.F.,(4,4),(2.66453525910035E-15,0.0918230658993515),
 .UNSPECIFIED.);
#331=B_SPLINE_CURVE_WITH_KNOTS('',3,(#11086,#11087,#11088,#11089),
 .UNSPECIFIED.,.F.,.F.,(4,4),(1.09261755714425,1.19656563806167),
 .UNSPECIFIED.);
#332=B_SPLINE_CURVE_WITH_KNOTS('',3,(#11111,#11112,#11113,#11114,#11115,
#11116),.UNSPECIFIED.,.F.,.F.,(4,2,4),(-0.972867842394702,-0.897435512998064,
-0.788327277048526),.UNSPECIFIED.);
#333=B_SPLINE_CURVE_WITH_KNOTS('',3,(#11409,#11410,#11411,#11412,#11413,
#11414,#11415,#11416,#11417,#11418,#11419,#11420),.UNSPECIFIED.,.F.,.F.,
(4,2,2,2,2,4),(1.00000000158624E-6,0.692107157618177,1.39024716069207,2.74744494620693,
4.13283236453521,5.48383660931837),.UNSPECIFIED.);
#334=B_SPLINE_CURVE_WITH_KNOTS('',3,(#11421,#11422,#11423,#11424,#11425,
#11426),.UNSPECIFIED.,.F.,.F.,(4,2,4),(0.00114961664817087,0.0016040168451492,
0.00313695506663806),.UNSPECIFIED.);
#335=B_SPLINE_CURVE_WITH_KNOTS('',3,(#11721,#11722,#11723,#11724,#11725,
#11726,#11727,#11728,#11729),.UNSPECIFIED.,.F.,.F.,(4,2,3,4),(0.,0.000802008422904852,
0.00160401684586607,0.00224980714452562),.UNSPECIFIED.);
#336=B_SPLINE_CURVE_WITH_KNOTS('',3,(#11731,#11732,#11733,#11734,#11735,
#11736),.UNSPECIFIED.,.F.,.F.,(4,2,4),(1.00000000468185E-6,1.2811788104379,
2.56201318882656),.UNSPECIFIED.);
#337=B_SPLINE_CURVE_WITH_KNOTS('',3,(#11743,#11744,#11745,#11746,#11747,
#11748,#11749),.UNSPECIFIED.,.F.,.F.,(4,1,2,4),(0.,0.000802008422543476,
0.00160401684508567,0.00313358895216331),.UNSPECIFIED.);
#338=B_SPLINE_CURVE_WITH_KNOTS('',3,(#12040,#12041,#12042,#12043,#12044,
#12045,#12046),.UNSPECIFIED.,.F.,.F.,(4,1,2,4),(0.,0.000802008422577623,
0.00160401684514919,0.00313695506663806),.UNSPECIFIED.);
#339=B_SPLINE_CURVE_WITH_KNOTS('',3,(#12047,#12048,#12049,#12050,#12051,
#12052,#12053,#12054,#12055),.UNSPECIFIED.,.F.,.F.,(4,2,3,4),(0.,0.000802008422906758,
0.00160401684587019,0.00313013376960513),.UNSPECIFIED.);
#340=B_SPLINE_CURVE_WITH_KNOTS('',3,(#12346,#12347,#12348,#12349,#12350,
#12351,#12352,#12353,#12354),.UNSPECIFIED.,.F.,.F.,(4,2,3,4),(0.,0.000802008422904855,
0.00160401684586608,0.00313011409353478),.UNSPECIFIED.);
#341=B_SPLINE_CURVE_WITH_KNOTS('',3,(#12355,#12356,#12357,#12358,#12359,
#12360,#12361),.UNSPECIFIED.,.F.,.F.,(4,1,2,4),(9.81307786677359E-18,0.000802008422543473,
0.00160401684508569,0.0031335889521633),.UNSPECIFIED.);
#342=B_SPLINE_CURVE_WITH_KNOTS('',3,(#12652,#12653,#12654,#12655,#12656,
#12657,#12658),.UNSPECIFIED.,.F.,.F.,(4,1,2,4),(0.,0.000802008422577623,
0.0016040168451492,0.00313695506663807),.UNSPECIFIED.);
#343=B_SPLINE_CURVE_WITH_KNOTS('',3,(#12659,#12660,#12661,#12662,#12663,
#12664,#12665,#12666,#12667),.UNSPECIFIED.,.F.,.F.,(4,2,3,4),(0.,0.000802008422906776,
0.00160401684587021,0.00313013376960513),.UNSPECIFIED.);
#344=B_SPLINE_CURVE_WITH_KNOTS('',3,(#12958,#12959,#12960,#12961,#12962,
#12963,#12964,#12965,#12966),.UNSPECIFIED.,.F.,.F.,(4,2,3,4),(0.,0.000802008422904862,
0.00160401684586608,0.00313011409353477),.UNSPECIFIED.);
#345=B_SPLINE_CURVE_WITH_KNOTS('',3,(#12967,#12968,#12969,#12970,#12971,
#12972,#12973),.UNSPECIFIED.,.F.,.F.,(4,1,2,4),(6.93889390390723E-18,0.000802008422543466,
0.00160401684508568,0.00313358895216331),.UNSPECIFIED.);
#346=B_SPLINE_CURVE_WITH_KNOTS('',3,(#13264,#13265,#13266,#13267,#13268,
#13269,#13270),.UNSPECIFIED.,.F.,.F.,(4,1,2,4),(0.,0.00080200842257763,
0.0016040168451492,0.00313695506663807),.UNSPECIFIED.);
#347=B_SPLINE_CURVE_WITH_KNOTS('',3,(#13271,#13272,#13273,#13274,#13275,
#13276,#13277,#13278,#13279),.UNSPECIFIED.,.F.,.F.,(4,2,3,4),(0.,0.000802008422906769,
0.0016040168458702,0.00313013376960513),.UNSPECIFIED.);
#348=B_SPLINE_CURVE_WITH_KNOTS('',3,(#13570,#13571,#13572,#13573,#13574,
#13575,#13576,#13577,#13578),.UNSPECIFIED.,.F.,.F.,(4,2,3,4),(0.,0.000802008422904853,
0.00160401684586608,0.00313011409353477),.UNSPECIFIED.);
#349=B_SPLINE_CURVE_WITH_KNOTS('',3,(#13579,#13580,#13581,#13582,#13583,
#13584,#13585),.UNSPECIFIED.,.F.,.F.,(4,1,2,4),(0.,0.000802008422543461,
0.00160401684508566,0.00313358895216331),.UNSPECIFIED.);
#350=B_SPLINE_CURVE_WITH_KNOTS('',3,(#14178,#14179,#14180,#14181,#14182,
#14183,#14184),.UNSPECIFIED.,.F.,.F.,(4,1,2,4),(6.93889390390723E-18,0.000802008422577189,
0.00160401684514838,0.00313692497239048),.UNSPECIFIED.);
#351=B_SPLINE_CURVE_WITH_KNOTS('',3,(#14475,#14476,#14477,#14478,#14479,
#14480,#14481),.UNSPECIFIED.,.F.,.F.,(4,1,2,4),(0.,0.000802008422543314,
0.0016040168450854,0.00313356353166786),.UNSPECIFIED.);
#352=B_SPLINE_CURVE_WITH_KNOTS('',3,(#14774,#14775,#14776,#14777,#14778,
#14779,#14780),.UNSPECIFIED.,.F.,.F.,(4,1,2,4),(0.,0.000802008422577183,
0.00160401684514837,0.00313692497239049),.UNSPECIFIED.);
#353=B_SPLINE_CURVE_WITH_KNOTS('',3,(#15071,#15072,#15073,#15074,#15075,
#15076,#15077),.UNSPECIFIED.,.F.,.F.,(4,1,2,4),(0.,0.000802008422543321,
0.0016040168450854,0.00313356353166786),.UNSPECIFIED.);
#354=B_SPLINE_CURVE_WITH_KNOTS('',3,(#15370,#15371,#15372,#15373,#15374,
#15375,#15376),.UNSPECIFIED.,.F.,.F.,(4,1,2,4),(9.81307786677359E-18,0.000802008422577179,
0.00160401684514837,0.0031369249723905),.UNSPECIFIED.);
#355=B_SPLINE_CURVE_WITH_KNOTS('',3,(#15667,#15668,#15669,#15670,#15671,
#15672,#15673),.UNSPECIFIED.,.F.,.F.,(4,1,2,4),(0.,0.00080200842254332,
0.0016040168450854,0.00313356353166787),.UNSPECIFIED.);
#356=B_SPLINE_CURVE_WITH_KNOTS('',3,(#15966,#15967,#15968,#15969,#15970,
#15971,#15972),.UNSPECIFIED.,.F.,.F.,(4,1,2,4),(0.,0.000802008422577182,
0.00160401684514837,0.00313692497239049),.UNSPECIFIED.);
#357=B_SPLINE_CURVE_WITH_KNOTS('',3,(#16263,#16264,#16265,#16266,#16267,
#16268,#16269),.UNSPECIFIED.,.F.,.F.,(4,1,2,4),(0.,0.000802008422543311,
0.00160401684508539,0.00313356353166786),.UNSPECIFIED.);
#358=B_SPLINE_CURVE_WITH_KNOTS('',3,(#16561,#16562,#16563,#16564,#16565,
#16566,#16567),.UNSPECIFIED.,.F.,.F.,(4,1,2,4),(0.,0.000802008422577623,
0.0016040168451492,0.00313695506663805),.UNSPECIFIED.);
#359=B_SPLINE_CURVE_WITH_KNOTS('',3,(#16568,#16569,#16570,#16571,#16572,
#16573,#16574,#16575,#16576),.UNSPECIFIED.,.F.,.F.,(4,2,3,4),(0.,0.000802008422906782,
0.00160401684587023,0.00313013376960512),.UNSPECIFIED.);
#360=B_SPLINE_CURVE_WITH_KNOTS('',3,(#16867,#16868,#16869,#16870,#16871,
#16872,#16873,#16874,#16875),.UNSPECIFIED.,.F.,.F.,(4,2,3,4),(0.,0.000802008422904849,
0.00160401684586607,0.00313011409353477),.UNSPECIFIED.);
#361=B_SPLINE_CURVE_WITH_KNOTS('',3,(#16876,#16877,#16878,#16879,#16880,
#16881),.UNSPECIFIED.,.F.,.F.,(4,2,4),(-0.322960607525434,-0.161416672138243,
0.),.UNSPECIFIED.);
#362=B_SPLINE_CURVE_WITH_KNOTS('',3,(#16949,#16950,#16951,#16952,#16953,
#16954,#16955,#16956,#16957,#16958,#16959,#16960,#16961,#16962,#16963,#16964),
 .UNSPECIFIED.,.F.,.F.,(4,3,3,3,3,4),(0.00869267220315778,0.00897347831546948,
0.00914767037620121,0.00934133695348868,0.00953512469214104,0.00960266854924464),
 .UNSPECIFIED.);
#363=B_SPLINE_CURVE_WITH_KNOTS('',3,(#16976,#16977,#16978,#16979,#16980,
#16981,#16982,#16983,#16984,#16985,#16986,#16987,#16988),.UNSPECIFIED.,
 .F.,.F.,(4,3,3,3,4),(0.014648624615312,0.0149251039211043,0.0151052218084313,
0.0153888521719278,0.0155618190015507),.UNSPECIFIED.);
#364=B_SPLINE_CURVE_WITH_KNOTS('',3,(#17007,#17008,#17009,#17010),
 .UNSPECIFIED.,.F.,.F.,(4,4),(-1.18244232933534,-1.12154327892906),
 .UNSPECIFIED.);
#365=B_SPLINE_CURVE_WITH_KNOTS('',3,(#17302,#17303,#17304,#17305,#17306,
#17307),.UNSPECIFIED.,.F.,.F.,(4,2,4),(-0.319108104097769,-0.159717462303668,
0.),.UNSPECIFIED.);
#366=B_SPLINE_CURVE_WITH_KNOTS('',3,(#17607,#17608,#17609,#17610,#17611,
#17612,#17613,#17614,#17615),.UNSPECIFIED.,.F.,.F.,(4,2,3,4),(0.,0.000802008422904865,
0.00160401684586611,0.00313011409353478),.UNSPECIFIED.);
#367=B_SPLINE_CURVE_WITH_KNOTS('',3,(#17616,#17617,#17618,#17619,#17620,
#17621,#17622),.UNSPECIFIED.,.F.,.F.,(4,1,2,4),(6.93889390390723E-18,0.000802008422543296,
0.00160401684508538,0.00313356353166788),.UNSPECIFIED.);
#368=B_SPLINE_CURVE_WITH_KNOTS('',3,(#17623,#17624,#17625,#17626,#17627,
#17628,#17629,#17630,#17631,#17632,#17633,#17634,#17635,#17636,#17637,#17638,
#17639,#17640,#17641,#17642,#17643,#17644,#17645,#17646,#17647,#17648,#17649,
#17650,#17651,#17652),.UNSPECIFIED.,.F.,.F.,(4,2,2,2,2,2,2,2,2,2,2,2,2,
2,4),(-0.422102272244324,-0.348146080556318,-0.281817985962111,-0.236711761741135,
-0.211595144460982,-0.211065138953951,-0.210876177667938,-0.210727417561504,
-0.210584548895218,-0.210388827790948,-0.209942749411974,-0.197138882545824,
-0.161673269341594,-0.105103214837917,0.),.UNSPECIFIED.);
#369=B_SPLINE_CURVE_WITH_KNOTS('',3,(#17960,#17961,#17962,#17963,#17964,
#17965),.UNSPECIFIED.,.F.,.F.,(4,2,4),(-0.280439425813684,-0.140217859912255,
0.),.UNSPECIFIED.);
#370=B_SPLINE_CURVE_WITH_KNOTS('',3,(#17966,#17967,#17968,#17969,#17970,
#17971,#17972),.UNSPECIFIED.,.F.,.F.,(4,1,2,4),(0.,0.00080200842257764,
0.00160401684514921,0.00313695506663809),.UNSPECIFIED.);
#371=B_SPLINE_CURVE_WITH_KNOTS('',3,(#18265,#18266,#18267,#18268,#18269,
#18270),.UNSPECIFIED.,.F.,.F.,(4,2,4),(-0.30638474699579,-0.153201892366487,
-9.99999968504403E-7),.UNSPECIFIED.);
#372=B_SPLINE_CURVE_WITH_KNOTS('',3,(#18286,#18287,#18288,#18289,#18290,
#18291,#18292,#18293,#18294,#18295,#18296,#18297,#18298,#18299,#18300,#18301,
#18302,#18303,#18304,#18305),.UNSPECIFIED.,.F.,.F.,(4,2,2,2,2,2,2,2,2,4),
(0.,0.623255442251575,1.23190737214536,2.44539704217141,2.79680652222767,
4.64794122889589,5.57465586747308,7.36134291536557,7.84478465660949,9.2535573537906),
 .UNSPECIFIED.);
#373=B_SPLINE_CURVE_WITH_KNOTS('',3,(#18318,#18319,#18320,#18321,#18322,
#18323),.UNSPECIFIED.,.F.,.F.,(4,2,4),(-0.420375087827024,-0.299144304587487,
-0.235961611475371),.UNSPECIFIED.);
#374=B_SPLINE_CURVE_WITH_KNOTS('',3,(#18360,#18361,#18362,#18363,#18364,
#18365),.UNSPECIFIED.,.F.,.F.,(4,2,4),(0.108137927283078,0.149564996746846,
0.157637941980081),.UNSPECIFIED.);
#375=B_SPLINE_CURVE_WITH_KNOTS('',3,(#18657,#18658,#18659,#18660,#18661,
#18662,#18663),.UNSPECIFIED.,.F.,.F.,(4,1,2,4),(0.,0.000802008422577636,
0.00160401684514921,0.00313695506663806),.UNSPECIFIED.);
#376=B_SPLINE_CURVE_WITH_KNOTS('',3,(#18665,#18666,#18667,#18668,#18669,
#18670,#18671,#18672,#18673,#18674,#18675,#18676,#18677,#18678,#18679,#18680,
#18681,#18682,#18683,#18684,#18685,#18686,#18687,#18688,#18689,#18690,#18691,
#18692,#18693,#18694,#18695,#18696,#18697,#18698,#18699,#18700,#18701,#18702),
 .UNSPECIFIED.,.F.,.F.,(4,2,2,2,2,2,2,2,2,2,2,2,2,2,2,2,2,2,4),(-0.728274932141156,
-0.62958437370879,-0.513230659588247,-0.435254656595599,-0.382758778659329,
-0.358199460630516,-0.35520801993891,-0.35357862650099,-0.353227607893641,
-0.353002007656128,-0.352824286806013,-0.352623194503785,-0.352288454767916,
-0.351064596075185,-0.343311205277017,-0.312348670606145,-0.254183071767702,
-0.170240832437228,0.),.UNSPECIFIED.);
#377=B_SPLINE_CURVE_WITH_KNOTS('',3,(#18993,#18994,#18995,#18996,#18997,
#18998,#18999),.UNSPECIFIED.,.F.,.F.,(4,1,2,4),(0.,0.000802008422543309,
0.00160401684508538,0.00313356353166786),.UNSPECIFIED.);
#378=B_SPLINE_CURVE_WITH_KNOTS('',3,(#19000,#19001,#19002,#19003,#19004,
#19005),.UNSPECIFIED.,.F.,.F.,(4,2,4),(-0.324384744695224,-0.162317646330996,
0.),.UNSPECIFIED.);
#379=B_SPLINE_CURVE_WITH_KNOTS('',3,(#19298,#19299,#19300,#19301,#19302,
#19303),.UNSPECIFIED.,.F.,.F.,(4,2,4),(-0.222197670544619,-0.111101699996788,
0.),.UNSPECIFIED.);
#380=B_SPLINE_CURVE_WITH_KNOTS('',3,(#19304,#19305,#19306,#19307,#19308,
#19309,#19310,#19311,#19312),.UNSPECIFIED.,.F.,.F.,(4,2,3,4),(0.,0.000802008422904865,
0.00160401684586609,0.00313011409353478),.UNSPECIFIED.);
#397=PLANE('',#3892);
#398=PLANE('',#3894);
#399=PLANE('',#3896);
#400=PLANE('',#3897);
#401=PLANE('',#3917);
#402=PLANE('',#3918);
#403=PLANE('',#3919);
#404=PLANE('',#3920);
#405=PLANE('',#3922);
#406=PLANE('',#3923);
#407=PLANE('',#3924);
#408=PLANE('',#3925);
#409=PLANE('',#3926);
#410=PLANE('',#3927);
#411=PLANE('',#3928);
#412=PLANE('',#3929);
#413=PLANE('',#3930);
#414=PLANE('',#3931);
#450=LINE('',#5017,#643);
#451=LINE('',#5023,#644);
#452=LINE('',#5047,#645);
#453=LINE('',#5097,#646);
#454=LINE('',#5120,#647);
#455=LINE('',#5124,#648);
#456=LINE('',#5145,#649);
#457=LINE('',#5149,#650);
#458=LINE('',#5164,#651);
#459=LINE('',#5178,#652);
#460=LINE('',#5182,#653);
#461=LINE('',#5203,#654);
#462=LINE('',#5206,#655);
#463=LINE('',#5210,#656);
#464=LINE('',#5220,#657);
#465=LINE('',#5231,#658);
#466=LINE('',#5255,#659);
#467=LINE('',#5265,#660);
#468=LINE('',#5276,#661);
#469=LINE('',#5286,#662);
#470=LINE('',#5297,#663);
#471=LINE('',#5307,#664);
#472=LINE('',#5318,#665);
#473=LINE('',#5328,#666);
#474=LINE('',#5339,#667);
#475=LINE('',#5349,#668);
#476=LINE('',#5360,#669);
#477=LINE('',#5370,#670);
#478=LINE('',#5381,#671);
#479=LINE('',#5391,#672);
#480=LINE('',#5402,#673);
#481=LINE('',#5412,#674);
#482=LINE('',#5417,#675);
#483=LINE('',#5427,#676);
#484=LINE('',#5438,#677);
#485=LINE('',#5448,#678);
#486=LINE('',#5459,#679);
#487=LINE('',#5469,#680);
#488=LINE('',#5480,#681);
#489=LINE('',#5490,#682);
#490=LINE('',#5501,#683);
#491=LINE('',#5511,#684);
#492=LINE('',#5522,#685);
#493=LINE('',#5532,#686);
#494=LINE('',#8030,#687);
#495=LINE('',#8334,#688);
#496=LINE('',#10866,#689);
#497=LINE('',#10867,#690);
#498=LINE('',#10870,#691);
#499=LINE('',#10879,#692);
#500=LINE('',#10890,#693);
#501=LINE('',#10891,#694);
#502=LINE('',#10894,#695);
#503=LINE('',#10903,#696);
#504=LINE('',#10914,#697);
#505=LINE('',#10915,#698);
#506=LINE('',#10918,#699);
#507=LINE('',#10927,#700);
#508=LINE('',#10938,#701);
#509=LINE('',#10939,#702);
#510=LINE('',#10942,#703);
#511=LINE('',#10951,#704);
#512=LINE('',#10954,#705);
#513=LINE('',#10963,#706);
#514=LINE('',#10966,#707);
#515=LINE('',#10975,#708);
#516=LINE('',#10986,#709);
#517=LINE('',#10987,#710);
#518=LINE('',#10990,#711);
#519=LINE('',#10999,#712);
#520=LINE('',#11010,#713);
#521=LINE('',#11011,#714);
#522=LINE('',#11014,#715);
#523=LINE('',#11023,#716);
#524=LINE('',#11034,#717);
#525=LINE('',#11035,#718);
#526=LINE('',#11038,#719);
#527=LINE('',#11048,#720);
#528=LINE('',#11063,#721);
#529=LINE('',#11064,#722);
#530=LINE('',#11076,#723);
#531=LINE('',#11090,#724);
#532=LINE('',#11102,#725);
#533=LINE('',#11428,#726);
#534=LINE('',#13877,#727);
#535=LINE('',#13886,#728);
#536=LINE('',#16883,#729);
#537=LINE('',#16886,#730);
#538=LINE('',#16888,#731);
#539=LINE('',#16891,#732);
#540=LINE('',#16893,#733);
#541=LINE('',#16895,#734);
#542=LINE('',#16898,#735);
#543=LINE('',#16899,#736);
#544=LINE('',#16901,#737);
#545=LINE('',#16902,#738);
#546=LINE('',#16906,#739);
#547=LINE('',#16922,#740);
#548=LINE('',#16939,#741);
#549=LINE('',#16974,#742);
#550=LINE('',#16998,#743);
#551=LINE('',#17959,#744);
#552=LINE('',#18272,#745);
#553=LINE('',#18317,#746);
#554=LINE('',#18340,#747);
#555=LINE('',#18341,#748);
#556=LINE('',#18344,#749);
#557=LINE('',#19297,#750);
#558=LINE('',#19314,#751);
#559=LINE('',#19315,#752);
#560=LINE('',#19316,#753);
#561=LINE('',#19317,#754);
#562=LINE('',#19319,#755);
#563=LINE('',#19320,#756);
#564=LINE('',#19323,#757);
#565=LINE('',#19324,#758);
#566=LINE('',#19326,#759);
#567=LINE('',#19328,#760);
#568=LINE('',#19330,#761);
#569=LINE('',#19331,#762);
#570=LINE('',#19339,#763);
#571=LINE('',#19340,#764);
#643=VECTOR('',#4171,40.);
#644=VECTOR('',#4178,46.);
#645=VECTOR('',#4187,40.);
#646=VECTOR('',#4198,1000.);
#647=VECTOR('',#4201,1000.);
#648=VECTOR('',#4204,1000.);
#649=VECTOR('',#4205,1000.);
#650=VECTOR('',#4208,10.);
#651=VECTOR('',#4209,36.);
#652=VECTOR('',#4212,1000.);
#653=VECTOR('',#4215,1000.);
#654=VECTOR('',#4216,1000.);
#655=VECTOR('',#4219,1000.);
#656=VECTOR('',#4222,1000.);
#657=VECTOR('',#4223,1000.);
#658=VECTOR('',#4226,1000.);
#659=VECTOR('',#4229,1000.);
#660=VECTOR('',#4230,1000.);
#661=VECTOR('',#4233,1000.);
#662=VECTOR('',#4234,1000.);
#663=VECTOR('',#4237,1000.);
#664=VECTOR('',#4238,1000.);
#665=VECTOR('',#4241,1000.);
#666=VECTOR('',#4242,1000.);
#667=VECTOR('',#4245,1000.);
#668=VECTOR('',#4246,1000.);
#669=VECTOR('',#4249,1000.);
#670=VECTOR('',#4250,1000.);
#671=VECTOR('',#4253,1000.);
#672=VECTOR('',#4254,1000.);
#673=VECTOR('',#4257,1000.);
#674=VECTOR('',#4258,1000.);
#675=VECTOR('',#4263,1000.);
#676=VECTOR('',#4264,1000.);
#677=VECTOR('',#4267,1000.);
#678=VECTOR('',#4268,1000.);
#679=VECTOR('',#4271,1000.);
#680=VECTOR('',#4272,1000.);
#681=VECTOR('',#4275,1000.);
#682=VECTOR('',#4276,1000.);
#683=VECTOR('',#4279,1000.);
#684=VECTOR('',#4280,1000.);
#685=VECTOR('',#4283,1000.);
#686=VECTOR('',#4284,1000.);
#687=VECTOR('',#4293,10.);
#688=VECTOR('',#4298,10.);
#689=VECTOR('',#4311,10.);
#690=VECTOR('',#4312,10.);
#691=VECTOR('',#4315,10.);
#692=VECTOR('',#4316,10.);
#693=VECTOR('',#4319,10.);
#694=VECTOR('',#4320,10.);
#695=VECTOR('',#4323,10.);
#696=VECTOR('',#4324,10.);
#697=VECTOR('',#4327,10.);
#698=VECTOR('',#4328,10.);
#699=VECTOR('',#4331,10.);
#700=VECTOR('',#4332,10.);
#701=VECTOR('',#4335,10.);
#702=VECTOR('',#4336,10.);
#703=VECTOR('',#4339,10.);
#704=VECTOR('',#4340,10.);
#705=VECTOR('',#4343,10.);
#706=VECTOR('',#4344,10.);
#707=VECTOR('',#4347,10.);
#708=VECTOR('',#4348,10.);
#709=VECTOR('',#4351,10.);
#710=VECTOR('',#4352,10.);
#711=VECTOR('',#4355,10.);
#712=VECTOR('',#4356,10.);
#713=VECTOR('',#4359,10.);
#714=VECTOR('',#4360,10.);
#715=VECTOR('',#4363,10.);
#716=VECTOR('',#4364,10.);
#717=VECTOR('',#4367,10.);
#718=VECTOR('',#4368,10.);
#719=VECTOR('',#4371,10.);
#720=VECTOR('',#4372,10.);
#721=VECTOR('',#4375,10.);
#722=VECTOR('',#4376,10.);
#723=VECTOR('',#4379,10.);
#724=VECTOR('',#4380,10.);
#725=VECTOR('',#4383,10.);
#726=VECTOR('',#4384,10.);
#727=VECTOR('',#4387,10.);
#728=VECTOR('',#4388,10.);
#729=VECTOR('',#4407,1000.);
#730=VECTOR('',#4410,1000.);
#731=VECTOR('',#4413,1000.);
#732=VECTOR('',#4416,1000.);
#733=VECTOR('',#4419,1000.);
#734=VECTOR('',#4420,1000.);
#735=VECTOR('',#4425,1000.);
#736=VECTOR('',#4426,1000.);
#737=VECTOR('',#4429,1000.);
#738=VECTOR('',#4430,1000.);
#739=VECTOR('',#4433,1000.);
#740=VECTOR('',#4434,1000.);
#741=VECTOR('',#4437,1000.);
#742=VECTOR('',#4440,1000.);
#743=VECTOR('',#4443,1000.);
#744=VECTOR('',#4446,10.);
#745=VECTOR('',#4447,10.);
#746=VECTOR('',#4452,10.);
#747=VECTOR('',#4455,10.);
#748=VECTOR('',#4456,10.);
#749=VECTOR('',#4459,10.);
#750=VECTOR('',#4464,10.);
#751=VECTOR('',#4467,1000.);
#752=VECTOR('',#4468,1000.);
#753=VECTOR('',#4469,1000.);
#754=VECTOR('',#4470,1000.);
#755=VECTOR('',#4473,1000.);
#756=VECTOR('',#4474,1000.);
#757=VECTOR('',#4477,1000.);
#758=VECTOR('',#4478,1000.);
#759=VECTOR('',#4481,1000.);
#760=VECTOR('',#4484,1000.);
#761=VECTOR('',#4487,1000.);
#762=VECTOR('',#4488,1000.);
#763=VECTOR('',#4503,1000.);
#764=VECTOR('',#4504,1000.);
#836=CYLINDRICAL_SURFACE('',#3814,40.);
#837=CYLINDRICAL_SURFACE('',#3817,46.);
#838=CYLINDRICAL_SURFACE('',#3820,40.);
#839=CYLINDRICAL_SURFACE('',#3825,46.);
#840=CYLINDRICAL_SURFACE('',#3828,36.);
#841=CYLINDRICAL_SURFACE('',#3834,46.);
#842=CYLINDRICAL_SURFACE('',#3835,46.);
#843=CYLINDRICAL_SURFACE('',#3836,46.);
#844=CYLINDRICAL_SURFACE('',#3837,46.);
#845=CYLINDRICAL_SURFACE('',#3838,46.);
#846=CYLINDRICAL_SURFACE('',#3839,46.);
#847=CYLINDRICAL_SURFACE('',#3840,46.);
#848=CYLINDRICAL_SURFACE('',#3841,46.);
#849=CYLINDRICAL_SURFACE('',#3842,46.);
#850=CYLINDRICAL_SURFACE('',#3843,46.);
#851=CYLINDRICAL_SURFACE('',#3845,46.);
#852=CYLINDRICAL_SURFACE('',#3846,46.);
#853=CYLINDRICAL_SURFACE('',#3847,46.);
#854=CYLINDRICAL_SURFACE('',#3848,46.);
#855=CYLINDRICAL_SURFACE('',#3849,46.);
#856=CYLINDRICAL_SURFACE('',#3850,46.);
#857=CYLINDRICAL_SURFACE('',#3862,48.7063293749999);
#858=CYLINDRICAL_SURFACE('',#3863,48.7063293749999);
#859=CYLINDRICAL_SURFACE('',#3864,48.7063293749999);
#860=CYLINDRICAL_SURFACE('',#3865,48.7063293749999);
#861=CYLINDRICAL_SURFACE('',#3866,48.7063293749999);
#862=CYLINDRICAL_SURFACE('',#3867,48.7063293749999);
#863=CYLINDRICAL_SURFACE('',#3868,48.7063293749999);
#864=CYLINDRICAL_SURFACE('',#3869,48.7063293749999);
#865=CYLINDRICAL_SURFACE('',#3870,48.7063293749999);
#866=CYLINDRICAL_SURFACE('',#3871,48.7063293749999);
#867=CYLINDRICAL_SURFACE('',#3872,48.7063293749999);
#868=CYLINDRICAL_SURFACE('',#3873,48.7063293749999);
#869=CYLINDRICAL_SURFACE('',#3874,48.7063293749999);
#870=CYLINDRICAL_SURFACE('',#3875,48.7063293749999);
#871=CYLINDRICAL_SURFACE('',#3876,48.7063293749999);
#872=CYLINDRICAL_SURFACE('',#3877,48.7063293749999);
#873=CYLINDRICAL_SURFACE('',#3878,48.7063293749999);
#874=CYLINDRICAL_SURFACE('',#3879,48.7063293749999);
#875=CYLINDRICAL_SURFACE('',#3880,48.7063293749999);
#876=CYLINDRICAL_SURFACE('',#3890,48.5805105169702);
#877=CYLINDRICAL_SURFACE('',#3898,46.);
#878=CYLINDRICAL_SURFACE('',#3899,46.);
#879=CYLINDRICAL_SURFACE('',#3900,46.);
#880=CYLINDRICAL_SURFACE('',#3901,46.);
#881=CYLINDRICAL_SURFACE('',#3904,48.7063293749999);
#882=CYLINDRICAL_SURFACE('',#3905,48.7063293749999);
#883=CYLINDRICAL_SURFACE('',#3906,48.7063293749999);
#884=CYLINDRICAL_SURFACE('',#3909,3.96875);
#885=CYLINDRICAL_SURFACE('',#3910,3.96875);
#886=CYLINDRICAL_SURFACE('',#3912,46.);
#887=CYLINDRICAL_SURFACE('',#3913,48.5805105169702);
#888=CYLINDRICAL_SURFACE('',#3914,3.96875);
#889=CYLINDRICAL_SURFACE('',#3915,46.);
#890=CYLINDRICAL_SURFACE('',#3921,3.96875);
#935=SHAPE_REPRESENTATION_RELATIONSHIP('SRR','None',#20719,#947);
#947=ADVANCED_BREP_SHAPE_REPRESENTATION('',(#971),#20649);
#959=STYLED_ITEM('',(#20786),#971);
#971=MANIFOLD_SOLID_BREP('Body1',#3654);
#987=FACE_OUTER_BOUND('',#1196,.T.);
#988=FACE_OUTER_BOUND('',#1197,.T.);
#989=FACE_OUTER_BOUND('',#1198,.T.);
#990=FACE_OUTER_BOUND('',#1199,.T.);
#991=FACE_OUTER_BOUND('',#1200,.T.);
#992=FACE_OUTER_BOUND('',#1201,.T.);
#993=FACE_OUTER_BOUND('',#1202,.T.);
#994=FACE_OUTER_BOUND('',#1203,.T.);
#995=FACE_OUTER_BOUND('',#1204,.T.);
#996=FACE_OUTER_BOUND('',#1205,.T.);
#997=FACE_OUTER_BOUND('',#1206,.T.);
#998=FACE_OUTER_BOUND('',#1207,.T.);
#999=FACE_OUTER_BOUND('',#1208,.T.);
#1000=FACE_OUTER_BOUND('',#1209,.T.);
#1001=FACE_OUTER_BOUND('',#1210,.T.);
#1002=FACE_OUTER_BOUND('',#1211,.T.);
#1003=FACE_OUTER_BOUND('',#1212,.T.);
#1004=FACE_OUTER_BOUND('',#1213,.T.);
#1005=FACE_OUTER_BOUND('',#1214,.T.);
#1006=FACE_OUTER_BOUND('',#1215,.T.);
#1007=FACE_OUTER_BOUND('',#1216,.T.);
#1008=FACE_OUTER_BOUND('',#1217,.T.);
#1009=FACE_OUTER_BOUND('',#1218,.T.);
#1010=FACE_OUTER_BOUND('',#1219,.T.);
#1011=FACE_OUTER_BOUND('',#1220,.T.);
#1012=FACE_OUTER_BOUND('',#1221,.T.);
#1013=FACE_OUTER_BOUND('',#1222,.T.);
#1014=FACE_OUTER_BOUND('',#1223,.T.);
#1015=FACE_OUTER_BOUND('',#1224,.T.);
#1016=FACE_OUTER_BOUND('',#1225,.T.);
#1017=FACE_OUTER_BOUND('',#1226,.T.);
#1018=FACE_OUTER_BOUND('',#1227,.T.);
#1019=FACE_OUTER_BOUND('',#1228,.T.);
#1020=FACE_OUTER_BOUND('',#1229,.T.);
#1021=FACE_OUTER_BOUND('',#1230,.T.);
#1022=FACE_OUTER_BOUND('',#1231,.T.);
#1023=FACE_OUTER_BOUND('',#1232,.T.);
#1024=FACE_OUTER_BOUND('',#1233,.T.);
#1025=FACE_OUTER_BOUND('',#1234,.T.);
#1026=FACE_OUTER_BOUND('',#1235,.T.);
#1027=FACE_OUTER_BOUND('',#1236,.T.);
#1028=FACE_OUTER_BOUND('',#1237,.T.);
#1029=FACE_OUTER_BOUND('',#1238,.T.);
#1030=FACE_OUTER_BOUND('',#1239,.T.);
#1031=FACE_OUTER_BOUND('',#1240,.T.);
#1032=FACE_OUTER_BOUND('',#1241,.T.);
#1033=FACE_OUTER_BOUND('',#1242,.T.);
#1034=FACE_OUTER_BOUND('',#1243,.T.);
#1035=FACE_OUTER_BOUND('',#1244,.T.);
#1036=FACE_OUTER_BOUND('',#1245,.T.);
#1037=FACE_OUTER_BOUND('',#1246,.T.);
#1038=FACE_OUTER_BOUND('',#1247,.T.);
#1039=FACE_OUTER_BOUND('',#1248,.T.);
#1040=FACE_OUTER_BOUND('',#1249,.T.);
#1041=FACE_OUTER_BOUND('',#1250,.T.);
#1042=FACE_OUTER_BOUND('',#1251,.T.);
#1043=FACE_OUTER_BOUND('',#1252,.T.);
#1044=FACE_OUTER_BOUND('',#1253,.T.);
#1045=FACE_OUTER_BOUND('',#1254,.T.);
#1046=FACE_OUTER_BOUND('',#1255,.T.);
#1047=FACE_OUTER_BOUND('',#1256,.T.);
#1048=FACE_OUTER_BOUND('',#1257,.T.);
#1049=FACE_OUTER_BOUND('',#1258,.T.);
#1050=FACE_OUTER_BOUND('',#1259,.T.);
#1051=FACE_OUTER_BOUND('',#1260,.T.);
#1052=FACE_OUTER_BOUND('',#1261,.T.);
#1053=FACE_OUTER_BOUND('',#1262,.T.);
#1054=FACE_OUTER_BOUND('',#1263,.T.);
#1055=FACE_OUTER_BOUND('',#1264,.T.);
#1056=FACE_OUTER_BOUND('',#1265,.T.);
#1057=FACE_OUTER_BOUND('',#1266,.T.);
#1058=FACE_OUTER_BOUND('',#1267,.T.);
#1059=FACE_OUTER_BOUND('',#1268,.T.);
#1060=FACE_OUTER_BOUND('',#1269,.T.);
#1061=FACE_OUTER_BOUND('',#1270,.T.);
#1062=FACE_OUTER_BOUND('',#1271,.T.);
#1063=FACE_OUTER_BOUND('',#1272,.T.);
#1064=FACE_OUTER_BOUND('',#1273,.T.);
#1065=FACE_OUTER_BOUND('',#1274,.T.);
#1066=FACE_OUTER_BOUND('',#1275,.T.);
#1067=FACE_OUTER_BOUND('',#1276,.T.);
#1068=FACE_OUTER_BOUND('',#1277,.T.);
#1069=FACE_OUTER_BOUND('',#1278,.T.);
#1070=FACE_OUTER_BOUND('',#1279,.T.);
#1071=FACE_OUTER_BOUND('',#1280,.T.);
#1072=FACE_OUTER_BOUND('',#1281,.T.);
#1073=FACE_OUTER_BOUND('',#1282,.T.);
#1074=FACE_OUTER_BOUND('',#1283,.T.);
#1075=FACE_OUTER_BOUND('',#1284,.T.);
#1076=FACE_OUTER_BOUND('',#1285,.T.);
#1077=FACE_OUTER_BOUND('',#1286,.T.);
#1078=FACE_OUTER_BOUND('',#1287,.T.);
#1079=FACE_OUTER_BOUND('',#1288,.T.);
#1080=FACE_OUTER_BOUND('',#1289,.T.);
#1081=FACE_OUTER_BOUND('',#1290,.T.);
#1082=FACE_OUTER_BOUND('',#1291,.T.);
#1083=FACE_OUTER_BOUND('',#1292,.T.);
#1084=FACE_OUTER_BOUND('',#1293,.T.);
#1085=FACE_OUTER_BOUND('',#1294,.T.);
#1086=FACE_OUTER_BOUND('',#1295,.T.);
#1087=FACE_OUTER_BOUND('',#1296,.T.);
#1088=FACE_OUTER_BOUND('',#1297,.T.);
#1089=FACE_OUTER_BOUND('',#1298,.T.);
#1090=FACE_OUTER_BOUND('',#1299,.T.);
#1091=FACE_OUTER_BOUND('',#1301,.T.);
#1092=FACE_OUTER_BOUND('',#1303,.T.);
#1093=FACE_OUTER_BOUND('',#1304,.T.);
#1094=FACE_OUTER_BOUND('',#1305,.T.);
#1095=FACE_OUTER_BOUND('',#1306,.T.);
#1096=FACE_OUTER_BOUND('',#1307,.T.);
#1097=FACE_OUTER_BOUND('',#1308,.T.);
#1098=FACE_OUTER_BOUND('',#1309,.T.);
#1099=FACE_OUTER_BOUND('',#1310,.T.);
#1100=FACE_OUTER_BOUND('',#1311,.T.);
#1101=FACE_OUTER_BOUND('',#1312,.T.);
#1102=FACE_OUTER_BOUND('',#1313,.T.);
#1196=EDGE_LOOP('',(#2418,#2419,#2420,#2421));
#1197=EDGE_LOOP('',(#2422,#2423,#2424,#2425));
#1198=EDGE_LOOP('',(#2426,#2427,#2428,#2429,#2430,#2431,#2432,#2433));
#1199=EDGE_LOOP('',(#2434,#2435,#2436,#2437,#2438));
#1200=EDGE_LOOP('',(#2439,#2440,#2441,#2442,#2443,#2444,#2445,#2446,#2447,
#2448,#2449,#2450,#2451,#2452,#2453,#2454,#2455,#2456,#2457,#2458));
#1201=EDGE_LOOP('',(#2459,#2460,#2461,#2462));
#1202=EDGE_LOOP('',(#2463,#2464,#2465,#2466));
#1203=EDGE_LOOP('',(#2467,#2468,#2469,#2470));
#1204=EDGE_LOOP('',(#2471,#2472,#2473,#2474));
#1205=EDGE_LOOP('',(#2475,#2476,#2477,#2478));
#1206=EDGE_LOOP('',(#2479,#2480,#2481,#2482));
#1207=EDGE_LOOP('',(#2483,#2484,#2485,#2486));
#1208=EDGE_LOOP('',(#2487,#2488,#2489,#2490));
#1209=EDGE_LOOP('',(#2491,#2492,#2493,#2494));
#1210=EDGE_LOOP('',(#2495,#2496,#2497,#2498));
#1211=EDGE_LOOP('',(#2499,#2500,#2501,#2502));
#1212=EDGE_LOOP('',(#2503,#2504,#2505,#2506));
#1213=EDGE_LOOP('',(#2507,#2508,#2509,#2510));
#1214=EDGE_LOOP('',(#2511,#2512,#2513,#2514));
#1215=EDGE_LOOP('',(#2515,#2516,#2517,#2518));
#1216=EDGE_LOOP('',(#2519,#2520,#2521,#2522));
#1217=EDGE_LOOP('',(#2523,#2524,#2525,#2526));
#1218=EDGE_LOOP('',(#2527,#2528,#2529,#2530));
#1219=EDGE_LOOP('',(#2531,#2532,#2533,#2534));
#1220=EDGE_LOOP('',(#2535,#2536,#2537,#2538));
#1221=EDGE_LOOP('',(#2539,#2540,#2541,#2542));
#1222=EDGE_LOOP('',(#2543,#2544,#2545,#2546));
#1223=EDGE_LOOP('',(#2547,#2548,#2549,#2550));
#1224=EDGE_LOOP('',(#2551,#2552,#2553,#2554,#2555));
#1225=EDGE_LOOP('',(#2556,#2557,#2558,#2559,#2560,#2561,#2562));
#1226=EDGE_LOOP('',(#2563,#2564,#2565,#2566));
#1227=EDGE_LOOP('',(#2567,#2568,#2569,#2570));
#1228=EDGE_LOOP('',(#2571,#2572,#2573,#2574));
#1229=EDGE_LOOP('',(#2575,#2576,#2577,#2578));
#1230=EDGE_LOOP('',(#2579,#2580,#2581,#2582));
#1231=EDGE_LOOP('',(#2583,#2584,#2585,#2586));
#1232=EDGE_LOOP('',(#2587,#2588,#2589,#2590));
#1233=EDGE_LOOP('',(#2591,#2592,#2593,#2594,#2595));
#1234=EDGE_LOOP('',(#2596,#2597,#2598,#2599));
#1235=EDGE_LOOP('',(#2600,#2601,#2602,#2603));
#1236=EDGE_LOOP('',(#2604,#2605,#2606,#2607));
#1237=EDGE_LOOP('',(#2608,#2609,#2610,#2611));
#1238=EDGE_LOOP('',(#2612,#2613,#2614,#2615));
#1239=EDGE_LOOP('',(#2616,#2617,#2618,#2619));
#1240=EDGE_LOOP('',(#2620,#2621,#2622,#2623));
#1241=EDGE_LOOP('',(#2624,#2625,#2626,#2627));
#1242=EDGE_LOOP('',(#2628,#2629,#2630,#2631));
#1243=EDGE_LOOP('',(#2632,#2633,#2634,#2635));
#1244=EDGE_LOOP('',(#2636,#2637,#2638,#2639));
#1245=EDGE_LOOP('',(#2640,#2641,#2642,#2643));
#1246=EDGE_LOOP('',(#2644,#2645,#2646,#2647));
#1247=EDGE_LOOP('',(#2648,#2649,#2650,#2651));
#1248=EDGE_LOOP('',(#2652,#2653,#2654,#2655));
#1249=EDGE_LOOP('',(#2656,#2657,#2658,#2659,#2660));
#1250=EDGE_LOOP('',(#2661,#2662,#2663,#2664));
#1251=EDGE_LOOP('',(#2665,#2666,#2667,#2668,#2669));
#1252=EDGE_LOOP('',(#2670,#2671,#2672,#2673));
#1253=EDGE_LOOP('',(#2674,#2675,#2676,#2677,#2678));
#1254=EDGE_LOOP('',(#2679,#2680,#2681,#2682,#2683));
#1255=EDGE_LOOP('',(#2684,#2685,#2686,#2687));
#1256=EDGE_LOOP('',(#2688,#2689,#2690,#2691));
#1257=EDGE_LOOP('',(#2692,#2693,#2694,#2695));
#1258=EDGE_LOOP('',(#2696,#2697,#2698,#2699));
#1259=EDGE_LOOP('',(#2700,#2701,#2702,#2703));
#1260=EDGE_LOOP('',(#2704,#2705,#2706,#2707));
#1261=EDGE_LOOP('',(#2708,#2709,#2710,#2711));
#1262=EDGE_LOOP('',(#2712,#2713,#2714,#2715));
#1263=EDGE_LOOP('',(#2716,#2717,#2718,#2719));
#1264=EDGE_LOOP('',(#2720,#2721,#2722,#2723));
#1265=EDGE_LOOP('',(#2724,#2725,#2726,#2727));
#1266=EDGE_LOOP('',(#2728,#2729,#2730,#2731));
#1267=EDGE_LOOP('',(#2732,#2733,#2734,#2735));
#1268=EDGE_LOOP('',(#2736,#2737,#2738,#2739));
#1269=EDGE_LOOP('',(#2740,#2741,#2742,#2743));
#1270=EDGE_LOOP('',(#2744,#2745,#2746,#2747));
#1271=EDGE_LOOP('',(#2748,#2749,#2750,#2751));
#1272=EDGE_LOOP('',(#2752,#2753,#2754,#2755,#2756));
#1273=EDGE_LOOP('',(#2757,#2758,#2759,#2760,#2761));
#1274=EDGE_LOOP('',(#2762,#2763,#2764,#2765,#2766));
#1275=EDGE_LOOP('',(#2767,#2768,#2769,#2770,#2771));
#1276=EDGE_LOOP('',(#2772,#2773,#2774,#2775));
#1277=EDGE_LOOP('',(#2776,#2777,#2778,#2779));
#1278=EDGE_LOOP('',(#2780,#2781,#2782,#2783));
#1279=EDGE_LOOP('',(#2784,#2785,#2786,#2787));
#1280=EDGE_LOOP('',(#2788,#2789,#2790,#2791));
#1281=EDGE_LOOP('',(#2792,#2793,#2794,#2795));
#1282=EDGE_LOOP('',(#2796,#2797,#2798,#2799,#2800,#2801));
#1283=EDGE_LOOP('',(#2802,#2803,#2804,#2805,#2806));
#1284=EDGE_LOOP('',(#2807,#2808,#2809,#2810,#2811));
#1285=EDGE_LOOP('',(#2812,#2813,#2814,#2815));
#1286=EDGE_LOOP('',(#2816,#2817,#2818,#2819));
#1287=EDGE_LOOP('',(#2820,#2821,#2822,#2823,#2824));
#1288=EDGE_LOOP('',(#2825,#2826,#2827,#2828,#2829,#2830));
#1289=EDGE_LOOP('',(#2831,#2832,#2833,#2834));
#1290=EDGE_LOOP('',(#2835,#2836,#2837,#2838,#2839));
#1291=EDGE_LOOP('',(#2840,#2841,#2842,#2843,#2844,#2845,#2846,#2847,#2848));
#1292=EDGE_LOOP('',(#2849,#2850,#2851,#2852,#2853,#2854,#2855,#2856,#2857,
#2858));
#1293=EDGE_LOOP('',(#2859,#2860,#2861));
#1294=EDGE_LOOP('',(#2862,#2863,#2864));
#1295=EDGE_LOOP('',(#2865,#2866,#2867,#2868,#2869,#2870,#2871,#2872,#2873,
#2874));
#1296=EDGE_LOOP('',(#2875,#2876,#2877));
#1297=EDGE_LOOP('',(#2878,#2879,#2880,#2881,#2882,#2883));
#1298=EDGE_LOOP('',(#2884,#2885,#2886,#2887,#2888));
#1299=EDGE_LOOP('',(#2889));
#1300=EDGE_LOOP('',(#2890));
#1301=EDGE_LOOP('',(#2891));
#1302=EDGE_LOOP('',(#2892));
#1303=EDGE_LOOP('',(#2893,#2894,#2895,#2896,#2897,#2898,#2899,#2900,#2901,
#2902,#2903,#2904,#2905));
#1304=EDGE_LOOP('',(#2906,#2907,#2908,#2909,#2910,#2911,#2912,#2913,#2914,
#2915,#2916,#2917,#2918,#2919,#2920,#2921,#2922,#2923,#2924,#2925,#2926,
#2927));
#1305=EDGE_LOOP('',(#2928,#2929,#2930,#2931,#2932,#2933,#2934,#2935,#2936,
#2937,#2938,#2939,#2940,#2941,#2942,#2943,#2944,#2945,#2946,#2947,#2948,
#2949));
#1306=EDGE_LOOP('',(#2950,#2951,#2952,#2953,#2954,#2955,#2956,#2957,#2958,
#2959,#2960,#2961,#2962,#2963,#2964,#2965,#2966,#2967,#2968));
#1307=EDGE_LOOP('',(#2969,#2970,#2971,#2972,#2973,#2974,#2975,#2976,#2977,
#2978,#2979,#2980,#2981,#2982,#2983,#2984,#2985,#2986,#2987));
#1308=EDGE_LOOP('',(#2988,#2989,#2990,#2991,#2992,#2993,#2994,#2995,#2996,
#2997,#2998,#2999,#3000,#3001,#3002,#3003,#3004,#3005,#3006,#3007,#3008,
#3009,#3010,#3011,#3012,#3013));
#1309=EDGE_LOOP('',(#3014,#3015,#3016,#3017,#3018,#3019,#3020,#3021,#3022,
#3023,#3024,#3025,#3026,#3027,#3028,#3029,#3030,#3031,#3032,#3033,#3034,
#3035,#3036,#3037,#3038,#3039));
#1310=EDGE_LOOP('',(#3040,#3041,#3042,#3043,#3044,#3045,#3046,#3047,#3048,
#3049,#3050,#3051,#3052,#3053,#3054,#3055,#3056,#3057,#3058,#3059,#3060,
#3061,#3062,#3063,#3064));
#1311=EDGE_LOOP('',(#3065,#3066,#3067,#3068,#3069,#3070,#3071,#3072,#3073,
#3074,#3075,#3076,#3077,#3078,#3079,#3080,#3081,#3082,#3083,#3084,#3085,
#3086,#3087,#3088,#3089));
#1312=EDGE_LOOP('',(#3090,#3091,#3092,#3093));
#1313=EDGE_LOOP('',(#3094));
#1314=EDGE_LOOP('',(#3095));
#1427=CIRCLE('',#3815,40.);
#1428=CIRCLE('',#3816,40.);
#1429=CIRCLE('',#3818,46.);
#1430=CIRCLE('',#3819,46.);
#1431=CIRCLE('',#3821,40.);
#1432=CIRCLE('',#3822,40.);
#1433=CIRCLE('',#3823,40.);
#1434=CIRCLE('',#3824,40.);
#1435=CIRCLE('',#3826,3.96373117189689);
#1436=CIRCLE('',#3827,46.);
#1437=CIRCLE('',#3829,36.);
#1438=CIRCLE('',#3830,36.);
#1439=CIRCLE('',#3831,36.);
#1440=CIRCLE('',#3832,36.);
#1441=CIRCLE('',#3833,36.);
#1442=CIRCLE('',#3844,46.);
#1443=CIRCLE('',#3851,9169.15281567978);
#1444=CIRCLE('',#3852,9169.15281635233);
#1445=CIRCLE('',#3853,9169.15281632149);
#1446=CIRCLE('',#3854,9169.15281507871);
#1447=CIRCLE('',#3855,48.723191004622);
#1448=CIRCLE('',#3856,48.5934304680711);
#1449=CIRCLE('',#3857,9189.55754674609);
#1450=CIRCLE('',#3858,9189.55754816358);
#1451=CIRCLE('',#3859,9189.5575479708);
#1452=CIRCLE('',#3860,9189.55754886945);
#1453=CIRCLE('',#3861,15.8748636894354);
#1454=CIRCLE('',#3881,48.5937195834179);
#1455=CIRCLE('',#3882,9169.15281371648);
#1456=CIRCLE('',#3883,9189.55754697953);
#1457=CIRCLE('',#3884,9169.15281729791);
#1458=CIRCLE('',#3885,9189.55754810571);
#1459=CIRCLE('',#3886,9169.15281617656);
#1460=CIRCLE('',#3887,9189.55754697953);
#1461=CIRCLE('',#3888,9169.15281646739);
#1462=CIRCLE('',#3889,9189.55754853012);
#1463=CIRCLE('',#3891,48.5805105169702);
#1464=CIRCLE('',#3893,48.5805105169702);
#1465=CIRCLE('',#3895,46.);
#1466=CIRCLE('',#3902,9169.15281622634);
#1467=CIRCLE('',#3903,46.0136265696391);
#1468=CIRCLE('',#3907,48.7063293750001);
#1469=CIRCLE('',#3908,9169.15281512294);
#1470=CIRCLE('',#3916,46.);
#1551=VERTEX_POINT('',#5014);
#1552=VERTEX_POINT('',#5016);
#1553=VERTEX_POINT('',#5020);
#1554=VERTEX_POINT('',#5022);
#1555=VERTEX_POINT('',#5026);
#1556=VERTEX_POINT('',#5027);
#1557=VERTEX_POINT('',#5029);
#1558=VERTEX_POINT('',#5044);
#1559=VERTEX_POINT('',#5046);
#1560=VERTEX_POINT('',#5049);
#1561=VERTEX_POINT('',#5066);
#1562=VERTEX_POINT('',#5067);
#1563=VERTEX_POINT('',#5086);
#1564=VERTEX_POINT('',#5088);
#1565=VERTEX_POINT('',#5090);
#1566=VERTEX_POINT('',#5099);
#1567=VERTEX_POINT('',#5100);
#1568=VERTEX_POINT('',#5119);
#1569=VERTEX_POINT('',#5121);
#1570=VERTEX_POINT('',#5123);
#1571=VERTEX_POINT('',#5125);
#1572=VERTEX_POINT('',#5144);
#1573=VERTEX_POINT('',#5146);
#1574=VERTEX_POINT('',#5148);
#1575=VERTEX_POINT('',#5150);
#1576=VERTEX_POINT('',#5163);
#1577=VERTEX_POINT('',#5166);
#1578=VERTEX_POINT('',#5177);
#1579=VERTEX_POINT('',#5179);
#1580=VERTEX_POINT('',#5181);
#1581=VERTEX_POINT('',#5183);
#1582=VERTEX_POINT('',#5202);
#1583=VERTEX_POINT('',#5204);
#1584=VERTEX_POINT('',#5208);
#1585=VERTEX_POINT('',#5209);
#1586=VERTEX_POINT('',#5211);
#1587=VERTEX_POINT('',#5219);
#1588=VERTEX_POINT('',#5229);
#1589=VERTEX_POINT('',#5230);
#1590=VERTEX_POINT('',#5232);
#1591=VERTEX_POINT('',#5240);
#1592=VERTEX_POINT('',#5253);
#1593=VERTEX_POINT('',#5254);
#1594=VERTEX_POINT('',#5256);
#1595=VERTEX_POINT('',#5264);
#1596=VERTEX_POINT('',#5274);
#1597=VERTEX_POINT('',#5275);
#1598=VERTEX_POINT('',#5277);
#1599=VERTEX_POINT('',#5285);
#1600=VERTEX_POINT('',#5295);
#1601=VERTEX_POINT('',#5296);
#1602=VERTEX_POINT('',#5298);
#1603=VERTEX_POINT('',#5306);
#1604=VERTEX_POINT('',#5316);
#1605=VERTEX_POINT('',#5317);
#1606=VERTEX_POINT('',#5319);
#1607=VERTEX_POINT('',#5327);
#1608=VERTEX_POINT('',#5337);
#1609=VERTEX_POINT('',#5338);
#1610=VERTEX_POINT('',#5340);
#1611=VERTEX_POINT('',#5348);
#1612=VERTEX_POINT('',#5358);
#1613=VERTEX_POINT('',#5359);
#1614=VERTEX_POINT('',#5361);
#1615=VERTEX_POINT('',#5369);
#1616=VERTEX_POINT('',#5379);
#1617=VERTEX_POINT('',#5380);
#1618=VERTEX_POINT('',#5382);
#1619=VERTEX_POINT('',#5390);
#1620=VERTEX_POINT('',#5400);
#1621=VERTEX_POINT('',#5401);
#1622=VERTEX_POINT('',#5403);
#1623=VERTEX_POINT('',#5411);
#1624=VERTEX_POINT('',#5415);
#1625=VERTEX_POINT('',#5416);
#1626=VERTEX_POINT('',#5418);
#1627=VERTEX_POINT('',#5426);
#1628=VERTEX_POINT('',#5436);
#1629=VERTEX_POINT('',#5437);
#1630=VERTEX_POINT('',#5439);
#1631=VERTEX_POINT('',#5447);
#1632=VERTEX_POINT('',#5457);
#1633=VERTEX_POINT('',#5458);
#1634=VERTEX_POINT('',#5460);
#1635=VERTEX_POINT('',#5468);
#1636=VERTEX_POINT('',#5478);
#1637=VERTEX_POINT('',#5479);
#1638=VERTEX_POINT('',#5481);
#1639=VERTEX_POINT('',#5489);
#1640=VERTEX_POINT('',#5499);
#1641=VERTEX_POINT('',#5500);
#1642=VERTEX_POINT('',#5502);
#1643=VERTEX_POINT('',#5510);
#1644=VERTEX_POINT('',#5520);
#1645=VERTEX_POINT('',#5521);
#1646=VERTEX_POINT('',#5523);
#1647=VERTEX_POINT('',#5531);
#1648=VERTEX_POINT('',#5830);
#1649=VERTEX_POINT('',#5831);
#1650=VERTEX_POINT('',#6137);
#1651=VERTEX_POINT('',#6145);
#1652=VERTEX_POINT('',#6452);
#1653=VERTEX_POINT('',#6453);
#1654=VERTEX_POINT('',#6759);
#1655=VERTEX_POINT('',#6767);
#1656=VERTEX_POINT('',#7074);
#1657=VERTEX_POINT('',#7075);
#1658=VERTEX_POINT('',#7381);
#1659=VERTEX_POINT('',#7389);
#1660=VERTEX_POINT('',#7696);
#1661=VERTEX_POINT('',#7697);
#1662=VERTEX_POINT('',#8003);
#1663=VERTEX_POINT('',#8011);
#1664=VERTEX_POINT('',#8019);
#1665=VERTEX_POINT('',#8321);
#1666=VERTEX_POINT('',#8329);
#1667=VERTEX_POINT('',#8331);
#1668=VERTEX_POINT('',#8333);
#1669=VERTEX_POINT('',#8335);
#1670=VERTEX_POINT('',#8634);
#1671=VERTEX_POINT('',#8642);
#1672=VERTEX_POINT('',#8941);
#1673=VERTEX_POINT('',#8942);
#1674=VERTEX_POINT('',#9256);
#1675=VERTEX_POINT('',#9264);
#1676=VERTEX_POINT('',#9563);
#1677=VERTEX_POINT('',#9564);
#1678=VERTEX_POINT('',#9878);
#1679=VERTEX_POINT('',#9886);
#1680=VERTEX_POINT('',#10185);
#1681=VERTEX_POINT('',#10186);
#1682=VERTEX_POINT('',#10500);
#1683=VERTEX_POINT('',#10501);
#1684=VERTEX_POINT('',#10509);
#1685=VERTEX_POINT('',#10517);
#1686=VERTEX_POINT('',#10821);
#1687=VERTEX_POINT('',#10822);
#1688=VERTEX_POINT('',#10830);
#1689=VERTEX_POINT('',#10840);
#1690=VERTEX_POINT('',#10848);
#1691=VERTEX_POINT('',#10857);
#1692=VERTEX_POINT('',#10858);
#1693=VERTEX_POINT('',#10869);
#1694=VERTEX_POINT('',#10871);
#1695=VERTEX_POINT('',#10881);
#1696=VERTEX_POINT('',#10882);
#1697=VERTEX_POINT('',#10893);
#1698=VERTEX_POINT('',#10895);
#1699=VERTEX_POINT('',#10905);
#1700=VERTEX_POINT('',#10906);
#1701=VERTEX_POINT('',#10917);
#1702=VERTEX_POINT('',#10919);
#1703=VERTEX_POINT('',#10929);
#1704=VERTEX_POINT('',#10930);
#1705=VERTEX_POINT('',#10941);
#1706=VERTEX_POINT('',#10943);
#1707=VERTEX_POINT('',#10953);
#1708=VERTEX_POINT('',#10955);
#1709=VERTEX_POINT('',#10965);
#1710=VERTEX_POINT('',#10967);
#1711=VERTEX_POINT('',#10977);
#1712=VERTEX_POINT('',#10978);
#1713=VERTEX_POINT('',#10989);
#1714=VERTEX_POINT('',#10991);
#1715=VERTEX_POINT('',#11001);
#1716=VERTEX_POINT('',#11002);
#1717=VERTEX_POINT('',#11013);
#1718=VERTEX_POINT('',#11015);
#1719=VERTEX_POINT('',#11025);
#1720=VERTEX_POINT('',#11026);
#1721=VERTEX_POINT('',#11037);
#1722=VERTEX_POINT('',#11039);
#1723=VERTEX_POINT('',#11047);
#1724=VERTEX_POINT('',#11054);
#1725=VERTEX_POINT('',#11055);
#1726=VERTEX_POINT('',#11066);
#1727=VERTEX_POINT('',#11067);
#1728=VERTEX_POINT('',#11075);
#1729=VERTEX_POINT('',#11077);
#1730=VERTEX_POINT('',#11085);
#1731=VERTEX_POINT('',#11092);
#1732=VERTEX_POINT('',#11093);
#1733=VERTEX_POINT('',#11101);
#1734=VERTEX_POINT('',#11103);
#1735=VERTEX_POINT('',#11407);
#1736=VERTEX_POINT('',#11408);
#1737=VERTEX_POINT('',#11427);
#1738=VERTEX_POINT('',#11720);
#1739=VERTEX_POINT('',#11730);
#1740=VERTEX_POINT('',#11737);
#1741=VERTEX_POINT('',#13876);
#1742=VERTEX_POINT('',#13878);
#1743=VERTEX_POINT('',#16884);
#1744=VERTEX_POINT('',#16889);
#1745=VERTEX_POINT('',#16894);
#1746=VERTEX_POINT('',#16904);
#1747=VERTEX_POINT('',#16905);
#1748=VERTEX_POINT('',#16907);
#1749=VERTEX_POINT('',#16921);
#1750=VERTEX_POINT('',#16937);
#1751=VERTEX_POINT('',#16938);
#1752=VERTEX_POINT('',#16940);
#1753=VERTEX_POINT('',#16948);
#1754=VERTEX_POINT('',#16973);
#1755=VERTEX_POINT('',#16975);
#1756=VERTEX_POINT('',#16997);
#1757=VERTEX_POINT('',#16999);
#1758=VERTEX_POINT('',#17598);
#1759=VERTEX_POINT('',#17599);
#1760=VERTEX_POINT('',#17943);
#1761=VERTEX_POINT('',#17944);
#1762=VERTEX_POINT('',#17958);
#1763=VERTEX_POINT('',#18263);
#1764=VERTEX_POINT('',#18264);
#1765=VERTEX_POINT('',#18271);
#1766=VERTEX_POINT('',#18273);
#1767=VERTEX_POINT('',#18285);
#1768=VERTEX_POINT('',#18308);
#1769=VERTEX_POINT('',#18309);
#1770=VERTEX_POINT('',#18325);
#1771=VERTEX_POINT('',#18326);
#1772=VERTEX_POINT('',#18343);
#1773=VERTEX_POINT('',#18345);
#1774=VERTEX_POINT('',#18359);
#1775=VERTEX_POINT('',#19296);
#1776=VERTEX_POINT('',#19321);
#1891=EDGE_CURVE('',#1551,#1551,#1427,.T.);
#1892=EDGE_CURVE('',#1551,#1552,#450,.T.);
#1893=EDGE_CURVE('',#1552,#1552,#1428,.T.);
#1894=EDGE_CURVE('',#1553,#1553,#1429,.T.);
#1895=EDGE_CURVE('',#1553,#1554,#451,.T.);
#1896=EDGE_CURVE('',#1554,#1554,#1430,.T.);
#1897=EDGE_CURVE('',#1555,#1556,#1431,.T.);
#1898=EDGE_CURVE('',#1557,#1556,#294,.T.);
#1899=EDGE_CURVE('',#1557,#1558,#1432,.T.);
#1900=EDGE_CURVE('',#1558,#1559,#452,.T.);
#1901=EDGE_CURVE('',#1559,#1559,#1433,.T.);
#1902=EDGE_CURVE('',#1558,#1560,#1434,.T.);
#1903=EDGE_CURVE('',#1555,#1560,#295,.T.);
#1904=EDGE_CURVE('',#1561,#1562,#296,.T.);
#1905=EDGE_CURVE('',#1563,#1562,#1435,.T.);
#1906=EDGE_CURVE('',#1564,#1563,#1436,.T.);
#1907=EDGE_CURVE('',#1565,#1564,#297,.T.);
#1908=EDGE_CURVE('',#1561,#1565,#453,.T.);
#1909=EDGE_CURVE('',#1566,#1567,#298,.F.);
#1910=EDGE_CURVE('',#1567,#1568,#454,.T.);
#1911=EDGE_CURVE('',#1568,#1569,#1437,.T.);
#1912=EDGE_CURVE('',#1569,#1570,#455,.T.);
#1913=EDGE_CURVE('',#1570,#1571,#299,.T.);
#1914=EDGE_CURVE('',#1571,#1572,#456,.T.);
#1915=EDGE_CURVE('',#1572,#1573,#1438,.T.);
#1916=EDGE_CURVE('',#1573,#1574,#457,.T.);
#1917=EDGE_CURVE('',#1574,#1575,#300,.T.);
#1918=EDGE_CURVE('',#1575,#1576,#458,.T.);
#1919=EDGE_CURVE('',#1576,#1576,#1439,.T.);
#1920=EDGE_CURVE('',#1575,#1577,#301,.T.);
#1921=EDGE_CURVE('',#1577,#1578,#459,.T.);
#1922=EDGE_CURVE('',#1578,#1579,#1440,.T.);
#1923=EDGE_CURVE('',#1579,#1580,#460,.T.);
#1924=EDGE_CURVE('',#1580,#1581,#302,.T.);
#1925=EDGE_CURVE('',#1581,#1582,#461,.T.);
#1926=EDGE_CURVE('',#1582,#1583,#1441,.T.);
#1927=EDGE_CURVE('',#1583,#1566,#462,.T.);
#1928=EDGE_CURVE('',#1584,#1585,#463,.T.);
#1929=EDGE_CURVE('',#1586,#1584,#197,.T.);
#1930=EDGE_CURVE('',#1587,#1586,#464,.T.);
#1931=EDGE_CURVE('',#1587,#1585,#198,.T.);
#1932=EDGE_CURVE('',#1588,#1589,#465,.T.);
#1933=EDGE_CURVE('',#1588,#1590,#199,.T.);
#1934=EDGE_CURVE('',#1591,#1590,#303,.T.);
#1935=EDGE_CURVE('',#1589,#1591,#200,.T.);
#1936=EDGE_CURVE('',#1592,#1593,#466,.T.);
#1937=EDGE_CURVE('',#1594,#1592,#201,.T.);
#1938=EDGE_CURVE('',#1595,#1594,#467,.T.);
#1939=EDGE_CURVE('',#1595,#1593,#202,.T.);
#1940=EDGE_CURVE('',#1596,#1597,#468,.T.);
#1941=EDGE_CURVE('',#1596,#1598,#203,.T.);
#1942=EDGE_CURVE('',#1599,#1598,#469,.T.);
#1943=EDGE_CURVE('',#1597,#1599,#204,.T.);
#1944=EDGE_CURVE('',#1600,#1601,#470,.T.);
#1945=EDGE_CURVE('',#1602,#1600,#205,.T.);
#1946=EDGE_CURVE('',#1603,#1602,#471,.T.);
#1947=EDGE_CURVE('',#1603,#1601,#206,.T.);
#1948=EDGE_CURVE('',#1604,#1605,#472,.T.);
#1949=EDGE_CURVE('',#1604,#1606,#207,.T.);
#1950=EDGE_CURVE('',#1607,#1606,#473,.T.);
#1951=EDGE_CURVE('',#1605,#1607,#208,.T.);
#1952=EDGE_CURVE('',#1608,#1609,#474,.T.);
#1953=EDGE_CURVE('',#1610,#1608,#209,.T.);
#1954=EDGE_CURVE('',#1611,#1610,#475,.T.);
#1955=EDGE_CURVE('',#1611,#1609,#210,.T.);
#1956=EDGE_CURVE('',#1612,#1613,#476,.T.);
#1957=EDGE_CURVE('',#1612,#1614,#211,.T.);
#1958=EDGE_CURVE('',#1615,#1614,#477,.T.);
#1959=EDGE_CURVE('',#1613,#1615,#212,.T.);
#1960=EDGE_CURVE('',#1616,#1617,#478,.T.);
#1961=EDGE_CURVE('',#1616,#1618,#213,.T.);
#1962=EDGE_CURVE('',#1619,#1618,#479,.T.);
#1963=EDGE_CURVE('',#1617,#1619,#214,.T.);
#1964=EDGE_CURVE('',#1620,#1621,#480,.T.);
#1965=EDGE_CURVE('',#1622,#1620,#215,.T.);
#1966=EDGE_CURVE('',#1623,#1622,#481,.T.);
#1967=EDGE_CURVE('',#1621,#1623,#1442,.T.);
#1968=EDGE_CURVE('',#1624,#1625,#482,.T.);
#1969=EDGE_CURVE('',#1624,#1626,#216,.T.);
#1970=EDGE_CURVE('',#1627,#1626,#483,.T.);
#1971=EDGE_CURVE('',#1625,#1627,#217,.T.);
#1972=EDGE_CURVE('',#1628,#1629,#484,.T.);
#1973=EDGE_CURVE('',#1630,#1628,#218,.T.);
#1974=EDGE_CURVE('',#1631,#1630,#485,.T.);
#1975=EDGE_CURVE('',#1631,#1629,#219,.T.);
#1976=EDGE_CURVE('',#1632,#1633,#486,.T.);
#1977=EDGE_CURVE('',#1632,#1634,#220,.T.);
#1978=EDGE_CURVE('',#1635,#1634,#487,.T.);
#1979=EDGE_CURVE('',#1633,#1635,#221,.T.);
#1980=EDGE_CURVE('',#1636,#1637,#488,.T.);
#1981=EDGE_CURVE('',#1638,#1636,#222,.T.);
#1982=EDGE_CURVE('',#1639,#1638,#489,.T.);
#1983=EDGE_CURVE('',#1639,#1637,#223,.T.);
#1984=EDGE_CURVE('',#1640,#1641,#490,.T.);
#1985=EDGE_CURVE('',#1640,#1642,#224,.T.);
#1986=EDGE_CURVE('',#1643,#1642,#491,.T.);
#1987=EDGE_CURVE('',#1641,#1643,#225,.T.);
#1988=EDGE_CURVE('',#1644,#1645,#492,.T.);
#1989=EDGE_CURVE('',#1646,#1644,#226,.T.);
#1990=EDGE_CURVE('',#1647,#1646,#493,.T.);
#1991=EDGE_CURVE('',#1647,#1645,#227,.T.);
#1992=EDGE_CURVE('',#1648,#1649,#228,.T.);
#1993=EDGE_CURVE('',#1649,#1593,#1443,.T.);
#1994=EDGE_CURVE('',#1595,#1648,#304,.T.);
#1995=EDGE_CURVE('',#1596,#1650,#305,.T.);
#1996=EDGE_CURVE('',#1650,#1651,#229,.T.);
#1997=EDGE_CURVE('',#1651,#1598,#306,.T.);
#1998=EDGE_CURVE('',#1652,#1653,#230,.T.);
#1999=EDGE_CURVE('',#1653,#1601,#1444,.T.);
#2000=EDGE_CURVE('',#1603,#1652,#307,.T.);
#2001=EDGE_CURVE('',#1604,#1654,#308,.T.);
#2002=EDGE_CURVE('',#1654,#1655,#231,.T.);
#2003=EDGE_CURVE('',#1655,#1606,#309,.T.);
#2004=EDGE_CURVE('',#1656,#1657,#232,.T.);
#2005=EDGE_CURVE('',#1657,#1609,#1445,.T.);
#2006=EDGE_CURVE('',#1611,#1656,#310,.T.);
#2007=EDGE_CURVE('',#1612,#1658,#311,.T.);
#2008=EDGE_CURVE('',#1658,#1659,#233,.T.);
#2009=EDGE_CURVE('',#1659,#1614,#312,.T.);
#2010=EDGE_CURVE('',#1660,#1661,#234,.T.);
#2011=EDGE_CURVE('',#1661,#1585,#1446,.T.);
#2012=EDGE_CURVE('',#1587,#1660,#313,.T.);
#2013=EDGE_CURVE('',#1588,#1662,#314,.T.);
#2014=EDGE_CURVE('',#1662,#1663,#235,.T.);
#2015=EDGE_CURVE('',#1663,#1664,#315,.T.);
#2016=EDGE_CURVE('',#1664,#1590,#494,.T.);
#2017=EDGE_CURVE('',#1616,#1665,#316,.T.);
#2018=EDGE_CURVE('',#1665,#1666,#1447,.T.);
#2019=EDGE_CURVE('',#1666,#1667,#1448,.T.);
#2020=EDGE_CURVE('',#1667,#1668,#495,.T.);
#2021=EDGE_CURVE('',#1668,#1669,#236,.T.);
#2022=EDGE_CURVE('',#1669,#1618,#1449,.T.);
#2023=EDGE_CURVE('',#1624,#1670,#317,.T.);
#2024=EDGE_CURVE('',#1670,#1671,#237,.T.);
#2025=EDGE_CURVE('',#1671,#1626,#1450,.T.);
#2026=EDGE_CURVE('',#1672,#1673,#238,.T.);
#2027=EDGE_CURVE('',#1673,#1629,#318,.T.);
#2028=EDGE_CURVE('',#1631,#1672,#319,.T.);
#2029=EDGE_CURVE('',#1632,#1674,#320,.T.);
#2030=EDGE_CURVE('',#1674,#1675,#239,.T.);
#2031=EDGE_CURVE('',#1675,#1634,#1451,.T.);
#2032=EDGE_CURVE('',#1676,#1677,#240,.T.);
#2033=EDGE_CURVE('',#1677,#1637,#321,.T.);
#2034=EDGE_CURVE('',#1639,#1676,#322,.T.);
#2035=EDGE_CURVE('',#1640,#1678,#323,.T.);
#2036=EDGE_CURVE('',#1678,#1679,#241,.T.);
#2037=EDGE_CURVE('',#1679,#1642,#1452,.T.);
#2038=EDGE_CURVE('',#1680,#1681,#242,.T.);
#2039=EDGE_CURVE('',#1681,#1645,#324,.T.);
#2040=EDGE_CURVE('',#1647,#1680,#325,.T.);
#2041=EDGE_CURVE('',#1682,#1683,#243,.T.);
#2042=EDGE_CURVE('',#1682,#1684,#326,.T.);
#2043=EDGE_CURVE('',#1684,#1685,#244,.T.);
#2044=EDGE_CURVE('',#1685,#1683,#327,.T.);
#2045=EDGE_CURVE('',#1686,#1687,#245,.T.);
#2046=EDGE_CURVE('',#1687,#1688,#328,.T.);
#2047=EDGE_CURVE('',#1689,#1688,#246,.T.);
#2048=EDGE_CURVE('',#1689,#1690,#1453,.T.);
#2049=EDGE_CURVE('',#1690,#1686,#329,.T.);
#2050=EDGE_CURVE('',#1691,#1692,#247,.T.);
#2051=EDGE_CURVE('',#1692,#1649,#496,.T.);
#2052=EDGE_CURVE('',#1648,#1691,#497,.T.);
#2053=EDGE_CURVE('',#1650,#1693,#498,.T.);
#2054=EDGE_CURVE('',#1693,#1694,#248,.T.);
#2055=EDGE_CURVE('',#1694,#1651,#499,.T.);
#2056=EDGE_CURVE('',#1695,#1696,#249,.T.);
#2057=EDGE_CURVE('',#1696,#1653,#500,.T.);
#2058=EDGE_CURVE('',#1652,#1695,#501,.T.);
#2059=EDGE_CURVE('',#1654,#1697,#502,.T.);
#2060=EDGE_CURVE('',#1697,#1698,#250,.T.);
#2061=EDGE_CURVE('',#1698,#1655,#503,.T.);
#2062=EDGE_CURVE('',#1699,#1700,#251,.T.);
#2063=EDGE_CURVE('',#1700,#1657,#504,.T.);
#2064=EDGE_CURVE('',#1656,#1699,#505,.T.);
#2065=EDGE_CURVE('',#1658,#1701,#506,.T.);
#2066=EDGE_CURVE('',#1701,#1702,#252,.T.);
#2067=EDGE_CURVE('',#1702,#1659,#507,.T.);
#2068=EDGE_CURVE('',#1703,#1704,#253,.T.);
#2069=EDGE_CURVE('',#1704,#1661,#508,.T.);
#2070=EDGE_CURVE('',#1660,#1703,#509,.T.);
#2071=EDGE_CURVE('',#1662,#1705,#510,.T.);
#2072=EDGE_CURVE('',#1705,#1706,#254,.T.);
#2073=EDGE_CURVE('',#1706,#1663,#511,.T.);
#2074=EDGE_CURVE('',#1668,#1707,#512,.T.);
#2075=EDGE_CURVE('',#1707,#1708,#255,.T.);
#2076=EDGE_CURVE('',#1708,#1669,#513,.T.);
#2077=EDGE_CURVE('',#1670,#1709,#514,.T.);
#2078=EDGE_CURVE('',#1709,#1710,#256,.T.);
#2079=EDGE_CURVE('',#1710,#1671,#515,.T.);
#2080=EDGE_CURVE('',#1711,#1712,#257,.T.);
#2081=EDGE_CURVE('',#1712,#1673,#516,.T.);
#2082=EDGE_CURVE('',#1672,#1711,#517,.T.);
#2083=EDGE_CURVE('',#1674,#1713,#518,.T.);
#2084=EDGE_CURVE('',#1713,#1714,#258,.T.);
#2085=EDGE_CURVE('',#1714,#1675,#519,.T.);
#2086=EDGE_CURVE('',#1715,#1716,#259,.T.);
#2087=EDGE_CURVE('',#1716,#1677,#520,.T.);
#2088=EDGE_CURVE('',#1676,#1715,#521,.T.);
#2089=EDGE_CURVE('',#1678,#1717,#522,.T.);
#2090=EDGE_CURVE('',#1717,#1718,#260,.T.);
#2091=EDGE_CURVE('',#1718,#1679,#523,.T.);
#2092=EDGE_CURVE('',#1719,#1720,#261,.T.);
#2093=EDGE_CURVE('',#1720,#1681,#524,.T.);
#2094=EDGE_CURVE('',#1680,#1719,#525,.T.);
#2095=EDGE_CURVE('',#1684,#1721,#526,.T.);
#2096=EDGE_CURVE('',#1721,#1722,#262,.T.);
#2097=EDGE_CURVE('',#1722,#1723,#527,.T.);
#2098=EDGE_CURVE('',#1723,#1685,#330,.T.);
#2099=EDGE_CURVE('',#1724,#1725,#263,.T.);
#2100=EDGE_CURVE('',#1725,#1687,#528,.T.);
#2101=EDGE_CURVE('',#1686,#1724,#529,.T.);
#2102=EDGE_CURVE('',#1726,#1727,#264,.T.);
#2103=EDGE_CURVE('',#1727,#1728,#530,.T.);
#2104=EDGE_CURVE('',#1729,#1728,#265,.T.);
#2105=EDGE_CURVE('',#1729,#1730,#331,.T.);
#2106=EDGE_CURVE('',#1730,#1726,#531,.T.);
#2107=EDGE_CURVE('',#1731,#1732,#266,.T.);
#2108=EDGE_CURVE('',#1731,#1733,#532,.T.);
#2109=EDGE_CURVE('',#1733,#1734,#267,.T.);
#2110=EDGE_CURVE('',#1734,#1732,#332,.T.);
#2111=EDGE_CURVE('',#1735,#1736,#333,.T.);
#2112=EDGE_CURVE('',#1736,#1692,#334,.T.);
#2113=EDGE_CURVE('',#1691,#1737,#533,.T.);
#2114=EDGE_CURVE('',#1737,#1735,#1454,.T.);
#2115=EDGE_CURVE('',#1693,#1738,#335,.T.);
#2116=EDGE_CURVE('',#1738,#1739,#336,.T.);
#2117=EDGE_CURVE('',#1739,#1740,#268,.T.);
#2118=EDGE_CURVE('',#1740,#1694,#337,.T.);
#2119=EDGE_CURVE('',#1592,#1696,#338,.T.);
#2120=EDGE_CURVE('',#1695,#1594,#339,.T.);
#2121=EDGE_CURVE('',#1697,#1597,#340,.T.);
#2122=EDGE_CURVE('',#1599,#1698,#341,.T.);
#2123=EDGE_CURVE('',#1600,#1700,#342,.T.);
#2124=EDGE_CURVE('',#1699,#1602,#343,.T.);
#2125=EDGE_CURVE('',#1701,#1605,#344,.T.);
#2126=EDGE_CURVE('',#1607,#1702,#345,.T.);
#2127=EDGE_CURVE('',#1608,#1704,#346,.T.);
#2128=EDGE_CURVE('',#1703,#1610,#347,.T.);
#2129=EDGE_CURVE('',#1705,#1613,#348,.T.);
#2130=EDGE_CURVE('',#1615,#1706,#349,.T.);
#2131=EDGE_CURVE('',#1707,#1741,#534,.T.);
#2132=EDGE_CURVE('',#1741,#1742,#269,.T.);
#2133=EDGE_CURVE('',#1742,#1708,#535,.T.);
#2134=EDGE_CURVE('',#1709,#1617,#1455,.T.);
#2135=EDGE_CURVE('',#1619,#1710,#350,.T.);
#2136=EDGE_CURVE('',#1620,#1712,#351,.T.);
#2137=EDGE_CURVE('',#1711,#1622,#1456,.T.);
#2138=EDGE_CURVE('',#1713,#1625,#1457,.T.);
#2139=EDGE_CURVE('',#1627,#1714,#352,.T.);
#2140=EDGE_CURVE('',#1628,#1716,#353,.T.);
#2141=EDGE_CURVE('',#1715,#1630,#1458,.T.);
#2142=EDGE_CURVE('',#1717,#1633,#1459,.T.);
#2143=EDGE_CURVE('',#1635,#1718,#354,.T.);
#2144=EDGE_CURVE('',#1636,#1720,#355,.T.);
#2145=EDGE_CURVE('',#1719,#1638,#1460,.T.);
#2146=EDGE_CURVE('',#1721,#1641,#1461,.T.);
#2147=EDGE_CURVE('',#1643,#1722,#356,.T.);
#2148=EDGE_CURVE('',#1644,#1725,#357,.T.);
#2149=EDGE_CURVE('',#1724,#1646,#1462,.T.);
#2150=EDGE_CURVE('',#1584,#1727,#358,.T.);
#2151=EDGE_CURVE('',#1726,#1586,#359,.T.);
#2152=EDGE_CURVE('',#1733,#1589,#360,.T.);
#2153=EDGE_CURVE('',#1591,#1734,#361,.T.);
#2154=EDGE_CURVE('',#1667,#1741,#536,.T.);
#2155=EDGE_CURVE('',#1743,#1666,#1463,.T.);
#2156=EDGE_CURVE('',#1742,#1743,#537,.T.);
#2157=EDGE_CURVE('',#1582,#1736,#538,.T.);
#2158=EDGE_CURVE('',#1735,#1744,#1464,.T.);
#2159=EDGE_CURVE('',#1744,#1583,#539,.T.);
#2160=EDGE_CURVE('',#1738,#1579,#540,.T.);
#2161=EDGE_CURVE('',#1578,#1745,#541,.T.);
#2162=EDGE_CURVE('',#1745,#1739,#1465,.T.);
#2163=EDGE_CURVE('',#1665,#1569,#542,.T.);
#2164=EDGE_CURVE('',#1568,#1743,#543,.T.);
#2165=EDGE_CURVE('',#1572,#1621,#544,.T.);
#2166=EDGE_CURVE('',#1623,#1573,#545,.T.);
#2167=EDGE_CURVE('',#1746,#1747,#546,.T.);
#2168=EDGE_CURVE('',#1746,#1748,#270,.T.);
#2169=EDGE_CURVE('',#1749,#1748,#547,.T.);
#2170=EDGE_CURVE('',#1747,#1749,#271,.T.);
#2171=EDGE_CURVE('',#1750,#1751,#548,.T.);
#2172=EDGE_CURVE('',#1752,#1750,#272,.T.);
#2173=EDGE_CURVE('',#1753,#1752,#362,.T.);
#2174=EDGE_CURVE('',#1753,#1751,#273,.T.);
#2175=EDGE_CURVE('',#1682,#1754,#549,.T.);
#2176=EDGE_CURVE('',#1755,#1683,#363,.T.);
#2177=EDGE_CURVE('',#1754,#1755,#274,.T.);
#2178=EDGE_CURVE('',#1756,#1688,#550,.T.);
#2179=EDGE_CURVE('',#1757,#1756,#275,.T.);
#2180=EDGE_CURVE('',#1689,#1757,#364,.T.);
#2181=EDGE_CURVE('',#1728,#1751,#1466,.T.);
#2182=EDGE_CURVE('',#1753,#1729,#365,.T.);
#2183=EDGE_CURVE('',#1758,#1759,#276,.T.);
#2184=EDGE_CURVE('',#1759,#1748,#366,.T.);
#2185=EDGE_CURVE('',#1746,#1731,#367,.T.);
#2186=EDGE_CURVE('',#1732,#1758,#368,.T.);
#2187=EDGE_CURVE('',#1760,#1761,#277,.T.);
#2188=EDGE_CURVE('',#1761,#1762,#551,.T.);
#2189=EDGE_CURVE('',#1762,#1562,#369,.T.);
#2190=EDGE_CURVE('',#1561,#1760,#370,.T.);
#2191=EDGE_CURVE('',#1763,#1764,#371,.T.);
#2192=EDGE_CURVE('',#1764,#1765,#552,.T.);
#2193=EDGE_CURVE('',#1765,#1766,#278,.T.);
#2194=EDGE_CURVE('',#1766,#1767,#372,.T.);
#2195=EDGE_CURVE('',#1763,#1767,#1467,.T.);
#2196=EDGE_CURVE('',#1768,#1769,#279,.T.);
#2197=EDGE_CURVE('',#1769,#1759,#553,.T.);
#2198=EDGE_CURVE('',#1758,#1768,#373,.T.);
#2199=EDGE_CURVE('',#1770,#1771,#280,.T.);
#2200=EDGE_CURVE('',#1771,#1761,#554,.T.);
#2201=EDGE_CURVE('',#1760,#1770,#555,.T.);
#2202=EDGE_CURVE('',#1765,#1772,#556,.T.);
#2203=EDGE_CURVE('',#1772,#1773,#281,.T.);
#2204=EDGE_CURVE('',#1773,#1774,#374,.T.);
#2205=EDGE_CURVE('',#1774,#1766,#1468,.T.);
#2206=EDGE_CURVE('',#1750,#1771,#375,.T.);
#2207=EDGE_CURVE('',#1770,#1754,#1469,.T.);
#2208=EDGE_CURVE('',#1755,#1752,#376,.T.);
#2209=EDGE_CURVE('',#1756,#1769,#377,.T.);
#2210=EDGE_CURVE('',#1768,#1757,#378,.T.);
#2211=EDGE_CURVE('',#1749,#1775,#557,.T.);
#2212=EDGE_CURVE('',#1775,#1773,#379,.T.);
#2213=EDGE_CURVE('',#1772,#1747,#380,.T.);
#2214=EDGE_CURVE('',#1570,#1565,#558,.T.);
#2215=EDGE_CURVE('',#1557,#1564,#559,.T.);
#2216=EDGE_CURVE('',#1774,#1556,#560,.T.);
#2217=EDGE_CURVE('',#1571,#1775,#561,.T.);
#2218=EDGE_CURVE('',#1762,#1581,#562,.T.);
#2219=EDGE_CURVE('',#1764,#1580,#563,.T.);
#2220=EDGE_CURVE('',#1763,#1776,#147,.T.);
#2221=EDGE_CURVE('',#1555,#1776,#564,.T.);
#2222=EDGE_CURVE('',#1563,#1560,#565,.T.);
#2223=EDGE_CURVE('',#1740,#1745,#566,.T.);
#2224=EDGE_CURVE('',#1744,#1737,#567,.T.);
#2225=EDGE_CURVE('',#1567,#1723,#568,.T.);
#2226=EDGE_CURVE('',#1566,#1730,#569,.T.);
#2227=EDGE_CURVE('',#1776,#1767,#1470,.T.);
#2228=EDGE_CURVE('',#1690,#1574,#570,.T.);
#2229=EDGE_CURVE('',#1664,#1577,#571,.T.);
#2418=ORIENTED_EDGE('',*,*,#1891,.F.);
#2419=ORIENTED_EDGE('',*,*,#1892,.T.);
#2420=ORIENTED_EDGE('',*,*,#1893,.T.);
#2421=ORIENTED_EDGE('',*,*,#1892,.F.);
#2422=ORIENTED_EDGE('',*,*,#1894,.T.);
#2423=ORIENTED_EDGE('',*,*,#1895,.T.);
#2424=ORIENTED_EDGE('',*,*,#1896,.T.);
#2425=ORIENTED_EDGE('',*,*,#1895,.F.);
#2426=ORIENTED_EDGE('',*,*,#1897,.T.);
#2427=ORIENTED_EDGE('',*,*,#1898,.F.);
#2428=ORIENTED_EDGE('',*,*,#1899,.T.);
#2429=ORIENTED_EDGE('',*,*,#1900,.T.);
#2430=ORIENTED_EDGE('',*,*,#1901,.F.);
#2431=ORIENTED_EDGE('',*,*,#1900,.F.);
#2432=ORIENTED_EDGE('',*,*,#1902,.T.);
#2433=ORIENTED_EDGE('',*,*,#1903,.F.);
#2434=ORIENTED_EDGE('',*,*,#1904,.T.);
#2435=ORIENTED_EDGE('',*,*,#1905,.F.);
#2436=ORIENTED_EDGE('',*,*,#1906,.F.);
#2437=ORIENTED_EDGE('',*,*,#1907,.F.);
#2438=ORIENTED_EDGE('',*,*,#1908,.F.);
#2439=ORIENTED_EDGE('',*,*,#1909,.T.);
#2440=ORIENTED_EDGE('',*,*,#1910,.T.);
#2441=ORIENTED_EDGE('',*,*,#1911,.T.);
#2442=ORIENTED_EDGE('',*,*,#1912,.T.);
#2443=ORIENTED_EDGE('',*,*,#1913,.T.);
#2444=ORIENTED_EDGE('',*,*,#1914,.T.);
#2445=ORIENTED_EDGE('',*,*,#1915,.T.);
#2446=ORIENTED_EDGE('',*,*,#1916,.T.);
#2447=ORIENTED_EDGE('',*,*,#1917,.T.);
#2448=ORIENTED_EDGE('',*,*,#1918,.T.);
#2449=ORIENTED_EDGE('',*,*,#1919,.T.);
#2450=ORIENTED_EDGE('',*,*,#1918,.F.);
#2451=ORIENTED_EDGE('',*,*,#1920,.T.);
#2452=ORIENTED_EDGE('',*,*,#1921,.T.);
#2453=ORIENTED_EDGE('',*,*,#1922,.T.);
#2454=ORIENTED_EDGE('',*,*,#1923,.T.);
#2455=ORIENTED_EDGE('',*,*,#1924,.T.);
#2456=ORIENTED_EDGE('',*,*,#1925,.T.);
#2457=ORIENTED_EDGE('',*,*,#1926,.T.);
#2458=ORIENTED_EDGE('',*,*,#1927,.T.);
#2459=ORIENTED_EDGE('',*,*,#1928,.F.);
#2460=ORIENTED_EDGE('',*,*,#1929,.F.);
#2461=ORIENTED_EDGE('',*,*,#1930,.F.);
#2462=ORIENTED_EDGE('',*,*,#1931,.T.);
#2463=ORIENTED_EDGE('',*,*,#1932,.F.);
#2464=ORIENTED_EDGE('',*,*,#1933,.T.);
#2465=ORIENTED_EDGE('',*,*,#1934,.F.);
#2466=ORIENTED_EDGE('',*,*,#1935,.F.);
#2467=ORIENTED_EDGE('',*,*,#1936,.F.);
#2468=ORIENTED_EDGE('',*,*,#1937,.F.);
#2469=ORIENTED_EDGE('',*,*,#1938,.F.);
#2470=ORIENTED_EDGE('',*,*,#1939,.T.);
#2471=ORIENTED_EDGE('',*,*,#1940,.F.);
#2472=ORIENTED_EDGE('',*,*,#1941,.T.);
#2473=ORIENTED_EDGE('',*,*,#1942,.F.);
#2474=ORIENTED_EDGE('',*,*,#1943,.F.);
#2475=ORIENTED_EDGE('',*,*,#1944,.F.);
#2476=ORIENTED_EDGE('',*,*,#1945,.F.);
#2477=ORIENTED_EDGE('',*,*,#1946,.F.);
#2478=ORIENTED_EDGE('',*,*,#1947,.T.);
#2479=ORIENTED_EDGE('',*,*,#1948,.F.);
#2480=ORIENTED_EDGE('',*,*,#1949,.T.);
#2481=ORIENTED_EDGE('',*,*,#1950,.F.);
#2482=ORIENTED_EDGE('',*,*,#1951,.F.);
#2483=ORIENTED_EDGE('',*,*,#1952,.F.);
#2484=ORIENTED_EDGE('',*,*,#1953,.F.);
#2485=ORIENTED_EDGE('',*,*,#1954,.F.);
#2486=ORIENTED_EDGE('',*,*,#1955,.T.);
#2487=ORIENTED_EDGE('',*,*,#1956,.F.);
#2488=ORIENTED_EDGE('',*,*,#1957,.T.);
#2489=ORIENTED_EDGE('',*,*,#1958,.F.);
#2490=ORIENTED_EDGE('',*,*,#1959,.F.);
#2491=ORIENTED_EDGE('',*,*,#1960,.F.);
#2492=ORIENTED_EDGE('',*,*,#1961,.T.);
#2493=ORIENTED_EDGE('',*,*,#1962,.F.);
#2494=ORIENTED_EDGE('',*,*,#1963,.F.);
#2495=ORIENTED_EDGE('',*,*,#1964,.F.);
#2496=ORIENTED_EDGE('',*,*,#1965,.F.);
#2497=ORIENTED_EDGE('',*,*,#1966,.F.);
#2498=ORIENTED_EDGE('',*,*,#1967,.F.);
#2499=ORIENTED_EDGE('',*,*,#1968,.F.);
#2500=ORIENTED_EDGE('',*,*,#1969,.T.);
#2501=ORIENTED_EDGE('',*,*,#1970,.F.);
#2502=ORIENTED_EDGE('',*,*,#1971,.F.);
#2503=ORIENTED_EDGE('',*,*,#1972,.F.);
#2504=ORIENTED_EDGE('',*,*,#1973,.F.);
#2505=ORIENTED_EDGE('',*,*,#1974,.F.);
#2506=ORIENTED_EDGE('',*,*,#1975,.T.);
#2507=ORIENTED_EDGE('',*,*,#1976,.F.);
#2508=ORIENTED_EDGE('',*,*,#1977,.T.);
#2509=ORIENTED_EDGE('',*,*,#1978,.F.);
#2510=ORIENTED_EDGE('',*,*,#1979,.F.);
#2511=ORIENTED_EDGE('',*,*,#1980,.F.);
#2512=ORIENTED_EDGE('',*,*,#1981,.F.);
#2513=ORIENTED_EDGE('',*,*,#1982,.F.);
#2514=ORIENTED_EDGE('',*,*,#1983,.T.);
#2515=ORIENTED_EDGE('',*,*,#1984,.F.);
#2516=ORIENTED_EDGE('',*,*,#1985,.T.);
#2517=ORIENTED_EDGE('',*,*,#1986,.F.);
#2518=ORIENTED_EDGE('',*,*,#1987,.F.);
#2519=ORIENTED_EDGE('',*,*,#1988,.F.);
#2520=ORIENTED_EDGE('',*,*,#1989,.F.);
#2521=ORIENTED_EDGE('',*,*,#1990,.F.);
#2522=ORIENTED_EDGE('',*,*,#1991,.T.);
#2523=ORIENTED_EDGE('',*,*,#1992,.T.);
#2524=ORIENTED_EDGE('',*,*,#1993,.T.);
#2525=ORIENTED_EDGE('',*,*,#1939,.F.);
#2526=ORIENTED_EDGE('',*,*,#1994,.T.);
#2527=ORIENTED_EDGE('',*,*,#1941,.F.);
#2528=ORIENTED_EDGE('',*,*,#1995,.T.);
#2529=ORIENTED_EDGE('',*,*,#1996,.T.);
#2530=ORIENTED_EDGE('',*,*,#1997,.T.);
#2531=ORIENTED_EDGE('',*,*,#1998,.T.);
#2532=ORIENTED_EDGE('',*,*,#1999,.T.);
#2533=ORIENTED_EDGE('',*,*,#1947,.F.);
#2534=ORIENTED_EDGE('',*,*,#2000,.T.);
#2535=ORIENTED_EDGE('',*,*,#1949,.F.);
#2536=ORIENTED_EDGE('',*,*,#2001,.T.);
#2537=ORIENTED_EDGE('',*,*,#2002,.T.);
#2538=ORIENTED_EDGE('',*,*,#2003,.T.);
#2539=ORIENTED_EDGE('',*,*,#2004,.T.);
#2540=ORIENTED_EDGE('',*,*,#2005,.T.);
#2541=ORIENTED_EDGE('',*,*,#1955,.F.);
#2542=ORIENTED_EDGE('',*,*,#2006,.T.);
#2543=ORIENTED_EDGE('',*,*,#1957,.F.);
#2544=ORIENTED_EDGE('',*,*,#2007,.T.);
#2545=ORIENTED_EDGE('',*,*,#2008,.T.);
#2546=ORIENTED_EDGE('',*,*,#2009,.T.);
#2547=ORIENTED_EDGE('',*,*,#2010,.T.);
#2548=ORIENTED_EDGE('',*,*,#2011,.T.);
#2549=ORIENTED_EDGE('',*,*,#1931,.F.);
#2550=ORIENTED_EDGE('',*,*,#2012,.T.);
#2551=ORIENTED_EDGE('',*,*,#1933,.F.);
#2552=ORIENTED_EDGE('',*,*,#2013,.T.);
#2553=ORIENTED_EDGE('',*,*,#2014,.T.);
#2554=ORIENTED_EDGE('',*,*,#2015,.T.);
#2555=ORIENTED_EDGE('',*,*,#2016,.T.);
#2556=ORIENTED_EDGE('',*,*,#1961,.F.);
#2557=ORIENTED_EDGE('',*,*,#2017,.T.);
#2558=ORIENTED_EDGE('',*,*,#2018,.T.);
#2559=ORIENTED_EDGE('',*,*,#2019,.T.);
#2560=ORIENTED_EDGE('',*,*,#2020,.T.);
#2561=ORIENTED_EDGE('',*,*,#2021,.T.);
#2562=ORIENTED_EDGE('',*,*,#2022,.T.);
#2563=ORIENTED_EDGE('',*,*,#1969,.F.);
#2564=ORIENTED_EDGE('',*,*,#2023,.T.);
#2565=ORIENTED_EDGE('',*,*,#2024,.T.);
#2566=ORIENTED_EDGE('',*,*,#2025,.T.);
#2567=ORIENTED_EDGE('',*,*,#2026,.T.);
#2568=ORIENTED_EDGE('',*,*,#2027,.T.);
#2569=ORIENTED_EDGE('',*,*,#1975,.F.);
#2570=ORIENTED_EDGE('',*,*,#2028,.T.);
#2571=ORIENTED_EDGE('',*,*,#1977,.F.);
#2572=ORIENTED_EDGE('',*,*,#2029,.T.);
#2573=ORIENTED_EDGE('',*,*,#2030,.T.);
#2574=ORIENTED_EDGE('',*,*,#2031,.T.);
#2575=ORIENTED_EDGE('',*,*,#2032,.T.);
#2576=ORIENTED_EDGE('',*,*,#2033,.T.);
#2577=ORIENTED_EDGE('',*,*,#1983,.F.);
#2578=ORIENTED_EDGE('',*,*,#2034,.T.);
#2579=ORIENTED_EDGE('',*,*,#1985,.F.);
#2580=ORIENTED_EDGE('',*,*,#2035,.T.);
#2581=ORIENTED_EDGE('',*,*,#2036,.T.);
#2582=ORIENTED_EDGE('',*,*,#2037,.T.);
#2583=ORIENTED_EDGE('',*,*,#2038,.T.);
#2584=ORIENTED_EDGE('',*,*,#2039,.T.);
#2585=ORIENTED_EDGE('',*,*,#1991,.F.);
#2586=ORIENTED_EDGE('',*,*,#2040,.T.);
#2587=ORIENTED_EDGE('',*,*,#2041,.F.);
#2588=ORIENTED_EDGE('',*,*,#2042,.T.);
#2589=ORIENTED_EDGE('',*,*,#2043,.T.);
#2590=ORIENTED_EDGE('',*,*,#2044,.T.);
#2591=ORIENTED_EDGE('',*,*,#2045,.T.);
#2592=ORIENTED_EDGE('',*,*,#2046,.T.);
#2593=ORIENTED_EDGE('',*,*,#2047,.F.);
#2594=ORIENTED_EDGE('',*,*,#2048,.T.);
#2595=ORIENTED_EDGE('',*,*,#2049,.T.);
#2596=ORIENTED_EDGE('',*,*,#2050,.T.);
#2597=ORIENTED_EDGE('',*,*,#2051,.T.);
#2598=ORIENTED_EDGE('',*,*,#1992,.F.);
#2599=ORIENTED_EDGE('',*,*,#2052,.T.);
#2600=ORIENTED_EDGE('',*,*,#1996,.F.);
#2601=ORIENTED_EDGE('',*,*,#2053,.T.);
#2602=ORIENTED_EDGE('',*,*,#2054,.T.);
#2603=ORIENTED_EDGE('',*,*,#2055,.T.);
#2604=ORIENTED_EDGE('',*,*,#2056,.T.);
#2605=ORIENTED_EDGE('',*,*,#2057,.T.);
#2606=ORIENTED_EDGE('',*,*,#1998,.F.);
#2607=ORIENTED_EDGE('',*,*,#2058,.T.);
#2608=ORIENTED_EDGE('',*,*,#2002,.F.);
#2609=ORIENTED_EDGE('',*,*,#2059,.T.);
#2610=ORIENTED_EDGE('',*,*,#2060,.T.);
#2611=ORIENTED_EDGE('',*,*,#2061,.T.);
#2612=ORIENTED_EDGE('',*,*,#2062,.T.);
#2613=ORIENTED_EDGE('',*,*,#2063,.T.);
#2614=ORIENTED_EDGE('',*,*,#2004,.F.);
#2615=ORIENTED_EDGE('',*,*,#2064,.T.);
#2616=ORIENTED_EDGE('',*,*,#2008,.F.);
#2617=ORIENTED_EDGE('',*,*,#2065,.T.);
#2618=ORIENTED_EDGE('',*,*,#2066,.T.);
#2619=ORIENTED_EDGE('',*,*,#2067,.T.);
#2620=ORIENTED_EDGE('',*,*,#2068,.T.);
#2621=ORIENTED_EDGE('',*,*,#2069,.T.);
#2622=ORIENTED_EDGE('',*,*,#2010,.F.);
#2623=ORIENTED_EDGE('',*,*,#2070,.T.);
#2624=ORIENTED_EDGE('',*,*,#2014,.F.);
#2625=ORIENTED_EDGE('',*,*,#2071,.T.);
#2626=ORIENTED_EDGE('',*,*,#2072,.T.);
#2627=ORIENTED_EDGE('',*,*,#2073,.T.);
#2628=ORIENTED_EDGE('',*,*,#2021,.F.);
#2629=ORIENTED_EDGE('',*,*,#2074,.T.);
#2630=ORIENTED_EDGE('',*,*,#2075,.T.);
#2631=ORIENTED_EDGE('',*,*,#2076,.T.);
#2632=ORIENTED_EDGE('',*,*,#2024,.F.);
#2633=ORIENTED_EDGE('',*,*,#2077,.T.);
#2634=ORIENTED_EDGE('',*,*,#2078,.T.);
#2635=ORIENTED_EDGE('',*,*,#2079,.T.);
#2636=ORIENTED_EDGE('',*,*,#2080,.T.);
#2637=ORIENTED_EDGE('',*,*,#2081,.T.);
#2638=ORIENTED_EDGE('',*,*,#2026,.F.);
#2639=ORIENTED_EDGE('',*,*,#2082,.T.);
#2640=ORIENTED_EDGE('',*,*,#2030,.F.);
#2641=ORIENTED_EDGE('',*,*,#2083,.T.);
#2642=ORIENTED_EDGE('',*,*,#2084,.T.);
#2643=ORIENTED_EDGE('',*,*,#2085,.T.);
#2644=ORIENTED_EDGE('',*,*,#2086,.T.);
#2645=ORIENTED_EDGE('',*,*,#2087,.T.);
#2646=ORIENTED_EDGE('',*,*,#2032,.F.);
#2647=ORIENTED_EDGE('',*,*,#2088,.T.);
#2648=ORIENTED_EDGE('',*,*,#2036,.F.);
#2649=ORIENTED_EDGE('',*,*,#2089,.T.);
#2650=ORIENTED_EDGE('',*,*,#2090,.T.);
#2651=ORIENTED_EDGE('',*,*,#2091,.T.);
#2652=ORIENTED_EDGE('',*,*,#2092,.T.);
#2653=ORIENTED_EDGE('',*,*,#2093,.T.);
#2654=ORIENTED_EDGE('',*,*,#2038,.F.);
#2655=ORIENTED_EDGE('',*,*,#2094,.T.);
#2656=ORIENTED_EDGE('',*,*,#2043,.F.);
#2657=ORIENTED_EDGE('',*,*,#2095,.T.);
#2658=ORIENTED_EDGE('',*,*,#2096,.T.);
#2659=ORIENTED_EDGE('',*,*,#2097,.T.);
#2660=ORIENTED_EDGE('',*,*,#2098,.T.);
#2661=ORIENTED_EDGE('',*,*,#2099,.T.);
#2662=ORIENTED_EDGE('',*,*,#2100,.T.);
#2663=ORIENTED_EDGE('',*,*,#2045,.F.);
#2664=ORIENTED_EDGE('',*,*,#2101,.T.);
#2665=ORIENTED_EDGE('',*,*,#2102,.T.);
#2666=ORIENTED_EDGE('',*,*,#2103,.T.);
#2667=ORIENTED_EDGE('',*,*,#2104,.F.);
#2668=ORIENTED_EDGE('',*,*,#2105,.T.);
#2669=ORIENTED_EDGE('',*,*,#2106,.T.);
#2670=ORIENTED_EDGE('',*,*,#2107,.F.);
#2671=ORIENTED_EDGE('',*,*,#2108,.T.);
#2672=ORIENTED_EDGE('',*,*,#2109,.T.);
#2673=ORIENTED_EDGE('',*,*,#2110,.T.);
#2674=ORIENTED_EDGE('',*,*,#2111,.T.);
#2675=ORIENTED_EDGE('',*,*,#2112,.T.);
#2676=ORIENTED_EDGE('',*,*,#2050,.F.);
#2677=ORIENTED_EDGE('',*,*,#2113,.T.);
#2678=ORIENTED_EDGE('',*,*,#2114,.T.);
#2679=ORIENTED_EDGE('',*,*,#2054,.F.);
#2680=ORIENTED_EDGE('',*,*,#2115,.T.);
#2681=ORIENTED_EDGE('',*,*,#2116,.T.);
#2682=ORIENTED_EDGE('',*,*,#2117,.T.);
#2683=ORIENTED_EDGE('',*,*,#2118,.T.);
#2684=ORIENTED_EDGE('',*,*,#1937,.T.);
#2685=ORIENTED_EDGE('',*,*,#2119,.T.);
#2686=ORIENTED_EDGE('',*,*,#2056,.F.);
#2687=ORIENTED_EDGE('',*,*,#2120,.T.);
#2688=ORIENTED_EDGE('',*,*,#2060,.F.);
#2689=ORIENTED_EDGE('',*,*,#2121,.T.);
#2690=ORIENTED_EDGE('',*,*,#1943,.T.);
#2691=ORIENTED_EDGE('',*,*,#2122,.T.);
#2692=ORIENTED_EDGE('',*,*,#1945,.T.);
#2693=ORIENTED_EDGE('',*,*,#2123,.T.);
#2694=ORIENTED_EDGE('',*,*,#2062,.F.);
#2695=ORIENTED_EDGE('',*,*,#2124,.T.);
#2696=ORIENTED_EDGE('',*,*,#2066,.F.);
#2697=ORIENTED_EDGE('',*,*,#2125,.T.);
#2698=ORIENTED_EDGE('',*,*,#1951,.T.);
#2699=ORIENTED_EDGE('',*,*,#2126,.T.);
#2700=ORIENTED_EDGE('',*,*,#1953,.T.);
#2701=ORIENTED_EDGE('',*,*,#2127,.T.);
#2702=ORIENTED_EDGE('',*,*,#2068,.F.);
#2703=ORIENTED_EDGE('',*,*,#2128,.T.);
#2704=ORIENTED_EDGE('',*,*,#2072,.F.);
#2705=ORIENTED_EDGE('',*,*,#2129,.T.);
#2706=ORIENTED_EDGE('',*,*,#1959,.T.);
#2707=ORIENTED_EDGE('',*,*,#2130,.T.);
#2708=ORIENTED_EDGE('',*,*,#2075,.F.);
#2709=ORIENTED_EDGE('',*,*,#2131,.T.);
#2710=ORIENTED_EDGE('',*,*,#2132,.T.);
#2711=ORIENTED_EDGE('',*,*,#2133,.T.);
#2712=ORIENTED_EDGE('',*,*,#2078,.F.);
#2713=ORIENTED_EDGE('',*,*,#2134,.T.);
#2714=ORIENTED_EDGE('',*,*,#1963,.T.);
#2715=ORIENTED_EDGE('',*,*,#2135,.T.);
#2716=ORIENTED_EDGE('',*,*,#1965,.T.);
#2717=ORIENTED_EDGE('',*,*,#2136,.T.);
#2718=ORIENTED_EDGE('',*,*,#2080,.F.);
#2719=ORIENTED_EDGE('',*,*,#2137,.T.);
#2720=ORIENTED_EDGE('',*,*,#2084,.F.);
#2721=ORIENTED_EDGE('',*,*,#2138,.T.);
#2722=ORIENTED_EDGE('',*,*,#1971,.T.);
#2723=ORIENTED_EDGE('',*,*,#2139,.T.);
#2724=ORIENTED_EDGE('',*,*,#1973,.T.);
#2725=ORIENTED_EDGE('',*,*,#2140,.T.);
#2726=ORIENTED_EDGE('',*,*,#2086,.F.);
#2727=ORIENTED_EDGE('',*,*,#2141,.T.);
#2728=ORIENTED_EDGE('',*,*,#2090,.F.);
#2729=ORIENTED_EDGE('',*,*,#2142,.T.);
#2730=ORIENTED_EDGE('',*,*,#1979,.T.);
#2731=ORIENTED_EDGE('',*,*,#2143,.T.);
#2732=ORIENTED_EDGE('',*,*,#1981,.T.);
#2733=ORIENTED_EDGE('',*,*,#2144,.T.);
#2734=ORIENTED_EDGE('',*,*,#2092,.F.);
#2735=ORIENTED_EDGE('',*,*,#2145,.T.);
#2736=ORIENTED_EDGE('',*,*,#2096,.F.);
#2737=ORIENTED_EDGE('',*,*,#2146,.T.);
#2738=ORIENTED_EDGE('',*,*,#1987,.T.);
#2739=ORIENTED_EDGE('',*,*,#2147,.T.);
#2740=ORIENTED_EDGE('',*,*,#1989,.T.);
#2741=ORIENTED_EDGE('',*,*,#2148,.T.);
#2742=ORIENTED_EDGE('',*,*,#2099,.F.);
#2743=ORIENTED_EDGE('',*,*,#2149,.T.);
#2744=ORIENTED_EDGE('',*,*,#1929,.T.);
#2745=ORIENTED_EDGE('',*,*,#2150,.T.);
#2746=ORIENTED_EDGE('',*,*,#2102,.F.);
#2747=ORIENTED_EDGE('',*,*,#2151,.T.);
#2748=ORIENTED_EDGE('',*,*,#2109,.F.);
#2749=ORIENTED_EDGE('',*,*,#2152,.T.);
#2750=ORIENTED_EDGE('',*,*,#1935,.T.);
#2751=ORIENTED_EDGE('',*,*,#2153,.T.);
#2752=ORIENTED_EDGE('',*,*,#2154,.F.);
#2753=ORIENTED_EDGE('',*,*,#2019,.F.);
#2754=ORIENTED_EDGE('',*,*,#2155,.F.);
#2755=ORIENTED_EDGE('',*,*,#2156,.F.);
#2756=ORIENTED_EDGE('',*,*,#2132,.F.);
#2757=ORIENTED_EDGE('',*,*,#1926,.F.);
#2758=ORIENTED_EDGE('',*,*,#2157,.T.);
#2759=ORIENTED_EDGE('',*,*,#2111,.F.);
#2760=ORIENTED_EDGE('',*,*,#2158,.T.);
#2761=ORIENTED_EDGE('',*,*,#2159,.T.);
#2762=ORIENTED_EDGE('',*,*,#2116,.F.);
#2763=ORIENTED_EDGE('',*,*,#2160,.T.);
#2764=ORIENTED_EDGE('',*,*,#1922,.F.);
#2765=ORIENTED_EDGE('',*,*,#2161,.T.);
#2766=ORIENTED_EDGE('',*,*,#2162,.T.);
#2767=ORIENTED_EDGE('',*,*,#2018,.F.);
#2768=ORIENTED_EDGE('',*,*,#2163,.T.);
#2769=ORIENTED_EDGE('',*,*,#1911,.F.);
#2770=ORIENTED_EDGE('',*,*,#2164,.T.);
#2771=ORIENTED_EDGE('',*,*,#2155,.T.);
#2772=ORIENTED_EDGE('',*,*,#1915,.F.);
#2773=ORIENTED_EDGE('',*,*,#2165,.T.);
#2774=ORIENTED_EDGE('',*,*,#1967,.T.);
#2775=ORIENTED_EDGE('',*,*,#2166,.T.);
#2776=ORIENTED_EDGE('',*,*,#2167,.F.);
#2777=ORIENTED_EDGE('',*,*,#2168,.T.);
#2778=ORIENTED_EDGE('',*,*,#2169,.F.);
#2779=ORIENTED_EDGE('',*,*,#2170,.F.);
#2780=ORIENTED_EDGE('',*,*,#2171,.F.);
#2781=ORIENTED_EDGE('',*,*,#2172,.F.);
#2782=ORIENTED_EDGE('',*,*,#2173,.F.);
#2783=ORIENTED_EDGE('',*,*,#2174,.T.);
#2784=ORIENTED_EDGE('',*,*,#2175,.F.);
#2785=ORIENTED_EDGE('',*,*,#2041,.T.);
#2786=ORIENTED_EDGE('',*,*,#2176,.F.);
#2787=ORIENTED_EDGE('',*,*,#2177,.F.);
#2788=ORIENTED_EDGE('',*,*,#2178,.F.);
#2789=ORIENTED_EDGE('',*,*,#2179,.F.);
#2790=ORIENTED_EDGE('',*,*,#2180,.F.);
#2791=ORIENTED_EDGE('',*,*,#2047,.T.);
#2792=ORIENTED_EDGE('',*,*,#2104,.T.);
#2793=ORIENTED_EDGE('',*,*,#2181,.T.);
#2794=ORIENTED_EDGE('',*,*,#2174,.F.);
#2795=ORIENTED_EDGE('',*,*,#2182,.T.);
#2796=ORIENTED_EDGE('',*,*,#2183,.T.);
#2797=ORIENTED_EDGE('',*,*,#2184,.T.);
#2798=ORIENTED_EDGE('',*,*,#2168,.F.);
#2799=ORIENTED_EDGE('',*,*,#2185,.T.);
#2800=ORIENTED_EDGE('',*,*,#2107,.T.);
#2801=ORIENTED_EDGE('',*,*,#2186,.T.);
#2802=ORIENTED_EDGE('',*,*,#2187,.T.);
#2803=ORIENTED_EDGE('',*,*,#2188,.T.);
#2804=ORIENTED_EDGE('',*,*,#2189,.T.);
#2805=ORIENTED_EDGE('',*,*,#1904,.F.);
#2806=ORIENTED_EDGE('',*,*,#2190,.T.);
#2807=ORIENTED_EDGE('',*,*,#2191,.T.);
#2808=ORIENTED_EDGE('',*,*,#2192,.T.);
#2809=ORIENTED_EDGE('',*,*,#2193,.T.);
#2810=ORIENTED_EDGE('',*,*,#2194,.T.);
#2811=ORIENTED_EDGE('',*,*,#2195,.F.);
#2812=ORIENTED_EDGE('',*,*,#2196,.T.);
#2813=ORIENTED_EDGE('',*,*,#2197,.T.);
#2814=ORIENTED_EDGE('',*,*,#2183,.F.);
#2815=ORIENTED_EDGE('',*,*,#2198,.T.);
#2816=ORIENTED_EDGE('',*,*,#2199,.T.);
#2817=ORIENTED_EDGE('',*,*,#2200,.T.);
#2818=ORIENTED_EDGE('',*,*,#2187,.F.);
#2819=ORIENTED_EDGE('',*,*,#2201,.T.);
#2820=ORIENTED_EDGE('',*,*,#2193,.F.);
#2821=ORIENTED_EDGE('',*,*,#2202,.T.);
#2822=ORIENTED_EDGE('',*,*,#2203,.T.);
#2823=ORIENTED_EDGE('',*,*,#2204,.T.);
#2824=ORIENTED_EDGE('',*,*,#2205,.T.);
#2825=ORIENTED_EDGE('',*,*,#2172,.T.);
#2826=ORIENTED_EDGE('',*,*,#2206,.T.);
#2827=ORIENTED_EDGE('',*,*,#2199,.F.);
#2828=ORIENTED_EDGE('',*,*,#2207,.T.);
#2829=ORIENTED_EDGE('',*,*,#2177,.T.);
#2830=ORIENTED_EDGE('',*,*,#2208,.T.);
#2831=ORIENTED_EDGE('',*,*,#2179,.T.);
#2832=ORIENTED_EDGE('',*,*,#2209,.T.);
#2833=ORIENTED_EDGE('',*,*,#2196,.F.);
#2834=ORIENTED_EDGE('',*,*,#2210,.T.);
#2835=ORIENTED_EDGE('',*,*,#2170,.T.);
#2836=ORIENTED_EDGE('',*,*,#2211,.T.);
#2837=ORIENTED_EDGE('',*,*,#2212,.T.);
#2838=ORIENTED_EDGE('',*,*,#2203,.F.);
#2839=ORIENTED_EDGE('',*,*,#2213,.T.);
#2840=ORIENTED_EDGE('',*,*,#1913,.F.);
#2841=ORIENTED_EDGE('',*,*,#2214,.T.);
#2842=ORIENTED_EDGE('',*,*,#1907,.T.);
#2843=ORIENTED_EDGE('',*,*,#2215,.F.);
#2844=ORIENTED_EDGE('',*,*,#1898,.T.);
#2845=ORIENTED_EDGE('',*,*,#2216,.F.);
#2846=ORIENTED_EDGE('',*,*,#2204,.F.);
#2847=ORIENTED_EDGE('',*,*,#2212,.F.);
#2848=ORIENTED_EDGE('',*,*,#2217,.F.);
#2849=ORIENTED_EDGE('',*,*,#2189,.F.);
#2850=ORIENTED_EDGE('',*,*,#2218,.T.);
#2851=ORIENTED_EDGE('',*,*,#1924,.F.);
#2852=ORIENTED_EDGE('',*,*,#2219,.F.);
#2853=ORIENTED_EDGE('',*,*,#2191,.F.);
#2854=ORIENTED_EDGE('',*,*,#2220,.T.);
#2855=ORIENTED_EDGE('',*,*,#2221,.F.);
#2856=ORIENTED_EDGE('',*,*,#1903,.T.);
#2857=ORIENTED_EDGE('',*,*,#2222,.F.);
#2858=ORIENTED_EDGE('',*,*,#1905,.T.);
#2859=ORIENTED_EDGE('',*,*,#2223,.F.);
#2860=ORIENTED_EDGE('',*,*,#2117,.F.);
#2861=ORIENTED_EDGE('',*,*,#2162,.F.);
#2862=ORIENTED_EDGE('',*,*,#2224,.F.);
#2863=ORIENTED_EDGE('',*,*,#2158,.F.);
#2864=ORIENTED_EDGE('',*,*,#2114,.F.);
#2865=ORIENTED_EDGE('',*,*,#2225,.F.);
#2866=ORIENTED_EDGE('',*,*,#1909,.F.);
#2867=ORIENTED_EDGE('',*,*,#2226,.T.);
#2868=ORIENTED_EDGE('',*,*,#2105,.F.);
#2869=ORIENTED_EDGE('',*,*,#2182,.F.);
#2870=ORIENTED_EDGE('',*,*,#2173,.T.);
#2871=ORIENTED_EDGE('',*,*,#2208,.F.);
#2872=ORIENTED_EDGE('',*,*,#2176,.T.);
#2873=ORIENTED_EDGE('',*,*,#2044,.F.);
#2874=ORIENTED_EDGE('',*,*,#2098,.F.);
#2875=ORIENTED_EDGE('',*,*,#2220,.F.);
#2876=ORIENTED_EDGE('',*,*,#2195,.T.);
#2877=ORIENTED_EDGE('',*,*,#2227,.F.);
#2878=ORIENTED_EDGE('',*,*,#2205,.F.);
#2879=ORIENTED_EDGE('',*,*,#2216,.T.);
#2880=ORIENTED_EDGE('',*,*,#1897,.F.);
#2881=ORIENTED_EDGE('',*,*,#2221,.T.);
#2882=ORIENTED_EDGE('',*,*,#2227,.T.);
#2883=ORIENTED_EDGE('',*,*,#2194,.F.);
#2884=ORIENTED_EDGE('',*,*,#1906,.T.);
#2885=ORIENTED_EDGE('',*,*,#2222,.T.);
#2886=ORIENTED_EDGE('',*,*,#1902,.F.);
#2887=ORIENTED_EDGE('',*,*,#1899,.F.);
#2888=ORIENTED_EDGE('',*,*,#2215,.T.);
#2889=ORIENTED_EDGE('',*,*,#1894,.F.);
#2890=ORIENTED_EDGE('',*,*,#1893,.F.);
#2891=ORIENTED_EDGE('',*,*,#1896,.F.);
#2892=ORIENTED_EDGE('',*,*,#1901,.T.);
#2893=ORIENTED_EDGE('',*,*,#2228,.F.);
#2894=ORIENTED_EDGE('',*,*,#2048,.F.);
#2895=ORIENTED_EDGE('',*,*,#2180,.T.);
#2896=ORIENTED_EDGE('',*,*,#2210,.F.);
#2897=ORIENTED_EDGE('',*,*,#2198,.F.);
#2898=ORIENTED_EDGE('',*,*,#2186,.F.);
#2899=ORIENTED_EDGE('',*,*,#2110,.F.);
#2900=ORIENTED_EDGE('',*,*,#2153,.F.);
#2901=ORIENTED_EDGE('',*,*,#1934,.T.);
#2902=ORIENTED_EDGE('',*,*,#2016,.F.);
#2903=ORIENTED_EDGE('',*,*,#2229,.T.);
#2904=ORIENTED_EDGE('',*,*,#1920,.F.);
#2905=ORIENTED_EDGE('',*,*,#1917,.F.);
#2906=ORIENTED_EDGE('',*,*,#2147,.F.);
#2907=ORIENTED_EDGE('',*,*,#1986,.T.);
#2908=ORIENTED_EDGE('',*,*,#2037,.F.);
#2909=ORIENTED_EDGE('',*,*,#2091,.F.);
#2910=ORIENTED_EDGE('',*,*,#2143,.F.);
#2911=ORIENTED_EDGE('',*,*,#1978,.T.);
#2912=ORIENTED_EDGE('',*,*,#2031,.F.);
#2913=ORIENTED_EDGE('',*,*,#2085,.F.);
#2914=ORIENTED_EDGE('',*,*,#2139,.F.);
#2915=ORIENTED_EDGE('',*,*,#1970,.T.);
#2916=ORIENTED_EDGE('',*,*,#2025,.F.);
#2917=ORIENTED_EDGE('',*,*,#2079,.F.);
#2918=ORIENTED_EDGE('',*,*,#2135,.F.);
#2919=ORIENTED_EDGE('',*,*,#1962,.T.);
#2920=ORIENTED_EDGE('',*,*,#2022,.F.);
#2921=ORIENTED_EDGE('',*,*,#2076,.F.);
#2922=ORIENTED_EDGE('',*,*,#2133,.F.);
#2923=ORIENTED_EDGE('',*,*,#2156,.T.);
#2924=ORIENTED_EDGE('',*,*,#2164,.F.);
#2925=ORIENTED_EDGE('',*,*,#1910,.F.);
#2926=ORIENTED_EDGE('',*,*,#2225,.T.);
#2927=ORIENTED_EDGE('',*,*,#2097,.F.);
#2928=ORIENTED_EDGE('',*,*,#2159,.F.);
#2929=ORIENTED_EDGE('',*,*,#2224,.T.);
#2930=ORIENTED_EDGE('',*,*,#2113,.F.);
#2931=ORIENTED_EDGE('',*,*,#2052,.F.);
#2932=ORIENTED_EDGE('',*,*,#1994,.F.);
#2933=ORIENTED_EDGE('',*,*,#1938,.T.);
#2934=ORIENTED_EDGE('',*,*,#2120,.F.);
#2935=ORIENTED_EDGE('',*,*,#2058,.F.);
#2936=ORIENTED_EDGE('',*,*,#2000,.F.);
#2937=ORIENTED_EDGE('',*,*,#1946,.T.);
#2938=ORIENTED_EDGE('',*,*,#2124,.F.);
#2939=ORIENTED_EDGE('',*,*,#2064,.F.);
#2940=ORIENTED_EDGE('',*,*,#2006,.F.);
#2941=ORIENTED_EDGE('',*,*,#1954,.T.);
#2942=ORIENTED_EDGE('',*,*,#2128,.F.);
#2943=ORIENTED_EDGE('',*,*,#2070,.F.);
#2944=ORIENTED_EDGE('',*,*,#2012,.F.);
#2945=ORIENTED_EDGE('',*,*,#1930,.T.);
#2946=ORIENTED_EDGE('',*,*,#2151,.F.);
#2947=ORIENTED_EDGE('',*,*,#2106,.F.);
#2948=ORIENTED_EDGE('',*,*,#2226,.F.);
#2949=ORIENTED_EDGE('',*,*,#1927,.F.);
#2950=ORIENTED_EDGE('',*,*,#2228,.T.);
#2951=ORIENTED_EDGE('',*,*,#1916,.F.);
#2952=ORIENTED_EDGE('',*,*,#2166,.F.);
#2953=ORIENTED_EDGE('',*,*,#1966,.T.);
#2954=ORIENTED_EDGE('',*,*,#2137,.F.);
#2955=ORIENTED_EDGE('',*,*,#2082,.F.);
#2956=ORIENTED_EDGE('',*,*,#2028,.F.);
#2957=ORIENTED_EDGE('',*,*,#1974,.T.);
#2958=ORIENTED_EDGE('',*,*,#2141,.F.);
#2959=ORIENTED_EDGE('',*,*,#2088,.F.);
#2960=ORIENTED_EDGE('',*,*,#2034,.F.);
#2961=ORIENTED_EDGE('',*,*,#1982,.T.);
#2962=ORIENTED_EDGE('',*,*,#2145,.F.);
#2963=ORIENTED_EDGE('',*,*,#2094,.F.);
#2964=ORIENTED_EDGE('',*,*,#2040,.F.);
#2965=ORIENTED_EDGE('',*,*,#1990,.T.);
#2966=ORIENTED_EDGE('',*,*,#2149,.F.);
#2967=ORIENTED_EDGE('',*,*,#2101,.F.);
#2968=ORIENTED_EDGE('',*,*,#2049,.F.);
#2969=ORIENTED_EDGE('',*,*,#2126,.F.);
#2970=ORIENTED_EDGE('',*,*,#1950,.T.);
#2971=ORIENTED_EDGE('',*,*,#2003,.F.);
#2972=ORIENTED_EDGE('',*,*,#2061,.F.);
#2973=ORIENTED_EDGE('',*,*,#2122,.F.);
#2974=ORIENTED_EDGE('',*,*,#1942,.T.);
#2975=ORIENTED_EDGE('',*,*,#1997,.F.);
#2976=ORIENTED_EDGE('',*,*,#2055,.F.);
#2977=ORIENTED_EDGE('',*,*,#2118,.F.);
#2978=ORIENTED_EDGE('',*,*,#2223,.T.);
#2979=ORIENTED_EDGE('',*,*,#2161,.F.);
#2980=ORIENTED_EDGE('',*,*,#1921,.F.);
#2981=ORIENTED_EDGE('',*,*,#2229,.F.);
#2982=ORIENTED_EDGE('',*,*,#2015,.F.);
#2983=ORIENTED_EDGE('',*,*,#2073,.F.);
#2984=ORIENTED_EDGE('',*,*,#2130,.F.);
#2985=ORIENTED_EDGE('',*,*,#1958,.T.);
#2986=ORIENTED_EDGE('',*,*,#2009,.F.);
#2987=ORIENTED_EDGE('',*,*,#2067,.F.);
#2988=ORIENTED_EDGE('',*,*,#2160,.F.);
#2989=ORIENTED_EDGE('',*,*,#2115,.F.);
#2990=ORIENTED_EDGE('',*,*,#2053,.F.);
#2991=ORIENTED_EDGE('',*,*,#1995,.F.);
#2992=ORIENTED_EDGE('',*,*,#1940,.T.);
#2993=ORIENTED_EDGE('',*,*,#2121,.F.);
#2994=ORIENTED_EDGE('',*,*,#2059,.F.);
#2995=ORIENTED_EDGE('',*,*,#2001,.F.);
#2996=ORIENTED_EDGE('',*,*,#1948,.T.);
#2997=ORIENTED_EDGE('',*,*,#2125,.F.);
#2998=ORIENTED_EDGE('',*,*,#2065,.F.);
#2999=ORIENTED_EDGE('',*,*,#2007,.F.);
#3000=ORIENTED_EDGE('',*,*,#1956,.T.);
#3001=ORIENTED_EDGE('',*,*,#2129,.F.);
#3002=ORIENTED_EDGE('',*,*,#2071,.F.);
#3003=ORIENTED_EDGE('',*,*,#2013,.F.);
#3004=ORIENTED_EDGE('',*,*,#1932,.T.);
#3005=ORIENTED_EDGE('',*,*,#2152,.F.);
#3006=ORIENTED_EDGE('',*,*,#2108,.F.);
#3007=ORIENTED_EDGE('',*,*,#2185,.F.);
#3008=ORIENTED_EDGE('',*,*,#2167,.T.);
#3009=ORIENTED_EDGE('',*,*,#2213,.F.);
#3010=ORIENTED_EDGE('',*,*,#2202,.F.);
#3011=ORIENTED_EDGE('',*,*,#2192,.F.);
#3012=ORIENTED_EDGE('',*,*,#2219,.T.);
#3013=ORIENTED_EDGE('',*,*,#1923,.F.);
#3014=ORIENTED_EDGE('',*,*,#2218,.F.);
#3015=ORIENTED_EDGE('',*,*,#2188,.F.);
#3016=ORIENTED_EDGE('',*,*,#2200,.F.);
#3017=ORIENTED_EDGE('',*,*,#2206,.F.);
#3018=ORIENTED_EDGE('',*,*,#2171,.T.);
#3019=ORIENTED_EDGE('',*,*,#2181,.F.);
#3020=ORIENTED_EDGE('',*,*,#2103,.F.);
#3021=ORIENTED_EDGE('',*,*,#2150,.F.);
#3022=ORIENTED_EDGE('',*,*,#1928,.T.);
#3023=ORIENTED_EDGE('',*,*,#2011,.F.);
#3024=ORIENTED_EDGE('',*,*,#2069,.F.);
#3025=ORIENTED_EDGE('',*,*,#2127,.F.);
#3026=ORIENTED_EDGE('',*,*,#1952,.T.);
#3027=ORIENTED_EDGE('',*,*,#2005,.F.);
#3028=ORIENTED_EDGE('',*,*,#2063,.F.);
#3029=ORIENTED_EDGE('',*,*,#2123,.F.);
#3030=ORIENTED_EDGE('',*,*,#1944,.T.);
#3031=ORIENTED_EDGE('',*,*,#1999,.F.);
#3032=ORIENTED_EDGE('',*,*,#2057,.F.);
#3033=ORIENTED_EDGE('',*,*,#2119,.F.);
#3034=ORIENTED_EDGE('',*,*,#1936,.T.);
#3035=ORIENTED_EDGE('',*,*,#1993,.F.);
#3036=ORIENTED_EDGE('',*,*,#2051,.F.);
#3037=ORIENTED_EDGE('',*,*,#2112,.F.);
#3038=ORIENTED_EDGE('',*,*,#2157,.F.);
#3039=ORIENTED_EDGE('',*,*,#1925,.F.);
#3040=ORIENTED_EDGE('',*,*,#2217,.T.);
#3041=ORIENTED_EDGE('',*,*,#2211,.F.);
#3042=ORIENTED_EDGE('',*,*,#2169,.T.);
#3043=ORIENTED_EDGE('',*,*,#2184,.F.);
#3044=ORIENTED_EDGE('',*,*,#2197,.F.);
#3045=ORIENTED_EDGE('',*,*,#2209,.F.);
#3046=ORIENTED_EDGE('',*,*,#2178,.T.);
#3047=ORIENTED_EDGE('',*,*,#2046,.F.);
#3048=ORIENTED_EDGE('',*,*,#2100,.F.);
#3049=ORIENTED_EDGE('',*,*,#2148,.F.);
#3050=ORIENTED_EDGE('',*,*,#1988,.T.);
#3051=ORIENTED_EDGE('',*,*,#2039,.F.);
#3052=ORIENTED_EDGE('',*,*,#2093,.F.);
#3053=ORIENTED_EDGE('',*,*,#2144,.F.);
#3054=ORIENTED_EDGE('',*,*,#1980,.T.);
#3055=ORIENTED_EDGE('',*,*,#2033,.F.);
#3056=ORIENTED_EDGE('',*,*,#2087,.F.);
#3057=ORIENTED_EDGE('',*,*,#2140,.F.);
#3058=ORIENTED_EDGE('',*,*,#1972,.T.);
#3059=ORIENTED_EDGE('',*,*,#2027,.F.);
#3060=ORIENTED_EDGE('',*,*,#2081,.F.);
#3061=ORIENTED_EDGE('',*,*,#2136,.F.);
#3062=ORIENTED_EDGE('',*,*,#1964,.T.);
#3063=ORIENTED_EDGE('',*,*,#2165,.F.);
#3064=ORIENTED_EDGE('',*,*,#1914,.F.);
#3065=ORIENTED_EDGE('',*,*,#2163,.F.);
#3066=ORIENTED_EDGE('',*,*,#2017,.F.);
#3067=ORIENTED_EDGE('',*,*,#1960,.T.);
#3068=ORIENTED_EDGE('',*,*,#2134,.F.);
#3069=ORIENTED_EDGE('',*,*,#2077,.F.);
#3070=ORIENTED_EDGE('',*,*,#2023,.F.);
#3071=ORIENTED_EDGE('',*,*,#1968,.T.);
#3072=ORIENTED_EDGE('',*,*,#2138,.F.);
#3073=ORIENTED_EDGE('',*,*,#2083,.F.);
#3074=ORIENTED_EDGE('',*,*,#2029,.F.);
#3075=ORIENTED_EDGE('',*,*,#1976,.T.);
#3076=ORIENTED_EDGE('',*,*,#2142,.F.);
#3077=ORIENTED_EDGE('',*,*,#2089,.F.);
#3078=ORIENTED_EDGE('',*,*,#2035,.F.);
#3079=ORIENTED_EDGE('',*,*,#1984,.T.);
#3080=ORIENTED_EDGE('',*,*,#2146,.F.);
#3081=ORIENTED_EDGE('',*,*,#2095,.F.);
#3082=ORIENTED_EDGE('',*,*,#2042,.F.);
#3083=ORIENTED_EDGE('',*,*,#2175,.T.);
#3084=ORIENTED_EDGE('',*,*,#2207,.F.);
#3085=ORIENTED_EDGE('',*,*,#2201,.F.);
#3086=ORIENTED_EDGE('',*,*,#2190,.F.);
#3087=ORIENTED_EDGE('',*,*,#1908,.T.);
#3088=ORIENTED_EDGE('',*,*,#2214,.F.);
#3089=ORIENTED_EDGE('',*,*,#1912,.F.);
#3090=ORIENTED_EDGE('',*,*,#2154,.T.);
#3091=ORIENTED_EDGE('',*,*,#2131,.F.);
#3092=ORIENTED_EDGE('',*,*,#2074,.F.);
#3093=ORIENTED_EDGE('',*,*,#2020,.F.);
#3094=ORIENTED_EDGE('',*,*,#1891,.T.);
#3095=ORIENTED_EDGE('',*,*,#1919,.F.);
#3449=ADVANCED_FACE('',(#987),#836,.F.);
#3450=ADVANCED_FACE('',(#988),#837,.T.);
#3451=ADVANCED_FACE('',(#989),#838,.T.);
#3452=ADVANCED_FACE('',(#990),#839,.T.);
#3453=ADVANCED_FACE('',(#991),#840,.F.);
#3454=ADVANCED_FACE('',(#992),#841,.T.);
#3455=ADVANCED_FACE('',(#993),#842,.T.);
#3456=ADVANCED_FACE('',(#994),#843,.T.);
#3457=ADVANCED_FACE('',(#995),#844,.T.);
#3458=ADVANCED_FACE('',(#996),#845,.T.);
#3459=ADVANCED_FACE('',(#997),#846,.T.);
#3460=ADVANCED_FACE('',(#998),#847,.T.);
#3461=ADVANCED_FACE('',(#999),#848,.T.);
#3462=ADVANCED_FACE('',(#1000),#849,.T.);
#3463=ADVANCED_FACE('',(#1001),#850,.T.);
#3464=ADVANCED_FACE('',(#1002),#851,.T.);
#3465=ADVANCED_FACE('',(#1003),#852,.T.);
#3466=ADVANCED_FACE('',(#1004),#853,.T.);
#3467=ADVANCED_FACE('',(#1005),#854,.T.);
#3468=ADVANCED_FACE('',(#1006),#855,.T.);
#3469=ADVANCED_FACE('',(#1007),#856,.T.);
#3470=ADVANCED_FACE('',(#1008),#152,.T.);
#3471=ADVANCED_FACE('',(#1009),#153,.T.);
#3472=ADVANCED_FACE('',(#1010),#154,.T.);
#3473=ADVANCED_FACE('',(#1011),#155,.T.);
#3474=ADVANCED_FACE('',(#1012),#156,.T.);
#3475=ADVANCED_FACE('',(#1013),#157,.T.);
#3476=ADVANCED_FACE('',(#1014),#158,.T.);
#3477=ADVANCED_FACE('',(#1015),#159,.T.);
#3478=ADVANCED_FACE('',(#1016),#160,.T.);
#3479=ADVANCED_FACE('',(#1017),#161,.T.);
#3480=ADVANCED_FACE('',(#1018),#162,.T.);
#3481=ADVANCED_FACE('',(#1019),#163,.T.);
#3482=ADVANCED_FACE('',(#1020),#164,.T.);
#3483=ADVANCED_FACE('',(#1021),#165,.T.);
#3484=ADVANCED_FACE('',(#1022),#166,.T.);
#3485=ADVANCED_FACE('',(#1023),#167,.T.);
#3486=ADVANCED_FACE('',(#1024),#168,.T.);
#3487=ADVANCED_FACE('',(#1025),#857,.T.);
#3488=ADVANCED_FACE('',(#1026),#858,.T.);
#3489=ADVANCED_FACE('',(#1027),#859,.T.);
#3490=ADVANCED_FACE('',(#1028),#860,.T.);
#3491=ADVANCED_FACE('',(#1029),#861,.T.);
#3492=ADVANCED_FACE('',(#1030),#862,.T.);
#3493=ADVANCED_FACE('',(#1031),#863,.T.);
#3494=ADVANCED_FACE('',(#1032),#864,.T.);
#3495=ADVANCED_FACE('',(#1033),#865,.T.);
#3496=ADVANCED_FACE('',(#1034),#866,.T.);
#3497=ADVANCED_FACE('',(#1035),#867,.T.);
#3498=ADVANCED_FACE('',(#1036),#868,.T.);
#3499=ADVANCED_FACE('',(#1037),#869,.T.);
#3500=ADVANCED_FACE('',(#1038),#870,.T.);
#3501=ADVANCED_FACE('',(#1039),#871,.T.);
#3502=ADVANCED_FACE('',(#1040),#872,.T.);
#3503=ADVANCED_FACE('',(#1041),#873,.T.);
#3504=ADVANCED_FACE('',(#1042),#874,.T.);
#3505=ADVANCED_FACE('',(#1043),#875,.T.);
#3506=ADVANCED_FACE('',(#1044),#169,.T.);
#3507=ADVANCED_FACE('',(#1045),#170,.T.);
#3508=ADVANCED_FACE('',(#1046),#171,.T.);
#3509=ADVANCED_FACE('',(#1047),#172,.T.);
#3510=ADVANCED_FACE('',(#1048),#173,.T.);
#3511=ADVANCED_FACE('',(#1049),#174,.T.);
#3512=ADVANCED_FACE('',(#1050),#175,.T.);
#3513=ADVANCED_FACE('',(#1051),#176,.T.);
#3514=ADVANCED_FACE('',(#1052),#177,.T.);
#3515=ADVANCED_FACE('',(#1053),#178,.T.);
#3516=ADVANCED_FACE('',(#1054),#179,.T.);
#3517=ADVANCED_FACE('',(#1055),#180,.T.);
#3518=ADVANCED_FACE('',(#1056),#181,.T.);
#3519=ADVANCED_FACE('',(#1057),#182,.T.);
#3520=ADVANCED_FACE('',(#1058),#183,.T.);
#3521=ADVANCED_FACE('',(#1059),#184,.T.);
#3522=ADVANCED_FACE('',(#1060),#185,.T.);
#3523=ADVANCED_FACE('',(#1061),#186,.T.);
#3524=ADVANCED_FACE('',(#1062),#187,.T.);
#3525=ADVANCED_FACE('',(#1063),#876,.F.);
#3526=ADVANCED_FACE('',(#1064),#397,.T.);
#3527=ADVANCED_FACE('',(#1065),#398,.T.);
#3528=ADVANCED_FACE('',(#1066),#399,.T.);
#3529=ADVANCED_FACE('',(#1067),#400,.T.);
#3530=ADVANCED_FACE('',(#1068),#877,.T.);
#3531=ADVANCED_FACE('',(#1069),#878,.T.);
#3532=ADVANCED_FACE('',(#1070),#879,.T.);
#3533=ADVANCED_FACE('',(#1071),#880,.T.);
#3534=ADVANCED_FACE('',(#1072),#188,.T.);
#3535=ADVANCED_FACE('',(#1073),#189,.T.);
#3536=ADVANCED_FACE('',(#1074),#190,.T.);
#3537=ADVANCED_FACE('',(#1075),#191,.T.);
#3538=ADVANCED_FACE('',(#1076),#881,.T.);
#3539=ADVANCED_FACE('',(#1077),#882,.T.);
#3540=ADVANCED_FACE('',(#1078),#883,.T.);
#3541=ADVANCED_FACE('',(#1079),#192,.T.);
#3542=ADVANCED_FACE('',(#1080),#193,.T.);
#3543=ADVANCED_FACE('',(#1081),#194,.T.);
#3544=ADVANCED_FACE('',(#1082),#884,.F.);
#3545=ADVANCED_FACE('',(#1083),#885,.F.);
#3546=ADVANCED_FACE('',(#1084),#886,.T.);
#3547=ADVANCED_FACE('',(#1085),#887,.F.);
#3548=ADVANCED_FACE('',(#1086),#888,.F.);
#3549=ADVANCED_FACE('',(#1087),#889,.T.);
#3550=ADVANCED_FACE('',(#1088),#401,.T.);
#3551=ADVANCED_FACE('',(#1089),#402,.T.);
#3552=ADVANCED_FACE('',(#1090,#124),#403,.F.);
#3553=ADVANCED_FACE('',(#1091,#125),#404,.F.);
#3554=ADVANCED_FACE('',(#1092),#890,.F.);
#3555=ADVANCED_FACE('',(#1093),#405,.T.);
#3556=ADVANCED_FACE('',(#1094),#406,.T.);
#3557=ADVANCED_FACE('',(#1095),#407,.T.);
#3558=ADVANCED_FACE('',(#1096),#408,.T.);
#3559=ADVANCED_FACE('',(#1097),#409,.T.);
#3560=ADVANCED_FACE('',(#1098),#410,.T.);
#3561=ADVANCED_FACE('',(#1099),#411,.T.);
#3562=ADVANCED_FACE('',(#1100),#412,.T.);
#3563=ADVANCED_FACE('',(#1101),#413,.T.);
#3564=ADVANCED_FACE('',(#1102,#126),#414,.T.);
#3654=CLOSED_SHELL('',(#3449,#3450,#3451,#3452,#3453,#3454,#3455,#3456,
#3457,#3458,#3459,#3460,#3461,#3462,#3463,#3464,#3465,#3466,#3467,#3468,
#3469,#3470,#3471,#3472,#3473,#3474,#3475,#3476,#3477,#3478,#3479,#3480,
#3481,#3482,#3483,#3484,#3485,#3486,#3487,#3488,#3489,#3490,#3491,#3492,
#3493,#3494,#3495,#3496,#3497,#3498,#3499,#3500,#3501,#3502,#3503,#3504,
#3505,#3506,#3507,#3508,#3509,#3510,#3511,#3512,#3513,#3514,#3515,#3516,
#3517,#3518,#3519,#3520,#3521,#3522,#3523,#3524,#3525,#3526,#3527,#3528,
#3529,#3530,#3531,#3532,#3533,#3534,#3535,#3536,#3537,#3538,#3539,#3540,
#3541,#3542,#3543,#3544,#3545,#3546,#3547,#3548,#3549,#3550,#3551,#3552,
#3553,#3554,#3555,#3556,#3557,#3558,#3559,#3560,#3561,#3562,#3563,#3564));
#3813=AXIS2_PLACEMENT_3D('',#5012,#4165,#4166);
#3814=AXIS2_PLACEMENT_3D('',#5013,#4167,#4168);
#3815=AXIS2_PLACEMENT_3D('',#5015,#4169,#4170);
#3816=AXIS2_PLACEMENT_3D('',#5018,#4172,#4173);
#3817=AXIS2_PLACEMENT_3D('',#5019,#4174,#4175);
#3818=AXIS2_PLACEMENT_3D('',#5021,#4176,#4177);
#3819=AXIS2_PLACEMENT_3D('',#5024,#4179,#4180);
#3820=AXIS2_PLACEMENT_3D('',#5025,#4181,#4182);
#3821=AXIS2_PLACEMENT_3D('',#5028,#4183,#4184);
#3822=AXIS2_PLACEMENT_3D('',#5045,#4185,#4186);
#3823=AXIS2_PLACEMENT_3D('',#5048,#4188,#4189);
#3824=AXIS2_PLACEMENT_3D('',#5050,#4190,#4191);
#3825=AXIS2_PLACEMENT_3D('',#5065,#4192,#4193);
#3826=AXIS2_PLACEMENT_3D('',#5087,#4194,#4195);
#3827=AXIS2_PLACEMENT_3D('',#5089,#4196,#4197);
#3828=AXIS2_PLACEMENT_3D('',#5098,#4199,#4200);
#3829=AXIS2_PLACEMENT_3D('',#5122,#4202,#4203);
#3830=AXIS2_PLACEMENT_3D('',#5147,#4206,#4207);
#3831=AXIS2_PLACEMENT_3D('',#5165,#4210,#4211);
#3832=AXIS2_PLACEMENT_3D('',#5180,#4213,#4214);
#3833=AXIS2_PLACEMENT_3D('',#5205,#4217,#4218);
#3834=AXIS2_PLACEMENT_3D('',#5207,#4220,#4221);
#3835=AXIS2_PLACEMENT_3D('',#5228,#4224,#4225);
#3836=AXIS2_PLACEMENT_3D('',#5252,#4227,#4228);
#3837=AXIS2_PLACEMENT_3D('',#5273,#4231,#4232);
#3838=AXIS2_PLACEMENT_3D('',#5294,#4235,#4236);
#3839=AXIS2_PLACEMENT_3D('',#5315,#4239,#4240);
#3840=AXIS2_PLACEMENT_3D('',#5336,#4243,#4244);
#3841=AXIS2_PLACEMENT_3D('',#5357,#4247,#4248);
#3842=AXIS2_PLACEMENT_3D('',#5378,#4251,#4252);
#3843=AXIS2_PLACEMENT_3D('',#5399,#4255,#4256);
#3844=AXIS2_PLACEMENT_3D('',#5413,#4259,#4260);
#3845=AXIS2_PLACEMENT_3D('',#5414,#4261,#4262);
#3846=AXIS2_PLACEMENT_3D('',#5435,#4265,#4266);
#3847=AXIS2_PLACEMENT_3D('',#5456,#4269,#4270);
#3848=AXIS2_PLACEMENT_3D('',#5477,#4273,#4274);
#3849=AXIS2_PLACEMENT_3D('',#5498,#4277,#4278);
#3850=AXIS2_PLACEMENT_3D('',#5519,#4281,#4282);
#3851=AXIS2_PLACEMENT_3D('',#5839,#4285,#4286);
#3852=AXIS2_PLACEMENT_3D('',#6461,#4287,#4288);
#3853=AXIS2_PLACEMENT_3D('',#7083,#4289,#4290);
#3854=AXIS2_PLACEMENT_3D('',#7705,#4291,#4292);
#3855=AXIS2_PLACEMENT_3D('',#8330,#4294,#4295);
#3856=AXIS2_PLACEMENT_3D('',#8332,#4296,#4297);
#3857=AXIS2_PLACEMENT_3D('',#8343,#4299,#4300);
#3858=AXIS2_PLACEMENT_3D('',#8650,#4301,#4302);
#3859=AXIS2_PLACEMENT_3D('',#9272,#4303,#4304);
#3860=AXIS2_PLACEMENT_3D('',#9894,#4305,#4306);
#3861=AXIS2_PLACEMENT_3D('',#10849,#4307,#4308);
#3862=AXIS2_PLACEMENT_3D('',#10856,#4309,#4310);
#3863=AXIS2_PLACEMENT_3D('',#10868,#4313,#4314);
#3864=AXIS2_PLACEMENT_3D('',#10880,#4317,#4318);
#3865=AXIS2_PLACEMENT_3D('',#10892,#4321,#4322);
#3866=AXIS2_PLACEMENT_3D('',#10904,#4325,#4326);
#3867=AXIS2_PLACEMENT_3D('',#10916,#4329,#4330);
#3868=AXIS2_PLACEMENT_3D('',#10928,#4333,#4334);
#3869=AXIS2_PLACEMENT_3D('',#10940,#4337,#4338);
#3870=AXIS2_PLACEMENT_3D('',#10952,#4341,#4342);
#3871=AXIS2_PLACEMENT_3D('',#10964,#4345,#4346);
#3872=AXIS2_PLACEMENT_3D('',#10976,#4349,#4350);
#3873=AXIS2_PLACEMENT_3D('',#10988,#4353,#4354);
#3874=AXIS2_PLACEMENT_3D('',#11000,#4357,#4358);
#3875=AXIS2_PLACEMENT_3D('',#11012,#4361,#4362);
#3876=AXIS2_PLACEMENT_3D('',#11024,#4365,#4366);
#3877=AXIS2_PLACEMENT_3D('',#11036,#4369,#4370);
#3878=AXIS2_PLACEMENT_3D('',#11053,#4373,#4374);
#3879=AXIS2_PLACEMENT_3D('',#11065,#4377,#4378);
#3880=AXIS2_PLACEMENT_3D('',#11091,#4381,#4382);
#3881=AXIS2_PLACEMENT_3D('',#11429,#4385,#4386);
#3882=AXIS2_PLACEMENT_3D('',#14177,#4389,#4390);
#3883=AXIS2_PLACEMENT_3D('',#14482,#4391,#4392);
#3884=AXIS2_PLACEMENT_3D('',#14773,#4393,#4394);
#3885=AXIS2_PLACEMENT_3D('',#15078,#4395,#4396);
#3886=AXIS2_PLACEMENT_3D('',#15369,#4397,#4398);
#3887=AXIS2_PLACEMENT_3D('',#15674,#4399,#4400);
#3888=AXIS2_PLACEMENT_3D('',#15965,#4401,#4402);
#3889=AXIS2_PLACEMENT_3D('',#16270,#4403,#4404);
#3890=AXIS2_PLACEMENT_3D('',#16882,#4405,#4406);
#3891=AXIS2_PLACEMENT_3D('',#16885,#4408,#4409);
#3892=AXIS2_PLACEMENT_3D('',#16887,#4411,#4412);
#3893=AXIS2_PLACEMENT_3D('',#16890,#4414,#4415);
#3894=AXIS2_PLACEMENT_3D('',#16892,#4417,#4418);
#3895=AXIS2_PLACEMENT_3D('',#16896,#4421,#4422);
#3896=AXIS2_PLACEMENT_3D('',#16897,#4423,#4424);
#3897=AXIS2_PLACEMENT_3D('',#16900,#4427,#4428);
#3898=AXIS2_PLACEMENT_3D('',#16903,#4431,#4432);
#3899=AXIS2_PLACEMENT_3D('',#16936,#4435,#4436);
#3900=AXIS2_PLACEMENT_3D('',#16972,#4438,#4439);
#3901=AXIS2_PLACEMENT_3D('',#16996,#4441,#4442);
#3902=AXIS2_PLACEMENT_3D('',#17301,#4444,#4445);
#3903=AXIS2_PLACEMENT_3D('',#18306,#4448,#4449);
#3904=AXIS2_PLACEMENT_3D('',#18307,#4450,#4451);
#3905=AXIS2_PLACEMENT_3D('',#18324,#4453,#4454);
#3906=AXIS2_PLACEMENT_3D('',#18342,#4457,#4458);
#3907=AXIS2_PLACEMENT_3D('',#18366,#4460,#4461);
#3908=AXIS2_PLACEMENT_3D('',#18664,#4462,#4463);
#3909=AXIS2_PLACEMENT_3D('',#19313,#4465,#4466);
#3910=AXIS2_PLACEMENT_3D('',#19318,#4471,#4472);
#3911=AXIS2_PLACEMENT_3D('',#19322,#4475,#4476);
#3912=AXIS2_PLACEMENT_3D('',#19325,#4479,#4480);
#3913=AXIS2_PLACEMENT_3D('',#19327,#4482,#4483);
#3914=AXIS2_PLACEMENT_3D('',#19329,#4485,#4486);
#3915=AXIS2_PLACEMENT_3D('',#19332,#4489,#4490);
#3916=AXIS2_PLACEMENT_3D('',#19333,#4491,#4492);
#3917=AXIS2_PLACEMENT_3D('',#19334,#4493,#4494);
#3918=AXIS2_PLACEMENT_3D('',#19335,#4495,#4496);
#3919=AXIS2_PLACEMENT_3D('',#19336,#4497,#4498);
#3920=AXIS2_PLACEMENT_3D('',#19337,#4499,#4500);
#3921=AXIS2_PLACEMENT_3D('',#19338,#4501,#4502);
#3922=AXIS2_PLACEMENT_3D('',#19341,#4505,#4506);
#3923=AXIS2_PLACEMENT_3D('',#19342,#4507,#4508);
#3924=AXIS2_PLACEMENT_3D('',#19343,#4509,#4510);
#3925=AXIS2_PLACEMENT_3D('',#19344,#4511,#4512);
#3926=AXIS2_PLACEMENT_3D('',#19345,#4513,#4514);
#3927=AXIS2_PLACEMENT_3D('',#19346,#4515,#4516);
#3928=AXIS2_PLACEMENT_3D('',#19347,#4517,#4518);
#3929=AXIS2_PLACEMENT_3D('',#19348,#4519,#4520);
#3930=AXIS2_PLACEMENT_3D('',#19349,#4521,#4522);
#3931=AXIS2_PLACEMENT_3D('',#19350,#4523,#4524);
#4165=DIRECTION('axis',(0.,0.,1.));
#4166=DIRECTION('refdir',(1.,0.,0.));
#4167=DIRECTION('center_axis',(0.,-1.,0.));
#4168=DIRECTION('ref_axis',(0.,0.,-1.));
#4169=DIRECTION('center_axis',(0.,-1.,0.));
#4170=DIRECTION('ref_axis',(0.,0.,-1.));
#4171=DIRECTION('',(0.,-1.,0.));
#4172=DIRECTION('center_axis',(0.,-1.,0.));
#4173=DIRECTION('ref_axis',(0.,0.,-1.));
#4174=DIRECTION('center_axis',(0.,-1.,0.));
#4175=DIRECTION('ref_axis',(0.,0.,-1.));
#4176=DIRECTION('center_axis',(0.,1.,0.));
#4177=DIRECTION('ref_axis',(0.,0.,1.));
#4178=DIRECTION('',(0.,1.,0.));
#4179=DIRECTION('center_axis',(0.,-1.,0.));
#4180=DIRECTION('ref_axis',(0.,0.,-1.));
#4181=DIRECTION('center_axis',(0.,1.,0.));
#4182=DIRECTION('ref_axis',(0.,0.,1.));
#4183=DIRECTION('center_axis',(0.,-1.,0.));
#4184=DIRECTION('ref_axis',(0.,0.,-1.));
#4185=DIRECTION('center_axis',(0.,-1.,0.));
#4186=DIRECTION('ref_axis',(0.,0.,-1.));
#4187=DIRECTION('',(0.,-1.,0.));
#4188=DIRECTION('center_axis',(0.,-1.,0.));
#4189=DIRECTION('ref_axis',(0.,0.,-1.));
#4190=DIRECTION('center_axis',(0.,-1.,0.));
#4191=DIRECTION('ref_axis',(0.,0.,-1.));
#4192=DIRECTION('center_axis',(0.,-1.,0.));
#4193=DIRECTION('ref_axis',(0.,0.,-1.));
#4194=DIRECTION('center_axis',(0.997075912644082,0.00470397725131907,-0.0762725181372069));
#4195=DIRECTION('ref_axis',(-0.0696482235815162,-0.354761993301017,-0.932358864955457));
#4196=DIRECTION('center_axis',(0.,-1.,0.));
#4197=DIRECTION('ref_axis',(0.,0.,-1.));
#4198=DIRECTION('',(0.,-1.,0.));
#4199=DIRECTION('center_axis',(0.,-1.,0.));
#4200=DIRECTION('ref_axis',(0.,0.,-1.));
#4201=DIRECTION('',(0.,1.,0.));
#4202=DIRECTION('center_axis',(0.,1.,0.));
#4203=DIRECTION('ref_axis',(0.,0.,1.));
#4204=DIRECTION('',(0.,-1.,0.));
#4205=DIRECTION('',(0.,1.,0.));
#4206=DIRECTION('center_axis',(0.,1.,0.));
#4207=DIRECTION('ref_axis',(0.,0.,1.));
#4208=DIRECTION('',(1.10691650854818E-16,-1.,-2.86740941221399E-8));
#4209=DIRECTION('',(0.,-1.,0.));
#4210=DIRECTION('center_axis',(0.,-1.,0.));
#4211=DIRECTION('ref_axis',(0.,0.,-1.));
#4212=DIRECTION('',(0.,1.,0.));
#4213=DIRECTION('center_axis',(0.,1.,0.));
#4214=DIRECTION('ref_axis',(0.,0.,1.));
#4215=DIRECTION('',(0.,-1.,0.));
#4216=DIRECTION('',(0.,1.,0.));
#4217=DIRECTION('center_axis',(0.,1.,0.));
#4218=DIRECTION('ref_axis',(0.,0.,1.));
#4219=DIRECTION('',(0.,-1.,0.));
#4220=DIRECTION('center_axis',(0.,-1.,0.));
#4221=DIRECTION('ref_axis',(0.,0.,-1.));
#4222=DIRECTION('',(0.,1.,0.));
#4223=DIRECTION('',(0.,-1.,0.));
#4224=DIRECTION('center_axis',(0.,-1.,0.));
#4225=DIRECTION('ref_axis',(0.,0.,-1.));
#4226=DIRECTION('',(0.,-1.,0.));
#4227=DIRECTION('center_axis',(0.,-1.,0.));
#4228=DIRECTION('ref_axis',(0.,0.,-1.));
#4229=DIRECTION('',(0.,1.,0.));
#4230=DIRECTION('',(0.,-1.,0.));
#4231=DIRECTION('center_axis',(0.,-1.,0.));
#4232=DIRECTION('ref_axis',(0.,0.,-1.));
#4233=DIRECTION('',(0.,-1.,0.));
#4234=DIRECTION('',(0.,1.,0.));
#4235=DIRECTION('center_axis',(0.,-1.,0.));
#4236=DIRECTION('ref_axis',(0.,0.,-1.));
#4237=DIRECTION('',(0.,1.,0.));
#4238=DIRECTION('',(0.,-1.,0.));
#4239=DIRECTION('center_axis',(0.,-1.,0.));
#4240=DIRECTION('ref_axis',(0.,0.,-1.));
#4241=DIRECTION('',(0.,-1.,0.));
#4242=DIRECTION('',(0.,1.,0.));
#4243=DIRECTION('center_axis',(0.,-1.,0.));
#4244=DIRECTION('ref_axis',(0.,0.,-1.));
#4245=DIRECTION('',(0.,1.,0.));
#4246=DIRECTION('',(0.,-1.,0.));
#4247=DIRECTION('center_axis',(0.,-1.,0.));
#4248=DIRECTION('ref_axis',(0.,0.,-1.));
#4249=DIRECTION('',(0.,-1.,0.));
#4250=DIRECTION('',(0.,1.,0.));
#4251=DIRECTION('center_axis',(0.,-1.,0.));
#4252=DIRECTION('ref_axis',(0.,0.,-1.));
#4253=DIRECTION('',(0.,-1.,0.));
#4254=DIRECTION('',(0.,1.,0.));
#4255=DIRECTION('center_axis',(0.,-1.,0.));
#4256=DIRECTION('ref_axis',(0.,0.,-1.));
#4257=DIRECTION('',(0.,1.,0.));
#4258=DIRECTION('',(0.,-1.,0.));
#4259=DIRECTION('center_axis',(0.,1.,0.));
#4260=DIRECTION('ref_axis',(0.,0.,1.));
#4261=DIRECTION('center_axis',(0.,-1.,0.));
#4262=DIRECTION('ref_axis',(0.,0.,-1.));
#4263=DIRECTION('',(0.,-1.,0.));
#4264=DIRECTION('',(0.,1.,0.));
#4265=DIRECTION('center_axis',(0.,-1.,0.));
#4266=DIRECTION('ref_axis',(0.,0.,-1.));
#4267=DIRECTION('',(0.,1.,0.));
#4268=DIRECTION('',(0.,-1.,0.));
#4269=DIRECTION('center_axis',(0.,-1.,0.));
#4270=DIRECTION('ref_axis',(0.,0.,-1.));
#4271=DIRECTION('',(0.,-1.,0.));
#4272=DIRECTION('',(0.,1.,0.));
#4273=DIRECTION('center_axis',(0.,-1.,0.));
#4274=DIRECTION('ref_axis',(0.,0.,-1.));
#4275=DIRECTION('',(0.,1.,0.));
#4276=DIRECTION('',(0.,-1.,0.));
#4277=DIRECTION('center_axis',(0.,-1.,0.));
#4278=DIRECTION('ref_axis',(0.,0.,-1.));
#4279=DIRECTION('',(0.,-1.,0.));
#4280=DIRECTION('',(0.,1.,0.));
#4281=DIRECTION('center_axis',(0.,-1.,0.));
#4282=DIRECTION('ref_axis',(0.,0.,-1.));
#4283=DIRECTION('',(0.,1.,0.));
#4284=DIRECTION('',(0.,-1.,0.));
#4285=DIRECTION('center_axis',(-3.19907349870672E-11,5.57863918680909E-11,
-1.));
#4286=DIRECTION('ref_axis',(0.497276552988426,-0.86759208724374,-6.43080746094552E-11));
#4287=DIRECTION('center_axis',(1.44525360935827E-11,-2.51909259187994E-11,
-1.));
#4288=DIRECTION('ref_axis',(0.497276552986562,-0.867592087244808,2.90423553376484E-11));
#4289=DIRECTION('center_axis',(2.06438449760594E-11,-3.59885479736367E-11,
-1.));
#4290=DIRECTION('ref_axis',(0.497276552992529,-0.867592087241388,4.14890795036576E-11));
#4291=DIRECTION('center_axis',(2.49698601097415E-10,-4.35514137287291E-10,
-1.));
#4292=DIRECTION('ref_axis',(0.497276552985414,-0.867592087245466,5.02017879038053E-10));
#4293=DIRECTION('',(-0.000444989806894056,-0.497981067250872,-0.867187787416171));
#4294=DIRECTION('center_axis',(-1.08672663735946E-6,-0.999999999999405,
-9.69822234025278E-8));
#4295=DIRECTION('ref_axis',(-0.993173427402032,1.09062071306982E-6,-0.116647087838961));
#4296=DIRECTION('center_axis',(0.00428782528366409,0.999862759747476,-0.0160023818382871));
#4297=DIRECTION('ref_axis',(-0.996010901071261,0.0028439177098952,-0.0891863054469385));
#4298=DIRECTION('',(-0.866340788146811,0.499453339955959,0.));
#4299=DIRECTION('center_axis',(-1.,-3.60743552086608E-12,-2.06811073586693E-12));
#4300=DIRECTION('ref_axis',(4.15820547561974E-12,-0.867588616792801,-0.497282607791137));
#4301=DIRECTION('center_axis',(-1.,2.25457668866882E-10,1.29269218462105E-10));
#4302=DIRECTION('ref_axis',(-2.59887841129028E-10,-0.867588616793689,-0.497282607789588));
#4303=DIRECTION('center_axis',(-1.,2.36263581335445E-10,1.35502142240452E-10));
#4304=DIRECTION('ref_axis',(-2.72362452364694E-10,-0.867588616792773,-0.497282607791186));
#4305=DIRECTION('center_axis',(-1.,-8.29625555327683E-11,-4.75813038765708E-11));
#4306=DIRECTION('ref_axis',(9.56387236821049E-11,-0.867588616796214,-0.497282607785183));
#4307=DIRECTION('center_axis',(0.0317847666407182,0.865934893847345,-0.499145758498639));
#4308=DIRECTION('ref_axis',(-0.999494736640691,0.0275404977324392,-0.0158679681183856));
#4309=DIRECTION('center_axis',(7.10542735760101E-15,1.,-2.08198488598457E-15));
#4310=DIRECTION('ref_axis',(-1.,7.11179816109987E-15,-1.28035472349601E-15));
#4311=DIRECTION('',(7.105427357601E-15,-1.,-8.88178419700125E-16));
#4312=DIRECTION('',(-4.44089209850063E-16,1.,7.105427357601E-15));
#4313=DIRECTION('center_axis',(7.10542735760101E-15,1.,-2.08198488598457E-15));
#4314=DIRECTION('ref_axis',(-1.,7.11179816109987E-15,-1.28035472349601E-15));
#4315=DIRECTION('',(-7.105427357601E-15,1.,-8.88178419700125E-16));
#4316=DIRECTION('',(4.44089209850063E-16,-1.,1.4210854715202E-14));
#4317=DIRECTION('center_axis',(7.10542735760101E-15,1.,-2.08198488598457E-15));
#4318=DIRECTION('ref_axis',(-1.,7.11179816109987E-15,-1.28035472349601E-15));
#4319=DIRECTION('',(1.4210854715202E-14,-1.,0.));
#4320=DIRECTION('',(0.,1.,0.));
#4321=DIRECTION('center_axis',(7.10542735760101E-15,1.,-2.08198488598457E-15));
#4322=DIRECTION('ref_axis',(-1.,7.11179816109987E-15,-1.28035472349601E-15));
#4323=DIRECTION('',(-7.10542735760105E-15,1.,-8.88178419700132E-16));
#4324=DIRECTION('',(0.,-1.,7.105427357601E-15));
#4325=DIRECTION('center_axis',(7.10542735760101E-15,1.,-2.08198488598457E-15));
#4326=DIRECTION('ref_axis',(-1.,7.11179816109987E-15,-1.28035472349601E-15));
#4327=DIRECTION('',(1.4210854715202E-14,-1.,0.));
#4328=DIRECTION('',(-8.88178419700119E-16,1.,1.42108547152019E-14));
#4329=DIRECTION('center_axis',(7.10542735760101E-15,1.,-2.08198488598457E-15));
#4330=DIRECTION('ref_axis',(-1.,7.11179816109987E-15,-1.28035472349601E-15));
#4331=DIRECTION('',(-7.10542735760095E-15,1.,-8.88178419700119E-16));
#4332=DIRECTION('',(0.,-1.,7.10542735760095E-15));
#4333=DIRECTION('center_axis',(7.10542735760101E-15,1.,-2.08198488598457E-15));
#4334=DIRECTION('ref_axis',(-1.,7.11179816109987E-15,-1.28035472349601E-15));
#4335=DIRECTION('',(7.10542735760098E-15,-1.,-8.88178419700122E-16));
#4336=DIRECTION('',(-4.44089209850063E-16,1.,7.105427357601E-15));
#4337=DIRECTION('center_axis',(7.10542735760101E-15,1.,-2.08198488598457E-15));
#4338=DIRECTION('ref_axis',(-1.,7.11179816109987E-15,-1.28035472349601E-15));
#4339=DIRECTION('',(-7.10542735760095E-15,1.,0.));
#4340=DIRECTION('',(4.44089209850069E-16,-1.,7.1054273576011E-15));
#4341=DIRECTION('center_axis',(7.10542735760101E-15,1.,-2.08198488598457E-15));
#4342=DIRECTION('ref_axis',(-1.,7.11179816109987E-15,-1.28035472349601E-15));
#4343=DIRECTION('',(0.,1.,4.44089209850059E-16));
#4344=DIRECTION('',(-8.88178419700113E-16,-1.,-7.1054273576009E-15));
#4345=DIRECTION('center_axis',(7.10542735760101E-15,1.,-2.08198488598457E-15));
#4346=DIRECTION('ref_axis',(-1.,7.11179816109987E-15,-1.28035472349601E-15));
#4347=DIRECTION('',(7.105427357601E-15,1.,1.33226762955019E-15));
#4348=DIRECTION('',(-4.44089209850066E-16,-1.,-1.42108547152021E-14));
#4349=DIRECTION('center_axis',(7.10542735760101E-15,1.,-2.08198488598457E-15));
#4350=DIRECTION('ref_axis',(-1.,7.11179816109987E-15,-1.28035472349601E-15));
#4351=DIRECTION('',(-1.42108547152019E-14,-1.,4.44089209850059E-16));
#4352=DIRECTION('',(2.22044604925028E-15,1.,0.));
#4353=DIRECTION('center_axis',(7.10542735760101E-15,1.,-2.08198488598457E-15));
#4354=DIRECTION('ref_axis',(-1.,7.11179816109987E-15,-1.28035472349601E-15));
#4355=DIRECTION('',(7.105427357601E-15,1.,1.33226762955019E-15));
#4356=DIRECTION('',(0.,-1.,-1.42108547152018E-14));
#4357=DIRECTION('center_axis',(7.10542735760101E-15,1.,-2.08198488598457E-15));
#4358=DIRECTION('ref_axis',(-1.,7.11179816109987E-15,-1.28035472349601E-15));
#4359=DIRECTION('',(-7.10542735760095E-15,-1.,0.));
#4360=DIRECTION('',(0.,1.,-7.10542735760105E-15));
#4361=DIRECTION('center_axis',(7.10542735760101E-15,1.,-2.08198488598457E-15));
#4362=DIRECTION('ref_axis',(-1.,7.11179816109987E-15,-1.28035472349601E-15));
#4363=DIRECTION('',(7.105427357601E-15,1.,0.));
#4364=DIRECTION('',(-1.33226762955017E-15,-1.,0.));
#4365=DIRECTION('center_axis',(7.10542735760101E-15,1.,-2.08198488598457E-15));
#4366=DIRECTION('ref_axis',(-1.,7.11179816109987E-15,-1.28035472349601E-15));
#4367=DIRECTION('',(-7.105427357601E-15,-1.,0.));
#4368=DIRECTION('',(0.,1.,-7.1054273576011E-15));
#4369=DIRECTION('center_axis',(7.10542735760101E-15,1.,-2.08198488598457E-15));
#4370=DIRECTION('ref_axis',(-1.,7.11179816109987E-15,-1.28035472349601E-15));
#4371=DIRECTION('',(0.,1.,8.88178419700119E-16));
#4372=DIRECTION('',(0.,-0.999999999998377,1.80186440497577E-6));
#4373=DIRECTION('center_axis',(7.10542735760101E-15,1.,-2.08198488598457E-15));
#4374=DIRECTION('ref_axis',(-1.,7.11179816109987E-15,-1.28035472349601E-15));
#4375=DIRECTION('',(-7.10542735760095E-15,-1.,8.88178419700119E-16));
#4376=DIRECTION('',(-4.44089209850063E-16,1.,-7.105427357601E-15));
#4377=DIRECTION('center_axis',(7.10542735760101E-15,1.,-2.08198488598457E-15));
#4378=DIRECTION('ref_axis',(-1.,7.11179816109987E-15,-1.28035472349601E-15));
#4379=DIRECTION('',(0.,-1.,0.));
#4380=DIRECTION('',(0.,0.999999999996769,-2.54218367618327E-6));
#4381=DIRECTION('center_axis',(7.10542735760101E-15,1.,-2.08198488598457E-15));
#4382=DIRECTION('ref_axis',(-1.,7.11179816109987E-15,-1.28035472349601E-15));
#4383=DIRECTION('',(-7.10542735760098E-15,1.,0.));
#4384=DIRECTION('',(4.95945076311269E-14,0.498176579235464,0.867075599876534));
#4385=DIRECTION('center_axis',(-0.0160023818376506,-0.999862759747457,-0.00428782529044036));
#4386=DIRECTION('ref_axis',(0.320435510218814,-0.00106615058948748,-0.947269733029473));
#4387=DIRECTION('',(0.867428142068955,0.497562476827584,0.));
#4388=DIRECTION('',(-1.14214331302317E-14,-0.499456113421034,-0.866339189213068));
#4389=DIRECTION('center_axis',(2.06991832786293E-12,-3.59568180778876E-12,
-1.));
#4390=DIRECTION('ref_axis',(-0.497276552985882,0.867592087245198,-4.14890694656058E-12));
#4391=DIRECTION('center_axis',(-1.,-1.62328252343351E-10,-9.30760508218548E-11));
#4392=DIRECTION('ref_axis',(-1.87119245189999E-10,0.867588616794545,0.497282607788095));
#4393=DIRECTION('center_axis',(-2.05762092679575E-12,3.60273289486777E-12,
-1.));
#4394=DIRECTION('ref_axis',(-0.49727655299199,0.867592087241697,4.14890918496442E-12));
#4395=DIRECTION('center_axis',(-1.,-3.60038429955364E-12,-2.08040818675628E-12));
#4396=DIRECTION('ref_axis',(-4.15820323995394E-12,0.867588616794733,0.497282607787766));
#4397=DIRECTION('center_axis',(9.83463793864226E-13,-1.82736732563426E-12,
-1.));
#4398=DIRECTION('ref_axis',(-0.497276552989786,0.86759208724296,-2.07446291715088E-12));
#4399=DIRECTION('center_axis',(-1.,-7.20764353951641E-12,-4.14882635868306E-12));
#4400=DIRECTION('ref_axis',(-8.31640865557086E-12,0.867588616794545,0.497282607788095));
#4401=DIRECTION('center_axis',(-3.71471154516616E-10,6.47861553957569E-10,
-1.));
#4402=DIRECTION('ref_axis',(-0.497276552987665,0.867592087244176,7.46803453090951E-10));
#4403=DIRECTION('center_axis',(-1.,2.43483740809469E-10,1.39629140633371E-10));
#4404=DIRECTION('ref_axis',(2.80678865049538E-10,0.867588616792504,0.497282607791656));
#4405=DIRECTION('center_axis',(0.,1.,0.));
#4406=DIRECTION('ref_axis',(0.,0.,1.));
#4407=DIRECTION('',(0.,1.,0.));
#4408=DIRECTION('center_axis',(0.,1.,0.));
#4409=DIRECTION('ref_axis',(0.,0.,1.));
#4410=DIRECTION('',(0.,-1.,0.));
#4411=DIRECTION('center_axis',(0.,1.,0.));
#4412=DIRECTION('ref_axis',(0.,0.,1.));
#4413=DIRECTION('',(1.,0.,0.));
#4414=DIRECTION('center_axis',(0.,1.,0.));
#4415=DIRECTION('ref_axis',(0.,0.,1.));
#4416=DIRECTION('',(0.,0.,1.));
#4417=DIRECTION('center_axis',(0.,1.,0.));
#4418=DIRECTION('ref_axis',(0.,0.,1.));
#4419=DIRECTION('',(-1.,0.,0.));
#4420=DIRECTION('',(0.,0.,1.));
#4421=DIRECTION('center_axis',(0.,1.,0.));
#4422=DIRECTION('ref_axis',(0.,0.,1.));
#4423=DIRECTION('center_axis',(0.,1.,0.));
#4424=DIRECTION('ref_axis',(0.,0.,1.));
#4425=DIRECTION('',(1.,0.,0.));
#4426=DIRECTION('',(0.,0.,-1.));
#4427=DIRECTION('center_axis',(0.,1.,0.));
#4428=DIRECTION('ref_axis',(0.,0.,1.));
#4429=DIRECTION('',(-1.,0.,0.));
#4430=DIRECTION('',(0.,0.,-1.));
#4431=DIRECTION('center_axis',(0.,-1.,0.));
#4432=DIRECTION('ref_axis',(-7.6571373978539E-16,0.,1.));
#4433=DIRECTION('',(0.,-1.,0.));
#4434=DIRECTION('',(0.,1.,0.));
#4435=DIRECTION('center_axis',(0.,-1.,0.));
#4436=DIRECTION('ref_axis',(0.,0.,-1.));
#4437=DIRECTION('',(0.,1.,0.));
#4438=DIRECTION('center_axis',(0.,-1.,0.));
#4439=DIRECTION('ref_axis',(0.,0.,-1.));
#4440=DIRECTION('',(0.,-1.,0.));
#4441=DIRECTION('center_axis',(0.,-1.,0.));
#4442=DIRECTION('ref_axis',(0.,0.,-1.));
#4443=DIRECTION('',(0.,1.,0.));
#4444=DIRECTION('center_axis',(1.72297863328963E-10,-3.00549238109471E-10,
-1.));
#4445=DIRECTION('ref_axis',(0.497276552987805,-0.867592087244096,3.4643382838297E-10));
#4446=DIRECTION('',(-0.867432536984531,-0.497554814850163,2.89113612764477E-13));
#4447=DIRECTION('',(0.866169166920262,0.499750912231943,-1.16493376777939E-12));
#4448=DIRECTION('center_axis',(0.00452829227180621,-0.999846933665442,-0.0168998168307887));
#4449=DIRECTION('ref_axis',(0.987523822777422,0.0018110409973824,0.157459263232029));
#4450=DIRECTION('center_axis',(7.10542735760101E-15,1.,-2.08198488598457E-15));
#4451=DIRECTION('ref_axis',(-1.,7.11179816109987E-15,-1.28035472349601E-15));
#4452=DIRECTION('',(0.,-1.,-4.44089209850063E-16));
#4453=DIRECTION('center_axis',(7.10542735760101E-15,1.,-2.08198488598457E-15));
#4454=DIRECTION('ref_axis',(-1.,7.11179816109987E-15,-1.28035472349601E-15));
#4455=DIRECTION('',(0.,-1.,0.));
#4456=DIRECTION('',(7.105427357601E-15,1.,0.));
#4457=DIRECTION('center_axis',(7.10542735760101E-15,1.,-2.08198488598457E-15));
#4458=DIRECTION('ref_axis',(-1.,7.11179816109987E-15,-1.28035472349601E-15));
#4459=DIRECTION('',(-7.10542735760098E-15,1.,-4.44089209850061E-16));
#4460=DIRECTION('center_axis',(-1.29725002468514E-15,1.,1.01665643334203E-15));
#4461=DIRECTION('ref_axis',(-0.522944117603135,-1.55000729152176E-15,0.852366969012924));
#4462=DIRECTION('center_axis',(7.17477267547079E-12,-1.26249893789538E-11,
-1.));
#4463=DIRECTION('ref_axis',(-0.497276552987957,0.867592087244008,-1.45211870849278E-11));
#4464=DIRECTION('',(-0.866183392751839,-0.499726255184689,9.87106629258188E-14));
#4465=DIRECTION('center_axis',(-1.,0.,0.));
#4466=DIRECTION('ref_axis',(0.,0.,1.));
#4467=DIRECTION('',(-1.,0.,0.));
#4468=DIRECTION('',(-1.,0.,0.));
#4469=DIRECTION('',(1.,0.,0.));
#4470=DIRECTION('',(-1.,0.,0.));
#4471=DIRECTION('center_axis',(-1.,0.,0.));
#4472=DIRECTION('ref_axis',(0.,0.,1.));
#4473=DIRECTION('',(-1.,0.,0.));
#4474=DIRECTION('',(-1.,0.,0.));
#4475=DIRECTION('center_axis',(0.998237545662555,0.00530728060715426,0.0591069809934184));
#4476=DIRECTION('ref_axis',(0.0565541720181457,-0.386905875987754,-0.920383327072743));
#4477=DIRECTION('',(1.,0.,0.));
#4478=DIRECTION('',(-1.,0.,0.));
#4479=DIRECTION('center_axis',(0.,-1.,0.));
#4480=DIRECTION('ref_axis',(0.,0.,-1.));
#4481=DIRECTION('',(0.,1.,0.));
#4482=DIRECTION('center_axis',(0.,1.,0.));
#4483=DIRECTION('ref_axis',(0.,0.,1.));
#4484=DIRECTION('',(0.,1.,0.));
#4485=DIRECTION('center_axis',(0.,0.,-1.));
#4486=DIRECTION('ref_axis',(-1.,0.,0.));
#4487=DIRECTION('',(0.,0.,-1.));
#4488=DIRECTION('',(0.,0.,-1.));
#4489=DIRECTION('center_axis',(0.,-1.,0.));
#4490=DIRECTION('ref_axis',(0.,0.,-1.));
#4491=DIRECTION('center_axis',(0.,-1.,0.));
#4492=DIRECTION('ref_axis',(0.,0.,-1.));
#4493=DIRECTION('center_axis',(0.,-1.,0.));
#4494=DIRECTION('ref_axis',(0.,0.,-1.));
#4495=DIRECTION('center_axis',(0.,-1.,0.));
#4496=DIRECTION('ref_axis',(0.,0.,-1.));
#4497=DIRECTION('center_axis',(0.,1.,0.));
#4498=DIRECTION('ref_axis',(0.,0.,1.));
#4499=DIRECTION('center_axis',(0.,-1.,0.));
#4500=DIRECTION('ref_axis',(0.,0.,-1.));
#4501=DIRECTION('center_axis',(0.,0.,-1.));
#4502=DIRECTION('ref_axis',(-1.,0.,0.));
#4503=DIRECTION('',(0.,0.,-1.));
#4504=DIRECTION('',(0.,0.,-1.));
#4505=DIRECTION('center_axis',(1.,1.27629810543002E-16,0.));
#4506=DIRECTION('ref_axis',(-1.27629810543002E-16,1.,0.));
#4507=DIRECTION('center_axis',(-1.,0.,0.));
#4508=DIRECTION('ref_axis',(0.,0.,1.));
#4509=DIRECTION('center_axis',(1.,1.27629810543002E-16,0.));
#4510=DIRECTION('ref_axis',(-1.27629810543002E-16,1.,0.));
#4511=DIRECTION('center_axis',(-1.,0.,0.));
#4512=DIRECTION('ref_axis',(0.,0.,1.));
#4513=DIRECTION('center_axis',(0.,0.,-1.));
#4514=DIRECTION('ref_axis',(-1.,0.,0.));
#4515=DIRECTION('center_axis',(0.,-1.40464835892948E-16,1.));
#4516=DIRECTION('ref_axis',(0.,-1.,-1.40464835892948E-16));
#4517=DIRECTION('center_axis',(0.,0.,-1.));
#4518=DIRECTION('ref_axis',(-1.,0.,0.));
#4519=DIRECTION('center_axis',(0.,-1.40464835892948E-16,1.));
#4520=DIRECTION('ref_axis',(0.,-1.,-1.40464835892948E-16));
#4521=DIRECTION('center_axis',(0.,-1.40464835892948E-16,1.));
#4522=DIRECTION('ref_axis',(0.,-1.,-1.40464835892948E-16));
#4523=DIRECTION('center_axis',(0.,-1.,0.));
#4524=DIRECTION('ref_axis',(0.,0.,-1.));
#5012=CARTESIAN_POINT('',(0.,0.,0.));
#5013=CARTESIAN_POINT('Origin',(0.,3.42,0.));
#5014=CARTESIAN_POINT('',(-4.89858719658941E-15,3.42,40.));
#5015=CARTESIAN_POINT('Origin',(0.,3.42,0.));
#5016=CARTESIAN_POINT('',(-4.89858719658941E-15,0.,40.));
#5017=CARTESIAN_POINT('',(-4.89858719658941E-15,3.42,40.));
#5018=CARTESIAN_POINT('Origin',(0.,0.,0.));
#5019=CARTESIAN_POINT('Origin',(0.,60.,0.));
#5020=CARTESIAN_POINT('',(-5.63337527607782E-15,0.,46.));
#5021=CARTESIAN_POINT('Origin',(0.,0.,0.));
#5022=CARTESIAN_POINT('',(-5.63337527607782E-15,20.,46.));
#5023=CARTESIAN_POINT('',(-5.63337527607782E-15,60.,46.));
#5024=CARTESIAN_POINT('Origin',(0.,20.,0.));
#5025=CARTESIAN_POINT('Origin',(0.,20.,0.));
#5026=CARTESIAN_POINT('',(39.8660227411065,28.,3.27112072623103));
#5027=CARTESIAN_POINT('',(-39.8660227411065,28.,3.27112072623103));
#5028=CARTESIAN_POINT('Origin',(0.,28.,0.));
#5029=CARTESIAN_POINT('',(-39.8000405653402,28.,-3.99459271982449));
#5030=CARTESIAN_POINT('Ctrl Pts',(-39.8000405653402,28.,-3.99459271982449));
#5031=CARTESIAN_POINT('Ctrl Pts',(-39.8202648350751,27.541880505153,-3.79308863359818));
#5032=CARTESIAN_POINT('Ctrl Pts',(-39.8478595264142,27.1249694755492,-3.5013875154554));
#5033=CARTESIAN_POINT('Ctrl Pts',(-39.902305612745,26.4396195203269,-2.81616960677907));
#5034=CARTESIAN_POINT('Ctrl Pts',(-39.9327182501717,26.1341927725789,-2.37013786718776));
#5035=CARTESIAN_POINT('Ctrl Pts',(-39.9787551488202,25.728954292425,-1.39236385403762));
#5036=CARTESIAN_POINT('Ctrl Pts',(-39.9938528018644,25.629163825102,-0.860588043983172));
#5037=CARTESIAN_POINT('Ctrl Pts',(-40.0028726554704,25.629163825102,0.136767468615171));
#5038=CARTESIAN_POINT('Ctrl Pts',(-39.9974053268697,25.7288296122476,0.668382268299115));
#5039=CARTESIAN_POINT('Ctrl Pts',(-39.9691084018832,26.1338587427398,1.64606843741232));
#5040=CARTESIAN_POINT('Ctrl Pts',(-39.9468068466375,26.4392073572614,2.09216112009085));
#5041=CARTESIAN_POINT('Ctrl Pts',(-39.90483592212,27.124631969712,2.77769565092216));
#5042=CARTESIAN_POINT('Ctrl Pts',(-39.8825619687711,27.5417352224658,3.06955273734297));
#5043=CARTESIAN_POINT('Ctrl Pts',(-39.8660227411065,28.,3.27112072623103));
#5044=CARTESIAN_POINT('',(-4.89858719658941E-15,28.,-40.));
#5045=CARTESIAN_POINT('Origin',(0.,28.,0.));
#5046=CARTESIAN_POINT('',(-4.89858719658941E-15,20.,-40.));
#5047=CARTESIAN_POINT('',(-4.89858719658941E-15,20.,-40.));
#5048=CARTESIAN_POINT('Origin',(0.,20.,0.));
#5049=CARTESIAN_POINT('',(39.8000405653402,28.,-3.99459271982449));
#5050=CARTESIAN_POINT('Origin',(0.,28.,0.));
#5051=CARTESIAN_POINT('Ctrl Pts',(39.8660227411065,28.,3.27112072623103));
#5052=CARTESIAN_POINT('Ctrl Pts',(39.8825619687711,27.5417352224658,3.06955273734297));
#5053=CARTESIAN_POINT('Ctrl Pts',(39.90483592212,27.124631969712,2.77769565092216));
#5054=CARTESIAN_POINT('Ctrl Pts',(39.9468068466375,26.4392073572614,2.09216112009085));
#5055=CARTESIAN_POINT('Ctrl Pts',(39.9691084018832,26.1338587427398,1.64606843741232));
#5056=CARTESIAN_POINT('Ctrl Pts',(39.9974053268697,25.7288296122476,0.668382268299116));
#5057=CARTESIAN_POINT('Ctrl Pts',(40.0028726554704,25.629163825102,0.136767468615172));
#5058=CARTESIAN_POINT('Ctrl Pts',(39.9938528018644,25.629163825102,-0.860588043983171));
#5059=CARTESIAN_POINT('Ctrl Pts',(39.9787551488202,25.728954292425,-1.39236385403762));
#5060=CARTESIAN_POINT('Ctrl Pts',(39.9327182501717,26.1341927725789,-2.37013786718776));
#5061=CARTESIAN_POINT('Ctrl Pts',(39.902305612745,26.4396195203269,-2.81616960677907));
#5062=CARTESIAN_POINT('Ctrl Pts',(39.8478595264142,27.1249694755492,-3.5013875154554));
#5063=CARTESIAN_POINT('Ctrl Pts',(39.8202648350751,27.541880505153,-3.79308863359818));
#5064=CARTESIAN_POINT('Ctrl Pts',(39.8000405653402,28.,-3.99459271982449));
#5065=CARTESIAN_POINT('Origin',(0.,60.,0.));
#5066=CARTESIAN_POINT('',(-45.7957082162897,30.5508791552084,-4.33048599679682));
#5067=CARTESIAN_POINT('',(45.8192253759653,28.1946814357457,-4.07413622090531));
#5068=CARTESIAN_POINT('Ctrl Pts',(-45.7957082162897,30.5508791552084,-4.3304859967968));
#5069=CARTESIAN_POINT('Ctrl Pts',(-45.2904567403498,30.4582791384642,-9.67361588686245));
#5070=CARTESIAN_POINT('Ctrl Pts',(-43.8539847608527,30.3636491983601,-14.8873227195869));
#5071=CARTESIAN_POINT('Ctrl Pts',(-39.2595475939355,30.1793388276773,-24.5606349388711));
#5072=CARTESIAN_POINT('Ctrl Pts',(-36.1445477184839,30.089019872629,-28.9501043330206));
#5073=CARTESIAN_POINT('Ctrl Pts',(-28.0998693561851,29.8910356446895,-36.9061963106983));
#5074=CARTESIAN_POINT('Ctrl Pts',(-23.0758554236481,29.7911290471386,-40.2389742761901));
#5075=CARTESIAN_POINT('Ctrl Pts',(-11.9484440491057,29.5822410004833,-44.83339037117));
#5076=CARTESIAN_POINT('Ctrl Pts',(-5.93853076275596,29.4754507871743,-46.0166322639478));
#5077=CARTESIAN_POINT('Ctrl Pts',(6.19463923460001,29.2702187768307,-45.9830112670864));
#5078=CARTESIAN_POINT('Ctrl Pts',(12.1989476144052,29.1632197696209,-44.7660144128937));
#5079=CARTESIAN_POINT('Ctrl Pts',(23.3037531300962,28.9544249372012,-40.1078138073594));
#5080=CARTESIAN_POINT('Ctrl Pts',(28.3109481824939,28.8543575036543,-36.744954507633));
#5081=CARTESIAN_POINT('Ctrl Pts',(36.3100560865774,28.6563561267642,-28.7419061208428));
#5082=CARTESIAN_POINT('Ctrl Pts',(39.398809462358,28.5662371851081,-24.3362112688292));
#5083=CARTESIAN_POINT('Ctrl Pts',(43.9371605347039,28.3817876471969,-14.6396372497778));
#5084=CARTESIAN_POINT('Ctrl Pts',(45.3439760357657,28.2871742724011,-9.4189640439544));
#5085=CARTESIAN_POINT('Ctrl Pts',(45.8192253759654,28.1946814357456,-4.07413622090525));
#5086=CARTESIAN_POINT('',(45.8262286142197,28.,-3.99459271982449));
#5087=CARTESIAN_POINT('Origin',(46.0952922108427,29.6008626071972,-0.378516324486955));
#5088=CARTESIAN_POINT('',(-45.8262286142197,28.,-3.99459271982449));
#5089=CARTESIAN_POINT('Origin',(0.,28.,0.));
#5090=CARTESIAN_POINT('',(-45.7957082162897,29.597913825102,-4.33048599679673));
#5091=CARTESIAN_POINT('Ctrl Pts',(-45.7957082162897,29.597913825102,-4.33048599679673));
#5092=CARTESIAN_POINT('Ctrl Pts',(-45.7957082162897,29.0993094464563,-4.33048599679673));
#5093=CARTESIAN_POINT('Ctrl Pts',(-45.8054776929032,28.5676691611987,-4.23078571512148));
#5094=CARTESIAN_POINT('Ctrl Pts',(-45.8242431489185,28.0524370568086,-4.01732005107389));
#5095=CARTESIAN_POINT('Ctrl Pts',(-45.8252258288706,28.0261543846796,-4.00609673885219));
#5096=CARTESIAN_POINT('Ctrl Pts',(-45.8262286142197,28.,-3.99459271982449));
#5097=CARTESIAN_POINT('',(-45.7957082162897,60.,-4.33048599679673));
#5098=CARTESIAN_POINT('Origin',(0.,60.,0.));
#5099=CARTESIAN_POINT('',(3.61293045337858,36.9438035983105,-35.8182458188427));
#5100=CARTESIAN_POINT('',(-4.32456637758084,36.9438035983105,-35.7393078506831));
#5101=CARTESIAN_POINT('Ctrl Pts',(-4.32456637758084,36.9438035983105,-35.7393078506831));
#5102=CARTESIAN_POINT('Ctrl Pts',(-4.32456637758084,36.4450208015675,-35.7393078506831));
#5103=CARTESIAN_POINT('Ctrl Pts',(-4.22479607288452,35.9133171831831,-35.7518200690335));
#5104=CARTESIAN_POINT('Ctrl Pts',(-3.81972115078383,34.9357522694673,-35.7973640118356));
#5105=CARTESIAN_POINT('Ctrl Pts',(-3.51444243124228,34.4898519148477,-35.8297856438023));
#5106=CARTESIAN_POINT('Ctrl Pts',(-2.81035536837098,33.7856002162544,-35.891877281823));
#5107=CARTESIAN_POINT('Ctrl Pts',(-2.36438104223203,33.4801763497608,-35.9256086610747));
#5108=CARTESIAN_POINT('Ctrl Pts',(-1.38661844382939,33.074889941751,-35.9766166372815));
#5109=CARTESIAN_POINT('Ctrl Pts',(-0.854788951444588,32.9750535983105,-35.9933095700074));
#5110=CARTESIAN_POINT('Ctrl Pts',(0.142732488159273,32.9750535983105,-36.0031693423161));
#5111=CARTESIAN_POINT('Ctrl Pts',(0.67436622526082,33.0747383580536,-35.9970058845568));
#5112=CARTESIAN_POINT('Ctrl Pts',(1.65202206260133,33.4797702852856,-35.9654003949313));
#5113=CARTESIAN_POINT('Ctrl Pts',(2.09807056759484,33.7850992008905,-35.9405439624699));
#5114=CARTESIAN_POINT('Ctrl Pts',(2.80252582511813,34.489417022928,-35.8924857314627));
#5115=CARTESIAN_POINT('Ctrl Pts',(3.10796993106093,34.9355112883736,-35.8661668197574));
#5116=CARTESIAN_POINT('Ctrl Pts',(3.51318310448797,35.913320036691,-35.828744662717));
#5117=CARTESIAN_POINT('Ctrl Pts',(3.61293362241916,36.44506523213,-35.8182454991865));
#5118=CARTESIAN_POINT('Ctrl Pts',(3.61293362241916,36.9438035983105,-35.8182454991865));
#5119=CARTESIAN_POINT('',(-4.32456003949879,57.,-35.73930861761));
#5120=CARTESIAN_POINT('',(-4.32456003949879,60.,-35.73930861761));
#5121=CARTESIAN_POINT('',(-35.7385910610862,57.,-4.33048599679673));
#5122=CARTESIAN_POINT('Origin',(0.,57.,0.));
#5123=CARTESIAN_POINT('',(-35.7385910610862,29.597913825102,-4.33048599679673));
#5124=CARTESIAN_POINT('',(-35.7385910610862,60.,-4.33048599679673));
#5125=CARTESIAN_POINT('',(-35.8188421083191,29.597913825102,3.60701400320327));
#5126=CARTESIAN_POINT('Ctrl Pts',(-35.7385910610862,29.597913825102,-4.33048599679673));
#5127=CARTESIAN_POINT('Ctrl Pts',(-35.7385910610862,29.0991306962933,-4.33048599679673));
#5128=CARTESIAN_POINT('Ctrl Pts',(-35.7511200860441,28.5674275274957,-4.23071553786938));
#5129=CARTESIAN_POINT('Ctrl Pts',(-35.7967317559948,27.5898649766328,-3.8256420007237));
#5130=CARTESIAN_POINT('Ctrl Pts',(-35.8292042530398,27.1439664630341,-3.52036488637474));
#5131=CARTESIAN_POINT('Ctrl Pts',(-35.8914128483252,26.4397150924934,-2.81628112104011));
#5132=CARTESIAN_POINT('Ctrl Pts',(-35.925218216728,26.1342902091051,-2.37030719253055));
#5133=CARTESIAN_POINT('Ctrl Pts',(-35.9763878543241,25.7290014455195,-1.39254337628737));
#5134=CARTESIAN_POINT('Ctrl Pts',(-35.9931684759662,25.629163825102,-0.860712147213517));
#5135=CARTESIAN_POINT('Ctrl Pts',(-36.0031923000525,25.629163825102,0.13680939481454));
#5136=CARTESIAN_POINT('Ctrl Pts',(-35.9971163491985,25.7288473393432,0.66844161100349));
#5137=CARTESIAN_POINT('Ctrl Pts',(-35.9656720315245,26.1338773873715,1.64609688970905));
#5138=CARTESIAN_POINT('Ctrl Pts',(-35.9408892795961,26.4392057398786,2.09214623166637));
#5139=CARTESIAN_POINT('Ctrl Pts',(-35.8929475807102,27.1435243342817,2.79660431841842));
#5140=CARTESIAN_POINT('Ctrl Pts',(-35.8666793391538,27.5896199855471,3.10204957133501));
#5141=CARTESIAN_POINT('Ctrl Pts',(-35.8293245843937,28.5674304286977,3.50726366036052));
#5142=CARTESIAN_POINT('Ctrl Pts',(-35.8188421083191,29.0991758664567,3.60701400320327));
#5143=CARTESIAN_POINT('Ctrl Pts',(-35.8188421083191,29.597913825102,3.60701400320327));
#5144=CARTESIAN_POINT('',(-35.8188421083191,57.,3.60701400320327));
#5145=CARTESIAN_POINT('',(-35.8188421083191,60.,3.60701400320327));
#5146=CARTESIAN_POINT('',(-4.32456003949879,57.,35.73930861761));
#5147=CARTESIAN_POINT('Origin',(0.,57.,0.));
#5148=CARTESIAN_POINT('',(-4.32456320853981,36.9438035983105,35.7393079465999));
#5149=CARTESIAN_POINT('',(-4.32456003949879,57.,35.73930861761));
#5150=CARTESIAN_POINT('',(2.49793749409559E-11,32.9910360529178,36.));
#5151=CARTESIAN_POINT('Ctrl Pts',(-4.32456637758084,36.9438035983105,35.7393078506831));
#5152=CARTESIAN_POINT('Ctrl Pts',(-4.32456637758084,36.4450208015675,35.7393078506831));
#5153=CARTESIAN_POINT('Ctrl Pts',(-4.22479607288452,35.9133171831831,35.7518200690335));
#5154=CARTESIAN_POINT('Ctrl Pts',(-3.81972115078383,34.9357522694673,35.7973640118356));
#5155=CARTESIAN_POINT('Ctrl Pts',(-3.51444243124228,34.4898519148477,35.8297856438023));
#5156=CARTESIAN_POINT('Ctrl Pts',(-2.81035536837098,33.7856002162544,35.891877281823));
#5157=CARTESIAN_POINT('Ctrl Pts',(-2.36438104223203,33.4801763497608,35.9256086610747));
#5158=CARTESIAN_POINT('Ctrl Pts',(-1.38661844382939,33.074889941751,35.9766166372815));
#5159=CARTESIAN_POINT('Ctrl Pts',(-0.854788951444588,32.9750535983105,35.9933095700074));
#5160=CARTESIAN_POINT('Ctrl Pts',(-0.238725233717463,32.9750535983105,35.9993989107907));
#5161=CARTESIAN_POINT('Ctrl Pts',(-0.119781262522339,32.9802536999292,36.));
#5162=CARTESIAN_POINT('Ctrl Pts',(4.99631239159193E-11,32.9910360529178,
36.));
#5163=CARTESIAN_POINT('',(-4.40872847693047E-15,3.42,36.));
#5164=CARTESIAN_POINT('',(-4.40872847693047E-15,60.,36.));
#5165=CARTESIAN_POINT('Origin',(0.,3.42,0.));
#5166=CARTESIAN_POINT('',(3.61293362241916,36.9438035983105,35.8182454991865));
#5167=CARTESIAN_POINT('Ctrl Pts',(4.99630892214498E-11,32.9910360529178,
36.));
#5168=CARTESIAN_POINT('Ctrl Pts',(0.390221549150756,33.0261626361231,36.));
#5169=CARTESIAN_POINT('Ctrl Pts',(0.78917426933185,33.1223020523269,35.99329438987));
#5170=CARTESIAN_POINT('Ctrl Pts',(1.65202206260133,33.4797702852856,35.9654003949313));
#5171=CARTESIAN_POINT('Ctrl Pts',(2.09807056759484,33.7850992008905,35.9405439624699));
#5172=CARTESIAN_POINT('Ctrl Pts',(2.80252582511813,34.489417022928,35.8924857314627));
#5173=CARTESIAN_POINT('Ctrl Pts',(3.10796993106093,34.9355112883736,35.8661668197574));
#5174=CARTESIAN_POINT('Ctrl Pts',(3.51318310448797,35.913320036691,35.828744662717));
#5175=CARTESIAN_POINT('Ctrl Pts',(3.61293362241916,36.44506523213,35.8182454991865));
#5176=CARTESIAN_POINT('Ctrl Pts',(3.61293362241916,36.9438035983105,35.8182454991865));
#5177=CARTESIAN_POINT('',(3.61292728433799,57.,35.8182461384988));
#5178=CARTESIAN_POINT('',(3.61292728433799,60.,35.8182461384988));
#5179=CARTESIAN_POINT('',(35.8188421083191,57.,3.60701400320327));
#5180=CARTESIAN_POINT('Origin',(0.,57.,0.));
#5181=CARTESIAN_POINT('',(35.8188421083191,29.597913825102,3.60701400320327));
#5182=CARTESIAN_POINT('',(35.8188421083191,60.,3.60701400320327));
#5183=CARTESIAN_POINT('',(35.7385910610862,29.597913825102,-4.33048599679673));
#5184=CARTESIAN_POINT('Ctrl Pts',(35.8188421083191,29.597913825102,3.60701400320327));
#5185=CARTESIAN_POINT('Ctrl Pts',(35.8188421083191,29.0991758664567,3.60701400320327));
#5186=CARTESIAN_POINT('Ctrl Pts',(35.8293245843937,28.5674304286977,3.50726366036052));
#5187=CARTESIAN_POINT('Ctrl Pts',(35.8666793391538,27.589619985547,3.102049571335));
#5188=CARTESIAN_POINT('Ctrl Pts',(35.8929475807102,27.1435243342817,2.79660431841842));
#5189=CARTESIAN_POINT('Ctrl Pts',(35.9408892795961,26.4392057398786,2.09214623166637));
#5190=CARTESIAN_POINT('Ctrl Pts',(35.9656720315245,26.1338773873715,1.64609688970904));
#5191=CARTESIAN_POINT('Ctrl Pts',(35.9971163491985,25.7288473393432,0.668441611003487));
#5192=CARTESIAN_POINT('Ctrl Pts',(36.0031923000525,25.629163825102,0.13680939481454));
#5193=CARTESIAN_POINT('Ctrl Pts',(35.9931684759662,25.629163825102,-0.860712147213517));
#5194=CARTESIAN_POINT('Ctrl Pts',(35.9763878543241,25.7290014455195,-1.39254337628737));
#5195=CARTESIAN_POINT('Ctrl Pts',(35.925218216728,26.1342902091051,-2.37030719253055));
#5196=CARTESIAN_POINT('Ctrl Pts',(35.8914128483252,26.4397150924934,-2.81628112104011));
#5197=CARTESIAN_POINT('Ctrl Pts',(35.8292042530398,27.1439664630341,-3.52036488637474));
#5198=CARTESIAN_POINT('Ctrl Pts',(35.7967317559948,27.5898649766328,-3.8256420007237));
#5199=CARTESIAN_POINT('Ctrl Pts',(35.7511200860441,28.5674275274957,-4.23071553786938));
#5200=CARTESIAN_POINT('Ctrl Pts',(35.7385910610862,29.0991306962933,-4.33048599679673));
#5201=CARTESIAN_POINT('Ctrl Pts',(35.7385910610862,29.597913825102,-4.33048599679673));
#5202=CARTESIAN_POINT('',(35.7385910610862,57.,-4.33048599679673));
#5203=CARTESIAN_POINT('',(35.7385910610862,60.,-4.33048599679673));
#5204=CARTESIAN_POINT('',(3.61292728433799,57.,-35.8182461384988));
#5205=CARTESIAN_POINT('Origin',(0.,57.,0.));
#5206=CARTESIAN_POINT('',(3.61292728433799,60.,-35.8182461384988));
#5207=CARTESIAN_POINT('Origin',(0.,60.,0.));
#5208=CARTESIAN_POINT('',(45.7957082162897,37.5741208584476,-4.33048599679664));
#5209=CARTESIAN_POINT('',(45.7957082162897,38.1991208721035,-4.33048599679673));
#5210=CARTESIAN_POINT('',(45.7957082162897,60.,-4.33048599679673));
#5211=CARTESIAN_POINT('',(3.61292728433797,38.688289262853,-45.8578974271399));
#5212=CARTESIAN_POINT('Ctrl Pts',(3.61292728433797,38.688289262853,-45.8578974271399));
#5213=CARTESIAN_POINT('Ctrl Pts',(13.9875081498765,38.5092320746522,-45.0405331698223));
#5214=CARTESIAN_POINT('Ctrl Pts',(23.,38.3333333333333,-39.8371685740842));
#5215=CARTESIAN_POINT('Ctrl Pts',(33.6743371481683,38.125,-33.6743371481684));
#5216=CARTESIAN_POINT('Ctrl Pts',(39.8371685740842,37.9166666666667,-23.));
#5217=CARTESIAN_POINT('Ctrl Pts',(44.8515840435634,37.7471553142903,-14.3147776366026));
#5218=CARTESIAN_POINT('Ctrl Pts',(45.7957082162897,37.5741208584476,-4.33048599679664));
#5219=CARTESIAN_POINT('',(3.61292728433799,39.3132892765089,-45.8578974271399));
#5220=CARTESIAN_POINT('',(3.61292728433799,60.,-45.8578974271399));
#5221=CARTESIAN_POINT('Ctrl Pts',(3.61292728433799,39.3132892765089,-45.8578974271399));
#5222=CARTESIAN_POINT('Ctrl Pts',(13.9875081498766,39.1342320883081,-45.0405331698222));
#5223=CARTESIAN_POINT('Ctrl Pts',(23.,38.9583333469893,-39.8371685740842));
#5224=CARTESIAN_POINT('Ctrl Pts',(33.6743371481683,38.7500000136559,-33.6743371481684));
#5225=CARTESIAN_POINT('Ctrl Pts',(39.8371685740842,38.5416666803226,-23.));
#5226=CARTESIAN_POINT('Ctrl Pts',(44.8515840435634,38.3721553279462,-14.3147776366027));
#5227=CARTESIAN_POINT('Ctrl Pts',(45.7957082162897,38.1991208721035,-4.33048599679673));
#5228=CARTESIAN_POINT('Origin',(0.,60.,0.));
#5229=CARTESIAN_POINT('',(45.858362923034,38.0633913333999,3.60701400320327));
#5230=CARTESIAN_POINT('',(45.858362923034,37.438391319744,3.60701400320326));
#5231=CARTESIAN_POINT('',(45.858362923034,60.,3.60701400320327));
#5232=CARTESIAN_POINT('',(3.61292728433719,36.9367107508029,45.85789742714));
#5233=CARTESIAN_POINT('Ctrl Pts',(45.858362923034,38.0633913333999,3.60701400320327));
#5234=CARTESIAN_POINT('Ctrl Pts',(45.0420919829705,37.8842847836873,13.9848082063042));
#5235=CARTESIAN_POINT('Ctrl Pts',(39.8371685740842,37.7083333469893,23.));
#5236=CARTESIAN_POINT('Ctrl Pts',(33.6743371481684,37.5000000136559,33.6743371481683));
#5237=CARTESIAN_POINT('Ctrl Pts',(23.,37.2916666803226,39.8371685740842));
#5238=CARTESIAN_POINT('Ctrl Pts',(13.9875081498762,37.1157679390038,45.0405331698225));
#5239=CARTESIAN_POINT('Ctrl Pts',(3.61292728433719,36.9367107508029,45.85789742714));
#5240=CARTESIAN_POINT('',(3.56213286848811,36.3108341932617,45.8618709760868));
#5241=CARTESIAN_POINT('Ctrl Pts',(3.56213286848809,36.3108341932617,45.8618709760868));
#5242=CARTESIAN_POINT('Ctrl Pts',(3.59615968466946,36.5214531232455,45.8592280825949));
#5243=CARTESIAN_POINT('Ctrl Pts',(3.61256125750481,36.7319034897672,45.8579262646664));
#5244=CARTESIAN_POINT('Ctrl Pts',(3.61292728433716,36.9367107508029,45.85789742714));
#5245=CARTESIAN_POINT('Ctrl Pts',(45.858362923034,37.438391319744,3.60701400320326));
#5246=CARTESIAN_POINT('Ctrl Pts',(45.0420919829705,37.2592847700314,13.9848082063042));
#5247=CARTESIAN_POINT('Ctrl Pts',(39.8371685740842,37.0833333333333,23.));
#5248=CARTESIAN_POINT('Ctrl Pts',(33.6743371481684,36.875,33.6743371481683));
#5249=CARTESIAN_POINT('Ctrl Pts',(23.,36.6666666666667,39.8371685740842));
#5250=CARTESIAN_POINT('Ctrl Pts',(13.9643142594927,36.490315245202,45.0539241686789));
#5251=CARTESIAN_POINT('Ctrl Pts',(3.56213286848811,36.3108341932617,45.8618709760868));
#5252=CARTESIAN_POINT('Origin',(0.,60.,0.));
#5253=CARTESIAN_POINT('',(45.7957082162897,52.5741208584476,-4.33048599679672));
#5254=CARTESIAN_POINT('',(45.7957082162897,53.1991208721035,-4.33048599679673));
#5255=CARTESIAN_POINT('',(45.7957082162897,60.,-4.33048599679673));
#5256=CARTESIAN_POINT('',(3.61292728433801,53.688289262853,-45.8578974271399));
#5257=CARTESIAN_POINT('Ctrl Pts',(3.61292728433801,53.688289262853,-45.8578974271399));
#5258=CARTESIAN_POINT('Ctrl Pts',(13.9875081498766,53.5092320746522,-45.0405331698222));
#5259=CARTESIAN_POINT('Ctrl Pts',(23.,53.3333333333333,-39.8371685740842));
#5260=CARTESIAN_POINT('Ctrl Pts',(33.6743371481683,53.125,-33.6743371481684));
#5261=CARTESIAN_POINT('Ctrl Pts',(39.8371685740842,52.9166666666667,-23.));
#5262=CARTESIAN_POINT('Ctrl Pts',(44.8515840435634,52.7471553142902,-14.3147776366027));
#5263=CARTESIAN_POINT('Ctrl Pts',(45.7957082162897,52.5741208584476,-4.33048599679672));
#5264=CARTESIAN_POINT('',(3.61292728433799,54.3132892765089,-45.8578974271399));
#5265=CARTESIAN_POINT('',(3.61292728433799,60.,-45.8578974271399));
#5266=CARTESIAN_POINT('Ctrl Pts',(3.61292728433799,54.3132892765089,-45.8578974271399));
#5267=CARTESIAN_POINT('Ctrl Pts',(13.9875081498766,54.1342320883081,-45.0405331698223));
#5268=CARTESIAN_POINT('Ctrl Pts',(23.,53.9583333469893,-39.8371685740842));
#5269=CARTESIAN_POINT('Ctrl Pts',(33.6743371481683,53.7500000136559,-33.6743371481684));
#5270=CARTESIAN_POINT('Ctrl Pts',(39.8371685740842,53.5416666803226,-23.));
#5271=CARTESIAN_POINT('Ctrl Pts',(44.8515840435634,53.3721553279462,-14.3147776366027));
#5272=CARTESIAN_POINT('Ctrl Pts',(45.7957082162897,53.1991208721035,-4.33048599679673));
#5273=CARTESIAN_POINT('Origin',(0.,60.,0.));
#5274=CARTESIAN_POINT('',(45.858362923034,53.0633913333999,3.60701400320327));
#5275=CARTESIAN_POINT('',(45.858362923034,52.438391319744,3.60701400320324));
#5276=CARTESIAN_POINT('',(45.858362923034,60.,3.60701400320327));
#5277=CARTESIAN_POINT('',(3.612927284338,51.936710750803,45.8578974271399));
#5278=CARTESIAN_POINT('Ctrl Pts',(45.858362923034,53.0633913333999,3.60701400320327));
#5279=CARTESIAN_POINT('Ctrl Pts',(45.0420919829705,52.8842847836873,13.9848082063043));
#5280=CARTESIAN_POINT('Ctrl Pts',(39.8371685740842,52.7083333469893,23.));
#5281=CARTESIAN_POINT('Ctrl Pts',(33.6743371481684,52.5000000136559,33.6743371481683));
#5282=CARTESIAN_POINT('Ctrl Pts',(23.,52.2916666803226,39.8371685740842));
#5283=CARTESIAN_POINT('Ctrl Pts',(13.9875081498766,52.1157679390038,45.0405331698223));
#5284=CARTESIAN_POINT('Ctrl Pts',(3.612927284338,51.9367107508029,45.8578974271399));
#5285=CARTESIAN_POINT('',(3.61292728433799,51.311710737147,45.8578974271399));
#5286=CARTESIAN_POINT('',(3.61292728433799,60.,45.8578974271399));
#5287=CARTESIAN_POINT('Ctrl Pts',(45.858362923034,52.438391319744,3.60701400320324));
#5288=CARTESIAN_POINT('Ctrl Pts',(45.0420919829705,52.2592847700314,13.9848082063043));
#5289=CARTESIAN_POINT('Ctrl Pts',(39.8371685740842,52.0833333333333,23.));
#5290=CARTESIAN_POINT('Ctrl Pts',(33.6743371481684,51.875,33.6743371481683));
#5291=CARTESIAN_POINT('Ctrl Pts',(23.,51.6666666666667,39.8371685740842));
#5292=CARTESIAN_POINT('Ctrl Pts',(13.9875081498766,51.4907679253478,45.0405331698222));
#5293=CARTESIAN_POINT('Ctrl Pts',(3.61292728433799,51.311710737147,45.8578974271399));
#5294=CARTESIAN_POINT('Origin',(0.,60.,0.));
#5295=CARTESIAN_POINT('',(45.7957082162897,47.5741208584476,-4.33048599679672));
#5296=CARTESIAN_POINT('',(45.7957082162897,48.1991208721035,-4.33048599679673));
#5297=CARTESIAN_POINT('',(45.7957082162897,60.,-4.33048599679673));
#5298=CARTESIAN_POINT('',(3.61292728433796,48.688289262853,-45.8578974271399));
#5299=CARTESIAN_POINT('Ctrl Pts',(3.61292728433796,48.688289262853,-45.8578974271399));
#5300=CARTESIAN_POINT('Ctrl Pts',(13.9875081498765,48.5092320746522,-45.0405331698222));
#5301=CARTESIAN_POINT('Ctrl Pts',(23.,48.3333333333333,-39.8371685740842));
#5302=CARTESIAN_POINT('Ctrl Pts',(33.6743371481683,48.125,-33.6743371481684));
#5303=CARTESIAN_POINT('Ctrl Pts',(39.8371685740842,47.9166666666667,-23.));
#5304=CARTESIAN_POINT('Ctrl Pts',(44.8515840435634,47.7471553142903,-14.3147776366027));
#5305=CARTESIAN_POINT('Ctrl Pts',(45.7957082162897,47.5741208584476,-4.33048599679672));
#5306=CARTESIAN_POINT('',(3.61292728433799,49.3132892765089,-45.8578974271399));
#5307=CARTESIAN_POINT('',(3.61292728433799,60.,-45.8578974271399));
#5308=CARTESIAN_POINT('Ctrl Pts',(3.61292728433799,49.3132892765089,-45.8578974271399));
#5309=CARTESIAN_POINT('Ctrl Pts',(13.9875081498766,49.1342320883081,-45.0405331698222));
#5310=CARTESIAN_POINT('Ctrl Pts',(23.,48.9583333469893,-39.8371685740842));
#5311=CARTESIAN_POINT('Ctrl Pts',(33.6743371481683,48.7500000136559,-33.6743371481684));
#5312=CARTESIAN_POINT('Ctrl Pts',(39.8371685740842,48.5416666803226,-23.));
#5313=CARTESIAN_POINT('Ctrl Pts',(44.8515840435634,48.3721553279462,-14.3147776366027));
#5314=CARTESIAN_POINT('Ctrl Pts',(45.7957082162897,48.1991208721035,-4.33048599679673));
#5315=CARTESIAN_POINT('Origin',(0.,60.,0.));
#5316=CARTESIAN_POINT('',(45.858362923034,48.0633913333999,3.60701400320327));
#5317=CARTESIAN_POINT('',(45.858362923034,47.438391319744,3.60701400320324));
#5318=CARTESIAN_POINT('',(45.858362923034,60.,3.60701400320327));
#5319=CARTESIAN_POINT('',(3.61292728433798,46.936710750803,45.8578974271399));
#5320=CARTESIAN_POINT('Ctrl Pts',(45.858362923034,48.0633913333999,3.60701400320327));
#5321=CARTESIAN_POINT('Ctrl Pts',(45.0420919829705,47.8842847836874,13.9848082063043));
#5322=CARTESIAN_POINT('Ctrl Pts',(39.8371685740842,47.7083333469893,23.));
#5323=CARTESIAN_POINT('Ctrl Pts',(33.6743371481684,47.5000000136559,33.6743371481683));
#5324=CARTESIAN_POINT('Ctrl Pts',(23.,47.2916666803226,39.8371685740842));
#5325=CARTESIAN_POINT('Ctrl Pts',(13.9875081498766,47.1157679390037,45.0405331698222));
#5326=CARTESIAN_POINT('Ctrl Pts',(3.61292728433798,46.9367107508029,45.8578974271399));
#5327=CARTESIAN_POINT('',(3.61292728433799,46.311710737147,45.8578974271399));
#5328=CARTESIAN_POINT('',(3.61292728433799,60.,45.8578974271399));
#5329=CARTESIAN_POINT('Ctrl Pts',(45.858362923034,47.438391319744,3.60701400320324));
#5330=CARTESIAN_POINT('Ctrl Pts',(45.0420919829705,47.2592847700314,13.9848082063043));
#5331=CARTESIAN_POINT('Ctrl Pts',(39.8371685740842,47.0833333333333,23.));
#5332=CARTESIAN_POINT('Ctrl Pts',(33.6743371481684,46.875,33.6743371481683));
#5333=CARTESIAN_POINT('Ctrl Pts',(23.,46.6666666666667,39.8371685740842));
#5334=CARTESIAN_POINT('Ctrl Pts',(13.9875081498766,46.4907679253478,45.0405331698222));
#5335=CARTESIAN_POINT('Ctrl Pts',(3.61292728433799,46.311710737147,45.8578974271399));
#5336=CARTESIAN_POINT('Origin',(0.,60.,0.));
#5337=CARTESIAN_POINT('',(45.7957082162897,42.5741208584476,-4.3304859967968));
#5338=CARTESIAN_POINT('',(45.7957082162897,43.1991208721035,-4.33048599679673));
#5339=CARTESIAN_POINT('',(45.7957082162897,60.,-4.33048599679673));
#5340=CARTESIAN_POINT('',(3.61292728433795,43.688289262853,-45.8578974271399));
#5341=CARTESIAN_POINT('Ctrl Pts',(3.61292728433794,43.688289262853,-45.8578974271399));
#5342=CARTESIAN_POINT('Ctrl Pts',(13.9875081498765,43.5092320746522,-45.0405331698223));
#5343=CARTESIAN_POINT('Ctrl Pts',(23.,43.3333333333333,-39.8371685740842));
#5344=CARTESIAN_POINT('Ctrl Pts',(33.6743371481683,43.125,-33.6743371481684));
#5345=CARTESIAN_POINT('Ctrl Pts',(39.8371685740842,42.9166666666667,-23.));
#5346=CARTESIAN_POINT('Ctrl Pts',(44.8515840435634,42.7471553142903,-14.3147776366027));
#5347=CARTESIAN_POINT('Ctrl Pts',(45.7957082162897,42.5741208584476,-4.3304859967968));
#5348=CARTESIAN_POINT('',(3.61292728433799,44.3132892765089,-45.8578974271399));
#5349=CARTESIAN_POINT('',(3.61292728433799,60.,-45.8578974271399));
#5350=CARTESIAN_POINT('Ctrl Pts',(3.61292728433799,44.3132892765089,-45.8578974271399));
#5351=CARTESIAN_POINT('Ctrl Pts',(13.9875081498766,44.1342320883081,-45.0405331698222));
#5352=CARTESIAN_POINT('Ctrl Pts',(23.,43.9583333469893,-39.8371685740842));
#5353=CARTESIAN_POINT('Ctrl Pts',(33.6743371481683,43.7500000136559,-33.6743371481684));
#5354=CARTESIAN_POINT('Ctrl Pts',(39.8371685740842,43.5416666803226,-23.));
#5355=CARTESIAN_POINT('Ctrl Pts',(44.8515840435634,43.3721553279462,-14.3147776366027));
#5356=CARTESIAN_POINT('Ctrl Pts',(45.7957082162897,43.1991208721035,-4.33048599679673));
#5357=CARTESIAN_POINT('Origin',(0.,60.,0.));
#5358=CARTESIAN_POINT('',(45.858362923034,43.0633913333999,3.60701400320327));
#5359=CARTESIAN_POINT('',(45.858362923034,42.438391319744,3.60701400320326));
#5360=CARTESIAN_POINT('',(45.858362923034,60.,3.60701400320327));
#5361=CARTESIAN_POINT('',(3.61292728433799,41.936710750803,45.8578974271399));
#5362=CARTESIAN_POINT('Ctrl Pts',(45.858362923034,43.0633913333999,3.60701400320327));
#5363=CARTESIAN_POINT('Ctrl Pts',(45.0420919829705,42.8842847836874,13.9848082063043));
#5364=CARTESIAN_POINT('Ctrl Pts',(39.8371685740842,42.7083333469893,23.));
#5365=CARTESIAN_POINT('Ctrl Pts',(33.6743371481684,42.5000000136559,33.6743371481683));
#5366=CARTESIAN_POINT('Ctrl Pts',(23.,42.2916666803226,39.8371685740842));
#5367=CARTESIAN_POINT('Ctrl Pts',(13.9875081498766,42.1157679390038,45.0405331698222));
#5368=CARTESIAN_POINT('Ctrl Pts',(3.61292728433799,41.936710750803,45.8578974271399));
#5369=CARTESIAN_POINT('',(3.61292728433799,41.311710737147,45.8578974271399));
#5370=CARTESIAN_POINT('',(3.61292728433799,60.,45.8578974271399));
#5371=CARTESIAN_POINT('Ctrl Pts',(45.858362923034,42.438391319744,3.60701400320326));
#5372=CARTESIAN_POINT('Ctrl Pts',(45.0420919829705,42.2592847700314,13.9848082063042));
#5373=CARTESIAN_POINT('Ctrl Pts',(39.8371685740842,42.0833333333333,23.));
#5374=CARTESIAN_POINT('Ctrl Pts',(33.6743371481684,41.875,33.6743371481683));
#5375=CARTESIAN_POINT('Ctrl Pts',(23.,41.6666666666667,39.8371685740842));
#5376=CARTESIAN_POINT('Ctrl Pts',(13.9875081498766,41.4907679253478,45.0405331698223));
#5377=CARTESIAN_POINT('Ctrl Pts',(3.61292728433799,41.311710737147,45.8578974271399));
#5378=CARTESIAN_POINT('Origin',(0.,60.,0.));
#5379=CARTESIAN_POINT('',(-45.7957082162897,55.5508791552084,-4.33048599679673));
#5380=CARTESIAN_POINT('',(-45.7957082162897,54.9258791415524,-4.33048599679671));
#5381=CARTESIAN_POINT('',(-45.7957082162897,60.,-4.33048599679673));
#5382=CARTESIAN_POINT('',(-4.32456003949879,54.4490181730497,-45.7962681936506));
#5383=CARTESIAN_POINT('Ctrl Pts',(-45.7957082162897,55.5508791552084,-4.33048599679673));
#5384=CARTESIAN_POINT('Ctrl Pts',(-44.8515840435634,55.3778446993657,-14.3147776366027));
#5385=CARTESIAN_POINT('Ctrl Pts',(-39.8371685740842,55.2083333469893,-23.));
#5386=CARTESIAN_POINT('Ctrl Pts',(-33.6743371481684,55.0000000136559,-33.6743371481684));
#5387=CARTESIAN_POINT('Ctrl Pts',(-23.,54.7916666803226,-39.8371685740842));
#5388=CARTESIAN_POINT('Ctrl Pts',(-14.3120776418265,54.6221026315676,-44.8531428862742));
#5389=CARTESIAN_POINT('Ctrl Pts',(-4.32456003949879,54.4490181730497,-45.7962681936506));
#5390=CARTESIAN_POINT('',(-4.32456003949879,53.8240181593938,-45.7962681936506));
#5391=CARTESIAN_POINT('',(-4.32456003949879,60.,-45.7962681936506));
#5392=CARTESIAN_POINT('Ctrl Pts',(-45.7957082162897,54.9258791415524,-4.33048599679671));
#5393=CARTESIAN_POINT('Ctrl Pts',(-44.8515840435634,54.7528446857097,-14.3147776366027));
#5394=CARTESIAN_POINT('Ctrl Pts',(-39.8371685740842,54.5833333333333,-23.));
#5395=CARTESIAN_POINT('Ctrl Pts',(-33.6743371481684,54.375,-33.6743371481684));
#5396=CARTESIAN_POINT('Ctrl Pts',(-23.,54.1666666666667,-39.8371685740842));
#5397=CARTESIAN_POINT('Ctrl Pts',(-14.3120776418265,53.9971026179117,-44.8531428862742));
#5398=CARTESIAN_POINT('Ctrl Pts',(-4.32456003949879,53.8240181593938,-45.7962681936506));
#5399=CARTESIAN_POINT('Origin',(0.,60.,0.));
#5400=CARTESIAN_POINT('',(-45.858362923034,55.061608680256,3.60701400320327));
#5401=CARTESIAN_POINT('',(-45.858362923034,57.,3.60701400320327));
#5402=CARTESIAN_POINT('',(-45.858362923034,60.,3.60701400320327));
#5403=CARTESIAN_POINT('',(-4.32456003949879,56.1759818406063,45.7962681936506));
#5404=CARTESIAN_POINT('Ctrl Pts',(-4.32456003949879,56.1759818406063,45.7962681936506));
#5405=CARTESIAN_POINT('Ctrl Pts',(-14.3120776418264,56.0028973820884,44.8531428862743));
#5406=CARTESIAN_POINT('Ctrl Pts',(-23.,55.8333333333333,39.8371685740842));
#5407=CARTESIAN_POINT('Ctrl Pts',(-33.6743371481683,55.625,33.6743371481684));
#5408=CARTESIAN_POINT('Ctrl Pts',(-39.8371685740842,55.4166666666667,23.));
#5409=CARTESIAN_POINT('Ctrl Pts',(-45.0420919829705,55.2407152299686,13.9848082063043));
#5410=CARTESIAN_POINT('Ctrl Pts',(-45.858362923034,55.061608680256,3.60701400320327));
#5411=CARTESIAN_POINT('',(-4.32456003949879,57.,45.7962681936506));
#5412=CARTESIAN_POINT('',(-4.32456003949879,60.,45.7962681936506));
#5413=CARTESIAN_POINT('Origin',(0.,57.,0.));
#5414=CARTESIAN_POINT('Origin',(0.,60.,0.));
#5415=CARTESIAN_POINT('',(-45.7957082162897,50.5508791552084,-4.33048599679673));
#5416=CARTESIAN_POINT('',(-45.7957082162897,49.9258791415524,-4.33048599679671));
#5417=CARTESIAN_POINT('',(-45.7957082162897,60.,-4.33048599679673));
#5418=CARTESIAN_POINT('',(-4.32456003949879,49.4490181730497,-45.7962681936506));
#5419=CARTESIAN_POINT('Ctrl Pts',(-45.7957082162897,50.5508791552084,-4.33048599679673));
#5420=CARTESIAN_POINT('Ctrl Pts',(-44.8515840435634,50.3778446993657,-14.3147776366027));
#5421=CARTESIAN_POINT('Ctrl Pts',(-39.8371685740842,50.2083333469893,-23.));
#5422=CARTESIAN_POINT('Ctrl Pts',(-33.6743371481684,50.0000000136559,-33.6743371481684));
#5423=CARTESIAN_POINT('Ctrl Pts',(-23.,49.7916666803226,-39.8371685740842));
#5424=CARTESIAN_POINT('Ctrl Pts',(-14.3120776418265,49.6221026315676,-44.8531428862742));
#5425=CARTESIAN_POINT('Ctrl Pts',(-4.32456003949879,49.4490181730497,-45.7962681936506));
#5426=CARTESIAN_POINT('',(-4.32456003949879,48.8240181593938,-45.7962681936506));
#5427=CARTESIAN_POINT('',(-4.32456003949879,60.,-45.7962681936506));
#5428=CARTESIAN_POINT('Ctrl Pts',(-45.7957082162897,49.9258791415524,-4.33048599679671));
#5429=CARTESIAN_POINT('Ctrl Pts',(-44.8515840435634,49.7528446857098,-14.3147776366027));
#5430=CARTESIAN_POINT('Ctrl Pts',(-39.8371685740842,49.5833333333333,-23.));
#5431=CARTESIAN_POINT('Ctrl Pts',(-33.6743371481684,49.375,-33.6743371481684));
#5432=CARTESIAN_POINT('Ctrl Pts',(-23.,49.1666666666667,-39.8371685740842));
#5433=CARTESIAN_POINT('Ctrl Pts',(-14.3120776418265,48.9971026179117,-44.8531428862742));
#5434=CARTESIAN_POINT('Ctrl Pts',(-4.32456003949879,48.8240181593938,-45.7962681936506));
#5435=CARTESIAN_POINT('Origin',(0.,60.,0.));
#5436=CARTESIAN_POINT('',(-45.858362923034,50.061608680256,3.60701400320326));
#5437=CARTESIAN_POINT('',(-45.858362923034,50.686608693912,3.60701400320327));
#5438=CARTESIAN_POINT('',(-45.858362923034,60.,3.60701400320327));
#5439=CARTESIAN_POINT('',(-4.32456003949879,51.1759818406062,45.7962681936506));
#5440=CARTESIAN_POINT('Ctrl Pts',(-4.32456003949879,51.1759818406063,45.7962681936506));
#5441=CARTESIAN_POINT('Ctrl Pts',(-14.3120776418264,51.0028973820884,44.8531428862743));
#5442=CARTESIAN_POINT('Ctrl Pts',(-23.,50.8333333333333,39.8371685740842));
#5443=CARTESIAN_POINT('Ctrl Pts',(-33.6743371481683,50.625,33.6743371481684));
#5444=CARTESIAN_POINT('Ctrl Pts',(-39.8371685740842,50.4166666666667,23.));
#5445=CARTESIAN_POINT('Ctrl Pts',(-45.0420919829705,50.2407152299686,13.9848082063043));
#5446=CARTESIAN_POINT('Ctrl Pts',(-45.858362923034,50.061608680256,3.60701400320326));
#5447=CARTESIAN_POINT('',(-4.32456003949877,51.8009818542622,45.7962681936506));
#5448=CARTESIAN_POINT('',(-4.32456003949879,60.,45.7962681936506));
#5449=CARTESIAN_POINT('Ctrl Pts',(-4.32456003949877,51.8009818542622,45.7962681936506));
#5450=CARTESIAN_POINT('Ctrl Pts',(-14.3120776418264,51.6278973957443,44.8531428862743));
#5451=CARTESIAN_POINT('Ctrl Pts',(-23.,51.4583333469893,39.8371685740842));
#5452=CARTESIAN_POINT('Ctrl Pts',(-33.6743371481683,51.2500000136559,33.6743371481684));
#5453=CARTESIAN_POINT('Ctrl Pts',(-39.8371685740842,51.0416666803226,23.));
#5454=CARTESIAN_POINT('Ctrl Pts',(-45.0420919829705,50.8657152436245,13.9848082063043));
#5455=CARTESIAN_POINT('Ctrl Pts',(-45.858362923034,50.686608693912,3.60701400320327));
#5456=CARTESIAN_POINT('Origin',(0.,60.,0.));
#5457=CARTESIAN_POINT('',(-45.7957082162897,45.5508791552084,-4.33048599679673));
#5458=CARTESIAN_POINT('',(-45.7957082162897,44.9258791415524,-4.33048599679682));
#5459=CARTESIAN_POINT('',(-45.7957082162897,60.,-4.33048599679673));
#5460=CARTESIAN_POINT('',(-4.32456003949874,44.4490181730497,-45.7962681936506));
#5461=CARTESIAN_POINT('Ctrl Pts',(-45.7957082162897,45.5508791552084,-4.33048599679673));
#5462=CARTESIAN_POINT('Ctrl Pts',(-44.8515840435634,45.3778446993657,-14.3147776366027));
#5463=CARTESIAN_POINT('Ctrl Pts',(-39.8371685740842,45.2083333469893,-23.));
#5464=CARTESIAN_POINT('Ctrl Pts',(-33.6743371481684,45.0000000136559,-33.6743371481684));
#5465=CARTESIAN_POINT('Ctrl Pts',(-23.,44.7916666803226,-39.8371685740842));
#5466=CARTESIAN_POINT('Ctrl Pts',(-14.3120776418264,44.6221026315676,-44.8531428862743));
#5467=CARTESIAN_POINT('Ctrl Pts',(-4.32456003949874,44.4490181730497,-45.7962681936506));
#5468=CARTESIAN_POINT('',(-4.32456003949879,43.8240181593938,-45.7962681936506));
#5469=CARTESIAN_POINT('',(-4.32456003949879,60.,-45.7962681936506));
#5470=CARTESIAN_POINT('Ctrl Pts',(-45.7957082162897,44.9258791415524,-4.33048599679682));
#5471=CARTESIAN_POINT('Ctrl Pts',(-44.8515840435634,44.7528446857097,-14.3147776366027));
#5472=CARTESIAN_POINT('Ctrl Pts',(-39.8371685740842,44.5833333333333,-23.));
#5473=CARTESIAN_POINT('Ctrl Pts',(-33.6743371481684,44.375,-33.6743371481684));
#5474=CARTESIAN_POINT('Ctrl Pts',(-23.,44.1666666666667,-39.8371685740842));
#5475=CARTESIAN_POINT('Ctrl Pts',(-14.3120776418264,43.9971026179117,-44.8531428862742));
#5476=CARTESIAN_POINT('Ctrl Pts',(-4.32456003949879,43.8240181593938,-45.7962681936506));
#5477=CARTESIAN_POINT('Origin',(0.,60.,0.));
#5478=CARTESIAN_POINT('',(-45.858362923034,45.061608680256,3.60701400320326));
#5479=CARTESIAN_POINT('',(-45.858362923034,45.686608693912,3.60701400320327));
#5480=CARTESIAN_POINT('',(-45.858362923034,60.,3.60701400320327));
#5481=CARTESIAN_POINT('',(-4.32456003949879,46.1759818406062,45.7962681936506));
#5482=CARTESIAN_POINT('Ctrl Pts',(-4.32456003949879,46.1759818406063,45.7962681936506));
#5483=CARTESIAN_POINT('Ctrl Pts',(-14.3120776418264,46.0028973820884,44.8531428862743));
#5484=CARTESIAN_POINT('Ctrl Pts',(-23.,45.8333333333333,39.8371685740842));
#5485=CARTESIAN_POINT('Ctrl Pts',(-33.6743371481683,45.625,33.6743371481684));
#5486=CARTESIAN_POINT('Ctrl Pts',(-39.8371685740842,45.4166666666667,23.));
#5487=CARTESIAN_POINT('Ctrl Pts',(-45.0420919829705,45.2407152299686,13.9848082063043));
#5488=CARTESIAN_POINT('Ctrl Pts',(-45.858362923034,45.0616086802561,3.60701400320326));
#5489=CARTESIAN_POINT('',(-4.32456003949882,46.8009818542622,45.7962681936506));
#5490=CARTESIAN_POINT('',(-4.32456003949879,60.,45.7962681936506));
#5491=CARTESIAN_POINT('Ctrl Pts',(-4.32456003949882,46.8009818542622,45.7962681936506));
#5492=CARTESIAN_POINT('Ctrl Pts',(-14.3120776418264,46.6278973957443,44.8531428862743));
#5493=CARTESIAN_POINT('Ctrl Pts',(-23.,46.4583333469893,39.8371685740842));
#5494=CARTESIAN_POINT('Ctrl Pts',(-33.6743371481683,46.2500000136559,33.6743371481684));
#5495=CARTESIAN_POINT('Ctrl Pts',(-39.8371685740842,46.0416666803226,23.));
#5496=CARTESIAN_POINT('Ctrl Pts',(-45.0420919829705,45.8657152436245,13.9848082063043));
#5497=CARTESIAN_POINT('Ctrl Pts',(-45.858362923034,45.686608693912,3.60701400320327));
#5498=CARTESIAN_POINT('Origin',(0.,60.,0.));
#5499=CARTESIAN_POINT('',(-45.7957082162897,40.5508791552084,-4.33048599679673));
#5500=CARTESIAN_POINT('',(-45.7957082162897,39.9258791415524,-4.33048599679679));
#5501=CARTESIAN_POINT('',(-45.7957082162897,60.,-4.33048599679673));
#5502=CARTESIAN_POINT('',(-4.32456003949876,39.4490181730497,-45.7962681936506));
#5503=CARTESIAN_POINT('Ctrl Pts',(-45.7957082162897,40.5508791552084,-4.33048599679673));
#5504=CARTESIAN_POINT('Ctrl Pts',(-44.8515840435634,40.3778446993657,-14.3147776366027));
#5505=CARTESIAN_POINT('Ctrl Pts',(-39.8371685740842,40.2083333469893,-23.));
#5506=CARTESIAN_POINT('Ctrl Pts',(-33.6743371481684,40.0000000136559,-33.6743371481684));
#5507=CARTESIAN_POINT('Ctrl Pts',(-23.,39.7916666803226,-39.8371685740842));
#5508=CARTESIAN_POINT('Ctrl Pts',(-14.3120776418264,39.6221026315676,-44.8531428862742));
#5509=CARTESIAN_POINT('Ctrl Pts',(-4.32456003949876,39.4490181730497,-45.7962681936506));
#5510=CARTESIAN_POINT('',(-4.32456003949879,38.8240181593937,-45.7962681936506));
#5511=CARTESIAN_POINT('',(-4.32456003949879,60.,-45.7962681936506));
#5512=CARTESIAN_POINT('Ctrl Pts',(-45.7957082162897,39.9258791415524,-4.33048599679679));
#5513=CARTESIAN_POINT('Ctrl Pts',(-44.8515840435634,39.7528446857097,-14.3147776366027));
#5514=CARTESIAN_POINT('Ctrl Pts',(-39.8371685740842,39.5833333333333,-23.));
#5515=CARTESIAN_POINT('Ctrl Pts',(-33.6743371481684,39.375,-33.6743371481684));
#5516=CARTESIAN_POINT('Ctrl Pts',(-23.,39.1666666666667,-39.8371685740842));
#5517=CARTESIAN_POINT('Ctrl Pts',(-14.3120776418264,38.9971026179116,-44.8531428862743));
#5518=CARTESIAN_POINT('Ctrl Pts',(-4.32456003949879,38.8240181593937,-45.7962681936506));
#5519=CARTESIAN_POINT('Origin',(0.,60.,0.));
#5520=CARTESIAN_POINT('',(-45.858362923034,40.061608680256,3.60701400320328));
#5521=CARTESIAN_POINT('',(-45.858362923034,40.686608693912,3.60701400320327));
#5522=CARTESIAN_POINT('',(-45.858362923034,60.,3.60701400320327));
#5523=CARTESIAN_POINT('',(-4.32456003949879,41.1759818406062,45.7962681936506));
#5524=CARTESIAN_POINT('Ctrl Pts',(-4.32456003949879,41.1759818406063,45.7962681936506));
#5525=CARTESIAN_POINT('Ctrl Pts',(-14.3120776418264,41.0028973820884,44.8531428862743));
#5526=CARTESIAN_POINT('Ctrl Pts',(-23.,40.8333333333333,39.8371685740842));
#5527=CARTESIAN_POINT('Ctrl Pts',(-33.6743371481683,40.625,33.6743371481684));
#5528=CARTESIAN_POINT('Ctrl Pts',(-39.8371685740842,40.4166666666667,23.));
#5529=CARTESIAN_POINT('Ctrl Pts',(-45.0420919829705,40.2407152299686,13.9848082063043));
#5530=CARTESIAN_POINT('Ctrl Pts',(-45.858362923034,40.061608680256,3.60701400320328));
#5531=CARTESIAN_POINT('',(-4.32456003949882,41.8009818542622,45.7962681936506));
#5532=CARTESIAN_POINT('',(-4.32456003949879,60.,45.7962681936506));
#5533=CARTESIAN_POINT('Ctrl Pts',(-4.32456003949882,41.8009818542622,45.7962681936506));
#5534=CARTESIAN_POINT('Ctrl Pts',(-14.3120776418264,41.6278973957443,44.8531428862743));
#5535=CARTESIAN_POINT('Ctrl Pts',(-23.,41.4583333469893,39.8371685740842));
#5536=CARTESIAN_POINT('Ctrl Pts',(-33.6743371481683,41.2500000136559,33.6743371481684));
#5537=CARTESIAN_POINT('Ctrl Pts',(-39.8371685740842,41.0416666803226,23.));
#5538=CARTESIAN_POINT('Ctrl Pts',(-45.0420919829705,40.8657152436245,13.9848082063043));
#5539=CARTESIAN_POINT('Ctrl Pts',(-45.858362923034,40.686608693912,3.60701400320327));
#5540=CARTESIAN_POINT('Ctrl Pts',(-46.,55.6250000136559,0.));
#5541=CARTESIAN_POINT('Ctrl Pts',(-46.,55.4166666803226,-12.3256628518316));
#5542=CARTESIAN_POINT('Ctrl Pts',(-39.8371685740842,55.2083333469893,-23.));
#5543=CARTESIAN_POINT('Ctrl Pts',(-33.6743371481684,55.0000000136559,-33.6743371481684));
#5544=CARTESIAN_POINT('Ctrl Pts',(-23.,54.7916666803226,-39.8371685740842));
#5545=CARTESIAN_POINT('Ctrl Pts',(-12.3256628518317,54.5833333469893,-46.));
#5546=CARTESIAN_POINT('Ctrl Pts',(-2.81668763803891E-15,54.3750000136559,
-46.));
#5547=CARTESIAN_POINT('Ctrl Pts',(12.3256628518316,54.1666666803226,-46.));
#5548=CARTESIAN_POINT('Ctrl Pts',(23.,53.9583333469893,-39.8371685740842));
#5549=CARTESIAN_POINT('Ctrl Pts',(33.6743371481683,53.7500000136559,-33.6743371481684));
#5550=CARTESIAN_POINT('Ctrl Pts',(39.8371685740842,53.5416666803226,-23.));
#5551=CARTESIAN_POINT('Ctrl Pts',(46.,53.3333333469893,-12.3256628518317));
#5552=CARTESIAN_POINT('Ctrl Pts',(46.,53.1250000136559,-5.63337527607782E-15));
#5553=CARTESIAN_POINT('Ctrl Pts',(46.,52.9166666803226,12.3256628518316));
#5554=CARTESIAN_POINT('Ctrl Pts',(39.8371685740842,52.7083333469893,23.));
#5555=CARTESIAN_POINT('Ctrl Pts',(33.6743371481684,52.5000000136559,33.6743371481683));
#5556=CARTESIAN_POINT('Ctrl Pts',(23.,52.2916666803226,39.8371685740842));
#5557=CARTESIAN_POINT('Ctrl Pts',(12.3256628518317,52.0833333469893,46.));
#5558=CARTESIAN_POINT('Ctrl Pts',(8.45006291411674E-15,51.8750000136559,
46.));
#5559=CARTESIAN_POINT('Ctrl Pts',(-12.3256628518316,51.6666666803226,46.));
#5560=CARTESIAN_POINT('Ctrl Pts',(-23.,51.4583333469893,39.8371685740842));
#5561=CARTESIAN_POINT('Ctrl Pts',(-33.6743371481683,51.2500000136559,33.6743371481684));
#5562=CARTESIAN_POINT('Ctrl Pts',(-39.8371685740842,51.0416666803226,23.));
#5563=CARTESIAN_POINT('Ctrl Pts',(-46.,50.8333333469893,12.3256628518317));
#5564=CARTESIAN_POINT('Ctrl Pts',(-46.,50.6250000136559,0.));
#5565=CARTESIAN_POINT('Ctrl Pts',(-46.,50.4166666803226,-12.3256628518316));
#5566=CARTESIAN_POINT('Ctrl Pts',(-39.8371685740842,50.2083333469893,-23.));
#5567=CARTESIAN_POINT('Ctrl Pts',(-33.6743371481684,50.0000000136559,-33.6743371481684));
#5568=CARTESIAN_POINT('Ctrl Pts',(-23.,49.7916666803226,-39.8371685740842));
#5569=CARTESIAN_POINT('Ctrl Pts',(-12.3256628518317,49.5833333469893,-46.));
#5570=CARTESIAN_POINT('Ctrl Pts',(-2.81668763803891E-15,49.3750000136559,
-46.));
#5571=CARTESIAN_POINT('Ctrl Pts',(12.3256628518316,49.1666666803226,-46.));
#5572=CARTESIAN_POINT('Ctrl Pts',(23.,48.9583333469893,-39.8371685740842));
#5573=CARTESIAN_POINT('Ctrl Pts',(33.6743371481683,48.7500000136559,-33.6743371481684));
#5574=CARTESIAN_POINT('Ctrl Pts',(39.8371685740842,48.5416666803226,-23.));
#5575=CARTESIAN_POINT('Ctrl Pts',(46.,48.3333333469893,-12.3256628518317));
#5576=CARTESIAN_POINT('Ctrl Pts',(46.,48.1250000136559,-5.63337527607782E-15));
#5577=CARTESIAN_POINT('Ctrl Pts',(46.,47.9166666803226,12.3256628518316));
#5578=CARTESIAN_POINT('Ctrl Pts',(39.8371685740842,47.7083333469893,23.));
#5579=CARTESIAN_POINT('Ctrl Pts',(33.6743371481684,47.5000000136559,33.6743371481683));
#5580=CARTESIAN_POINT('Ctrl Pts',(23.,47.2916666803226,39.8371685740842));
#5581=CARTESIAN_POINT('Ctrl Pts',(12.3256628518317,47.0833333469893,46.));
#5582=CARTESIAN_POINT('Ctrl Pts',(8.45006291411674E-15,46.8750000136559,
46.));
#5583=CARTESIAN_POINT('Ctrl Pts',(-12.3256628518316,46.6666666803226,46.));
#5584=CARTESIAN_POINT('Ctrl Pts',(-23.,46.4583333469893,39.8371685740842));
#5585=CARTESIAN_POINT('Ctrl Pts',(-33.6743371481683,46.2500000136559,33.6743371481684));
#5586=CARTESIAN_POINT('Ctrl Pts',(-39.8371685740842,46.0416666803226,23.));
#5587=CARTESIAN_POINT('Ctrl Pts',(-46.,45.8333333469892,12.3256628518317));
#5588=CARTESIAN_POINT('Ctrl Pts',(-46.,45.6250000136559,0.));
#5589=CARTESIAN_POINT('Ctrl Pts',(-46.,45.4166666803226,-12.3256628518316));
#5590=CARTESIAN_POINT('Ctrl Pts',(-39.8371685740842,45.2083333469893,-23.));
#5591=CARTESIAN_POINT('Ctrl Pts',(-33.6743371481684,45.0000000136559,-33.6743371481684));
#5592=CARTESIAN_POINT('Ctrl Pts',(-23.,44.7916666803226,-39.8371685740842));
#5593=CARTESIAN_POINT('Ctrl Pts',(-12.3256628518317,44.5833333469893,-46.));
#5594=CARTESIAN_POINT('Ctrl Pts',(-2.81668763803891E-15,44.3750000136559,
-46.));
#5595=CARTESIAN_POINT('Ctrl Pts',(12.3256628518316,44.1666666803226,-46.));
#5596=CARTESIAN_POINT('Ctrl Pts',(23.,43.9583333469893,-39.8371685740842));
#5597=CARTESIAN_POINT('Ctrl Pts',(33.6743371481683,43.7500000136559,-33.6743371481684));
#5598=CARTESIAN_POINT('Ctrl Pts',(39.8371685740842,43.5416666803226,-23.));
#5599=CARTESIAN_POINT('Ctrl Pts',(46.,43.3333333469893,-12.3256628518317));
#5600=CARTESIAN_POINT('Ctrl Pts',(46.,43.1250000136559,-5.63337527607782E-15));
#5601=CARTESIAN_POINT('Ctrl Pts',(46.,42.9166666803226,12.3256628518316));
#5602=CARTESIAN_POINT('Ctrl Pts',(39.8371685740842,42.7083333469893,23.));
#5603=CARTESIAN_POINT('Ctrl Pts',(33.6743371481684,42.5000000136559,33.6743371481683));
#5604=CARTESIAN_POINT('Ctrl Pts',(23.,42.2916666803226,39.8371685740842));
#5605=CARTESIAN_POINT('Ctrl Pts',(12.3256628518317,42.0833333469893,46.));
#5606=CARTESIAN_POINT('Ctrl Pts',(8.45006291411674E-15,41.8750000136559,
46.));
#5607=CARTESIAN_POINT('Ctrl Pts',(-12.3256628518316,41.6666666803226,46.));
#5608=CARTESIAN_POINT('Ctrl Pts',(-23.,41.4583333469893,39.8371685740842));
#5609=CARTESIAN_POINT('Ctrl Pts',(-33.6743371481683,41.2500000136559,33.6743371481684));
#5610=CARTESIAN_POINT('Ctrl Pts',(-39.8371685740842,41.0416666803226,23.));
#5611=CARTESIAN_POINT('Ctrl Pts',(-46.,40.8333333469893,12.3256628518317));
#5612=CARTESIAN_POINT('Ctrl Pts',(-46.,40.6250000136559,0.));
#5613=CARTESIAN_POINT('Ctrl Pts',(-46.,40.4166666803226,-12.3256628518316));
#5614=CARTESIAN_POINT('Ctrl Pts',(-39.8371685740842,40.2083333469893,-23.));
#5615=CARTESIAN_POINT('Ctrl Pts',(-33.6743371481684,40.0000000136559,-33.6743371481684));
#5616=CARTESIAN_POINT('Ctrl Pts',(-23.,39.7916666803226,-39.8371685740842));
#5617=CARTESIAN_POINT('Ctrl Pts',(-12.3256628518317,39.5833333469893,-46.));
#5618=CARTESIAN_POINT('Ctrl Pts',(-2.81668763803891E-15,39.3750000136559,
-46.));
#5619=CARTESIAN_POINT('Ctrl Pts',(12.3256628518316,39.1666666803226,-46.));
#5620=CARTESIAN_POINT('Ctrl Pts',(23.,38.9583333469893,-39.8371685740842));
#5621=CARTESIAN_POINT('Ctrl Pts',(33.6743371481683,38.7500000136559,-33.6743371481684));
#5622=CARTESIAN_POINT('Ctrl Pts',(39.8371685740842,38.5416666803226,-23.));
#5623=CARTESIAN_POINT('Ctrl Pts',(46.,38.3333333469893,-12.3256628518317));
#5624=CARTESIAN_POINT('Ctrl Pts',(46.,38.1250000136559,-5.63337527607782E-15));
#5625=CARTESIAN_POINT('Ctrl Pts',(46.,37.9166666803226,12.3256628518316));
#5626=CARTESIAN_POINT('Ctrl Pts',(39.8371685740842,37.7083333469893,23.));
#5627=CARTESIAN_POINT('Ctrl Pts',(33.6743371481684,37.5000000136559,33.6743371481683));
#5628=CARTESIAN_POINT('Ctrl Pts',(23.,37.2916666803226,39.8371685740842));
#5629=CARTESIAN_POINT('Ctrl Pts',(12.3256628518317,37.0833333469893,46.));
#5630=CARTESIAN_POINT('Ctrl Pts',(8.45006291411674E-15,36.8750000136559,
46.));
#5631=CARTESIAN_POINT('Ctrl Pts',(-12.3256628518316,36.6666666803226,46.));
#5632=CARTESIAN_POINT('Ctrl Pts',(-23.,36.4583333469893,39.8371685740842));
#5633=CARTESIAN_POINT('Ctrl Pts',(-33.6743371481683,36.2500000136559,33.6743371481684));
#5634=CARTESIAN_POINT('Ctrl Pts',(-39.8371685740842,36.0416666803226,23.));
#5635=CARTESIAN_POINT('Ctrl Pts',(-46.,35.8333333469893,12.3256628518317));
#5636=CARTESIAN_POINT('Ctrl Pts',(-46.,35.6250000136559,0.));
#5637=CARTESIAN_POINT('Ctrl Pts',(-46.,35.4166666803226,-12.3256628518316));
#5638=CARTESIAN_POINT('Ctrl Pts',(-39.8371685740842,35.2083333469893,-23.));
#5639=CARTESIAN_POINT('Ctrl Pts',(-33.6743371481684,35.0000000136559,-33.6743371481684));
#5640=CARTESIAN_POINT('Ctrl Pts',(-23.,34.7916666803226,-39.8371685740842));
#5641=CARTESIAN_POINT('Ctrl Pts',(-12.3256628518317,34.5833333469893,-46.));
#5642=CARTESIAN_POINT('Ctrl Pts',(-2.81668763803891E-15,34.3750000136559,
-46.));
#5643=CARTESIAN_POINT('Ctrl Pts',(12.3256628518316,34.1666666803226,-46.));
#5644=CARTESIAN_POINT('Ctrl Pts',(23.,33.9583333469893,-39.8371685740842));
#5645=CARTESIAN_POINT('Ctrl Pts',(33.6743371481683,33.7500000136559,-33.6743371481684));
#5646=CARTESIAN_POINT('Ctrl Pts',(39.8371685740842,33.5416666803226,-23.));
#5647=CARTESIAN_POINT('Ctrl Pts',(46.,33.3333333469893,-12.3256628518317));
#5648=CARTESIAN_POINT('Ctrl Pts',(46.,33.1250000136559,-5.63337527607782E-15));
#5649=CARTESIAN_POINT('Ctrl Pts',(46.,32.9166666803226,12.3256628518316));
#5650=CARTESIAN_POINT('Ctrl Pts',(39.8371685740842,32.7083333469893,23.));
#5651=CARTESIAN_POINT('Ctrl Pts',(33.6743371481684,32.5000000136559,33.6743371481683));
#5652=CARTESIAN_POINT('Ctrl Pts',(23.,32.2916666803226,39.8371685740842));
#5653=CARTESIAN_POINT('Ctrl Pts',(12.3256628518317,32.0833333469893,46.));
#5654=CARTESIAN_POINT('Ctrl Pts',(8.45006291411674E-15,31.8750000136559,
46.));
#5655=CARTESIAN_POINT('Ctrl Pts',(-12.3256628518316,31.6666666803226,46.));
#5656=CARTESIAN_POINT('Ctrl Pts',(-23.,31.4583333469893,39.8371685740842));
#5657=CARTESIAN_POINT('Ctrl Pts',(-33.6743371481683,31.2500000136559,33.6743371481684));
#5658=CARTESIAN_POINT('Ctrl Pts',(-39.8371685740842,31.0416666803226,23.));
#5659=CARTESIAN_POINT('Ctrl Pts',(-46.,30.8333333469893,12.3256628518317));
#5660=CARTESIAN_POINT('Ctrl Pts',(-46.,30.6250000136559,0.));
#5661=CARTESIAN_POINT('Ctrl Pts',(-46.,30.4166666803226,-12.3256628518316));
#5662=CARTESIAN_POINT('Ctrl Pts',(-39.8371685740842,30.2083333469893,-23.));
#5663=CARTESIAN_POINT('Ctrl Pts',(-33.6743371481684,30.0000000136559,-33.6743371481684));
#5664=CARTESIAN_POINT('Ctrl Pts',(-23.,29.7916666803226,-39.8371685740842));
#5665=CARTESIAN_POINT('Ctrl Pts',(-12.3256628518317,29.5833333469893,-46.));
#5666=CARTESIAN_POINT('Ctrl Pts',(-2.81668763803891E-15,29.3750000136559,
-46.));
#5667=CARTESIAN_POINT('Ctrl Pts',(12.3256628518316,29.1666666803226,-46.));
#5668=CARTESIAN_POINT('Ctrl Pts',(23.,28.9583333469893,-39.8371685740842));
#5669=CARTESIAN_POINT('Ctrl Pts',(33.6743371481683,28.7500000136559,-33.6743371481684));
#5670=CARTESIAN_POINT('Ctrl Pts',(39.8371685740842,28.5416666803226,-23.));
#5671=CARTESIAN_POINT('Ctrl Pts',(46.,28.3333333469893,-12.3256628518317));
#5672=CARTESIAN_POINT('Ctrl Pts',(46.,28.1250000136559,-5.63337527607782E-15));
#5673=CARTESIAN_POINT('Ctrl Pts',(46.,27.9166666803226,12.3256628518316));
#5674=CARTESIAN_POINT('Ctrl Pts',(39.8371685740842,27.7083333469893,23.));
#5675=CARTESIAN_POINT('Ctrl Pts',(33.6743371481684,27.5000000136559,33.6743371481683));
#5676=CARTESIAN_POINT('Ctrl Pts',(23.,27.2916666803226,39.8371685740842));
#5677=CARTESIAN_POINT('Ctrl Pts',(12.3256628518317,27.0833333469893,46.));
#5678=CARTESIAN_POINT('Ctrl Pts',(8.45006291411674E-15,26.8750000136559,
46.));
#5679=CARTESIAN_POINT('Ctrl Pts',(-12.3256628518316,26.6666666803226,46.));
#5680=CARTESIAN_POINT('Ctrl Pts',(-23.,26.4583333469893,39.8371685740842));
#5681=CARTESIAN_POINT('Ctrl Pts',(-33.6743371481683,26.2500000136559,33.6743371481684));
#5682=CARTESIAN_POINT('Ctrl Pts',(-39.8371685740842,26.0416666803226,23.));
#5683=CARTESIAN_POINT('Ctrl Pts',(-46.,25.8333333469893,12.3256628518317));
#5684=CARTESIAN_POINT('Ctrl Pts',(-46.,25.6250000136559,0.));
#5685=CARTESIAN_POINT('Ctrl Pts',(-48.706329375,57.187500006828,-1.8898197019151E-14));
#5686=CARTESIAN_POINT('Ctrl Pts',(-48.706329375,56.9791666734946,-13.0508216223155));
#5687=CARTESIAN_POINT('Ctrl Pts',(-42.1809185638422,56.7708333401613,-24.3531646875));
#5688=CARTESIAN_POINT('Ctrl Pts',(-35.6555077526845,56.562500006828,-35.6555077526845));
#5689=CARTESIAN_POINT('Ctrl Pts',(-24.3531646875,56.3541666734946,-42.1809185638423));
#5690=CARTESIAN_POINT('Ctrl Pts',(-13.0508216223155,56.1458333401613,-48.706329375));
#5691=CARTESIAN_POINT('Ctrl Pts',(1.59157945007855E-14,55.937500006828,
-48.706329375));
#5692=CARTESIAN_POINT('Ctrl Pts',(13.0508216223155,55.7291666734946,-48.706329375));
#5693=CARTESIAN_POINT('Ctrl Pts',(24.3531646875,55.5208333401613,-42.1809185638422));
#5694=CARTESIAN_POINT('Ctrl Pts',(35.6555077526845,55.312500006828,-35.6555077526845));
#5695=CARTESIAN_POINT('Ctrl Pts',(42.1809185638422,55.1041666734946,-24.3531646875));
#5696=CARTESIAN_POINT('Ctrl Pts',(48.706329375,54.8958333401613,-13.0508216223155));
#5697=CARTESIAN_POINT('Ctrl Pts',(48.706329375,54.687500006828,1.293339198242E-14));
#5698=CARTESIAN_POINT('Ctrl Pts',(48.706329375,54.4791666734946,13.0508216223155));
#5699=CARTESIAN_POINT('Ctrl Pts',(42.1809185638422,54.2708333401613,24.3531646875));
#5700=CARTESIAN_POINT('Ctrl Pts',(35.6555077526845,54.062500006828,35.6555077526845));
#5701=CARTESIAN_POINT('Ctrl Pts',(24.3531646875,53.8541666734946,42.1809185638422));
#5702=CARTESIAN_POINT('Ctrl Pts',(13.0508216223155,53.6458333401613,48.706329375));
#5703=CARTESIAN_POINT('Ctrl Pts',(-9.95098946405443E-15,53.437500006828,
48.706329375));
#5704=CARTESIAN_POINT('Ctrl Pts',(-13.0508216223155,53.2291666734946,48.706329375));
#5705=CARTESIAN_POINT('Ctrl Pts',(-24.3531646875,53.0208333401613,42.1809185638423));
#5706=CARTESIAN_POINT('Ctrl Pts',(-35.6555077526845,52.812500006828,35.6555077526845));
#5707=CARTESIAN_POINT('Ctrl Pts',(-42.1809185638422,52.6041666734946,24.3531646875));
#5708=CARTESIAN_POINT('Ctrl Pts',(-48.706329375,52.3958333401613,13.0508216223155));
#5709=CARTESIAN_POINT('Ctrl Pts',(-48.706329375,52.187500006828,-1.8898197019151E-14));
#5710=CARTESIAN_POINT('Ctrl Pts',(-48.706329375,51.9791666734946,-13.0508216223155));
#5711=CARTESIAN_POINT('Ctrl Pts',(-42.1809185638422,51.7708333401613,-24.3531646875));
#5712=CARTESIAN_POINT('Ctrl Pts',(-35.6555077526845,51.562500006828,-35.6555077526845));
#5713=CARTESIAN_POINT('Ctrl Pts',(-24.3531646875,51.3541666734946,-42.1809185638423));
#5714=CARTESIAN_POINT('Ctrl Pts',(-13.0508216223155,51.1458333401613,-48.706329375));
#5715=CARTESIAN_POINT('Ctrl Pts',(1.59157945007855E-14,50.937500006828,
-48.706329375));
#5716=CARTESIAN_POINT('Ctrl Pts',(13.0508216223155,50.7291666734946,-48.706329375));
#5717=CARTESIAN_POINT('Ctrl Pts',(24.3531646875,50.5208333401613,-42.1809185638422));
#5718=CARTESIAN_POINT('Ctrl Pts',(35.6555077526845,50.312500006828,-35.6555077526845));
#5719=CARTESIAN_POINT('Ctrl Pts',(42.1809185638422,50.1041666734946,-24.3531646875));
#5720=CARTESIAN_POINT('Ctrl Pts',(48.706329375,49.8958333401613,-13.0508216223155));
#5721=CARTESIAN_POINT('Ctrl Pts',(48.706329375,49.687500006828,1.293339198242E-14));
#5722=CARTESIAN_POINT('Ctrl Pts',(48.706329375,49.4791666734946,13.0508216223155));
#5723=CARTESIAN_POINT('Ctrl Pts',(42.1809185638422,49.2708333401613,24.3531646875));
#5724=CARTESIAN_POINT('Ctrl Pts',(35.6555077526845,49.062500006828,35.6555077526845));
#5725=CARTESIAN_POINT('Ctrl Pts',(24.3531646875,48.8541666734946,42.1809185638422));
#5726=CARTESIAN_POINT('Ctrl Pts',(13.0508216223155,48.6458333401613,48.706329375));
#5727=CARTESIAN_POINT('Ctrl Pts',(-9.95098946405443E-15,48.437500006828,
48.706329375));
#5728=CARTESIAN_POINT('Ctrl Pts',(-13.0508216223155,48.2291666734946,48.706329375));
#5729=CARTESIAN_POINT('Ctrl Pts',(-24.3531646875,48.0208333401613,42.1809185638423));
#5730=CARTESIAN_POINT('Ctrl Pts',(-35.6555077526845,47.812500006828,35.6555077526845));
#5731=CARTESIAN_POINT('Ctrl Pts',(-42.1809185638422,47.6041666734946,24.3531646875));
#5732=CARTESIAN_POINT('Ctrl Pts',(-48.706329375,47.3958333401613,13.0508216223155));
#5733=CARTESIAN_POINT('Ctrl Pts',(-48.706329375,47.187500006828,-1.8898197019151E-14));
#5734=CARTESIAN_POINT('Ctrl Pts',(-48.706329375,46.9791666734946,-13.0508216223155));
#5735=CARTESIAN_POINT('Ctrl Pts',(-42.1809185638422,46.7708333401613,-24.3531646875));
#5736=CARTESIAN_POINT('Ctrl Pts',(-35.6555077526845,46.562500006828,-35.6555077526845));
#5737=CARTESIAN_POINT('Ctrl Pts',(-24.3531646875,46.3541666734946,-42.1809185638423));
#5738=CARTESIAN_POINT('Ctrl Pts',(-13.0508216223155,46.1458333401613,-48.706329375));
#5739=CARTESIAN_POINT('Ctrl Pts',(1.59157945007855E-14,45.937500006828,
-48.706329375));
#5740=CARTESIAN_POINT('Ctrl Pts',(13.0508216223155,45.7291666734946,-48.706329375));
#5741=CARTESIAN_POINT('Ctrl Pts',(24.3531646875,45.5208333401613,-42.1809185638422));
#5742=CARTESIAN_POINT('Ctrl Pts',(35.6555077526845,45.312500006828,-35.6555077526845));
#5743=CARTESIAN_POINT('Ctrl Pts',(42.1809185638422,45.1041666734946,-24.3531646875));
#5744=CARTESIAN_POINT('Ctrl Pts',(48.706329375,44.8958333401613,-13.0508216223155));
#5745=CARTESIAN_POINT('Ctrl Pts',(48.706329375,44.687500006828,1.293339198242E-14));
#5746=CARTESIAN_POINT('Ctrl Pts',(48.706329375,44.4791666734946,13.0508216223155));
#5747=CARTESIAN_POINT('Ctrl Pts',(42.1809185638422,44.2708333401613,24.3531646875));
#5748=CARTESIAN_POINT('Ctrl Pts',(35.6555077526845,44.062500006828,35.6555077526845));
#5749=CARTESIAN_POINT('Ctrl Pts',(24.3531646875,43.8541666734946,42.1809185638422));
#5750=CARTESIAN_POINT('Ctrl Pts',(13.0508216223155,43.6458333401613,48.706329375));
#5751=CARTESIAN_POINT('Ctrl Pts',(-9.95098946405443E-15,43.437500006828,
48.706329375));
#5752=CARTESIAN_POINT('Ctrl Pts',(-13.0508216223155,43.2291666734946,48.706329375));
#5753=CARTESIAN_POINT('Ctrl Pts',(-24.3531646875,43.0208333401613,42.1809185638423));
#5754=CARTESIAN_POINT('Ctrl Pts',(-35.6555077526845,42.812500006828,35.6555077526845));
#5755=CARTESIAN_POINT('Ctrl Pts',(-42.1809185638422,42.6041666734946,24.3531646875));
#5756=CARTESIAN_POINT('Ctrl Pts',(-48.706329375,42.3958333401613,13.0508216223155));
#5757=CARTESIAN_POINT('Ctrl Pts',(-48.706329375,42.187500006828,-1.8898197019151E-14));
#5758=CARTESIAN_POINT('Ctrl Pts',(-48.706329375,41.9791666734946,-13.0508216223155));
#5759=CARTESIAN_POINT('Ctrl Pts',(-42.1809185638422,41.7708333401613,-24.3531646875));
#5760=CARTESIAN_POINT('Ctrl Pts',(-35.6555077526845,41.562500006828,-35.6555077526845));
#5761=CARTESIAN_POINT('Ctrl Pts',(-24.3531646875,41.3541666734946,-42.1809185638423));
#5762=CARTESIAN_POINT('Ctrl Pts',(-13.0508216223155,41.1458333401613,-48.706329375));
#5763=CARTESIAN_POINT('Ctrl Pts',(1.59157945007855E-14,40.937500006828,
-48.706329375));
#5764=CARTESIAN_POINT('Ctrl Pts',(13.0508216223155,40.7291666734946,-48.706329375));
#5765=CARTESIAN_POINT('Ctrl Pts',(24.3531646875,40.5208333401613,-42.1809185638422));
#5766=CARTESIAN_POINT('Ctrl Pts',(35.6555077526845,40.312500006828,-35.6555077526845));
#5767=CARTESIAN_POINT('Ctrl Pts',(42.1809185638422,40.1041666734946,-24.3531646875));
#5768=CARTESIAN_POINT('Ctrl Pts',(48.706329375,39.8958333401613,-13.0508216223155));
#5769=CARTESIAN_POINT('Ctrl Pts',(48.706329375,39.687500006828,1.293339198242E-14));
#5770=CARTESIAN_POINT('Ctrl Pts',(48.706329375,39.4791666734946,13.0508216223155));
#5771=CARTESIAN_POINT('Ctrl Pts',(42.1809185638422,39.2708333401613,24.3531646875));
#5772=CARTESIAN_POINT('Ctrl Pts',(35.6555077526845,39.062500006828,35.6555077526845));
#5773=CARTESIAN_POINT('Ctrl Pts',(24.3531646875,38.8541666734946,42.1809185638422));
#5774=CARTESIAN_POINT('Ctrl Pts',(13.0508216223155,38.6458333401613,48.706329375));
#5775=CARTESIAN_POINT('Ctrl Pts',(-9.95098946405443E-15,38.437500006828,
48.706329375));
#5776=CARTESIAN_POINT('Ctrl Pts',(-13.0508216223155,38.2291666734946,48.706329375));
#5777=CARTESIAN_POINT('Ctrl Pts',(-24.3531646875,38.0208333401613,42.1809185638423));
#5778=CARTESIAN_POINT('Ctrl Pts',(-35.6555077526845,37.812500006828,35.6555077526845));
#5779=CARTESIAN_POINT('Ctrl Pts',(-42.1809185638422,37.6041666734946,24.3531646875));
#5780=CARTESIAN_POINT('Ctrl Pts',(-48.706329375,37.3958333401613,13.0508216223155));
#5781=CARTESIAN_POINT('Ctrl Pts',(-48.706329375,37.187500006828,-1.8898197019151E-14));
#5782=CARTESIAN_POINT('Ctrl Pts',(-48.706329375,36.9791666734946,-13.0508216223155));
#5783=CARTESIAN_POINT('Ctrl Pts',(-42.1809185638422,36.7708333401613,-24.3531646875));
#5784=CARTESIAN_POINT('Ctrl Pts',(-35.6555077526845,36.562500006828,-35.6555077526845));
#5785=CARTESIAN_POINT('Ctrl Pts',(-24.3531646875,36.3541666734946,-42.1809185638423));
#5786=CARTESIAN_POINT('Ctrl Pts',(-13.0508216223155,36.1458333401613,-48.706329375));
#5787=CARTESIAN_POINT('Ctrl Pts',(1.59157945007855E-14,35.937500006828,
-48.706329375));
#5788=CARTESIAN_POINT('Ctrl Pts',(13.0508216223155,35.7291666734946,-48.706329375));
#5789=CARTESIAN_POINT('Ctrl Pts',(24.3531646875,35.5208333401613,-42.1809185638422));
#5790=CARTESIAN_POINT('Ctrl Pts',(35.6555077526845,35.312500006828,-35.6555077526845));
#5791=CARTESIAN_POINT('Ctrl Pts',(42.1809185638422,35.1041666734946,-24.3531646875));
#5792=CARTESIAN_POINT('Ctrl Pts',(48.706329375,34.8958333401613,-13.0508216223155));
#5793=CARTESIAN_POINT('Ctrl Pts',(48.706329375,34.687500006828,1.293339198242E-14));
#5794=CARTESIAN_POINT('Ctrl Pts',(48.706329375,34.4791666734946,13.0508216223155));
#5795=CARTESIAN_POINT('Ctrl Pts',(42.1809185638422,34.2708333401613,24.3531646875));
#5796=CARTESIAN_POINT('Ctrl Pts',(35.6555077526845,34.062500006828,35.6555077526845));
#5797=CARTESIAN_POINT('Ctrl Pts',(24.3531646875,33.8541666734946,42.1809185638422));
#5798=CARTESIAN_POINT('Ctrl Pts',(13.0508216223155,33.6458333401613,48.706329375));
#5799=CARTESIAN_POINT('Ctrl Pts',(-9.95098946405443E-15,33.437500006828,
48.706329375));
#5800=CARTESIAN_POINT('Ctrl Pts',(-13.0508216223155,33.2291666734946,48.706329375));
#5801=CARTESIAN_POINT('Ctrl Pts',(-24.3531646875,33.0208333401613,42.1809185638423));
#5802=CARTESIAN_POINT('Ctrl Pts',(-35.6555077526845,32.812500006828,35.6555077526845));
#5803=CARTESIAN_POINT('Ctrl Pts',(-42.1809185638422,32.6041666734946,24.3531646875));
#5804=CARTESIAN_POINT('Ctrl Pts',(-48.706329375,32.3958333401613,13.0508216223155));
#5805=CARTESIAN_POINT('Ctrl Pts',(-48.706329375,32.187500006828,-1.8898197019151E-14));
#5806=CARTESIAN_POINT('Ctrl Pts',(-48.706329375,31.9791666734946,-13.0508216223155));
#5807=CARTESIAN_POINT('Ctrl Pts',(-42.1809185638422,31.7708333401613,-24.3531646875));
#5808=CARTESIAN_POINT('Ctrl Pts',(-35.6555077526845,31.562500006828,-35.6555077526845));
#5809=CARTESIAN_POINT('Ctrl Pts',(-24.3531646875,31.3541666734946,-42.1809185638423));
#5810=CARTESIAN_POINT('Ctrl Pts',(-13.0508216223155,31.1458333401613,-48.706329375));
#5811=CARTESIAN_POINT('Ctrl Pts',(1.59157945007855E-14,30.937500006828,
-48.706329375));
#5812=CARTESIAN_POINT('Ctrl Pts',(13.0508216223155,30.7291666734946,-48.706329375));
#5813=CARTESIAN_POINT('Ctrl Pts',(24.3531646875,30.5208333401613,-42.1809185638422));
#5814=CARTESIAN_POINT('Ctrl Pts',(35.6555077526845,30.312500006828,-35.6555077526845));
#5815=CARTESIAN_POINT('Ctrl Pts',(42.1809185638422,30.1041666734946,-24.3531646875));
#5816=CARTESIAN_POINT('Ctrl Pts',(48.706329375,29.8958333401613,-13.0508216223155));
#5817=CARTESIAN_POINT('Ctrl Pts',(48.706329375,29.687500006828,1.293339198242E-14));
#5818=CARTESIAN_POINT('Ctrl Pts',(48.706329375,29.4791666734946,13.0508216223155));
#5819=CARTESIAN_POINT('Ctrl Pts',(42.1809185638422,29.2708333401613,24.3531646875));
#5820=CARTESIAN_POINT('Ctrl Pts',(35.6555077526845,29.062500006828,35.6555077526845));
#5821=CARTESIAN_POINT('Ctrl Pts',(24.3531646875,28.8541666734946,42.1809185638422));
#5822=CARTESIAN_POINT('Ctrl Pts',(13.0508216223155,28.6458333401613,48.706329375));
#5823=CARTESIAN_POINT('Ctrl Pts',(-9.95098946405443E-15,28.437500006828,
48.706329375));
#5824=CARTESIAN_POINT('Ctrl Pts',(-13.0508216223155,28.2291666734946,48.706329375));
#5825=CARTESIAN_POINT('Ctrl Pts',(-24.3531646875,28.0208333401613,42.1809185638423));
#5826=CARTESIAN_POINT('Ctrl Pts',(-35.6555077526845,27.812500006828,35.6555077526845));
#5827=CARTESIAN_POINT('Ctrl Pts',(-42.1809185638422,27.6041666734946,24.3531646875));
#5828=CARTESIAN_POINT('Ctrl Pts',(-48.706329375,27.3958333401613,13.0508216223155));
#5829=CARTESIAN_POINT('Ctrl Pts',(-48.706329375,27.187500006828,-1.8898197019151E-14));
#5830=CARTESIAN_POINT('',(3.61292728433799,55.8792520480092,-48.5721450795008));
#5831=CARTESIAN_POINT('',(48.5134353784345,54.7574536451604,-4.33048599679674));
#5832=CARTESIAN_POINT('Ctrl Pts',(3.61292728433799,55.8792520480093,-48.5721450795008));
#5833=CARTESIAN_POINT('Ctrl Pts',(14.7133549689477,55.6985216017707,-47.7464652997852));
#5834=CARTESIAN_POINT('Ctrl Pts',(24.3531646875,55.5208333401613,-42.1809185638422));
#5835=CARTESIAN_POINT('Ctrl Pts',(35.6555077526845,55.312500006828,-35.6555077526845));
#5836=CARTESIAN_POINT('Ctrl Pts',(42.1809185638422,55.1041666734946,-24.3531646875));
#5837=CARTESIAN_POINT('Ctrl Pts',(47.5573898704235,54.9325149229327,-15.0408432190651));
#5838=CARTESIAN_POINT('Ctrl Pts',(48.5134353784344,54.7574536451604,-4.33048599679674));
#5839=CARTESIAN_POINT('Origin',(-4513.80899778907,8008.28355048454,-4.33048540714616));
#5840=CARTESIAN_POINT('Ctrl Pts',(3.61292728433799,54.3132892765089,-45.8578974271399));
#5841=CARTESIAN_POINT('Ctrl Pts',(3.612927284338,54.4468822859549,-46.089460636719));
#5842=CARTESIAN_POINT('Ctrl Pts',(3.61292728433798,54.7140705280012,-46.5525857733052));
#5843=CARTESIAN_POINT('Ctrl Pts',(3.61292728433799,54.9812630238615,-47.0157084557285));
#5844=CARTESIAN_POINT('Ctrl Pts',(3.61292728433799,55.3696539378594,-47.6888965792834));
#5845=CARTESIAN_POINT('Ctrl Pts',(3.61292728433799,55.624451287085,-48.1305218136162));
#5846=CARTESIAN_POINT('Ctrl Pts',(3.61292728433799,55.8792520480092,-48.5721450795008));
#5847=CARTESIAN_POINT('Ctrl Pts',(-46.,55.6250000136559,0.));
#5848=CARTESIAN_POINT('Ctrl Pts',(-46.,55.4166666803226,-12.3256628518316));
#5849=CARTESIAN_POINT('Ctrl Pts',(-39.8371685740842,55.2083333469893,-23.));
#5850=CARTESIAN_POINT('Ctrl Pts',(-33.6743371481684,55.0000000136559,-33.6743371481684));
#5851=CARTESIAN_POINT('Ctrl Pts',(-23.,54.7916666803226,-39.8371685740842));
#5852=CARTESIAN_POINT('Ctrl Pts',(-12.3256628518317,54.5833333469893,-46.));
#5853=CARTESIAN_POINT('Ctrl Pts',(-2.81668763803891E-15,54.3750000136559,
-46.));
#5854=CARTESIAN_POINT('Ctrl Pts',(12.3256628518316,54.1666666803226,-46.));
#5855=CARTESIAN_POINT('Ctrl Pts',(23.,53.9583333469893,-39.8371685740842));
#5856=CARTESIAN_POINT('Ctrl Pts',(33.6743371481683,53.7500000136559,-33.6743371481684));
#5857=CARTESIAN_POINT('Ctrl Pts',(39.8371685740842,53.5416666803226,-23.));
#5858=CARTESIAN_POINT('Ctrl Pts',(46.,53.3333333469893,-12.3256628518317));
#5859=CARTESIAN_POINT('Ctrl Pts',(46.,53.1250000136559,-5.63337527607782E-15));
#5860=CARTESIAN_POINT('Ctrl Pts',(46.,52.9166666803226,12.3256628518316));
#5861=CARTESIAN_POINT('Ctrl Pts',(39.8371685740842,52.7083333469893,23.));
#5862=CARTESIAN_POINT('Ctrl Pts',(33.6743371481684,52.5000000136559,33.6743371481683));
#5863=CARTESIAN_POINT('Ctrl Pts',(23.,52.2916666803226,39.8371685740842));
#5864=CARTESIAN_POINT('Ctrl Pts',(12.3256628518317,52.0833333469893,46.));
#5865=CARTESIAN_POINT('Ctrl Pts',(8.45006291411674E-15,51.8750000136559,
46.));
#5866=CARTESIAN_POINT('Ctrl Pts',(-12.3256628518316,51.6666666803226,46.));
#5867=CARTESIAN_POINT('Ctrl Pts',(-23.,51.4583333469893,39.8371685740842));
#5868=CARTESIAN_POINT('Ctrl Pts',(-33.6743371481683,51.2500000136559,33.6743371481684));
#5869=CARTESIAN_POINT('Ctrl Pts',(-39.8371685740842,51.0416666803226,23.));
#5870=CARTESIAN_POINT('Ctrl Pts',(-46.,50.8333333469893,12.3256628518317));
#5871=CARTESIAN_POINT('Ctrl Pts',(-46.,50.6250000136559,0.));
#5872=CARTESIAN_POINT('Ctrl Pts',(-46.,50.4166666803226,-12.3256628518316));
#5873=CARTESIAN_POINT('Ctrl Pts',(-39.8371685740842,50.2083333469893,-23.));
#5874=CARTESIAN_POINT('Ctrl Pts',(-33.6743371481684,50.0000000136559,-33.6743371481684));
#5875=CARTESIAN_POINT('Ctrl Pts',(-23.,49.7916666803226,-39.8371685740842));
#5876=CARTESIAN_POINT('Ctrl Pts',(-12.3256628518317,49.5833333469893,-46.));
#5877=CARTESIAN_POINT('Ctrl Pts',(-2.81668763803891E-15,49.3750000136559,
-46.));
#5878=CARTESIAN_POINT('Ctrl Pts',(12.3256628518316,49.1666666803226,-46.));
#5879=CARTESIAN_POINT('Ctrl Pts',(23.,48.9583333469893,-39.8371685740842));
#5880=CARTESIAN_POINT('Ctrl Pts',(33.6743371481683,48.7500000136559,-33.6743371481684));
#5881=CARTESIAN_POINT('Ctrl Pts',(39.8371685740842,48.5416666803226,-23.));
#5882=CARTESIAN_POINT('Ctrl Pts',(46.,48.3333333469893,-12.3256628518317));
#5883=CARTESIAN_POINT('Ctrl Pts',(46.,48.1250000136559,-5.63337527607782E-15));
#5884=CARTESIAN_POINT('Ctrl Pts',(46.,47.9166666803226,12.3256628518316));
#5885=CARTESIAN_POINT('Ctrl Pts',(39.8371685740842,47.7083333469893,23.));
#5886=CARTESIAN_POINT('Ctrl Pts',(33.6743371481684,47.5000000136559,33.6743371481683));
#5887=CARTESIAN_POINT('Ctrl Pts',(23.,47.2916666803226,39.8371685740842));
#5888=CARTESIAN_POINT('Ctrl Pts',(12.3256628518317,47.0833333469893,46.));
#5889=CARTESIAN_POINT('Ctrl Pts',(8.45006291411674E-15,46.8750000136559,
46.));
#5890=CARTESIAN_POINT('Ctrl Pts',(-12.3256628518316,46.6666666803226,46.));
#5891=CARTESIAN_POINT('Ctrl Pts',(-23.,46.4583333469893,39.8371685740842));
#5892=CARTESIAN_POINT('Ctrl Pts',(-33.6743371481683,46.2500000136559,33.6743371481684));
#5893=CARTESIAN_POINT('Ctrl Pts',(-39.8371685740842,46.0416666803226,23.));
#5894=CARTESIAN_POINT('Ctrl Pts',(-46.,45.8333333469892,12.3256628518317));
#5895=CARTESIAN_POINT('Ctrl Pts',(-46.,45.6250000136559,0.));
#5896=CARTESIAN_POINT('Ctrl Pts',(-46.,45.4166666803226,-12.3256628518316));
#5897=CARTESIAN_POINT('Ctrl Pts',(-39.8371685740842,45.2083333469893,-23.));
#5898=CARTESIAN_POINT('Ctrl Pts',(-33.6743371481684,45.0000000136559,-33.6743371481684));
#5899=CARTESIAN_POINT('Ctrl Pts',(-23.,44.7916666803226,-39.8371685740842));
#5900=CARTESIAN_POINT('Ctrl Pts',(-12.3256628518317,44.5833333469893,-46.));
#5901=CARTESIAN_POINT('Ctrl Pts',(-2.81668763803891E-15,44.3750000136559,
-46.));
#5902=CARTESIAN_POINT('Ctrl Pts',(12.3256628518316,44.1666666803226,-46.));
#5903=CARTESIAN_POINT('Ctrl Pts',(23.,43.9583333469893,-39.8371685740842));
#5904=CARTESIAN_POINT('Ctrl Pts',(33.6743371481683,43.7500000136559,-33.6743371481684));
#5905=CARTESIAN_POINT('Ctrl Pts',(39.8371685740842,43.5416666803226,-23.));
#5906=CARTESIAN_POINT('Ctrl Pts',(46.,43.3333333469893,-12.3256628518317));
#5907=CARTESIAN_POINT('Ctrl Pts',(46.,43.1250000136559,-5.63337527607782E-15));
#5908=CARTESIAN_POINT('Ctrl Pts',(46.,42.9166666803226,12.3256628518316));
#5909=CARTESIAN_POINT('Ctrl Pts',(39.8371685740842,42.7083333469893,23.));
#5910=CARTESIAN_POINT('Ctrl Pts',(33.6743371481684,42.5000000136559,33.6743371481683));
#5911=CARTESIAN_POINT('Ctrl Pts',(23.,42.2916666803226,39.8371685740842));
#5912=CARTESIAN_POINT('Ctrl Pts',(12.3256628518317,42.0833333469893,46.));
#5913=CARTESIAN_POINT('Ctrl Pts',(8.45006291411674E-15,41.8750000136559,
46.));
#5914=CARTESIAN_POINT('Ctrl Pts',(-12.3256628518316,41.6666666803226,46.));
#5915=CARTESIAN_POINT('Ctrl Pts',(-23.,41.4583333469893,39.8371685740842));
#5916=CARTESIAN_POINT('Ctrl Pts',(-33.6743371481683,41.2500000136559,33.6743371481684));
#5917=CARTESIAN_POINT('Ctrl Pts',(-39.8371685740842,41.0416666803226,23.));
#5918=CARTESIAN_POINT('Ctrl Pts',(-46.,40.8333333469893,12.3256628518317));
#5919=CARTESIAN_POINT('Ctrl Pts',(-46.,40.6250000136559,0.));
#5920=CARTESIAN_POINT('Ctrl Pts',(-46.,40.4166666803226,-12.3256628518316));
#5921=CARTESIAN_POINT('Ctrl Pts',(-39.8371685740842,40.2083333469893,-23.));
#5922=CARTESIAN_POINT('Ctrl Pts',(-33.6743371481684,40.0000000136559,-33.6743371481684));
#5923=CARTESIAN_POINT('Ctrl Pts',(-23.,39.7916666803226,-39.8371685740842));
#5924=CARTESIAN_POINT('Ctrl Pts',(-12.3256628518317,39.5833333469893,-46.));
#5925=CARTESIAN_POINT('Ctrl Pts',(-2.81668763803891E-15,39.3750000136559,
-46.));
#5926=CARTESIAN_POINT('Ctrl Pts',(12.3256628518316,39.1666666803226,-46.));
#5927=CARTESIAN_POINT('Ctrl Pts',(23.,38.9583333469893,-39.8371685740842));
#5928=CARTESIAN_POINT('Ctrl Pts',(33.6743371481683,38.7500000136559,-33.6743371481684));
#5929=CARTESIAN_POINT('Ctrl Pts',(39.8371685740842,38.5416666803226,-23.));
#5930=CARTESIAN_POINT('Ctrl Pts',(46.,38.3333333469893,-12.3256628518317));
#5931=CARTESIAN_POINT('Ctrl Pts',(46.,38.1250000136559,-5.63337527607782E-15));
#5932=CARTESIAN_POINT('Ctrl Pts',(46.,37.9166666803226,12.3256628518316));
#5933=CARTESIAN_POINT('Ctrl Pts',(39.8371685740842,37.7083333469893,23.));
#5934=CARTESIAN_POINT('Ctrl Pts',(33.6743371481684,37.5000000136559,33.6743371481683));
#5935=CARTESIAN_POINT('Ctrl Pts',(23.,37.2916666803226,39.8371685740842));
#5936=CARTESIAN_POINT('Ctrl Pts',(12.3256628518317,37.0833333469893,46.));
#5937=CARTESIAN_POINT('Ctrl Pts',(8.45006291411674E-15,36.8750000136559,
46.));
#5938=CARTESIAN_POINT('Ctrl Pts',(-12.3256628518316,36.6666666803226,46.));
#5939=CARTESIAN_POINT('Ctrl Pts',(-23.,36.4583333469893,39.8371685740842));
#5940=CARTESIAN_POINT('Ctrl Pts',(-33.6743371481683,36.2500000136559,33.6743371481684));
#5941=CARTESIAN_POINT('Ctrl Pts',(-39.8371685740842,36.0416666803226,23.));
#5942=CARTESIAN_POINT('Ctrl Pts',(-46.,35.8333333469893,12.3256628518317));
#5943=CARTESIAN_POINT('Ctrl Pts',(-46.,35.6250000136559,0.));
#5944=CARTESIAN_POINT('Ctrl Pts',(-46.,35.4166666803226,-12.3256628518316));
#5945=CARTESIAN_POINT('Ctrl Pts',(-39.8371685740842,35.2083333469893,-23.));
#5946=CARTESIAN_POINT('Ctrl Pts',(-33.6743371481684,35.0000000136559,-33.6743371481684));
#5947=CARTESIAN_POINT('Ctrl Pts',(-23.,34.7916666803226,-39.8371685740842));
#5948=CARTESIAN_POINT('Ctrl Pts',(-12.3256628518317,34.5833333469893,-46.));
#5949=CARTESIAN_POINT('Ctrl Pts',(-2.81668763803891E-15,34.3750000136559,
-46.));
#5950=CARTESIAN_POINT('Ctrl Pts',(12.3256628518316,34.1666666803226,-46.));
#5951=CARTESIAN_POINT('Ctrl Pts',(23.,33.9583333469893,-39.8371685740842));
#5952=CARTESIAN_POINT('Ctrl Pts',(33.6743371481683,33.7500000136559,-33.6743371481684));
#5953=CARTESIAN_POINT('Ctrl Pts',(39.8371685740842,33.5416666803226,-23.));
#5954=CARTESIAN_POINT('Ctrl Pts',(46.,33.3333333469893,-12.3256628518317));
#5955=CARTESIAN_POINT('Ctrl Pts',(46.,33.1250000136559,-5.63337527607782E-15));
#5956=CARTESIAN_POINT('Ctrl Pts',(46.,32.9166666803226,12.3256628518316));
#5957=CARTESIAN_POINT('Ctrl Pts',(39.8371685740842,32.7083333469893,23.));
#5958=CARTESIAN_POINT('Ctrl Pts',(33.6743371481684,32.5000000136559,33.6743371481683));
#5959=CARTESIAN_POINT('Ctrl Pts',(23.,32.2916666803226,39.8371685740842));
#5960=CARTESIAN_POINT('Ctrl Pts',(12.3256628518317,32.0833333469893,46.));
#5961=CARTESIAN_POINT('Ctrl Pts',(8.45006291411674E-15,31.8750000136559,
46.));
#5962=CARTESIAN_POINT('Ctrl Pts',(-12.3256628518316,31.6666666803226,46.));
#5963=CARTESIAN_POINT('Ctrl Pts',(-23.,31.4583333469893,39.8371685740842));
#5964=CARTESIAN_POINT('Ctrl Pts',(-33.6743371481683,31.2500000136559,33.6743371481684));
#5965=CARTESIAN_POINT('Ctrl Pts',(-39.8371685740842,31.0416666803226,23.));
#5966=CARTESIAN_POINT('Ctrl Pts',(-46.,30.8333333469893,12.3256628518317));
#5967=CARTESIAN_POINT('Ctrl Pts',(-46.,30.6250000136559,0.));
#5968=CARTESIAN_POINT('Ctrl Pts',(-46.,30.4166666803226,-12.3256628518316));
#5969=CARTESIAN_POINT('Ctrl Pts',(-39.8371685740842,30.2083333469893,-23.));
#5970=CARTESIAN_POINT('Ctrl Pts',(-33.6743371481684,30.0000000136559,-33.6743371481684));
#5971=CARTESIAN_POINT('Ctrl Pts',(-23.,29.7916666803226,-39.8371685740842));
#5972=CARTESIAN_POINT('Ctrl Pts',(-12.3256628518317,29.5833333469893,-46.));
#5973=CARTESIAN_POINT('Ctrl Pts',(-2.81668763803891E-15,29.3750000136559,
-46.));
#5974=CARTESIAN_POINT('Ctrl Pts',(12.3256628518316,29.1666666803226,-46.));
#5975=CARTESIAN_POINT('Ctrl Pts',(23.,28.9583333469893,-39.8371685740842));
#5976=CARTESIAN_POINT('Ctrl Pts',(33.6743371481683,28.7500000136559,-33.6743371481684));
#5977=CARTESIAN_POINT('Ctrl Pts',(39.8371685740842,28.5416666803226,-23.));
#5978=CARTESIAN_POINT('Ctrl Pts',(46.,28.3333333469893,-12.3256628518317));
#5979=CARTESIAN_POINT('Ctrl Pts',(46.,28.1250000136559,-5.63337527607782E-15));
#5980=CARTESIAN_POINT('Ctrl Pts',(46.,27.9166666803226,12.3256628518316));
#5981=CARTESIAN_POINT('Ctrl Pts',(39.8371685740842,27.7083333469893,23.));
#5982=CARTESIAN_POINT('Ctrl Pts',(33.6743371481684,27.5000000136559,33.6743371481683));
#5983=CARTESIAN_POINT('Ctrl Pts',(23.,27.2916666803226,39.8371685740842));
#5984=CARTESIAN_POINT('Ctrl Pts',(12.3256628518317,27.0833333469893,46.));
#5985=CARTESIAN_POINT('Ctrl Pts',(8.45006291411674E-15,26.8750000136559,
46.));
#5986=CARTESIAN_POINT('Ctrl Pts',(-12.3256628518316,26.6666666803226,46.));
#5987=CARTESIAN_POINT('Ctrl Pts',(-23.,26.4583333469893,39.8371685740842));
#5988=CARTESIAN_POINT('Ctrl Pts',(-33.6743371481683,26.2500000136559,33.6743371481684));
#5989=CARTESIAN_POINT('Ctrl Pts',(-39.8371685740842,26.0416666803226,23.));
#5990=CARTESIAN_POINT('Ctrl Pts',(-46.,25.8333333469893,12.3256628518317));
#5991=CARTESIAN_POINT('Ctrl Pts',(-46.,25.6250000136559,0.));
#5992=CARTESIAN_POINT('Ctrl Pts',(-48.706329375,57.187500006828,-1.8898197019151E-14));
#5993=CARTESIAN_POINT('Ctrl Pts',(-48.706329375,56.9791666734946,-13.0508216223155));
#5994=CARTESIAN_POINT('Ctrl Pts',(-42.1809185638422,56.7708333401613,-24.3531646875));
#5995=CARTESIAN_POINT('Ctrl Pts',(-35.6555077526845,56.562500006828,-35.6555077526845));
#5996=CARTESIAN_POINT('Ctrl Pts',(-24.3531646875,56.3541666734946,-42.1809185638423));
#5997=CARTESIAN_POINT('Ctrl Pts',(-13.0508216223155,56.1458333401613,-48.706329375));
#5998=CARTESIAN_POINT('Ctrl Pts',(1.59157945007855E-14,55.937500006828,
-48.706329375));
#5999=CARTESIAN_POINT('Ctrl Pts',(13.0508216223155,55.7291666734946,-48.706329375));
#6000=CARTESIAN_POINT('Ctrl Pts',(24.3531646875,55.5208333401613,-42.1809185638422));
#6001=CARTESIAN_POINT('Ctrl Pts',(35.6555077526845,55.312500006828,-35.6555077526845));
#6002=CARTESIAN_POINT('Ctrl Pts',(42.1809185638422,55.1041666734946,-24.3531646875));
#6003=CARTESIAN_POINT('Ctrl Pts',(48.706329375,54.8958333401613,-13.0508216223155));
#6004=CARTESIAN_POINT('Ctrl Pts',(48.706329375,54.687500006828,1.293339198242E-14));
#6005=CARTESIAN_POINT('Ctrl Pts',(48.706329375,54.4791666734946,13.0508216223155));
#6006=CARTESIAN_POINT('Ctrl Pts',(42.1809185638422,54.2708333401613,24.3531646875));
#6007=CARTESIAN_POINT('Ctrl Pts',(35.6555077526845,54.062500006828,35.6555077526845));
#6008=CARTESIAN_POINT('Ctrl Pts',(24.3531646875,53.8541666734946,42.1809185638422));
#6009=CARTESIAN_POINT('Ctrl Pts',(13.0508216223155,53.6458333401613,48.706329375));
#6010=CARTESIAN_POINT('Ctrl Pts',(-9.95098946405443E-15,53.437500006828,
48.706329375));
#6011=CARTESIAN_POINT('Ctrl Pts',(-13.0508216223155,53.2291666734946,48.706329375));
#6012=CARTESIAN_POINT('Ctrl Pts',(-24.3531646875,53.0208333401613,42.1809185638423));
#6013=CARTESIAN_POINT('Ctrl Pts',(-35.6555077526845,52.812500006828,35.6555077526845));
#6014=CARTESIAN_POINT('Ctrl Pts',(-42.1809185638422,52.6041666734946,24.3531646875));
#6015=CARTESIAN_POINT('Ctrl Pts',(-48.706329375,52.3958333401613,13.0508216223155));
#6016=CARTESIAN_POINT('Ctrl Pts',(-48.706329375,52.187500006828,-1.8898197019151E-14));
#6017=CARTESIAN_POINT('Ctrl Pts',(-48.706329375,51.9791666734946,-13.0508216223155));
#6018=CARTESIAN_POINT('Ctrl Pts',(-42.1809185638422,51.7708333401613,-24.3531646875));
#6019=CARTESIAN_POINT('Ctrl Pts',(-35.6555077526845,51.562500006828,-35.6555077526845));
#6020=CARTESIAN_POINT('Ctrl Pts',(-24.3531646875,51.3541666734946,-42.1809185638423));
#6021=CARTESIAN_POINT('Ctrl Pts',(-13.0508216223155,51.1458333401613,-48.706329375));
#6022=CARTESIAN_POINT('Ctrl Pts',(1.59157945007855E-14,50.937500006828,
-48.706329375));
#6023=CARTESIAN_POINT('Ctrl Pts',(13.0508216223155,50.7291666734946,-48.706329375));
#6024=CARTESIAN_POINT('Ctrl Pts',(24.3531646875,50.5208333401613,-42.1809185638422));
#6025=CARTESIAN_POINT('Ctrl Pts',(35.6555077526845,50.312500006828,-35.6555077526845));
#6026=CARTESIAN_POINT('Ctrl Pts',(42.1809185638422,50.1041666734946,-24.3531646875));
#6027=CARTESIAN_POINT('Ctrl Pts',(48.706329375,49.8958333401613,-13.0508216223155));
#6028=CARTESIAN_POINT('Ctrl Pts',(48.706329375,49.687500006828,1.293339198242E-14));
#6029=CARTESIAN_POINT('Ctrl Pts',(48.706329375,49.4791666734946,13.0508216223155));
#6030=CARTESIAN_POINT('Ctrl Pts',(42.1809185638422,49.2708333401613,24.3531646875));
#6031=CARTESIAN_POINT('Ctrl Pts',(35.6555077526845,49.062500006828,35.6555077526845));
#6032=CARTESIAN_POINT('Ctrl Pts',(24.3531646875,48.8541666734946,42.1809185638422));
#6033=CARTESIAN_POINT('Ctrl Pts',(13.0508216223155,48.6458333401613,48.706329375));
#6034=CARTESIAN_POINT('Ctrl Pts',(-9.95098946405443E-15,48.437500006828,
48.706329375));
#6035=CARTESIAN_POINT('Ctrl Pts',(-13.0508216223155,48.2291666734946,48.706329375));
#6036=CARTESIAN_POINT('Ctrl Pts',(-24.3531646875,48.0208333401613,42.1809185638423));
#6037=CARTESIAN_POINT('Ctrl Pts',(-35.6555077526845,47.812500006828,35.6555077526845));
#6038=CARTESIAN_POINT('Ctrl Pts',(-42.1809185638422,47.6041666734946,24.3531646875));
#6039=CARTESIAN_POINT('Ctrl Pts',(-48.706329375,47.3958333401613,13.0508216223155));
#6040=CARTESIAN_POINT('Ctrl Pts',(-48.706329375,47.187500006828,-1.8898197019151E-14));
#6041=CARTESIAN_POINT('Ctrl Pts',(-48.706329375,46.9791666734946,-13.0508216223155));
#6042=CARTESIAN_POINT('Ctrl Pts',(-42.1809185638422,46.7708333401613,-24.3531646875));
#6043=CARTESIAN_POINT('Ctrl Pts',(-35.6555077526845,46.562500006828,-35.6555077526845));
#6044=CARTESIAN_POINT('Ctrl Pts',(-24.3531646875,46.3541666734946,-42.1809185638423));
#6045=CARTESIAN_POINT('Ctrl Pts',(-13.0508216223155,46.1458333401613,-48.706329375));
#6046=CARTESIAN_POINT('Ctrl Pts',(1.59157945007855E-14,45.937500006828,
-48.706329375));
#6047=CARTESIAN_POINT('Ctrl Pts',(13.0508216223155,45.7291666734946,-48.706329375));
#6048=CARTESIAN_POINT('Ctrl Pts',(24.3531646875,45.5208333401613,-42.1809185638422));
#6049=CARTESIAN_POINT('Ctrl Pts',(35.6555077526845,45.312500006828,-35.6555077526845));
#6050=CARTESIAN_POINT('Ctrl Pts',(42.1809185638422,45.1041666734946,-24.3531646875));
#6051=CARTESIAN_POINT('Ctrl Pts',(48.706329375,44.8958333401613,-13.0508216223155));
#6052=CARTESIAN_POINT('Ctrl Pts',(48.706329375,44.687500006828,1.293339198242E-14));
#6053=CARTESIAN_POINT('Ctrl Pts',(48.706329375,44.4791666734946,13.0508216223155));
#6054=CARTESIAN_POINT('Ctrl Pts',(42.1809185638422,44.2708333401613,24.3531646875));
#6055=CARTESIAN_POINT('Ctrl Pts',(35.6555077526845,44.062500006828,35.6555077526845));
#6056=CARTESIAN_POINT('Ctrl Pts',(24.3531646875,43.8541666734946,42.1809185638422));
#6057=CARTESIAN_POINT('Ctrl Pts',(13.0508216223155,43.6458333401613,48.706329375));
#6058=CARTESIAN_POINT('Ctrl Pts',(-9.95098946405443E-15,43.437500006828,
48.706329375));
#6059=CARTESIAN_POINT('Ctrl Pts',(-13.0508216223155,43.2291666734946,48.706329375));
#6060=CARTESIAN_POINT('Ctrl Pts',(-24.3531646875,43.0208333401613,42.1809185638423));
#6061=CARTESIAN_POINT('Ctrl Pts',(-35.6555077526845,42.812500006828,35.6555077526845));
#6062=CARTESIAN_POINT('Ctrl Pts',(-42.1809185638422,42.6041666734946,24.3531646875));
#6063=CARTESIAN_POINT('Ctrl Pts',(-48.706329375,42.3958333401613,13.0508216223155));
#6064=CARTESIAN_POINT('Ctrl Pts',(-48.706329375,42.187500006828,-1.8898197019151E-14));
#6065=CARTESIAN_POINT('Ctrl Pts',(-48.706329375,41.9791666734946,-13.0508216223155));
#6066=CARTESIAN_POINT('Ctrl Pts',(-42.1809185638422,41.7708333401613,-24.3531646875));
#6067=CARTESIAN_POINT('Ctrl Pts',(-35.6555077526845,41.562500006828,-35.6555077526845));
#6068=CARTESIAN_POINT('Ctrl Pts',(-24.3531646875,41.3541666734946,-42.1809185638423));
#6069=CARTESIAN_POINT('Ctrl Pts',(-13.0508216223155,41.1458333401613,-48.706329375));
#6070=CARTESIAN_POINT('Ctrl Pts',(1.59157945007855E-14,40.937500006828,
-48.706329375));
#6071=CARTESIAN_POINT('Ctrl Pts',(13.0508216223155,40.7291666734946,-48.706329375));
#6072=CARTESIAN_POINT('Ctrl Pts',(24.3531646875,40.5208333401613,-42.1809185638422));
#6073=CARTESIAN_POINT('Ctrl Pts',(35.6555077526845,40.312500006828,-35.6555077526845));
#6074=CARTESIAN_POINT('Ctrl Pts',(42.1809185638422,40.1041666734946,-24.3531646875));
#6075=CARTESIAN_POINT('Ctrl Pts',(48.706329375,39.8958333401613,-13.0508216223155));
#6076=CARTESIAN_POINT('Ctrl Pts',(48.706329375,39.687500006828,1.293339198242E-14));
#6077=CARTESIAN_POINT('Ctrl Pts',(48.706329375,39.4791666734946,13.0508216223155));
#6078=CARTESIAN_POINT('Ctrl Pts',(42.1809185638422,39.2708333401613,24.3531646875));
#6079=CARTESIAN_POINT('Ctrl Pts',(35.6555077526845,39.062500006828,35.6555077526845));
#6080=CARTESIAN_POINT('Ctrl Pts',(24.3531646875,38.8541666734946,42.1809185638422));
#6081=CARTESIAN_POINT('Ctrl Pts',(13.0508216223155,38.6458333401613,48.706329375));
#6082=CARTESIAN_POINT('Ctrl Pts',(-9.95098946405443E-15,38.437500006828,
48.706329375));
#6083=CARTESIAN_POINT('Ctrl Pts',(-13.0508216223155,38.2291666734946,48.706329375));
#6084=CARTESIAN_POINT('Ctrl Pts',(-24.3531646875,38.0208333401613,42.1809185638423));
#6085=CARTESIAN_POINT('Ctrl Pts',(-35.6555077526845,37.812500006828,35.6555077526845));
#6086=CARTESIAN_POINT('Ctrl Pts',(-42.1809185638422,37.6041666734946,24.3531646875));
#6087=CARTESIAN_POINT('Ctrl Pts',(-48.706329375,37.3958333401613,13.0508216223155));
#6088=CARTESIAN_POINT('Ctrl Pts',(-48.706329375,37.187500006828,-1.8898197019151E-14));
#6089=CARTESIAN_POINT('Ctrl Pts',(-48.706329375,36.9791666734946,-13.0508216223155));
#6090=CARTESIAN_POINT('Ctrl Pts',(-42.1809185638422,36.7708333401613,-24.3531646875));
#6091=CARTESIAN_POINT('Ctrl Pts',(-35.6555077526845,36.562500006828,-35.6555077526845));
#6092=CARTESIAN_POINT('Ctrl Pts',(-24.3531646875,36.3541666734946,-42.1809185638423));
#6093=CARTESIAN_POINT('Ctrl Pts',(-13.0508216223155,36.1458333401613,-48.706329375));
#6094=CARTESIAN_POINT('Ctrl Pts',(1.59157945007855E-14,35.937500006828,
-48.706329375));
#6095=CARTESIAN_POINT('Ctrl Pts',(13.0508216223155,35.7291666734946,-48.706329375));
#6096=CARTESIAN_POINT('Ctrl Pts',(24.3531646875,35.5208333401613,-42.1809185638422));
#6097=CARTESIAN_POINT('Ctrl Pts',(35.6555077526845,35.312500006828,-35.6555077526845));
#6098=CARTESIAN_POINT('Ctrl Pts',(42.1809185638422,35.1041666734946,-24.3531646875));
#6099=CARTESIAN_POINT('Ctrl Pts',(48.706329375,34.8958333401613,-13.0508216223155));
#6100=CARTESIAN_POINT('Ctrl Pts',(48.706329375,34.687500006828,1.293339198242E-14));
#6101=CARTESIAN_POINT('Ctrl Pts',(48.706329375,34.4791666734946,13.0508216223155));
#6102=CARTESIAN_POINT('Ctrl Pts',(42.1809185638422,34.2708333401613,24.3531646875));
#6103=CARTESIAN_POINT('Ctrl Pts',(35.6555077526845,34.062500006828,35.6555077526845));
#6104=CARTESIAN_POINT('Ctrl Pts',(24.3531646875,33.8541666734946,42.1809185638422));
#6105=CARTESIAN_POINT('Ctrl Pts',(13.0508216223155,33.6458333401613,48.706329375));
#6106=CARTESIAN_POINT('Ctrl Pts',(-9.95098946405443E-15,33.437500006828,
48.706329375));
#6107=CARTESIAN_POINT('Ctrl Pts',(-13.0508216223155,33.2291666734946,48.706329375));
#6108=CARTESIAN_POINT('Ctrl Pts',(-24.3531646875,33.0208333401613,42.1809185638423));
#6109=CARTESIAN_POINT('Ctrl Pts',(-35.6555077526845,32.812500006828,35.6555077526845));
#6110=CARTESIAN_POINT('Ctrl Pts',(-42.1809185638422,32.6041666734946,24.3531646875));
#6111=CARTESIAN_POINT('Ctrl Pts',(-48.706329375,32.3958333401613,13.0508216223155));
#6112=CARTESIAN_POINT('Ctrl Pts',(-48.706329375,32.187500006828,-1.8898197019151E-14));
#6113=CARTESIAN_POINT('Ctrl Pts',(-48.706329375,31.9791666734946,-13.0508216223155));
#6114=CARTESIAN_POINT('Ctrl Pts',(-42.1809185638422,31.7708333401613,-24.3531646875));
#6115=CARTESIAN_POINT('Ctrl Pts',(-35.6555077526845,31.562500006828,-35.6555077526845));
#6116=CARTESIAN_POINT('Ctrl Pts',(-24.3531646875,31.3541666734946,-42.1809185638423));
#6117=CARTESIAN_POINT('Ctrl Pts',(-13.0508216223155,31.1458333401613,-48.706329375));
#6118=CARTESIAN_POINT('Ctrl Pts',(1.59157945007855E-14,30.937500006828,
-48.706329375));
#6119=CARTESIAN_POINT('Ctrl Pts',(13.0508216223155,30.7291666734946,-48.706329375));
#6120=CARTESIAN_POINT('Ctrl Pts',(24.3531646875,30.5208333401613,-42.1809185638422));
#6121=CARTESIAN_POINT('Ctrl Pts',(35.6555077526845,30.312500006828,-35.6555077526845));
#6122=CARTESIAN_POINT('Ctrl Pts',(42.1809185638422,30.1041666734946,-24.3531646875));
#6123=CARTESIAN_POINT('Ctrl Pts',(48.706329375,29.8958333401613,-13.0508216223155));
#6124=CARTESIAN_POINT('Ctrl Pts',(48.706329375,29.687500006828,1.293339198242E-14));
#6125=CARTESIAN_POINT('Ctrl Pts',(48.706329375,29.4791666734946,13.0508216223155));
#6126=CARTESIAN_POINT('Ctrl Pts',(42.1809185638422,29.2708333401613,24.3531646875));
#6127=CARTESIAN_POINT('Ctrl Pts',(35.6555077526845,29.062500006828,35.6555077526845));
#6128=CARTESIAN_POINT('Ctrl Pts',(24.3531646875,28.8541666734946,42.1809185638422));
#6129=CARTESIAN_POINT('Ctrl Pts',(13.0508216223155,28.6458333401613,48.706329375));
#6130=CARTESIAN_POINT('Ctrl Pts',(-9.95098946405443E-15,28.437500006828,
48.706329375));
#6131=CARTESIAN_POINT('Ctrl Pts',(-13.0508216223155,28.2291666734946,48.706329375));
#6132=CARTESIAN_POINT('Ctrl Pts',(-24.3531646875,28.0208333401613,42.1809185638423));
#6133=CARTESIAN_POINT('Ctrl Pts',(-35.6555077526845,27.812500006828,35.6555077526845));
#6134=CARTESIAN_POINT('Ctrl Pts',(-42.1809185638422,27.6041666734946,24.3531646875));
#6135=CARTESIAN_POINT('Ctrl Pts',(-48.706329375,27.3958333401613,13.0508216223155));
#6136=CARTESIAN_POINT('Ctrl Pts',(-48.706329375,27.187500006828,-1.8898197019151E-14));
#6137=CARTESIAN_POINT('',(48.5725845633798,54.6293483229262,3.60701400320328));
#6138=CARTESIAN_POINT('Ctrl Pts',(45.858362923034,53.0633913333999,3.60701400320327));
#6139=CARTESIAN_POINT('Ctrl Pts',(46.089925771934,53.1969849680263,3.60701400320327));
#6140=CARTESIAN_POINT('Ctrl Pts',(46.5530501979845,53.4641744416604,3.60701400320329));
#6141=CARTESIAN_POINT('Ctrl Pts',(47.0161721905706,53.7313681332063,3.60701400320326));
#6142=CARTESIAN_POINT('Ctrl Pts',(47.689351986232,54.1197565257476,3.60701400320326));
#6143=CARTESIAN_POINT('Ctrl Pts',(48.1309692507095,54.3745507329179,3.60701400320328));
#6144=CARTESIAN_POINT('Ctrl Pts',(48.5725845633798,54.6293483229262,3.60701400320328));
#6145=CARTESIAN_POINT('',(3.612927284338,53.4957479656467,48.5721450795008));
#6146=CARTESIAN_POINT('Ctrl Pts',(48.5725845633798,54.6293483229262,3.60701400320328));
#6147=CARTESIAN_POINT('Ctrl Pts',(47.7480251419552,54.4485714020251,14.7106532430575));
#6148=CARTESIAN_POINT('Ctrl Pts',(42.1809185638422,54.2708333401613,24.3531646875));
#6149=CARTESIAN_POINT('Ctrl Pts',(35.6555077526845,54.062500006828,35.6555077526845));
#6150=CARTESIAN_POINT('Ctrl Pts',(24.3531646875,53.8541666734946,42.1809185638422));
#6151=CARTESIAN_POINT('Ctrl Pts',(14.7133549689477,53.6764784118853,47.7464652997852));
#6152=CARTESIAN_POINT('Ctrl Pts',(3.612927284338,53.4957479656467,48.5721450795008));
#6153=CARTESIAN_POINT('Ctrl Pts',(3.612927284338,53.4957479656467,48.5721450795008));
#6154=CARTESIAN_POINT('Ctrl Pts',(3.612927284338,53.3625660950884,48.3403451622817));
#6155=CARTESIAN_POINT('Ctrl Pts',(3.612927284338,53.2293911846469,48.1085412459393));
#6156=CARTESIAN_POINT('Ctrl Pts',(3.612927284338,52.9630558994543,47.6449250631479));
#6157=CARTESIAN_POINT('Ctrl Pts',(3.61292728433799,52.8298955244832,47.4131127965212));
#6158=CARTESIAN_POINT('Ctrl Pts',(3.61292728433799,52.6967427432646,47.1812961682826));
#6159=CARTESIAN_POINT('Ctrl Pts',(3.61292728433799,52.4433704509922,46.7401795055578));
#6160=CARTESIAN_POINT('Ctrl Pts',(3.612927284338,52.1900256371662,46.2990470581854));
#6161=CARTESIAN_POINT('Ctrl Pts',(3.612927284338,51.936710750803,45.8578974271399));
#6162=CARTESIAN_POINT('Ctrl Pts',(-46.,55.6250000136559,0.));
#6163=CARTESIAN_POINT('Ctrl Pts',(-46.,55.4166666803226,-12.3256628518316));
#6164=CARTESIAN_POINT('Ctrl Pts',(-39.8371685740842,55.2083333469893,-23.));
#6165=CARTESIAN_POINT('Ctrl Pts',(-33.6743371481684,55.0000000136559,-33.6743371481684));
#6166=CARTESIAN_POINT('Ctrl Pts',(-23.,54.7916666803226,-39.8371685740842));
#6167=CARTESIAN_POINT('Ctrl Pts',(-12.3256628518317,54.5833333469893,-46.));
#6168=CARTESIAN_POINT('Ctrl Pts',(-2.81668763803891E-15,54.3750000136559,
-46.));
#6169=CARTESIAN_POINT('Ctrl Pts',(12.3256628518316,54.1666666803226,-46.));
#6170=CARTESIAN_POINT('Ctrl Pts',(23.,53.9583333469893,-39.8371685740842));
#6171=CARTESIAN_POINT('Ctrl Pts',(33.6743371481683,53.7500000136559,-33.6743371481684));
#6172=CARTESIAN_POINT('Ctrl Pts',(39.8371685740842,53.5416666803226,-23.));
#6173=CARTESIAN_POINT('Ctrl Pts',(46.,53.3333333469893,-12.3256628518317));
#6174=CARTESIAN_POINT('Ctrl Pts',(46.,53.1250000136559,-5.63337527607782E-15));
#6175=CARTESIAN_POINT('Ctrl Pts',(46.,52.9166666803226,12.3256628518316));
#6176=CARTESIAN_POINT('Ctrl Pts',(39.8371685740842,52.7083333469893,23.));
#6177=CARTESIAN_POINT('Ctrl Pts',(33.6743371481684,52.5000000136559,33.6743371481683));
#6178=CARTESIAN_POINT('Ctrl Pts',(23.,52.2916666803226,39.8371685740842));
#6179=CARTESIAN_POINT('Ctrl Pts',(12.3256628518317,52.0833333469893,46.));
#6180=CARTESIAN_POINT('Ctrl Pts',(8.45006291411674E-15,51.8750000136559,
46.));
#6181=CARTESIAN_POINT('Ctrl Pts',(-12.3256628518316,51.6666666803226,46.));
#6182=CARTESIAN_POINT('Ctrl Pts',(-23.,51.4583333469893,39.8371685740842));
#6183=CARTESIAN_POINT('Ctrl Pts',(-33.6743371481683,51.2500000136559,33.6743371481684));
#6184=CARTESIAN_POINT('Ctrl Pts',(-39.8371685740842,51.0416666803226,23.));
#6185=CARTESIAN_POINT('Ctrl Pts',(-46.,50.8333333469893,12.3256628518317));
#6186=CARTESIAN_POINT('Ctrl Pts',(-46.,50.6250000136559,0.));
#6187=CARTESIAN_POINT('Ctrl Pts',(-46.,50.4166666803226,-12.3256628518316));
#6188=CARTESIAN_POINT('Ctrl Pts',(-39.8371685740842,50.2083333469893,-23.));
#6189=CARTESIAN_POINT('Ctrl Pts',(-33.6743371481684,50.0000000136559,-33.6743371481684));
#6190=CARTESIAN_POINT('Ctrl Pts',(-23.,49.7916666803226,-39.8371685740842));
#6191=CARTESIAN_POINT('Ctrl Pts',(-12.3256628518317,49.5833333469893,-46.));
#6192=CARTESIAN_POINT('Ctrl Pts',(-2.81668763803891E-15,49.3750000136559,
-46.));
#6193=CARTESIAN_POINT('Ctrl Pts',(12.3256628518316,49.1666666803226,-46.));
#6194=CARTESIAN_POINT('Ctrl Pts',(23.,48.9583333469893,-39.8371685740842));
#6195=CARTESIAN_POINT('Ctrl Pts',(33.6743371481683,48.7500000136559,-33.6743371481684));
#6196=CARTESIAN_POINT('Ctrl Pts',(39.8371685740842,48.5416666803226,-23.));
#6197=CARTESIAN_POINT('Ctrl Pts',(46.,48.3333333469893,-12.3256628518317));
#6198=CARTESIAN_POINT('Ctrl Pts',(46.,48.1250000136559,-5.63337527607782E-15));
#6199=CARTESIAN_POINT('Ctrl Pts',(46.,47.9166666803226,12.3256628518316));
#6200=CARTESIAN_POINT('Ctrl Pts',(39.8371685740842,47.7083333469893,23.));
#6201=CARTESIAN_POINT('Ctrl Pts',(33.6743371481684,47.5000000136559,33.6743371481683));
#6202=CARTESIAN_POINT('Ctrl Pts',(23.,47.2916666803226,39.8371685740842));
#6203=CARTESIAN_POINT('Ctrl Pts',(12.3256628518317,47.0833333469893,46.));
#6204=CARTESIAN_POINT('Ctrl Pts',(8.45006291411674E-15,46.8750000136559,
46.));
#6205=CARTESIAN_POINT('Ctrl Pts',(-12.3256628518316,46.6666666803226,46.));
#6206=CARTESIAN_POINT('Ctrl Pts',(-23.,46.4583333469893,39.8371685740842));
#6207=CARTESIAN_POINT('Ctrl Pts',(-33.6743371481683,46.2500000136559,33.6743371481684));
#6208=CARTESIAN_POINT('Ctrl Pts',(-39.8371685740842,46.0416666803226,23.));
#6209=CARTESIAN_POINT('Ctrl Pts',(-46.,45.8333333469892,12.3256628518317));
#6210=CARTESIAN_POINT('Ctrl Pts',(-46.,45.6250000136559,0.));
#6211=CARTESIAN_POINT('Ctrl Pts',(-46.,45.4166666803226,-12.3256628518316));
#6212=CARTESIAN_POINT('Ctrl Pts',(-39.8371685740842,45.2083333469893,-23.));
#6213=CARTESIAN_POINT('Ctrl Pts',(-33.6743371481684,45.0000000136559,-33.6743371481684));
#6214=CARTESIAN_POINT('Ctrl Pts',(-23.,44.7916666803226,-39.8371685740842));
#6215=CARTESIAN_POINT('Ctrl Pts',(-12.3256628518317,44.5833333469893,-46.));
#6216=CARTESIAN_POINT('Ctrl Pts',(-2.81668763803891E-15,44.3750000136559,
-46.));
#6217=CARTESIAN_POINT('Ctrl Pts',(12.3256628518316,44.1666666803226,-46.));
#6218=CARTESIAN_POINT('Ctrl Pts',(23.,43.9583333469893,-39.8371685740842));
#6219=CARTESIAN_POINT('Ctrl Pts',(33.6743371481683,43.7500000136559,-33.6743371481684));
#6220=CARTESIAN_POINT('Ctrl Pts',(39.8371685740842,43.5416666803226,-23.));
#6221=CARTESIAN_POINT('Ctrl Pts',(46.,43.3333333469893,-12.3256628518317));
#6222=CARTESIAN_POINT('Ctrl Pts',(46.,43.1250000136559,-5.63337527607782E-15));
#6223=CARTESIAN_POINT('Ctrl Pts',(46.,42.9166666803226,12.3256628518316));
#6224=CARTESIAN_POINT('Ctrl Pts',(39.8371685740842,42.7083333469893,23.));
#6225=CARTESIAN_POINT('Ctrl Pts',(33.6743371481684,42.5000000136559,33.6743371481683));
#6226=CARTESIAN_POINT('Ctrl Pts',(23.,42.2916666803226,39.8371685740842));
#6227=CARTESIAN_POINT('Ctrl Pts',(12.3256628518317,42.0833333469893,46.));
#6228=CARTESIAN_POINT('Ctrl Pts',(8.45006291411674E-15,41.8750000136559,
46.));
#6229=CARTESIAN_POINT('Ctrl Pts',(-12.3256628518316,41.6666666803226,46.));
#6230=CARTESIAN_POINT('Ctrl Pts',(-23.,41.4583333469893,39.8371685740842));
#6231=CARTESIAN_POINT('Ctrl Pts',(-33.6743371481683,41.2500000136559,33.6743371481684));
#6232=CARTESIAN_POINT('Ctrl Pts',(-39.8371685740842,41.0416666803226,23.));
#6233=CARTESIAN_POINT('Ctrl Pts',(-46.,40.8333333469893,12.3256628518317));
#6234=CARTESIAN_POINT('Ctrl Pts',(-46.,40.6250000136559,0.));
#6235=CARTESIAN_POINT('Ctrl Pts',(-46.,40.4166666803226,-12.3256628518316));
#6236=CARTESIAN_POINT('Ctrl Pts',(-39.8371685740842,40.2083333469893,-23.));
#6237=CARTESIAN_POINT('Ctrl Pts',(-33.6743371481684,40.0000000136559,-33.6743371481684));
#6238=CARTESIAN_POINT('Ctrl Pts',(-23.,39.7916666803226,-39.8371685740842));
#6239=CARTESIAN_POINT('Ctrl Pts',(-12.3256628518317,39.5833333469893,-46.));
#6240=CARTESIAN_POINT('Ctrl Pts',(-2.81668763803891E-15,39.3750000136559,
-46.));
#6241=CARTESIAN_POINT('Ctrl Pts',(12.3256628518316,39.1666666803226,-46.));
#6242=CARTESIAN_POINT('Ctrl Pts',(23.,38.9583333469893,-39.8371685740842));
#6243=CARTESIAN_POINT('Ctrl Pts',(33.6743371481683,38.7500000136559,-33.6743371481684));
#6244=CARTESIAN_POINT('Ctrl Pts',(39.8371685740842,38.5416666803226,-23.));
#6245=CARTESIAN_POINT('Ctrl Pts',(46.,38.3333333469893,-12.3256628518317));
#6246=CARTESIAN_POINT('Ctrl Pts',(46.,38.1250000136559,-5.63337527607782E-15));
#6247=CARTESIAN_POINT('Ctrl Pts',(46.,37.9166666803226,12.3256628518316));
#6248=CARTESIAN_POINT('Ctrl Pts',(39.8371685740842,37.7083333469893,23.));
#6249=CARTESIAN_POINT('Ctrl Pts',(33.6743371481684,37.5000000136559,33.6743371481683));
#6250=CARTESIAN_POINT('Ctrl Pts',(23.,37.2916666803226,39.8371685740842));
#6251=CARTESIAN_POINT('Ctrl Pts',(12.3256628518317,37.0833333469893,46.));
#6252=CARTESIAN_POINT('Ctrl Pts',(8.45006291411674E-15,36.8750000136559,
46.));
#6253=CARTESIAN_POINT('Ctrl Pts',(-12.3256628518316,36.6666666803226,46.));
#6254=CARTESIAN_POINT('Ctrl Pts',(-23.,36.4583333469893,39.8371685740842));
#6255=CARTESIAN_POINT('Ctrl Pts',(-33.6743371481683,36.2500000136559,33.6743371481684));
#6256=CARTESIAN_POINT('Ctrl Pts',(-39.8371685740842,36.0416666803226,23.));
#6257=CARTESIAN_POINT('Ctrl Pts',(-46.,35.8333333469893,12.3256628518317));
#6258=CARTESIAN_POINT('Ctrl Pts',(-46.,35.6250000136559,0.));
#6259=CARTESIAN_POINT('Ctrl Pts',(-46.,35.4166666803226,-12.3256628518316));
#6260=CARTESIAN_POINT('Ctrl Pts',(-39.8371685740842,35.2083333469893,-23.));
#6261=CARTESIAN_POINT('Ctrl Pts',(-33.6743371481684,35.0000000136559,-33.6743371481684));
#6262=CARTESIAN_POINT('Ctrl Pts',(-23.,34.7916666803226,-39.8371685740842));
#6263=CARTESIAN_POINT('Ctrl Pts',(-12.3256628518317,34.5833333469893,-46.));
#6264=CARTESIAN_POINT('Ctrl Pts',(-2.81668763803891E-15,34.3750000136559,
-46.));
#6265=CARTESIAN_POINT('Ctrl Pts',(12.3256628518316,34.1666666803226,-46.));
#6266=CARTESIAN_POINT('Ctrl Pts',(23.,33.9583333469893,-39.8371685740842));
#6267=CARTESIAN_POINT('Ctrl Pts',(33.6743371481683,33.7500000136559,-33.6743371481684));
#6268=CARTESIAN_POINT('Ctrl Pts',(39.8371685740842,33.5416666803226,-23.));
#6269=CARTESIAN_POINT('Ctrl Pts',(46.,33.3333333469893,-12.3256628518317));
#6270=CARTESIAN_POINT('Ctrl Pts',(46.,33.1250000136559,-5.63337527607782E-15));
#6271=CARTESIAN_POINT('Ctrl Pts',(46.,32.9166666803226,12.3256628518316));
#6272=CARTESIAN_POINT('Ctrl Pts',(39.8371685740842,32.7083333469893,23.));
#6273=CARTESIAN_POINT('Ctrl Pts',(33.6743371481684,32.5000000136559,33.6743371481683));
#6274=CARTESIAN_POINT('Ctrl Pts',(23.,32.2916666803226,39.8371685740842));
#6275=CARTESIAN_POINT('Ctrl Pts',(12.3256628518317,32.0833333469893,46.));
#6276=CARTESIAN_POINT('Ctrl Pts',(8.45006291411674E-15,31.8750000136559,
46.));
#6277=CARTESIAN_POINT('Ctrl Pts',(-12.3256628518316,31.6666666803226,46.));
#6278=CARTESIAN_POINT('Ctrl Pts',(-23.,31.4583333469893,39.8371685740842));
#6279=CARTESIAN_POINT('Ctrl Pts',(-33.6743371481683,31.2500000136559,33.6743371481684));
#6280=CARTESIAN_POINT('Ctrl Pts',(-39.8371685740842,31.0416666803226,23.));
#6281=CARTESIAN_POINT('Ctrl Pts',(-46.,30.8333333469893,12.3256628518317));
#6282=CARTESIAN_POINT('Ctrl Pts',(-46.,30.6250000136559,0.));
#6283=CARTESIAN_POINT('Ctrl Pts',(-46.,30.4166666803226,-12.3256628518316));
#6284=CARTESIAN_POINT('Ctrl Pts',(-39.8371685740842,30.2083333469893,-23.));
#6285=CARTESIAN_POINT('Ctrl Pts',(-33.6743371481684,30.0000000136559,-33.6743371481684));
#6286=CARTESIAN_POINT('Ctrl Pts',(-23.,29.7916666803226,-39.8371685740842));
#6287=CARTESIAN_POINT('Ctrl Pts',(-12.3256628518317,29.5833333469893,-46.));
#6288=CARTESIAN_POINT('Ctrl Pts',(-2.81668763803891E-15,29.3750000136559,
-46.));
#6289=CARTESIAN_POINT('Ctrl Pts',(12.3256628518316,29.1666666803226,-46.));
#6290=CARTESIAN_POINT('Ctrl Pts',(23.,28.9583333469893,-39.8371685740842));
#6291=CARTESIAN_POINT('Ctrl Pts',(33.6743371481683,28.7500000136559,-33.6743371481684));
#6292=CARTESIAN_POINT('Ctrl Pts',(39.8371685740842,28.5416666803226,-23.));
#6293=CARTESIAN_POINT('Ctrl Pts',(46.,28.3333333469893,-12.3256628518317));
#6294=CARTESIAN_POINT('Ctrl Pts',(46.,28.1250000136559,-5.63337527607782E-15));
#6295=CARTESIAN_POINT('Ctrl Pts',(46.,27.9166666803226,12.3256628518316));
#6296=CARTESIAN_POINT('Ctrl Pts',(39.8371685740842,27.7083333469893,23.));
#6297=CARTESIAN_POINT('Ctrl Pts',(33.6743371481684,27.5000000136559,33.6743371481683));
#6298=CARTESIAN_POINT('Ctrl Pts',(23.,27.2916666803226,39.8371685740842));
#6299=CARTESIAN_POINT('Ctrl Pts',(12.3256628518317,27.0833333469893,46.));
#6300=CARTESIAN_POINT('Ctrl Pts',(8.45006291411674E-15,26.8750000136559,
46.));
#6301=CARTESIAN_POINT('Ctrl Pts',(-12.3256628518316,26.6666666803226,46.));
#6302=CARTESIAN_POINT('Ctrl Pts',(-23.,26.4583333469893,39.8371685740842));
#6303=CARTESIAN_POINT('Ctrl Pts',(-33.6743371481683,26.2500000136559,33.6743371481684));
#6304=CARTESIAN_POINT('Ctrl Pts',(-39.8371685740842,26.0416666803226,23.));
#6305=CARTESIAN_POINT('Ctrl Pts',(-46.,25.8333333469893,12.3256628518317));
#6306=CARTESIAN_POINT('Ctrl Pts',(-46.,25.6250000136559,0.));
#6307=CARTESIAN_POINT('Ctrl Pts',(-48.706329375,57.187500006828,-1.8898197019151E-14));
#6308=CARTESIAN_POINT('Ctrl Pts',(-48.706329375,56.9791666734946,-13.0508216223155));
#6309=CARTESIAN_POINT('Ctrl Pts',(-42.1809185638422,56.7708333401613,-24.3531646875));
#6310=CARTESIAN_POINT('Ctrl Pts',(-35.6555077526845,56.562500006828,-35.6555077526845));
#6311=CARTESIAN_POINT('Ctrl Pts',(-24.3531646875,56.3541666734946,-42.1809185638423));
#6312=CARTESIAN_POINT('Ctrl Pts',(-13.0508216223155,56.1458333401613,-48.706329375));
#6313=CARTESIAN_POINT('Ctrl Pts',(1.59157945007855E-14,55.937500006828,
-48.706329375));
#6314=CARTESIAN_POINT('Ctrl Pts',(13.0508216223155,55.7291666734946,-48.706329375));
#6315=CARTESIAN_POINT('Ctrl Pts',(24.3531646875,55.5208333401613,-42.1809185638422));
#6316=CARTESIAN_POINT('Ctrl Pts',(35.6555077526845,55.312500006828,-35.6555077526845));
#6317=CARTESIAN_POINT('Ctrl Pts',(42.1809185638422,55.1041666734946,-24.3531646875));
#6318=CARTESIAN_POINT('Ctrl Pts',(48.706329375,54.8958333401613,-13.0508216223155));
#6319=CARTESIAN_POINT('Ctrl Pts',(48.706329375,54.687500006828,1.293339198242E-14));
#6320=CARTESIAN_POINT('Ctrl Pts',(48.706329375,54.4791666734946,13.0508216223155));
#6321=CARTESIAN_POINT('Ctrl Pts',(42.1809185638422,54.2708333401613,24.3531646875));
#6322=CARTESIAN_POINT('Ctrl Pts',(35.6555077526845,54.062500006828,35.6555077526845));
#6323=CARTESIAN_POINT('Ctrl Pts',(24.3531646875,53.8541666734946,42.1809185638422));
#6324=CARTESIAN_POINT('Ctrl Pts',(13.0508216223155,53.6458333401613,48.706329375));
#6325=CARTESIAN_POINT('Ctrl Pts',(-9.95098946405443E-15,53.437500006828,
48.706329375));
#6326=CARTESIAN_POINT('Ctrl Pts',(-13.0508216223155,53.2291666734946,48.706329375));
#6327=CARTESIAN_POINT('Ctrl Pts',(-24.3531646875,53.0208333401613,42.1809185638423));
#6328=CARTESIAN_POINT('Ctrl Pts',(-35.6555077526845,52.812500006828,35.6555077526845));
#6329=CARTESIAN_POINT('Ctrl Pts',(-42.1809185638422,52.6041666734946,24.3531646875));
#6330=CARTESIAN_POINT('Ctrl Pts',(-48.706329375,52.3958333401613,13.0508216223155));
#6331=CARTESIAN_POINT('Ctrl Pts',(-48.706329375,52.187500006828,-1.8898197019151E-14));
#6332=CARTESIAN_POINT('Ctrl Pts',(-48.706329375,51.9791666734946,-13.0508216223155));
#6333=CARTESIAN_POINT('Ctrl Pts',(-42.1809185638422,51.7708333401613,-24.3531646875));
#6334=CARTESIAN_POINT('Ctrl Pts',(-35.6555077526845,51.562500006828,-35.6555077526845));
#6335=CARTESIAN_POINT('Ctrl Pts',(-24.3531646875,51.3541666734946,-42.1809185638423));
#6336=CARTESIAN_POINT('Ctrl Pts',(-13.0508216223155,51.1458333401613,-48.706329375));
#6337=CARTESIAN_POINT('Ctrl Pts',(1.59157945007855E-14,50.937500006828,
-48.706329375));
#6338=CARTESIAN_POINT('Ctrl Pts',(13.0508216223155,50.7291666734946,-48.706329375));
#6339=CARTESIAN_POINT('Ctrl Pts',(24.3531646875,50.5208333401613,-42.1809185638422));
#6340=CARTESIAN_POINT('Ctrl Pts',(35.6555077526845,50.312500006828,-35.6555077526845));
#6341=CARTESIAN_POINT('Ctrl Pts',(42.1809185638422,50.1041666734946,-24.3531646875));
#6342=CARTESIAN_POINT('Ctrl Pts',(48.706329375,49.8958333401613,-13.0508216223155));
#6343=CARTESIAN_POINT('Ctrl Pts',(48.706329375,49.687500006828,1.293339198242E-14));
#6344=CARTESIAN_POINT('Ctrl Pts',(48.706329375,49.4791666734946,13.0508216223155));
#6345=CARTESIAN_POINT('Ctrl Pts',(42.1809185638422,49.2708333401613,24.3531646875));
#6346=CARTESIAN_POINT('Ctrl Pts',(35.6555077526845,49.062500006828,35.6555077526845));
#6347=CARTESIAN_POINT('Ctrl Pts',(24.3531646875,48.8541666734946,42.1809185638422));
#6348=CARTESIAN_POINT('Ctrl Pts',(13.0508216223155,48.6458333401613,48.706329375));
#6349=CARTESIAN_POINT('Ctrl Pts',(-9.95098946405443E-15,48.437500006828,
48.706329375));
#6350=CARTESIAN_POINT('Ctrl Pts',(-13.0508216223155,48.2291666734946,48.706329375));
#6351=CARTESIAN_POINT('Ctrl Pts',(-24.3531646875,48.0208333401613,42.1809185638423));
#6352=CARTESIAN_POINT('Ctrl Pts',(-35.6555077526845,47.812500006828,35.6555077526845));
#6353=CARTESIAN_POINT('Ctrl Pts',(-42.1809185638422,47.6041666734946,24.3531646875));
#6354=CARTESIAN_POINT('Ctrl Pts',(-48.706329375,47.3958333401613,13.0508216223155));
#6355=CARTESIAN_POINT('Ctrl Pts',(-48.706329375,47.187500006828,-1.8898197019151E-14));
#6356=CARTESIAN_POINT('Ctrl Pts',(-48.706329375,46.9791666734946,-13.0508216223155));
#6357=CARTESIAN_POINT('Ctrl Pts',(-42.1809185638422,46.7708333401613,-24.3531646875));
#6358=CARTESIAN_POINT('Ctrl Pts',(-35.6555077526845,46.562500006828,-35.6555077526845));
#6359=CARTESIAN_POINT('Ctrl Pts',(-24.3531646875,46.3541666734946,-42.1809185638423));
#6360=CARTESIAN_POINT('Ctrl Pts',(-13.0508216223155,46.1458333401613,-48.706329375));
#6361=CARTESIAN_POINT('Ctrl Pts',(1.59157945007855E-14,45.937500006828,
-48.706329375));
#6362=CARTESIAN_POINT('Ctrl Pts',(13.0508216223155,45.7291666734946,-48.706329375));
#6363=CARTESIAN_POINT('Ctrl Pts',(24.3531646875,45.5208333401613,-42.1809185638422));
#6364=CARTESIAN_POINT('Ctrl Pts',(35.6555077526845,45.312500006828,-35.6555077526845));
#6365=CARTESIAN_POINT('Ctrl Pts',(42.1809185638422,45.1041666734946,-24.3531646875));
#6366=CARTESIAN_POINT('Ctrl Pts',(48.706329375,44.8958333401613,-13.0508216223155));
#6367=CARTESIAN_POINT('Ctrl Pts',(48.706329375,44.687500006828,1.293339198242E-14));
#6368=CARTESIAN_POINT('Ctrl Pts',(48.706329375,44.4791666734946,13.0508216223155));
#6369=CARTESIAN_POINT('Ctrl Pts',(42.1809185638422,44.2708333401613,24.3531646875));
#6370=CARTESIAN_POINT('Ctrl Pts',(35.6555077526845,44.062500006828,35.6555077526845));
#6371=CARTESIAN_POINT('Ctrl Pts',(24.3531646875,43.8541666734946,42.1809185638422));
#6372=CARTESIAN_POINT('Ctrl Pts',(13.0508216223155,43.6458333401613,48.706329375));
#6373=CARTESIAN_POINT('Ctrl Pts',(-9.95098946405443E-15,43.437500006828,
48.706329375));
#6374=CARTESIAN_POINT('Ctrl Pts',(-13.0508216223155,43.2291666734946,48.706329375));
#6375=CARTESIAN_POINT('Ctrl Pts',(-24.3531646875,43.0208333401613,42.1809185638423));
#6376=CARTESIAN_POINT('Ctrl Pts',(-35.6555077526845,42.812500006828,35.6555077526845));
#6377=CARTESIAN_POINT('Ctrl Pts',(-42.1809185638422,42.6041666734946,24.3531646875));
#6378=CARTESIAN_POINT('Ctrl Pts',(-48.706329375,42.3958333401613,13.0508216223155));
#6379=CARTESIAN_POINT('Ctrl Pts',(-48.706329375,42.187500006828,-1.8898197019151E-14));
#6380=CARTESIAN_POINT('Ctrl Pts',(-48.706329375,41.9791666734946,-13.0508216223155));
#6381=CARTESIAN_POINT('Ctrl Pts',(-42.1809185638422,41.7708333401613,-24.3531646875));
#6382=CARTESIAN_POINT('Ctrl Pts',(-35.6555077526845,41.562500006828,-35.6555077526845));
#6383=CARTESIAN_POINT('Ctrl Pts',(-24.3531646875,41.3541666734946,-42.1809185638423));
#6384=CARTESIAN_POINT('Ctrl Pts',(-13.0508216223155,41.1458333401613,-48.706329375));
#6385=CARTESIAN_POINT('Ctrl Pts',(1.59157945007855E-14,40.937500006828,
-48.706329375));
#6386=CARTESIAN_POINT('Ctrl Pts',(13.0508216223155,40.7291666734946,-48.706329375));
#6387=CARTESIAN_POINT('Ctrl Pts',(24.3531646875,40.5208333401613,-42.1809185638422));
#6388=CARTESIAN_POINT('Ctrl Pts',(35.6555077526845,40.312500006828,-35.6555077526845));
#6389=CARTESIAN_POINT('Ctrl Pts',(42.1809185638422,40.1041666734946,-24.3531646875));
#6390=CARTESIAN_POINT('Ctrl Pts',(48.706329375,39.8958333401613,-13.0508216223155));
#6391=CARTESIAN_POINT('Ctrl Pts',(48.706329375,39.687500006828,1.293339198242E-14));
#6392=CARTESIAN_POINT('Ctrl Pts',(48.706329375,39.4791666734946,13.0508216223155));
#6393=CARTESIAN_POINT('Ctrl Pts',(42.1809185638422,39.2708333401613,24.3531646875));
#6394=CARTESIAN_POINT('Ctrl Pts',(35.6555077526845,39.062500006828,35.6555077526845));
#6395=CARTESIAN_POINT('Ctrl Pts',(24.3531646875,38.8541666734946,42.1809185638422));
#6396=CARTESIAN_POINT('Ctrl Pts',(13.0508216223155,38.6458333401613,48.706329375));
#6397=CARTESIAN_POINT('Ctrl Pts',(-9.95098946405443E-15,38.437500006828,
48.706329375));
#6398=CARTESIAN_POINT('Ctrl Pts',(-13.0508216223155,38.2291666734946,48.706329375));
#6399=CARTESIAN_POINT('Ctrl Pts',(-24.3531646875,38.0208333401613,42.1809185638423));
#6400=CARTESIAN_POINT('Ctrl Pts',(-35.6555077526845,37.812500006828,35.6555077526845));
#6401=CARTESIAN_POINT('Ctrl Pts',(-42.1809185638422,37.6041666734946,24.3531646875));
#6402=CARTESIAN_POINT('Ctrl Pts',(-48.706329375,37.3958333401613,13.0508216223155));
#6403=CARTESIAN_POINT('Ctrl Pts',(-48.706329375,37.187500006828,-1.8898197019151E-14));
#6404=CARTESIAN_POINT('Ctrl Pts',(-48.706329375,36.9791666734946,-13.0508216223155));
#6405=CARTESIAN_POINT('Ctrl Pts',(-42.1809185638422,36.7708333401613,-24.3531646875));
#6406=CARTESIAN_POINT('Ctrl Pts',(-35.6555077526845,36.562500006828,-35.6555077526845));
#6407=CARTESIAN_POINT('Ctrl Pts',(-24.3531646875,36.3541666734946,-42.1809185638423));
#6408=CARTESIAN_POINT('Ctrl Pts',(-13.0508216223155,36.1458333401613,-48.706329375));
#6409=CARTESIAN_POINT('Ctrl Pts',(1.59157945007855E-14,35.937500006828,
-48.706329375));
#6410=CARTESIAN_POINT('Ctrl Pts',(13.0508216223155,35.7291666734946,-48.706329375));
#6411=CARTESIAN_POINT('Ctrl Pts',(24.3531646875,35.5208333401613,-42.1809185638422));
#6412=CARTESIAN_POINT('Ctrl Pts',(35.6555077526845,35.312500006828,-35.6555077526845));
#6413=CARTESIAN_POINT('Ctrl Pts',(42.1809185638422,35.1041666734946,-24.3531646875));
#6414=CARTESIAN_POINT('Ctrl Pts',(48.706329375,34.8958333401613,-13.0508216223155));
#6415=CARTESIAN_POINT('Ctrl Pts',(48.706329375,34.687500006828,1.293339198242E-14));
#6416=CARTESIAN_POINT('Ctrl Pts',(48.706329375,34.4791666734946,13.0508216223155));
#6417=CARTESIAN_POINT('Ctrl Pts',(42.1809185638422,34.2708333401613,24.3531646875));
#6418=CARTESIAN_POINT('Ctrl Pts',(35.6555077526845,34.062500006828,35.6555077526845));
#6419=CARTESIAN_POINT('Ctrl Pts',(24.3531646875,33.8541666734946,42.1809185638422));
#6420=CARTESIAN_POINT('Ctrl Pts',(13.0508216223155,33.6458333401613,48.706329375));
#6421=CARTESIAN_POINT('Ctrl Pts',(-9.95098946405443E-15,33.437500006828,
48.706329375));
#6422=CARTESIAN_POINT('Ctrl Pts',(-13.0508216223155,33.2291666734946,48.706329375));
#6423=CARTESIAN_POINT('Ctrl Pts',(-24.3531646875,33.0208333401613,42.1809185638423));
#6424=CARTESIAN_POINT('Ctrl Pts',(-35.6555077526845,32.812500006828,35.6555077526845));
#6425=CARTESIAN_POINT('Ctrl Pts',(-42.1809185638422,32.6041666734946,24.3531646875));
#6426=CARTESIAN_POINT('Ctrl Pts',(-48.706329375,32.3958333401613,13.0508216223155));
#6427=CARTESIAN_POINT('Ctrl Pts',(-48.706329375,32.187500006828,-1.8898197019151E-14));
#6428=CARTESIAN_POINT('Ctrl Pts',(-48.706329375,31.9791666734946,-13.0508216223155));
#6429=CARTESIAN_POINT('Ctrl Pts',(-42.1809185638422,31.7708333401613,-24.3531646875));
#6430=CARTESIAN_POINT('Ctrl Pts',(-35.6555077526845,31.562500006828,-35.6555077526845));
#6431=CARTESIAN_POINT('Ctrl Pts',(-24.3531646875,31.3541666734946,-42.1809185638423));
#6432=CARTESIAN_POINT('Ctrl Pts',(-13.0508216223155,31.1458333401613,-48.706329375));
#6433=CARTESIAN_POINT('Ctrl Pts',(1.59157945007855E-14,30.937500006828,
-48.706329375));
#6434=CARTESIAN_POINT('Ctrl Pts',(13.0508216223155,30.7291666734946,-48.706329375));
#6435=CARTESIAN_POINT('Ctrl Pts',(24.3531646875,30.5208333401613,-42.1809185638422));
#6436=CARTESIAN_POINT('Ctrl Pts',(35.6555077526845,30.312500006828,-35.6555077526845));
#6437=CARTESIAN_POINT('Ctrl Pts',(42.1809185638422,30.1041666734946,-24.3531646875));
#6438=CARTESIAN_POINT('Ctrl Pts',(48.706329375,29.8958333401613,-13.0508216223155));
#6439=CARTESIAN_POINT('Ctrl Pts',(48.706329375,29.687500006828,1.293339198242E-14));
#6440=CARTESIAN_POINT('Ctrl Pts',(48.706329375,29.4791666734946,13.0508216223155));
#6441=CARTESIAN_POINT('Ctrl Pts',(42.1809185638422,29.2708333401613,24.3531646875));
#6442=CARTESIAN_POINT('Ctrl Pts',(35.6555077526845,29.062500006828,35.6555077526845));
#6443=CARTESIAN_POINT('Ctrl Pts',(24.3531646875,28.8541666734946,42.1809185638422));
#6444=CARTESIAN_POINT('Ctrl Pts',(13.0508216223155,28.6458333401613,48.706329375));
#6445=CARTESIAN_POINT('Ctrl Pts',(-9.95098946405443E-15,28.437500006828,
48.706329375));
#6446=CARTESIAN_POINT('Ctrl Pts',(-13.0508216223155,28.2291666734946,48.706329375));
#6447=CARTESIAN_POINT('Ctrl Pts',(-24.3531646875,28.0208333401613,42.1809185638423));
#6448=CARTESIAN_POINT('Ctrl Pts',(-35.6555077526845,27.812500006828,35.6555077526845));
#6449=CARTESIAN_POINT('Ctrl Pts',(-42.1809185638422,27.6041666734946,24.3531646875));
#6450=CARTESIAN_POINT('Ctrl Pts',(-48.706329375,27.3958333401613,13.0508216223155));
#6451=CARTESIAN_POINT('Ctrl Pts',(-48.706329375,27.187500006828,-1.8898197019151E-14));
#6452=CARTESIAN_POINT('',(3.612927284338,50.8792520480092,-48.5721450795008));
#6453=CARTESIAN_POINT('',(48.5134353784345,49.7574536451604,-4.33048599679671));
#6454=CARTESIAN_POINT('Ctrl Pts',(3.612927284338,50.8792520480092,-48.5721450795008));
#6455=CARTESIAN_POINT('Ctrl Pts',(14.7133549689477,50.6985216017706,-47.7464652997852));
#6456=CARTESIAN_POINT('Ctrl Pts',(24.3531646875,50.5208333401613,-42.1809185638422));
#6457=CARTESIAN_POINT('Ctrl Pts',(35.6555077526845,50.312500006828,-35.6555077526845));
#6458=CARTESIAN_POINT('Ctrl Pts',(42.1809185638422,50.1041666734946,-24.3531646875));
#6459=CARTESIAN_POINT('Ctrl Pts',(47.5573898704235,49.9325149229327,-15.0408432190651));
#6460=CARTESIAN_POINT('Ctrl Pts',(48.5134353784345,49.7574536451604,-4.33048599679671));
#6461=CARTESIAN_POINT('Origin',(-4513.80899810642,8003.28355107783,-4.33048626309052));
#6462=CARTESIAN_POINT('Ctrl Pts',(3.61292728433799,49.3132892765089,-45.8578974271399));
#6463=CARTESIAN_POINT('Ctrl Pts',(3.61292728433801,49.4468822859549,-46.089460636719));
#6464=CARTESIAN_POINT('Ctrl Pts',(3.612927284338,49.7140705280012,-46.5525857733052));
#6465=CARTESIAN_POINT('Ctrl Pts',(3.61292728433798,49.9812630238615,-47.0157084557285));
#6466=CARTESIAN_POINT('Ctrl Pts',(3.61292728433798,50.3696539378594,-47.6888965792834));
#6467=CARTESIAN_POINT('Ctrl Pts',(3.612927284338,50.624451287085,-48.1305218136162));
#6468=CARTESIAN_POINT('Ctrl Pts',(3.612927284338,50.8792520480092,-48.5721450795008));
#6469=CARTESIAN_POINT('Ctrl Pts',(-46.,55.6250000136559,0.));
#6470=CARTESIAN_POINT('Ctrl Pts',(-46.,55.4166666803226,-12.3256628518316));
#6471=CARTESIAN_POINT('Ctrl Pts',(-39.8371685740842,55.2083333469893,-23.));
#6472=CARTESIAN_POINT('Ctrl Pts',(-33.6743371481684,55.0000000136559,-33.6743371481684));
#6473=CARTESIAN_POINT('Ctrl Pts',(-23.,54.7916666803226,-39.8371685740842));
#6474=CARTESIAN_POINT('Ctrl Pts',(-12.3256628518317,54.5833333469893,-46.));
#6475=CARTESIAN_POINT('Ctrl Pts',(-2.81668763803891E-15,54.3750000136559,
-46.));
#6476=CARTESIAN_POINT('Ctrl Pts',(12.3256628518316,54.1666666803226,-46.));
#6477=CARTESIAN_POINT('Ctrl Pts',(23.,53.9583333469893,-39.8371685740842));
#6478=CARTESIAN_POINT('Ctrl Pts',(33.6743371481683,53.7500000136559,-33.6743371481684));
#6479=CARTESIAN_POINT('Ctrl Pts',(39.8371685740842,53.5416666803226,-23.));
#6480=CARTESIAN_POINT('Ctrl Pts',(46.,53.3333333469893,-12.3256628518317));
#6481=CARTESIAN_POINT('Ctrl Pts',(46.,53.1250000136559,-5.63337527607782E-15));
#6482=CARTESIAN_POINT('Ctrl Pts',(46.,52.9166666803226,12.3256628518316));
#6483=CARTESIAN_POINT('Ctrl Pts',(39.8371685740842,52.7083333469893,23.));
#6484=CARTESIAN_POINT('Ctrl Pts',(33.6743371481684,52.5000000136559,33.6743371481683));
#6485=CARTESIAN_POINT('Ctrl Pts',(23.,52.2916666803226,39.8371685740842));
#6486=CARTESIAN_POINT('Ctrl Pts',(12.3256628518317,52.0833333469893,46.));
#6487=CARTESIAN_POINT('Ctrl Pts',(8.45006291411674E-15,51.8750000136559,
46.));
#6488=CARTESIAN_POINT('Ctrl Pts',(-12.3256628518316,51.6666666803226,46.));
#6489=CARTESIAN_POINT('Ctrl Pts',(-23.,51.4583333469893,39.8371685740842));
#6490=CARTESIAN_POINT('Ctrl Pts',(-33.6743371481683,51.2500000136559,33.6743371481684));
#6491=CARTESIAN_POINT('Ctrl Pts',(-39.8371685740842,51.0416666803226,23.));
#6492=CARTESIAN_POINT('Ctrl Pts',(-46.,50.8333333469893,12.3256628518317));
#6493=CARTESIAN_POINT('Ctrl Pts',(-46.,50.6250000136559,0.));
#6494=CARTESIAN_POINT('Ctrl Pts',(-46.,50.4166666803226,-12.3256628518316));
#6495=CARTESIAN_POINT('Ctrl Pts',(-39.8371685740842,50.2083333469893,-23.));
#6496=CARTESIAN_POINT('Ctrl Pts',(-33.6743371481684,50.0000000136559,-33.6743371481684));
#6497=CARTESIAN_POINT('Ctrl Pts',(-23.,49.7916666803226,-39.8371685740842));
#6498=CARTESIAN_POINT('Ctrl Pts',(-12.3256628518317,49.5833333469893,-46.));
#6499=CARTESIAN_POINT('Ctrl Pts',(-2.81668763803891E-15,49.3750000136559,
-46.));
#6500=CARTESIAN_POINT('Ctrl Pts',(12.3256628518316,49.1666666803226,-46.));
#6501=CARTESIAN_POINT('Ctrl Pts',(23.,48.9583333469893,-39.8371685740842));
#6502=CARTESIAN_POINT('Ctrl Pts',(33.6743371481683,48.7500000136559,-33.6743371481684));
#6503=CARTESIAN_POINT('Ctrl Pts',(39.8371685740842,48.5416666803226,-23.));
#6504=CARTESIAN_POINT('Ctrl Pts',(46.,48.3333333469893,-12.3256628518317));
#6505=CARTESIAN_POINT('Ctrl Pts',(46.,48.1250000136559,-5.63337527607782E-15));
#6506=CARTESIAN_POINT('Ctrl Pts',(46.,47.9166666803226,12.3256628518316));
#6507=CARTESIAN_POINT('Ctrl Pts',(39.8371685740842,47.7083333469893,23.));
#6508=CARTESIAN_POINT('Ctrl Pts',(33.6743371481684,47.5000000136559,33.6743371481683));
#6509=CARTESIAN_POINT('Ctrl Pts',(23.,47.2916666803226,39.8371685740842));
#6510=CARTESIAN_POINT('Ctrl Pts',(12.3256628518317,47.0833333469893,46.));
#6511=CARTESIAN_POINT('Ctrl Pts',(8.45006291411674E-15,46.8750000136559,
46.));
#6512=CARTESIAN_POINT('Ctrl Pts',(-12.3256628518316,46.6666666803226,46.));
#6513=CARTESIAN_POINT('Ctrl Pts',(-23.,46.4583333469893,39.8371685740842));
#6514=CARTESIAN_POINT('Ctrl Pts',(-33.6743371481683,46.2500000136559,33.6743371481684));
#6515=CARTESIAN_POINT('Ctrl Pts',(-39.8371685740842,46.0416666803226,23.));
#6516=CARTESIAN_POINT('Ctrl Pts',(-46.,45.8333333469892,12.3256628518317));
#6517=CARTESIAN_POINT('Ctrl Pts',(-46.,45.6250000136559,0.));
#6518=CARTESIAN_POINT('Ctrl Pts',(-46.,45.4166666803226,-12.3256628518316));
#6519=CARTESIAN_POINT('Ctrl Pts',(-39.8371685740842,45.2083333469893,-23.));
#6520=CARTESIAN_POINT('Ctrl Pts',(-33.6743371481684,45.0000000136559,-33.6743371481684));
#6521=CARTESIAN_POINT('Ctrl Pts',(-23.,44.7916666803226,-39.8371685740842));
#6522=CARTESIAN_POINT('Ctrl Pts',(-12.3256628518317,44.5833333469893,-46.));
#6523=CARTESIAN_POINT('Ctrl Pts',(-2.81668763803891E-15,44.3750000136559,
-46.));
#6524=CARTESIAN_POINT('Ctrl Pts',(12.3256628518316,44.1666666803226,-46.));
#6525=CARTESIAN_POINT('Ctrl Pts',(23.,43.9583333469893,-39.8371685740842));
#6526=CARTESIAN_POINT('Ctrl Pts',(33.6743371481683,43.7500000136559,-33.6743371481684));
#6527=CARTESIAN_POINT('Ctrl Pts',(39.8371685740842,43.5416666803226,-23.));
#6528=CARTESIAN_POINT('Ctrl Pts',(46.,43.3333333469893,-12.3256628518317));
#6529=CARTESIAN_POINT('Ctrl Pts',(46.,43.1250000136559,-5.63337527607782E-15));
#6530=CARTESIAN_POINT('Ctrl Pts',(46.,42.9166666803226,12.3256628518316));
#6531=CARTESIAN_POINT('Ctrl Pts',(39.8371685740842,42.7083333469893,23.));
#6532=CARTESIAN_POINT('Ctrl Pts',(33.6743371481684,42.5000000136559,33.6743371481683));
#6533=CARTESIAN_POINT('Ctrl Pts',(23.,42.2916666803226,39.8371685740842));
#6534=CARTESIAN_POINT('Ctrl Pts',(12.3256628518317,42.0833333469893,46.));
#6535=CARTESIAN_POINT('Ctrl Pts',(8.45006291411674E-15,41.8750000136559,
46.));
#6536=CARTESIAN_POINT('Ctrl Pts',(-12.3256628518316,41.6666666803226,46.));
#6537=CARTESIAN_POINT('Ctrl Pts',(-23.,41.4583333469893,39.8371685740842));
#6538=CARTESIAN_POINT('Ctrl Pts',(-33.6743371481683,41.2500000136559,33.6743371481684));
#6539=CARTESIAN_POINT('Ctrl Pts',(-39.8371685740842,41.0416666803226,23.));
#6540=CARTESIAN_POINT('Ctrl Pts',(-46.,40.8333333469893,12.3256628518317));
#6541=CARTESIAN_POINT('Ctrl Pts',(-46.,40.6250000136559,0.));
#6542=CARTESIAN_POINT('Ctrl Pts',(-46.,40.4166666803226,-12.3256628518316));
#6543=CARTESIAN_POINT('Ctrl Pts',(-39.8371685740842,40.2083333469893,-23.));
#6544=CARTESIAN_POINT('Ctrl Pts',(-33.6743371481684,40.0000000136559,-33.6743371481684));
#6545=CARTESIAN_POINT('Ctrl Pts',(-23.,39.7916666803226,-39.8371685740842));
#6546=CARTESIAN_POINT('Ctrl Pts',(-12.3256628518317,39.5833333469893,-46.));
#6547=CARTESIAN_POINT('Ctrl Pts',(-2.81668763803891E-15,39.3750000136559,
-46.));
#6548=CARTESIAN_POINT('Ctrl Pts',(12.3256628518316,39.1666666803226,-46.));
#6549=CARTESIAN_POINT('Ctrl Pts',(23.,38.9583333469893,-39.8371685740842));
#6550=CARTESIAN_POINT('Ctrl Pts',(33.6743371481683,38.7500000136559,-33.6743371481684));
#6551=CARTESIAN_POINT('Ctrl Pts',(39.8371685740842,38.5416666803226,-23.));
#6552=CARTESIAN_POINT('Ctrl Pts',(46.,38.3333333469893,-12.3256628518317));
#6553=CARTESIAN_POINT('Ctrl Pts',(46.,38.1250000136559,-5.63337527607782E-15));
#6554=CARTESIAN_POINT('Ctrl Pts',(46.,37.9166666803226,12.3256628518316));
#6555=CARTESIAN_POINT('Ctrl Pts',(39.8371685740842,37.7083333469893,23.));
#6556=CARTESIAN_POINT('Ctrl Pts',(33.6743371481684,37.5000000136559,33.6743371481683));
#6557=CARTESIAN_POINT('Ctrl Pts',(23.,37.2916666803226,39.8371685740842));
#6558=CARTESIAN_POINT('Ctrl Pts',(12.3256628518317,37.0833333469893,46.));
#6559=CARTESIAN_POINT('Ctrl Pts',(8.45006291411674E-15,36.8750000136559,
46.));
#6560=CARTESIAN_POINT('Ctrl Pts',(-12.3256628518316,36.6666666803226,46.));
#6561=CARTESIAN_POINT('Ctrl Pts',(-23.,36.4583333469893,39.8371685740842));
#6562=CARTESIAN_POINT('Ctrl Pts',(-33.6743371481683,36.2500000136559,33.6743371481684));
#6563=CARTESIAN_POINT('Ctrl Pts',(-39.8371685740842,36.0416666803226,23.));
#6564=CARTESIAN_POINT('Ctrl Pts',(-46.,35.8333333469893,12.3256628518317));
#6565=CARTESIAN_POINT('Ctrl Pts',(-46.,35.6250000136559,0.));
#6566=CARTESIAN_POINT('Ctrl Pts',(-46.,35.4166666803226,-12.3256628518316));
#6567=CARTESIAN_POINT('Ctrl Pts',(-39.8371685740842,35.2083333469893,-23.));
#6568=CARTESIAN_POINT('Ctrl Pts',(-33.6743371481684,35.0000000136559,-33.6743371481684));
#6569=CARTESIAN_POINT('Ctrl Pts',(-23.,34.7916666803226,-39.8371685740842));
#6570=CARTESIAN_POINT('Ctrl Pts',(-12.3256628518317,34.5833333469893,-46.));
#6571=CARTESIAN_POINT('Ctrl Pts',(-2.81668763803891E-15,34.3750000136559,
-46.));
#6572=CARTESIAN_POINT('Ctrl Pts',(12.3256628518316,34.1666666803226,-46.));
#6573=CARTESIAN_POINT('Ctrl Pts',(23.,33.9583333469893,-39.8371685740842));
#6574=CARTESIAN_POINT('Ctrl Pts',(33.6743371481683,33.7500000136559,-33.6743371481684));
#6575=CARTESIAN_POINT('Ctrl Pts',(39.8371685740842,33.5416666803226,-23.));
#6576=CARTESIAN_POINT('Ctrl Pts',(46.,33.3333333469893,-12.3256628518317));
#6577=CARTESIAN_POINT('Ctrl Pts',(46.,33.1250000136559,-5.63337527607782E-15));
#6578=CARTESIAN_POINT('Ctrl Pts',(46.,32.9166666803226,12.3256628518316));
#6579=CARTESIAN_POINT('Ctrl Pts',(39.8371685740842,32.7083333469893,23.));
#6580=CARTESIAN_POINT('Ctrl Pts',(33.6743371481684,32.5000000136559,33.6743371481683));
#6581=CARTESIAN_POINT('Ctrl Pts',(23.,32.2916666803226,39.8371685740842));
#6582=CARTESIAN_POINT('Ctrl Pts',(12.3256628518317,32.0833333469893,46.));
#6583=CARTESIAN_POINT('Ctrl Pts',(8.45006291411674E-15,31.8750000136559,
46.));
#6584=CARTESIAN_POINT('Ctrl Pts',(-12.3256628518316,31.6666666803226,46.));
#6585=CARTESIAN_POINT('Ctrl Pts',(-23.,31.4583333469893,39.8371685740842));
#6586=CARTESIAN_POINT('Ctrl Pts',(-33.6743371481683,31.2500000136559,33.6743371481684));
#6587=CARTESIAN_POINT('Ctrl Pts',(-39.8371685740842,31.0416666803226,23.));
#6588=CARTESIAN_POINT('Ctrl Pts',(-46.,30.8333333469893,12.3256628518317));
#6589=CARTESIAN_POINT('Ctrl Pts',(-46.,30.6250000136559,0.));
#6590=CARTESIAN_POINT('Ctrl Pts',(-46.,30.4166666803226,-12.3256628518316));
#6591=CARTESIAN_POINT('Ctrl Pts',(-39.8371685740842,30.2083333469893,-23.));
#6592=CARTESIAN_POINT('Ctrl Pts',(-33.6743371481684,30.0000000136559,-33.6743371481684));
#6593=CARTESIAN_POINT('Ctrl Pts',(-23.,29.7916666803226,-39.8371685740842));
#6594=CARTESIAN_POINT('Ctrl Pts',(-12.3256628518317,29.5833333469893,-46.));
#6595=CARTESIAN_POINT('Ctrl Pts',(-2.81668763803891E-15,29.3750000136559,
-46.));
#6596=CARTESIAN_POINT('Ctrl Pts',(12.3256628518316,29.1666666803226,-46.));
#6597=CARTESIAN_POINT('Ctrl Pts',(23.,28.9583333469893,-39.8371685740842));
#6598=CARTESIAN_POINT('Ctrl Pts',(33.6743371481683,28.7500000136559,-33.6743371481684));
#6599=CARTESIAN_POINT('Ctrl Pts',(39.8371685740842,28.5416666803226,-23.));
#6600=CARTESIAN_POINT('Ctrl Pts',(46.,28.3333333469893,-12.3256628518317));
#6601=CARTESIAN_POINT('Ctrl Pts',(46.,28.1250000136559,-5.63337527607782E-15));
#6602=CARTESIAN_POINT('Ctrl Pts',(46.,27.9166666803226,12.3256628518316));
#6603=CARTESIAN_POINT('Ctrl Pts',(39.8371685740842,27.7083333469893,23.));
#6604=CARTESIAN_POINT('Ctrl Pts',(33.6743371481684,27.5000000136559,33.6743371481683));
#6605=CARTESIAN_POINT('Ctrl Pts',(23.,27.2916666803226,39.8371685740842));
#6606=CARTESIAN_POINT('Ctrl Pts',(12.3256628518317,27.0833333469893,46.));
#6607=CARTESIAN_POINT('Ctrl Pts',(8.45006291411674E-15,26.8750000136559,
46.));
#6608=CARTESIAN_POINT('Ctrl Pts',(-12.3256628518316,26.6666666803226,46.));
#6609=CARTESIAN_POINT('Ctrl Pts',(-23.,26.4583333469893,39.8371685740842));
#6610=CARTESIAN_POINT('Ctrl Pts',(-33.6743371481683,26.2500000136559,33.6743371481684));
#6611=CARTESIAN_POINT('Ctrl Pts',(-39.8371685740842,26.0416666803226,23.));
#6612=CARTESIAN_POINT('Ctrl Pts',(-46.,25.8333333469893,12.3256628518317));
#6613=CARTESIAN_POINT('Ctrl Pts',(-46.,25.6250000136559,0.));
#6614=CARTESIAN_POINT('Ctrl Pts',(-48.706329375,57.187500006828,-1.8898197019151E-14));
#6615=CARTESIAN_POINT('Ctrl Pts',(-48.706329375,56.9791666734946,-13.0508216223155));
#6616=CARTESIAN_POINT('Ctrl Pts',(-42.1809185638422,56.7708333401613,-24.3531646875));
#6617=CARTESIAN_POINT('Ctrl Pts',(-35.6555077526845,56.562500006828,-35.6555077526845));
#6618=CARTESIAN_POINT('Ctrl Pts',(-24.3531646875,56.3541666734946,-42.1809185638423));
#6619=CARTESIAN_POINT('Ctrl Pts',(-13.0508216223155,56.1458333401613,-48.706329375));
#6620=CARTESIAN_POINT('Ctrl Pts',(1.59157945007855E-14,55.937500006828,
-48.706329375));
#6621=CARTESIAN_POINT('Ctrl Pts',(13.0508216223155,55.7291666734946,-48.706329375));
#6622=CARTESIAN_POINT('Ctrl Pts',(24.3531646875,55.5208333401613,-42.1809185638422));
#6623=CARTESIAN_POINT('Ctrl Pts',(35.6555077526845,55.312500006828,-35.6555077526845));
#6624=CARTESIAN_POINT('Ctrl Pts',(42.1809185638422,55.1041666734946,-24.3531646875));
#6625=CARTESIAN_POINT('Ctrl Pts',(48.706329375,54.8958333401613,-13.0508216223155));
#6626=CARTESIAN_POINT('Ctrl Pts',(48.706329375,54.687500006828,1.293339198242E-14));
#6627=CARTESIAN_POINT('Ctrl Pts',(48.706329375,54.4791666734946,13.0508216223155));
#6628=CARTESIAN_POINT('Ctrl Pts',(42.1809185638422,54.2708333401613,24.3531646875));
#6629=CARTESIAN_POINT('Ctrl Pts',(35.6555077526845,54.062500006828,35.6555077526845));
#6630=CARTESIAN_POINT('Ctrl Pts',(24.3531646875,53.8541666734946,42.1809185638422));
#6631=CARTESIAN_POINT('Ctrl Pts',(13.0508216223155,53.6458333401613,48.706329375));
#6632=CARTESIAN_POINT('Ctrl Pts',(-9.95098946405443E-15,53.437500006828,
48.706329375));
#6633=CARTESIAN_POINT('Ctrl Pts',(-13.0508216223155,53.2291666734946,48.706329375));
#6634=CARTESIAN_POINT('Ctrl Pts',(-24.3531646875,53.0208333401613,42.1809185638423));
#6635=CARTESIAN_POINT('Ctrl Pts',(-35.6555077526845,52.812500006828,35.6555077526845));
#6636=CARTESIAN_POINT('Ctrl Pts',(-42.1809185638422,52.6041666734946,24.3531646875));
#6637=CARTESIAN_POINT('Ctrl Pts',(-48.706329375,52.3958333401613,13.0508216223155));
#6638=CARTESIAN_POINT('Ctrl Pts',(-48.706329375,52.187500006828,-1.8898197019151E-14));
#6639=CARTESIAN_POINT('Ctrl Pts',(-48.706329375,51.9791666734946,-13.0508216223155));
#6640=CARTESIAN_POINT('Ctrl Pts',(-42.1809185638422,51.7708333401613,-24.3531646875));
#6641=CARTESIAN_POINT('Ctrl Pts',(-35.6555077526845,51.562500006828,-35.6555077526845));
#6642=CARTESIAN_POINT('Ctrl Pts',(-24.3531646875,51.3541666734946,-42.1809185638423));
#6643=CARTESIAN_POINT('Ctrl Pts',(-13.0508216223155,51.1458333401613,-48.706329375));
#6644=CARTESIAN_POINT('Ctrl Pts',(1.59157945007855E-14,50.937500006828,
-48.706329375));
#6645=CARTESIAN_POINT('Ctrl Pts',(13.0508216223155,50.7291666734946,-48.706329375));
#6646=CARTESIAN_POINT('Ctrl Pts',(24.3531646875,50.5208333401613,-42.1809185638422));
#6647=CARTESIAN_POINT('Ctrl Pts',(35.6555077526845,50.312500006828,-35.6555077526845));
#6648=CARTESIAN_POINT('Ctrl Pts',(42.1809185638422,50.1041666734946,-24.3531646875));
#6649=CARTESIAN_POINT('Ctrl Pts',(48.706329375,49.8958333401613,-13.0508216223155));
#6650=CARTESIAN_POINT('Ctrl Pts',(48.706329375,49.687500006828,1.293339198242E-14));
#6651=CARTESIAN_POINT('Ctrl Pts',(48.706329375,49.4791666734946,13.0508216223155));
#6652=CARTESIAN_POINT('Ctrl Pts',(42.1809185638422,49.2708333401613,24.3531646875));
#6653=CARTESIAN_POINT('Ctrl Pts',(35.6555077526845,49.062500006828,35.6555077526845));
#6654=CARTESIAN_POINT('Ctrl Pts',(24.3531646875,48.8541666734946,42.1809185638422));
#6655=CARTESIAN_POINT('Ctrl Pts',(13.0508216223155,48.6458333401613,48.706329375));
#6656=CARTESIAN_POINT('Ctrl Pts',(-9.95098946405443E-15,48.437500006828,
48.706329375));
#6657=CARTESIAN_POINT('Ctrl Pts',(-13.0508216223155,48.2291666734946,48.706329375));
#6658=CARTESIAN_POINT('Ctrl Pts',(-24.3531646875,48.0208333401613,42.1809185638423));
#6659=CARTESIAN_POINT('Ctrl Pts',(-35.6555077526845,47.812500006828,35.6555077526845));
#6660=CARTESIAN_POINT('Ctrl Pts',(-42.1809185638422,47.6041666734946,24.3531646875));
#6661=CARTESIAN_POINT('Ctrl Pts',(-48.706329375,47.3958333401613,13.0508216223155));
#6662=CARTESIAN_POINT('Ctrl Pts',(-48.706329375,47.187500006828,-1.8898197019151E-14));
#6663=CARTESIAN_POINT('Ctrl Pts',(-48.706329375,46.9791666734946,-13.0508216223155));
#6664=CARTESIAN_POINT('Ctrl Pts',(-42.1809185638422,46.7708333401613,-24.3531646875));
#6665=CARTESIAN_POINT('Ctrl Pts',(-35.6555077526845,46.562500006828,-35.6555077526845));
#6666=CARTESIAN_POINT('Ctrl Pts',(-24.3531646875,46.3541666734946,-42.1809185638423));
#6667=CARTESIAN_POINT('Ctrl Pts',(-13.0508216223155,46.1458333401613,-48.706329375));
#6668=CARTESIAN_POINT('Ctrl Pts',(1.59157945007855E-14,45.937500006828,
-48.706329375));
#6669=CARTESIAN_POINT('Ctrl Pts',(13.0508216223155,45.7291666734946,-48.706329375));
#6670=CARTESIAN_POINT('Ctrl Pts',(24.3531646875,45.5208333401613,-42.1809185638422));
#6671=CARTESIAN_POINT('Ctrl Pts',(35.6555077526845,45.312500006828,-35.6555077526845));
#6672=CARTESIAN_POINT('Ctrl Pts',(42.1809185638422,45.1041666734946,-24.3531646875));
#6673=CARTESIAN_POINT('Ctrl Pts',(48.706329375,44.8958333401613,-13.0508216223155));
#6674=CARTESIAN_POINT('Ctrl Pts',(48.706329375,44.687500006828,1.293339198242E-14));
#6675=CARTESIAN_POINT('Ctrl Pts',(48.706329375,44.4791666734946,13.0508216223155));
#6676=CARTESIAN_POINT('Ctrl Pts',(42.1809185638422,44.2708333401613,24.3531646875));
#6677=CARTESIAN_POINT('Ctrl Pts',(35.6555077526845,44.062500006828,35.6555077526845));
#6678=CARTESIAN_POINT('Ctrl Pts',(24.3531646875,43.8541666734946,42.1809185638422));
#6679=CARTESIAN_POINT('Ctrl Pts',(13.0508216223155,43.6458333401613,48.706329375));
#6680=CARTESIAN_POINT('Ctrl Pts',(-9.95098946405443E-15,43.437500006828,
48.706329375));
#6681=CARTESIAN_POINT('Ctrl Pts',(-13.0508216223155,43.2291666734946,48.706329375));
#6682=CARTESIAN_POINT('Ctrl Pts',(-24.3531646875,43.0208333401613,42.1809185638423));
#6683=CARTESIAN_POINT('Ctrl Pts',(-35.6555077526845,42.812500006828,35.6555077526845));
#6684=CARTESIAN_POINT('Ctrl Pts',(-42.1809185638422,42.6041666734946,24.3531646875));
#6685=CARTESIAN_POINT('Ctrl Pts',(-48.706329375,42.3958333401613,13.0508216223155));
#6686=CARTESIAN_POINT('Ctrl Pts',(-48.706329375,42.187500006828,-1.8898197019151E-14));
#6687=CARTESIAN_POINT('Ctrl Pts',(-48.706329375,41.9791666734946,-13.0508216223155));
#6688=CARTESIAN_POINT('Ctrl Pts',(-42.1809185638422,41.7708333401613,-24.3531646875));
#6689=CARTESIAN_POINT('Ctrl Pts',(-35.6555077526845,41.562500006828,-35.6555077526845));
#6690=CARTESIAN_POINT('Ctrl Pts',(-24.3531646875,41.3541666734946,-42.1809185638423));
#6691=CARTESIAN_POINT('Ctrl Pts',(-13.0508216223155,41.1458333401613,-48.706329375));
#6692=CARTESIAN_POINT('Ctrl Pts',(1.59157945007855E-14,40.937500006828,
-48.706329375));
#6693=CARTESIAN_POINT('Ctrl Pts',(13.0508216223155,40.7291666734946,-48.706329375));
#6694=CARTESIAN_POINT('Ctrl Pts',(24.3531646875,40.5208333401613,-42.1809185638422));
#6695=CARTESIAN_POINT('Ctrl Pts',(35.6555077526845,40.312500006828,-35.6555077526845));
#6696=CARTESIAN_POINT('Ctrl Pts',(42.1809185638422,40.1041666734946,-24.3531646875));
#6697=CARTESIAN_POINT('Ctrl Pts',(48.706329375,39.8958333401613,-13.0508216223155));
#6698=CARTESIAN_POINT('Ctrl Pts',(48.706329375,39.687500006828,1.293339198242E-14));
#6699=CARTESIAN_POINT('Ctrl Pts',(48.706329375,39.4791666734946,13.0508216223155));
#6700=CARTESIAN_POINT('Ctrl Pts',(42.1809185638422,39.2708333401613,24.3531646875));
#6701=CARTESIAN_POINT('Ctrl Pts',(35.6555077526845,39.062500006828,35.6555077526845));
#6702=CARTESIAN_POINT('Ctrl Pts',(24.3531646875,38.8541666734946,42.1809185638422));
#6703=CARTESIAN_POINT('Ctrl Pts',(13.0508216223155,38.6458333401613,48.706329375));
#6704=CARTESIAN_POINT('Ctrl Pts',(-9.95098946405443E-15,38.437500006828,
48.706329375));
#6705=CARTESIAN_POINT('Ctrl Pts',(-13.0508216223155,38.2291666734946,48.706329375));
#6706=CARTESIAN_POINT('Ctrl Pts',(-24.3531646875,38.0208333401613,42.1809185638423));
#6707=CARTESIAN_POINT('Ctrl Pts',(-35.6555077526845,37.812500006828,35.6555077526845));
#6708=CARTESIAN_POINT('Ctrl Pts',(-42.1809185638422,37.6041666734946,24.3531646875));
#6709=CARTESIAN_POINT('Ctrl Pts',(-48.706329375,37.3958333401613,13.0508216223155));
#6710=CARTESIAN_POINT('Ctrl Pts',(-48.706329375,37.187500006828,-1.8898197019151E-14));
#6711=CARTESIAN_POINT('Ctrl Pts',(-48.706329375,36.9791666734946,-13.0508216223155));
#6712=CARTESIAN_POINT('Ctrl Pts',(-42.1809185638422,36.7708333401613,-24.3531646875));
#6713=CARTESIAN_POINT('Ctrl Pts',(-35.6555077526845,36.562500006828,-35.6555077526845));
#6714=CARTESIAN_POINT('Ctrl Pts',(-24.3531646875,36.3541666734946,-42.1809185638423));
#6715=CARTESIAN_POINT('Ctrl Pts',(-13.0508216223155,36.1458333401613,-48.706329375));
#6716=CARTESIAN_POINT('Ctrl Pts',(1.59157945007855E-14,35.937500006828,
-48.706329375));
#6717=CARTESIAN_POINT('Ctrl Pts',(13.0508216223155,35.7291666734946,-48.706329375));
#6718=CARTESIAN_POINT('Ctrl Pts',(24.3531646875,35.5208333401613,-42.1809185638422));
#6719=CARTESIAN_POINT('Ctrl Pts',(35.6555077526845,35.312500006828,-35.6555077526845));
#6720=CARTESIAN_POINT('Ctrl Pts',(42.1809185638422,35.1041666734946,-24.3531646875));
#6721=CARTESIAN_POINT('Ctrl Pts',(48.706329375,34.8958333401613,-13.0508216223155));
#6722=CARTESIAN_POINT('Ctrl Pts',(48.706329375,34.687500006828,1.293339198242E-14));
#6723=CARTESIAN_POINT('Ctrl Pts',(48.706329375,34.4791666734946,13.0508216223155));
#6724=CARTESIAN_POINT('Ctrl Pts',(42.1809185638422,34.2708333401613,24.3531646875));
#6725=CARTESIAN_POINT('Ctrl Pts',(35.6555077526845,34.062500006828,35.6555077526845));
#6726=CARTESIAN_POINT('Ctrl Pts',(24.3531646875,33.8541666734946,42.1809185638422));
#6727=CARTESIAN_POINT('Ctrl Pts',(13.0508216223155,33.6458333401613,48.706329375));
#6728=CARTESIAN_POINT('Ctrl Pts',(-9.95098946405443E-15,33.437500006828,
48.706329375));
#6729=CARTESIAN_POINT('Ctrl Pts',(-13.0508216223155,33.2291666734946,48.706329375));
#6730=CARTESIAN_POINT('Ctrl Pts',(-24.3531646875,33.0208333401613,42.1809185638423));
#6731=CARTESIAN_POINT('Ctrl Pts',(-35.6555077526845,32.812500006828,35.6555077526845));
#6732=CARTESIAN_POINT('Ctrl Pts',(-42.1809185638422,32.6041666734946,24.3531646875));
#6733=CARTESIAN_POINT('Ctrl Pts',(-48.706329375,32.3958333401613,13.0508216223155));
#6734=CARTESIAN_POINT('Ctrl Pts',(-48.706329375,32.187500006828,-1.8898197019151E-14));
#6735=CARTESIAN_POINT('Ctrl Pts',(-48.706329375,31.9791666734946,-13.0508216223155));
#6736=CARTESIAN_POINT('Ctrl Pts',(-42.1809185638422,31.7708333401613,-24.3531646875));
#6737=CARTESIAN_POINT('Ctrl Pts',(-35.6555077526845,31.562500006828,-35.6555077526845));
#6738=CARTESIAN_POINT('Ctrl Pts',(-24.3531646875,31.3541666734946,-42.1809185638423));
#6739=CARTESIAN_POINT('Ctrl Pts',(-13.0508216223155,31.1458333401613,-48.706329375));
#6740=CARTESIAN_POINT('Ctrl Pts',(1.59157945007855E-14,30.937500006828,
-48.706329375));
#6741=CARTESIAN_POINT('Ctrl Pts',(13.0508216223155,30.7291666734946,-48.706329375));
#6742=CARTESIAN_POINT('Ctrl Pts',(24.3531646875,30.5208333401613,-42.1809185638422));
#6743=CARTESIAN_POINT('Ctrl Pts',(35.6555077526845,30.312500006828,-35.6555077526845));
#6744=CARTESIAN_POINT('Ctrl Pts',(42.1809185638422,30.1041666734946,-24.3531646875));
#6745=CARTESIAN_POINT('Ctrl Pts',(48.706329375,29.8958333401613,-13.0508216223155));
#6746=CARTESIAN_POINT('Ctrl Pts',(48.706329375,29.687500006828,1.293339198242E-14));
#6747=CARTESIAN_POINT('Ctrl Pts',(48.706329375,29.4791666734946,13.0508216223155));
#6748=CARTESIAN_POINT('Ctrl Pts',(42.1809185638422,29.2708333401613,24.3531646875));
#6749=CARTESIAN_POINT('Ctrl Pts',(35.6555077526845,29.062500006828,35.6555077526845));
#6750=CARTESIAN_POINT('Ctrl Pts',(24.3531646875,28.8541666734946,42.1809185638422));
#6751=CARTESIAN_POINT('Ctrl Pts',(13.0508216223155,28.6458333401613,48.706329375));
#6752=CARTESIAN_POINT('Ctrl Pts',(-9.95098946405443E-15,28.437500006828,
48.706329375));
#6753=CARTESIAN_POINT('Ctrl Pts',(-13.0508216223155,28.2291666734946,48.706329375));
#6754=CARTESIAN_POINT('Ctrl Pts',(-24.3531646875,28.0208333401613,42.1809185638423));
#6755=CARTESIAN_POINT('Ctrl Pts',(-35.6555077526845,27.812500006828,35.6555077526845));
#6756=CARTESIAN_POINT('Ctrl Pts',(-42.1809185638422,27.6041666734946,24.3531646875));
#6757=CARTESIAN_POINT('Ctrl Pts',(-48.706329375,27.3958333401613,13.0508216223155));
#6758=CARTESIAN_POINT('Ctrl Pts',(-48.706329375,27.187500006828,-1.8898197019151E-14));
#6759=CARTESIAN_POINT('',(48.5725845633798,49.6293483229262,3.60701400320328));
#6760=CARTESIAN_POINT('Ctrl Pts',(45.858362923034,48.0633913333999,3.60701400320327));
#6761=CARTESIAN_POINT('Ctrl Pts',(46.089925771934,48.1969849680263,3.60701400320324));
#6762=CARTESIAN_POINT('Ctrl Pts',(46.5530501979845,48.4641744416604,3.60701400320326));
#6763=CARTESIAN_POINT('Ctrl Pts',(47.0161721905706,48.7313681332063,3.60701400320324));
#6764=CARTESIAN_POINT('Ctrl Pts',(47.6893519862319,49.1197565257476,3.60701400320324));
#6765=CARTESIAN_POINT('Ctrl Pts',(48.1309692507095,49.3745507329179,3.60701400320328));
#6766=CARTESIAN_POINT('Ctrl Pts',(48.5725845633798,49.6293483229262,3.60701400320328));
#6767=CARTESIAN_POINT('',(3.61292728433797,48.4957479656467,48.5721450795008));
#6768=CARTESIAN_POINT('Ctrl Pts',(48.5725845633798,49.6293483229262,3.60701400320328));
#6769=CARTESIAN_POINT('Ctrl Pts',(47.7480251419552,49.4485714020251,14.7106532430575));
#6770=CARTESIAN_POINT('Ctrl Pts',(42.1809185638422,49.2708333401613,24.3531646875));
#6771=CARTESIAN_POINT('Ctrl Pts',(35.6555077526845,49.062500006828,35.6555077526845));
#6772=CARTESIAN_POINT('Ctrl Pts',(24.3531646875,48.8541666734946,42.1809185638422));
#6773=CARTESIAN_POINT('Ctrl Pts',(14.7133549689477,48.6764784118853,47.7464652997852));
#6774=CARTESIAN_POINT('Ctrl Pts',(3.61292728433797,48.4957479656467,48.5721450795008));
#6775=CARTESIAN_POINT('Ctrl Pts',(3.61292728433797,48.4957479656467,48.5721450795008));
#6776=CARTESIAN_POINT('Ctrl Pts',(3.61292728433797,48.3625660950884,48.3403451622817));
#6777=CARTESIAN_POINT('Ctrl Pts',(3.612927284338,48.2293911846469,48.1085412459393));
#6778=CARTESIAN_POINT('Ctrl Pts',(3.612927284338,47.9630558994543,47.6449250631479));
#6779=CARTESIAN_POINT('Ctrl Pts',(3.61292728433804,47.8298955244832,47.4131127965212));
#6780=CARTESIAN_POINT('Ctrl Pts',(3.61292728433804,47.6967427432646,47.1812961682826));
#6781=CARTESIAN_POINT('Ctrl Pts',(3.61292728433804,47.4433704509922,46.7401795055578));
#6782=CARTESIAN_POINT('Ctrl Pts',(3.61292728433798,47.1900256371662,46.2990470581854));
#6783=CARTESIAN_POINT('Ctrl Pts',(3.61292728433798,46.936710750803,45.8578974271399));
#6784=CARTESIAN_POINT('Ctrl Pts',(-46.,55.6250000136559,0.));
#6785=CARTESIAN_POINT('Ctrl Pts',(-46.,55.4166666803226,-12.3256628518316));
#6786=CARTESIAN_POINT('Ctrl Pts',(-39.8371685740842,55.2083333469893,-23.));
#6787=CARTESIAN_POINT('Ctrl Pts',(-33.6743371481684,55.0000000136559,-33.6743371481684));
#6788=CARTESIAN_POINT('Ctrl Pts',(-23.,54.7916666803226,-39.8371685740842));
#6789=CARTESIAN_POINT('Ctrl Pts',(-12.3256628518317,54.5833333469893,-46.));
#6790=CARTESIAN_POINT('Ctrl Pts',(-2.81668763803891E-15,54.3750000136559,
-46.));
#6791=CARTESIAN_POINT('Ctrl Pts',(12.3256628518316,54.1666666803226,-46.));
#6792=CARTESIAN_POINT('Ctrl Pts',(23.,53.9583333469893,-39.8371685740842));
#6793=CARTESIAN_POINT('Ctrl Pts',(33.6743371481683,53.7500000136559,-33.6743371481684));
#6794=CARTESIAN_POINT('Ctrl Pts',(39.8371685740842,53.5416666803226,-23.));
#6795=CARTESIAN_POINT('Ctrl Pts',(46.,53.3333333469893,-12.3256628518317));
#6796=CARTESIAN_POINT('Ctrl Pts',(46.,53.1250000136559,-5.63337527607782E-15));
#6797=CARTESIAN_POINT('Ctrl Pts',(46.,52.9166666803226,12.3256628518316));
#6798=CARTESIAN_POINT('Ctrl Pts',(39.8371685740842,52.7083333469893,23.));
#6799=CARTESIAN_POINT('Ctrl Pts',(33.6743371481684,52.5000000136559,33.6743371481683));
#6800=CARTESIAN_POINT('Ctrl Pts',(23.,52.2916666803226,39.8371685740842));
#6801=CARTESIAN_POINT('Ctrl Pts',(12.3256628518317,52.0833333469893,46.));
#6802=CARTESIAN_POINT('Ctrl Pts',(8.45006291411674E-15,51.8750000136559,
46.));
#6803=CARTESIAN_POINT('Ctrl Pts',(-12.3256628518316,51.6666666803226,46.));
#6804=CARTESIAN_POINT('Ctrl Pts',(-23.,51.4583333469893,39.8371685740842));
#6805=CARTESIAN_POINT('Ctrl Pts',(-33.6743371481683,51.2500000136559,33.6743371481684));
#6806=CARTESIAN_POINT('Ctrl Pts',(-39.8371685740842,51.0416666803226,23.));
#6807=CARTESIAN_POINT('Ctrl Pts',(-46.,50.8333333469893,12.3256628518317));
#6808=CARTESIAN_POINT('Ctrl Pts',(-46.,50.6250000136559,0.));
#6809=CARTESIAN_POINT('Ctrl Pts',(-46.,50.4166666803226,-12.3256628518316));
#6810=CARTESIAN_POINT('Ctrl Pts',(-39.8371685740842,50.2083333469893,-23.));
#6811=CARTESIAN_POINT('Ctrl Pts',(-33.6743371481684,50.0000000136559,-33.6743371481684));
#6812=CARTESIAN_POINT('Ctrl Pts',(-23.,49.7916666803226,-39.8371685740842));
#6813=CARTESIAN_POINT('Ctrl Pts',(-12.3256628518317,49.5833333469893,-46.));
#6814=CARTESIAN_POINT('Ctrl Pts',(-2.81668763803891E-15,49.3750000136559,
-46.));
#6815=CARTESIAN_POINT('Ctrl Pts',(12.3256628518316,49.1666666803226,-46.));
#6816=CARTESIAN_POINT('Ctrl Pts',(23.,48.9583333469893,-39.8371685740842));
#6817=CARTESIAN_POINT('Ctrl Pts',(33.6743371481683,48.7500000136559,-33.6743371481684));
#6818=CARTESIAN_POINT('Ctrl Pts',(39.8371685740842,48.5416666803226,-23.));
#6819=CARTESIAN_POINT('Ctrl Pts',(46.,48.3333333469893,-12.3256628518317));
#6820=CARTESIAN_POINT('Ctrl Pts',(46.,48.1250000136559,-5.63337527607782E-15));
#6821=CARTESIAN_POINT('Ctrl Pts',(46.,47.9166666803226,12.3256628518316));
#6822=CARTESIAN_POINT('Ctrl Pts',(39.8371685740842,47.7083333469893,23.));
#6823=CARTESIAN_POINT('Ctrl Pts',(33.6743371481684,47.5000000136559,33.6743371481683));
#6824=CARTESIAN_POINT('Ctrl Pts',(23.,47.2916666803226,39.8371685740842));
#6825=CARTESIAN_POINT('Ctrl Pts',(12.3256628518317,47.0833333469893,46.));
#6826=CARTESIAN_POINT('Ctrl Pts',(8.45006291411674E-15,46.8750000136559,
46.));
#6827=CARTESIAN_POINT('Ctrl Pts',(-12.3256628518316,46.6666666803226,46.));
#6828=CARTESIAN_POINT('Ctrl Pts',(-23.,46.4583333469893,39.8371685740842));
#6829=CARTESIAN_POINT('Ctrl Pts',(-33.6743371481683,46.2500000136559,33.6743371481684));
#6830=CARTESIAN_POINT('Ctrl Pts',(-39.8371685740842,46.0416666803226,23.));
#6831=CARTESIAN_POINT('Ctrl Pts',(-46.,45.8333333469892,12.3256628518317));
#6832=CARTESIAN_POINT('Ctrl Pts',(-46.,45.6250000136559,0.));
#6833=CARTESIAN_POINT('Ctrl Pts',(-46.,45.4166666803226,-12.3256628518316));
#6834=CARTESIAN_POINT('Ctrl Pts',(-39.8371685740842,45.2083333469893,-23.));
#6835=CARTESIAN_POINT('Ctrl Pts',(-33.6743371481684,45.0000000136559,-33.6743371481684));
#6836=CARTESIAN_POINT('Ctrl Pts',(-23.,44.7916666803226,-39.8371685740842));
#6837=CARTESIAN_POINT('Ctrl Pts',(-12.3256628518317,44.5833333469893,-46.));
#6838=CARTESIAN_POINT('Ctrl Pts',(-2.81668763803891E-15,44.3750000136559,
-46.));
#6839=CARTESIAN_POINT('Ctrl Pts',(12.3256628518316,44.1666666803226,-46.));
#6840=CARTESIAN_POINT('Ctrl Pts',(23.,43.9583333469893,-39.8371685740842));
#6841=CARTESIAN_POINT('Ctrl Pts',(33.6743371481683,43.7500000136559,-33.6743371481684));
#6842=CARTESIAN_POINT('Ctrl Pts',(39.8371685740842,43.5416666803226,-23.));
#6843=CARTESIAN_POINT('Ctrl Pts',(46.,43.3333333469893,-12.3256628518317));
#6844=CARTESIAN_POINT('Ctrl Pts',(46.,43.1250000136559,-5.63337527607782E-15));
#6845=CARTESIAN_POINT('Ctrl Pts',(46.,42.9166666803226,12.3256628518316));
#6846=CARTESIAN_POINT('Ctrl Pts',(39.8371685740842,42.7083333469893,23.));
#6847=CARTESIAN_POINT('Ctrl Pts',(33.6743371481684,42.5000000136559,33.6743371481683));
#6848=CARTESIAN_POINT('Ctrl Pts',(23.,42.2916666803226,39.8371685740842));
#6849=CARTESIAN_POINT('Ctrl Pts',(12.3256628518317,42.0833333469893,46.));
#6850=CARTESIAN_POINT('Ctrl Pts',(8.45006291411674E-15,41.8750000136559,
46.));
#6851=CARTESIAN_POINT('Ctrl Pts',(-12.3256628518316,41.6666666803226,46.));
#6852=CARTESIAN_POINT('Ctrl Pts',(-23.,41.4583333469893,39.8371685740842));
#6853=CARTESIAN_POINT('Ctrl Pts',(-33.6743371481683,41.2500000136559,33.6743371481684));
#6854=CARTESIAN_POINT('Ctrl Pts',(-39.8371685740842,41.0416666803226,23.));
#6855=CARTESIAN_POINT('Ctrl Pts',(-46.,40.8333333469893,12.3256628518317));
#6856=CARTESIAN_POINT('Ctrl Pts',(-46.,40.6250000136559,0.));
#6857=CARTESIAN_POINT('Ctrl Pts',(-46.,40.4166666803226,-12.3256628518316));
#6858=CARTESIAN_POINT('Ctrl Pts',(-39.8371685740842,40.2083333469893,-23.));
#6859=CARTESIAN_POINT('Ctrl Pts',(-33.6743371481684,40.0000000136559,-33.6743371481684));
#6860=CARTESIAN_POINT('Ctrl Pts',(-23.,39.7916666803226,-39.8371685740842));
#6861=CARTESIAN_POINT('Ctrl Pts',(-12.3256628518317,39.5833333469893,-46.));
#6862=CARTESIAN_POINT('Ctrl Pts',(-2.81668763803891E-15,39.3750000136559,
-46.));
#6863=CARTESIAN_POINT('Ctrl Pts',(12.3256628518316,39.1666666803226,-46.));
#6864=CARTESIAN_POINT('Ctrl Pts',(23.,38.9583333469893,-39.8371685740842));
#6865=CARTESIAN_POINT('Ctrl Pts',(33.6743371481683,38.7500000136559,-33.6743371481684));
#6866=CARTESIAN_POINT('Ctrl Pts',(39.8371685740842,38.5416666803226,-23.));
#6867=CARTESIAN_POINT('Ctrl Pts',(46.,38.3333333469893,-12.3256628518317));
#6868=CARTESIAN_POINT('Ctrl Pts',(46.,38.1250000136559,-5.63337527607782E-15));
#6869=CARTESIAN_POINT('Ctrl Pts',(46.,37.9166666803226,12.3256628518316));
#6870=CARTESIAN_POINT('Ctrl Pts',(39.8371685740842,37.7083333469893,23.));
#6871=CARTESIAN_POINT('Ctrl Pts',(33.6743371481684,37.5000000136559,33.6743371481683));
#6872=CARTESIAN_POINT('Ctrl Pts',(23.,37.2916666803226,39.8371685740842));
#6873=CARTESIAN_POINT('Ctrl Pts',(12.3256628518317,37.0833333469893,46.));
#6874=CARTESIAN_POINT('Ctrl Pts',(8.45006291411674E-15,36.8750000136559,
46.));
#6875=CARTESIAN_POINT('Ctrl Pts',(-12.3256628518316,36.6666666803226,46.));
#6876=CARTESIAN_POINT('Ctrl Pts',(-23.,36.4583333469893,39.8371685740842));
#6877=CARTESIAN_POINT('Ctrl Pts',(-33.6743371481683,36.2500000136559,33.6743371481684));
#6878=CARTESIAN_POINT('Ctrl Pts',(-39.8371685740842,36.0416666803226,23.));
#6879=CARTESIAN_POINT('Ctrl Pts',(-46.,35.8333333469893,12.3256628518317));
#6880=CARTESIAN_POINT('Ctrl Pts',(-46.,35.6250000136559,0.));
#6881=CARTESIAN_POINT('Ctrl Pts',(-46.,35.4166666803226,-12.3256628518316));
#6882=CARTESIAN_POINT('Ctrl Pts',(-39.8371685740842,35.2083333469893,-23.));
#6883=CARTESIAN_POINT('Ctrl Pts',(-33.6743371481684,35.0000000136559,-33.6743371481684));
#6884=CARTESIAN_POINT('Ctrl Pts',(-23.,34.7916666803226,-39.8371685740842));
#6885=CARTESIAN_POINT('Ctrl Pts',(-12.3256628518317,34.5833333469893,-46.));
#6886=CARTESIAN_POINT('Ctrl Pts',(-2.81668763803891E-15,34.3750000136559,
-46.));
#6887=CARTESIAN_POINT('Ctrl Pts',(12.3256628518316,34.1666666803226,-46.));
#6888=CARTESIAN_POINT('Ctrl Pts',(23.,33.9583333469893,-39.8371685740842));
#6889=CARTESIAN_POINT('Ctrl Pts',(33.6743371481683,33.7500000136559,-33.6743371481684));
#6890=CARTESIAN_POINT('Ctrl Pts',(39.8371685740842,33.5416666803226,-23.));
#6891=CARTESIAN_POINT('Ctrl Pts',(46.,33.3333333469893,-12.3256628518317));
#6892=CARTESIAN_POINT('Ctrl Pts',(46.,33.1250000136559,-5.63337527607782E-15));
#6893=CARTESIAN_POINT('Ctrl Pts',(46.,32.9166666803226,12.3256628518316));
#6894=CARTESIAN_POINT('Ctrl Pts',(39.8371685740842,32.7083333469893,23.));
#6895=CARTESIAN_POINT('Ctrl Pts',(33.6743371481684,32.5000000136559,33.6743371481683));
#6896=CARTESIAN_POINT('Ctrl Pts',(23.,32.2916666803226,39.8371685740842));
#6897=CARTESIAN_POINT('Ctrl Pts',(12.3256628518317,32.0833333469893,46.));
#6898=CARTESIAN_POINT('Ctrl Pts',(8.45006291411674E-15,31.8750000136559,
46.));
#6899=CARTESIAN_POINT('Ctrl Pts',(-12.3256628518316,31.6666666803226,46.));
#6900=CARTESIAN_POINT('Ctrl Pts',(-23.,31.4583333469893,39.8371685740842));
#6901=CARTESIAN_POINT('Ctrl Pts',(-33.6743371481683,31.2500000136559,33.6743371481684));
#6902=CARTESIAN_POINT('Ctrl Pts',(-39.8371685740842,31.0416666803226,23.));
#6903=CARTESIAN_POINT('Ctrl Pts',(-46.,30.8333333469893,12.3256628518317));
#6904=CARTESIAN_POINT('Ctrl Pts',(-46.,30.6250000136559,0.));
#6905=CARTESIAN_POINT('Ctrl Pts',(-46.,30.4166666803226,-12.3256628518316));
#6906=CARTESIAN_POINT('Ctrl Pts',(-39.8371685740842,30.2083333469893,-23.));
#6907=CARTESIAN_POINT('Ctrl Pts',(-33.6743371481684,30.0000000136559,-33.6743371481684));
#6908=CARTESIAN_POINT('Ctrl Pts',(-23.,29.7916666803226,-39.8371685740842));
#6909=CARTESIAN_POINT('Ctrl Pts',(-12.3256628518317,29.5833333469893,-46.));
#6910=CARTESIAN_POINT('Ctrl Pts',(-2.81668763803891E-15,29.3750000136559,
-46.));
#6911=CARTESIAN_POINT('Ctrl Pts',(12.3256628518316,29.1666666803226,-46.));
#6912=CARTESIAN_POINT('Ctrl Pts',(23.,28.9583333469893,-39.8371685740842));
#6913=CARTESIAN_POINT('Ctrl Pts',(33.6743371481683,28.7500000136559,-33.6743371481684));
#6914=CARTESIAN_POINT('Ctrl Pts',(39.8371685740842,28.5416666803226,-23.));
#6915=CARTESIAN_POINT('Ctrl Pts',(46.,28.3333333469893,-12.3256628518317));
#6916=CARTESIAN_POINT('Ctrl Pts',(46.,28.1250000136559,-5.63337527607782E-15));
#6917=CARTESIAN_POINT('Ctrl Pts',(46.,27.9166666803226,12.3256628518316));
#6918=CARTESIAN_POINT('Ctrl Pts',(39.8371685740842,27.7083333469893,23.));
#6919=CARTESIAN_POINT('Ctrl Pts',(33.6743371481684,27.5000000136559,33.6743371481683));
#6920=CARTESIAN_POINT('Ctrl Pts',(23.,27.2916666803226,39.8371685740842));
#6921=CARTESIAN_POINT('Ctrl Pts',(12.3256628518317,27.0833333469893,46.));
#6922=CARTESIAN_POINT('Ctrl Pts',(8.45006291411674E-15,26.8750000136559,
46.));
#6923=CARTESIAN_POINT('Ctrl Pts',(-12.3256628518316,26.6666666803226,46.));
#6924=CARTESIAN_POINT('Ctrl Pts',(-23.,26.4583333469893,39.8371685740842));
#6925=CARTESIAN_POINT('Ctrl Pts',(-33.6743371481683,26.2500000136559,33.6743371481684));
#6926=CARTESIAN_POINT('Ctrl Pts',(-39.8371685740842,26.0416666803226,23.));
#6927=CARTESIAN_POINT('Ctrl Pts',(-46.,25.8333333469893,12.3256628518317));
#6928=CARTESIAN_POINT('Ctrl Pts',(-46.,25.6250000136559,0.));
#6929=CARTESIAN_POINT('Ctrl Pts',(-48.706329375,57.187500006828,-1.8898197019151E-14));
#6930=CARTESIAN_POINT('Ctrl Pts',(-48.706329375,56.9791666734946,-13.0508216223155));
#6931=CARTESIAN_POINT('Ctrl Pts',(-42.1809185638422,56.7708333401613,-24.3531646875));
#6932=CARTESIAN_POINT('Ctrl Pts',(-35.6555077526845,56.562500006828,-35.6555077526845));
#6933=CARTESIAN_POINT('Ctrl Pts',(-24.3531646875,56.3541666734946,-42.1809185638423));
#6934=CARTESIAN_POINT('Ctrl Pts',(-13.0508216223155,56.1458333401613,-48.706329375));
#6935=CARTESIAN_POINT('Ctrl Pts',(1.59157945007855E-14,55.937500006828,
-48.706329375));
#6936=CARTESIAN_POINT('Ctrl Pts',(13.0508216223155,55.7291666734946,-48.706329375));
#6937=CARTESIAN_POINT('Ctrl Pts',(24.3531646875,55.5208333401613,-42.1809185638422));
#6938=CARTESIAN_POINT('Ctrl Pts',(35.6555077526845,55.312500006828,-35.6555077526845));
#6939=CARTESIAN_POINT('Ctrl Pts',(42.1809185638422,55.1041666734946,-24.3531646875));
#6940=CARTESIAN_POINT('Ctrl Pts',(48.706329375,54.8958333401613,-13.0508216223155));
#6941=CARTESIAN_POINT('Ctrl Pts',(48.706329375,54.687500006828,1.293339198242E-14));
#6942=CARTESIAN_POINT('Ctrl Pts',(48.706329375,54.4791666734946,13.0508216223155));
#6943=CARTESIAN_POINT('Ctrl Pts',(42.1809185638422,54.2708333401613,24.3531646875));
#6944=CARTESIAN_POINT('Ctrl Pts',(35.6555077526845,54.062500006828,35.6555077526845));
#6945=CARTESIAN_POINT('Ctrl Pts',(24.3531646875,53.8541666734946,42.1809185638422));
#6946=CARTESIAN_POINT('Ctrl Pts',(13.0508216223155,53.6458333401613,48.706329375));
#6947=CARTESIAN_POINT('Ctrl Pts',(-9.95098946405443E-15,53.437500006828,
48.706329375));
#6948=CARTESIAN_POINT('Ctrl Pts',(-13.0508216223155,53.2291666734946,48.706329375));
#6949=CARTESIAN_POINT('Ctrl Pts',(-24.3531646875,53.0208333401613,42.1809185638423));
#6950=CARTESIAN_POINT('Ctrl Pts',(-35.6555077526845,52.812500006828,35.6555077526845));
#6951=CARTESIAN_POINT('Ctrl Pts',(-42.1809185638422,52.6041666734946,24.3531646875));
#6952=CARTESIAN_POINT('Ctrl Pts',(-48.706329375,52.3958333401613,13.0508216223155));
#6953=CARTESIAN_POINT('Ctrl Pts',(-48.706329375,52.187500006828,-1.8898197019151E-14));
#6954=CARTESIAN_POINT('Ctrl Pts',(-48.706329375,51.9791666734946,-13.0508216223155));
#6955=CARTESIAN_POINT('Ctrl Pts',(-42.1809185638422,51.7708333401613,-24.3531646875));
#6956=CARTESIAN_POINT('Ctrl Pts',(-35.6555077526845,51.562500006828,-35.6555077526845));
#6957=CARTESIAN_POINT('Ctrl Pts',(-24.3531646875,51.3541666734946,-42.1809185638423));
#6958=CARTESIAN_POINT('Ctrl Pts',(-13.0508216223155,51.1458333401613,-48.706329375));
#6959=CARTESIAN_POINT('Ctrl Pts',(1.59157945007855E-14,50.937500006828,
-48.706329375));
#6960=CARTESIAN_POINT('Ctrl Pts',(13.0508216223155,50.7291666734946,-48.706329375));
#6961=CARTESIAN_POINT('Ctrl Pts',(24.3531646875,50.5208333401613,-42.1809185638422));
#6962=CARTESIAN_POINT('Ctrl Pts',(35.6555077526845,50.312500006828,-35.6555077526845));
#6963=CARTESIAN_POINT('Ctrl Pts',(42.1809185638422,50.1041666734946,-24.3531646875));
#6964=CARTESIAN_POINT('Ctrl Pts',(48.706329375,49.8958333401613,-13.0508216223155));
#6965=CARTESIAN_POINT('Ctrl Pts',(48.706329375,49.687500006828,1.293339198242E-14));
#6966=CARTESIAN_POINT('Ctrl Pts',(48.706329375,49.4791666734946,13.0508216223155));
#6967=CARTESIAN_POINT('Ctrl Pts',(42.1809185638422,49.2708333401613,24.3531646875));
#6968=CARTESIAN_POINT('Ctrl Pts',(35.6555077526845,49.062500006828,35.6555077526845));
#6969=CARTESIAN_POINT('Ctrl Pts',(24.3531646875,48.8541666734946,42.1809185638422));
#6970=CARTESIAN_POINT('Ctrl Pts',(13.0508216223155,48.6458333401613,48.706329375));
#6971=CARTESIAN_POINT('Ctrl Pts',(-9.95098946405443E-15,48.437500006828,
48.706329375));
#6972=CARTESIAN_POINT('Ctrl Pts',(-13.0508216223155,48.2291666734946,48.706329375));
#6973=CARTESIAN_POINT('Ctrl Pts',(-24.3531646875,48.0208333401613,42.1809185638423));
#6974=CARTESIAN_POINT('Ctrl Pts',(-35.6555077526845,47.812500006828,35.6555077526845));
#6975=CARTESIAN_POINT('Ctrl Pts',(-42.1809185638422,47.6041666734946,24.3531646875));
#6976=CARTESIAN_POINT('Ctrl Pts',(-48.706329375,47.3958333401613,13.0508216223155));
#6977=CARTESIAN_POINT('Ctrl Pts',(-48.706329375,47.187500006828,-1.8898197019151E-14));
#6978=CARTESIAN_POINT('Ctrl Pts',(-48.706329375,46.9791666734946,-13.0508216223155));
#6979=CARTESIAN_POINT('Ctrl Pts',(-42.1809185638422,46.7708333401613,-24.3531646875));
#6980=CARTESIAN_POINT('Ctrl Pts',(-35.6555077526845,46.562500006828,-35.6555077526845));
#6981=CARTESIAN_POINT('Ctrl Pts',(-24.3531646875,46.3541666734946,-42.1809185638423));
#6982=CARTESIAN_POINT('Ctrl Pts',(-13.0508216223155,46.1458333401613,-48.706329375));
#6983=CARTESIAN_POINT('Ctrl Pts',(1.59157945007855E-14,45.937500006828,
-48.706329375));
#6984=CARTESIAN_POINT('Ctrl Pts',(13.0508216223155,45.7291666734946,-48.706329375));
#6985=CARTESIAN_POINT('Ctrl Pts',(24.3531646875,45.5208333401613,-42.1809185638422));
#6986=CARTESIAN_POINT('Ctrl Pts',(35.6555077526845,45.312500006828,-35.6555077526845));
#6987=CARTESIAN_POINT('Ctrl Pts',(42.1809185638422,45.1041666734946,-24.3531646875));
#6988=CARTESIAN_POINT('Ctrl Pts',(48.706329375,44.8958333401613,-13.0508216223155));
#6989=CARTESIAN_POINT('Ctrl Pts',(48.706329375,44.687500006828,1.293339198242E-14));
#6990=CARTESIAN_POINT('Ctrl Pts',(48.706329375,44.4791666734946,13.0508216223155));
#6991=CARTESIAN_POINT('Ctrl Pts',(42.1809185638422,44.2708333401613,24.3531646875));
#6992=CARTESIAN_POINT('Ctrl Pts',(35.6555077526845,44.062500006828,35.6555077526845));
#6993=CARTESIAN_POINT('Ctrl Pts',(24.3531646875,43.8541666734946,42.1809185638422));
#6994=CARTESIAN_POINT('Ctrl Pts',(13.0508216223155,43.6458333401613,48.706329375));
#6995=CARTESIAN_POINT('Ctrl Pts',(-9.95098946405443E-15,43.437500006828,
48.706329375));
#6996=CARTESIAN_POINT('Ctrl Pts',(-13.0508216223155,43.2291666734946,48.706329375));
#6997=CARTESIAN_POINT('Ctrl Pts',(-24.3531646875,43.0208333401613,42.1809185638423));
#6998=CARTESIAN_POINT('Ctrl Pts',(-35.6555077526845,42.812500006828,35.6555077526845));
#6999=CARTESIAN_POINT('Ctrl Pts',(-42.1809185638422,42.6041666734946,24.3531646875));
#7000=CARTESIAN_POINT('Ctrl Pts',(-48.706329375,42.3958333401613,13.0508216223155));
#7001=CARTESIAN_POINT('Ctrl Pts',(-48.706329375,42.187500006828,-1.8898197019151E-14));
#7002=CARTESIAN_POINT('Ctrl Pts',(-48.706329375,41.9791666734946,-13.0508216223155));
#7003=CARTESIAN_POINT('Ctrl Pts',(-42.1809185638422,41.7708333401613,-24.3531646875));
#7004=CARTESIAN_POINT('Ctrl Pts',(-35.6555077526845,41.562500006828,-35.6555077526845));
#7005=CARTESIAN_POINT('Ctrl Pts',(-24.3531646875,41.3541666734946,-42.1809185638423));
#7006=CARTESIAN_POINT('Ctrl Pts',(-13.0508216223155,41.1458333401613,-48.706329375));
#7007=CARTESIAN_POINT('Ctrl Pts',(1.59157945007855E-14,40.937500006828,
-48.706329375));
#7008=CARTESIAN_POINT('Ctrl Pts',(13.0508216223155,40.7291666734946,-48.706329375));
#7009=CARTESIAN_POINT('Ctrl Pts',(24.3531646875,40.5208333401613,-42.1809185638422));
#7010=CARTESIAN_POINT('Ctrl Pts',(35.6555077526845,40.312500006828,-35.6555077526845));
#7011=CARTESIAN_POINT('Ctrl Pts',(42.1809185638422,40.1041666734946,-24.3531646875));
#7012=CARTESIAN_POINT('Ctrl Pts',(48.706329375,39.8958333401613,-13.0508216223155));
#7013=CARTESIAN_POINT('Ctrl Pts',(48.706329375,39.687500006828,1.293339198242E-14));
#7014=CARTESIAN_POINT('Ctrl Pts',(48.706329375,39.4791666734946,13.0508216223155));
#7015=CARTESIAN_POINT('Ctrl Pts',(42.1809185638422,39.2708333401613,24.3531646875));
#7016=CARTESIAN_POINT('Ctrl Pts',(35.6555077526845,39.062500006828,35.6555077526845));
#7017=CARTESIAN_POINT('Ctrl Pts',(24.3531646875,38.8541666734946,42.1809185638422));
#7018=CARTESIAN_POINT('Ctrl Pts',(13.0508216223155,38.6458333401613,48.706329375));
#7019=CARTESIAN_POINT('Ctrl Pts',(-9.95098946405443E-15,38.437500006828,
48.706329375));
#7020=CARTESIAN_POINT('Ctrl Pts',(-13.0508216223155,38.2291666734946,48.706329375));
#7021=CARTESIAN_POINT('Ctrl Pts',(-24.3531646875,38.0208333401613,42.1809185638423));
#7022=CARTESIAN_POINT('Ctrl Pts',(-35.6555077526845,37.812500006828,35.6555077526845));
#7023=CARTESIAN_POINT('Ctrl Pts',(-42.1809185638422,37.6041666734946,24.3531646875));
#7024=CARTESIAN_POINT('Ctrl Pts',(-48.706329375,37.3958333401613,13.0508216223155));
#7025=CARTESIAN_POINT('Ctrl Pts',(-48.706329375,37.187500006828,-1.8898197019151E-14));
#7026=CARTESIAN_POINT('Ctrl Pts',(-48.706329375,36.9791666734946,-13.0508216223155));
#7027=CARTESIAN_POINT('Ctrl Pts',(-42.1809185638422,36.7708333401613,-24.3531646875));
#7028=CARTESIAN_POINT('Ctrl Pts',(-35.6555077526845,36.562500006828,-35.6555077526845));
#7029=CARTESIAN_POINT('Ctrl Pts',(-24.3531646875,36.3541666734946,-42.1809185638423));
#7030=CARTESIAN_POINT('Ctrl Pts',(-13.0508216223155,36.1458333401613,-48.706329375));
#7031=CARTESIAN_POINT('Ctrl Pts',(1.59157945007855E-14,35.937500006828,
-48.706329375));
#7032=CARTESIAN_POINT('Ctrl Pts',(13.0508216223155,35.7291666734946,-48.706329375));
#7033=CARTESIAN_POINT('Ctrl Pts',(24.3531646875,35.5208333401613,-42.1809185638422));
#7034=CARTESIAN_POINT('Ctrl Pts',(35.6555077526845,35.312500006828,-35.6555077526845));
#7035=CARTESIAN_POINT('Ctrl Pts',(42.1809185638422,35.1041666734946,-24.3531646875));
#7036=CARTESIAN_POINT('Ctrl Pts',(48.706329375,34.8958333401613,-13.0508216223155));
#7037=CARTESIAN_POINT('Ctrl Pts',(48.706329375,34.687500006828,1.293339198242E-14));
#7038=CARTESIAN_POINT('Ctrl Pts',(48.706329375,34.4791666734946,13.0508216223155));
#7039=CARTESIAN_POINT('Ctrl Pts',(42.1809185638422,34.2708333401613,24.3531646875));
#7040=CARTESIAN_POINT('Ctrl Pts',(35.6555077526845,34.062500006828,35.6555077526845));
#7041=CARTESIAN_POINT('Ctrl Pts',(24.3531646875,33.8541666734946,42.1809185638422));
#7042=CARTESIAN_POINT('Ctrl Pts',(13.0508216223155,33.6458333401613,48.706329375));
#7043=CARTESIAN_POINT('Ctrl Pts',(-9.95098946405443E-15,33.437500006828,
48.706329375));
#7044=CARTESIAN_POINT('Ctrl Pts',(-13.0508216223155,33.2291666734946,48.706329375));
#7045=CARTESIAN_POINT('Ctrl Pts',(-24.3531646875,33.0208333401613,42.1809185638423));
#7046=CARTESIAN_POINT('Ctrl Pts',(-35.6555077526845,32.812500006828,35.6555077526845));
#7047=CARTESIAN_POINT('Ctrl Pts',(-42.1809185638422,32.6041666734946,24.3531646875));
#7048=CARTESIAN_POINT('Ctrl Pts',(-48.706329375,32.3958333401613,13.0508216223155));
#7049=CARTESIAN_POINT('Ctrl Pts',(-48.706329375,32.187500006828,-1.8898197019151E-14));
#7050=CARTESIAN_POINT('Ctrl Pts',(-48.706329375,31.9791666734946,-13.0508216223155));
#7051=CARTESIAN_POINT('Ctrl Pts',(-42.1809185638422,31.7708333401613,-24.3531646875));
#7052=CARTESIAN_POINT('Ctrl Pts',(-35.6555077526845,31.562500006828,-35.6555077526845));
#7053=CARTESIAN_POINT('Ctrl Pts',(-24.3531646875,31.3541666734946,-42.1809185638423));
#7054=CARTESIAN_POINT('Ctrl Pts',(-13.0508216223155,31.1458333401613,-48.706329375));
#7055=CARTESIAN_POINT('Ctrl Pts',(1.59157945007855E-14,30.937500006828,
-48.706329375));
#7056=CARTESIAN_POINT('Ctrl Pts',(13.0508216223155,30.7291666734946,-48.706329375));
#7057=CARTESIAN_POINT('Ctrl Pts',(24.3531646875,30.5208333401613,-42.1809185638422));
#7058=CARTESIAN_POINT('Ctrl Pts',(35.6555077526845,30.312500006828,-35.6555077526845));
#7059=CARTESIAN_POINT('Ctrl Pts',(42.1809185638422,30.1041666734946,-24.3531646875));
#7060=CARTESIAN_POINT('Ctrl Pts',(48.706329375,29.8958333401613,-13.0508216223155));
#7061=CARTESIAN_POINT('Ctrl Pts',(48.706329375,29.687500006828,1.293339198242E-14));
#7062=CARTESIAN_POINT('Ctrl Pts',(48.706329375,29.4791666734946,13.0508216223155));
#7063=CARTESIAN_POINT('Ctrl Pts',(42.1809185638422,29.2708333401613,24.3531646875));
#7064=CARTESIAN_POINT('Ctrl Pts',(35.6555077526845,29.062500006828,35.6555077526845));
#7065=CARTESIAN_POINT('Ctrl Pts',(24.3531646875,28.8541666734946,42.1809185638422));
#7066=CARTESIAN_POINT('Ctrl Pts',(13.0508216223155,28.6458333401613,48.706329375));
#7067=CARTESIAN_POINT('Ctrl Pts',(-9.95098946405443E-15,28.437500006828,
48.706329375));
#7068=CARTESIAN_POINT('Ctrl Pts',(-13.0508216223155,28.2291666734946,48.706329375));
#7069=CARTESIAN_POINT('Ctrl Pts',(-24.3531646875,28.0208333401613,42.1809185638423));
#7070=CARTESIAN_POINT('Ctrl Pts',(-35.6555077526845,27.812500006828,35.6555077526845));
#7071=CARTESIAN_POINT('Ctrl Pts',(-42.1809185638422,27.6041666734946,24.3531646875));
#7072=CARTESIAN_POINT('Ctrl Pts',(-48.706329375,27.3958333401613,13.0508216223155));
#7073=CARTESIAN_POINT('Ctrl Pts',(-48.706329375,27.187500006828,-1.8898197019151E-14));
#7074=CARTESIAN_POINT('',(3.61292728433799,45.8792520480092,-48.5721450795008));
#7075=CARTESIAN_POINT('',(48.5134353784345,44.7574536451604,-4.33048599679671));
#7076=CARTESIAN_POINT('Ctrl Pts',(3.61292728433799,45.8792520480092,-48.5721450795008));
#7077=CARTESIAN_POINT('Ctrl Pts',(14.7133549689477,45.6985216017706,-47.7464652997852));
#7078=CARTESIAN_POINT('Ctrl Pts',(24.3531646875,45.5208333401613,-42.1809185638422));
#7079=CARTESIAN_POINT('Ctrl Pts',(35.6555077526845,45.312500006828,-35.6555077526845));
#7080=CARTESIAN_POINT('Ctrl Pts',(42.1809185638422,45.1041666734946,-24.3531646875));
#7081=CARTESIAN_POINT('Ctrl Pts',(47.5573898704235,44.9325149229327,-15.0408432190651));
#7082=CARTESIAN_POINT('Ctrl Pts',(48.5134353784345,44.7574536451604,-4.33048599679671));
#7083=CARTESIAN_POINT('Origin',(-4513.8089981458,7998.28355101971,-4.33048637721644));
#7084=CARTESIAN_POINT('Ctrl Pts',(3.61292728433799,44.3132892765089,-45.8578974271399));
#7085=CARTESIAN_POINT('Ctrl Pts',(3.61292728433796,44.4468822859549,-46.089460636719));
#7086=CARTESIAN_POINT('Ctrl Pts',(3.61292728433805,44.7140705280012,-46.5525857733052));
#7087=CARTESIAN_POINT('Ctrl Pts',(3.61292728433797,44.9812630238616,-47.0157084557285));
#7088=CARTESIAN_POINT('Ctrl Pts',(3.61292728433797,45.3696539378594,-47.6888965792834));
#7089=CARTESIAN_POINT('Ctrl Pts',(3.61292728433799,45.624451287085,-48.1305218136162));
#7090=CARTESIAN_POINT('Ctrl Pts',(3.61292728433799,45.8792520480092,-48.5721450795008));
#7091=CARTESIAN_POINT('Ctrl Pts',(-46.,55.6250000136559,0.));
#7092=CARTESIAN_POINT('Ctrl Pts',(-46.,55.4166666803226,-12.3256628518316));
#7093=CARTESIAN_POINT('Ctrl Pts',(-39.8371685740842,55.2083333469893,-23.));
#7094=CARTESIAN_POINT('Ctrl Pts',(-33.6743371481684,55.0000000136559,-33.6743371481684));
#7095=CARTESIAN_POINT('Ctrl Pts',(-23.,54.7916666803226,-39.8371685740842));
#7096=CARTESIAN_POINT('Ctrl Pts',(-12.3256628518317,54.5833333469893,-46.));
#7097=CARTESIAN_POINT('Ctrl Pts',(-2.81668763803891E-15,54.3750000136559,
-46.));
#7098=CARTESIAN_POINT('Ctrl Pts',(12.3256628518316,54.1666666803226,-46.));
#7099=CARTESIAN_POINT('Ctrl Pts',(23.,53.9583333469893,-39.8371685740842));
#7100=CARTESIAN_POINT('Ctrl Pts',(33.6743371481683,53.7500000136559,-33.6743371481684));
#7101=CARTESIAN_POINT('Ctrl Pts',(39.8371685740842,53.5416666803226,-23.));
#7102=CARTESIAN_POINT('Ctrl Pts',(46.,53.3333333469893,-12.3256628518317));
#7103=CARTESIAN_POINT('Ctrl Pts',(46.,53.1250000136559,-5.63337527607782E-15));
#7104=CARTESIAN_POINT('Ctrl Pts',(46.,52.9166666803226,12.3256628518316));
#7105=CARTESIAN_POINT('Ctrl Pts',(39.8371685740842,52.7083333469893,23.));
#7106=CARTESIAN_POINT('Ctrl Pts',(33.6743371481684,52.5000000136559,33.6743371481683));
#7107=CARTESIAN_POINT('Ctrl Pts',(23.,52.2916666803226,39.8371685740842));
#7108=CARTESIAN_POINT('Ctrl Pts',(12.3256628518317,52.0833333469893,46.));
#7109=CARTESIAN_POINT('Ctrl Pts',(8.45006291411674E-15,51.8750000136559,
46.));
#7110=CARTESIAN_POINT('Ctrl Pts',(-12.3256628518316,51.6666666803226,46.));
#7111=CARTESIAN_POINT('Ctrl Pts',(-23.,51.4583333469893,39.8371685740842));
#7112=CARTESIAN_POINT('Ctrl Pts',(-33.6743371481683,51.2500000136559,33.6743371481684));
#7113=CARTESIAN_POINT('Ctrl Pts',(-39.8371685740842,51.0416666803226,23.));
#7114=CARTESIAN_POINT('Ctrl Pts',(-46.,50.8333333469893,12.3256628518317));
#7115=CARTESIAN_POINT('Ctrl Pts',(-46.,50.6250000136559,0.));
#7116=CARTESIAN_POINT('Ctrl Pts',(-46.,50.4166666803226,-12.3256628518316));
#7117=CARTESIAN_POINT('Ctrl Pts',(-39.8371685740842,50.2083333469893,-23.));
#7118=CARTESIAN_POINT('Ctrl Pts',(-33.6743371481684,50.0000000136559,-33.6743371481684));
#7119=CARTESIAN_POINT('Ctrl Pts',(-23.,49.7916666803226,-39.8371685740842));
#7120=CARTESIAN_POINT('Ctrl Pts',(-12.3256628518317,49.5833333469893,-46.));
#7121=CARTESIAN_POINT('Ctrl Pts',(-2.81668763803891E-15,49.3750000136559,
-46.));
#7122=CARTESIAN_POINT('Ctrl Pts',(12.3256628518316,49.1666666803226,-46.));
#7123=CARTESIAN_POINT('Ctrl Pts',(23.,48.9583333469893,-39.8371685740842));
#7124=CARTESIAN_POINT('Ctrl Pts',(33.6743371481683,48.7500000136559,-33.6743371481684));
#7125=CARTESIAN_POINT('Ctrl Pts',(39.8371685740842,48.5416666803226,-23.));
#7126=CARTESIAN_POINT('Ctrl Pts',(46.,48.3333333469893,-12.3256628518317));
#7127=CARTESIAN_POINT('Ctrl Pts',(46.,48.1250000136559,-5.63337527607782E-15));
#7128=CARTESIAN_POINT('Ctrl Pts',(46.,47.9166666803226,12.3256628518316));
#7129=CARTESIAN_POINT('Ctrl Pts',(39.8371685740842,47.7083333469893,23.));
#7130=CARTESIAN_POINT('Ctrl Pts',(33.6743371481684,47.5000000136559,33.6743371481683));
#7131=CARTESIAN_POINT('Ctrl Pts',(23.,47.2916666803226,39.8371685740842));
#7132=CARTESIAN_POINT('Ctrl Pts',(12.3256628518317,47.0833333469893,46.));
#7133=CARTESIAN_POINT('Ctrl Pts',(8.45006291411674E-15,46.8750000136559,
46.));
#7134=CARTESIAN_POINT('Ctrl Pts',(-12.3256628518316,46.6666666803226,46.));
#7135=CARTESIAN_POINT('Ctrl Pts',(-23.,46.4583333469893,39.8371685740842));
#7136=CARTESIAN_POINT('Ctrl Pts',(-33.6743371481683,46.2500000136559,33.6743371481684));
#7137=CARTESIAN_POINT('Ctrl Pts',(-39.8371685740842,46.0416666803226,23.));
#7138=CARTESIAN_POINT('Ctrl Pts',(-46.,45.8333333469892,12.3256628518317));
#7139=CARTESIAN_POINT('Ctrl Pts',(-46.,45.6250000136559,0.));
#7140=CARTESIAN_POINT('Ctrl Pts',(-46.,45.4166666803226,-12.3256628518316));
#7141=CARTESIAN_POINT('Ctrl Pts',(-39.8371685740842,45.2083333469893,-23.));
#7142=CARTESIAN_POINT('Ctrl Pts',(-33.6743371481684,45.0000000136559,-33.6743371481684));
#7143=CARTESIAN_POINT('Ctrl Pts',(-23.,44.7916666803226,-39.8371685740842));
#7144=CARTESIAN_POINT('Ctrl Pts',(-12.3256628518317,44.5833333469893,-46.));
#7145=CARTESIAN_POINT('Ctrl Pts',(-2.81668763803891E-15,44.3750000136559,
-46.));
#7146=CARTESIAN_POINT('Ctrl Pts',(12.3256628518316,44.1666666803226,-46.));
#7147=CARTESIAN_POINT('Ctrl Pts',(23.,43.9583333469893,-39.8371685740842));
#7148=CARTESIAN_POINT('Ctrl Pts',(33.6743371481683,43.7500000136559,-33.6743371481684));
#7149=CARTESIAN_POINT('Ctrl Pts',(39.8371685740842,43.5416666803226,-23.));
#7150=CARTESIAN_POINT('Ctrl Pts',(46.,43.3333333469893,-12.3256628518317));
#7151=CARTESIAN_POINT('Ctrl Pts',(46.,43.1250000136559,-5.63337527607782E-15));
#7152=CARTESIAN_POINT('Ctrl Pts',(46.,42.9166666803226,12.3256628518316));
#7153=CARTESIAN_POINT('Ctrl Pts',(39.8371685740842,42.7083333469893,23.));
#7154=CARTESIAN_POINT('Ctrl Pts',(33.6743371481684,42.5000000136559,33.6743371481683));
#7155=CARTESIAN_POINT('Ctrl Pts',(23.,42.2916666803226,39.8371685740842));
#7156=CARTESIAN_POINT('Ctrl Pts',(12.3256628518317,42.0833333469893,46.));
#7157=CARTESIAN_POINT('Ctrl Pts',(8.45006291411674E-15,41.8750000136559,
46.));
#7158=CARTESIAN_POINT('Ctrl Pts',(-12.3256628518316,41.6666666803226,46.));
#7159=CARTESIAN_POINT('Ctrl Pts',(-23.,41.4583333469893,39.8371685740842));
#7160=CARTESIAN_POINT('Ctrl Pts',(-33.6743371481683,41.2500000136559,33.6743371481684));
#7161=CARTESIAN_POINT('Ctrl Pts',(-39.8371685740842,41.0416666803226,23.));
#7162=CARTESIAN_POINT('Ctrl Pts',(-46.,40.8333333469893,12.3256628518317));
#7163=CARTESIAN_POINT('Ctrl Pts',(-46.,40.6250000136559,0.));
#7164=CARTESIAN_POINT('Ctrl Pts',(-46.,40.4166666803226,-12.3256628518316));
#7165=CARTESIAN_POINT('Ctrl Pts',(-39.8371685740842,40.2083333469893,-23.));
#7166=CARTESIAN_POINT('Ctrl Pts',(-33.6743371481684,40.0000000136559,-33.6743371481684));
#7167=CARTESIAN_POINT('Ctrl Pts',(-23.,39.7916666803226,-39.8371685740842));
#7168=CARTESIAN_POINT('Ctrl Pts',(-12.3256628518317,39.5833333469893,-46.));
#7169=CARTESIAN_POINT('Ctrl Pts',(-2.81668763803891E-15,39.3750000136559,
-46.));
#7170=CARTESIAN_POINT('Ctrl Pts',(12.3256628518316,39.1666666803226,-46.));
#7171=CARTESIAN_POINT('Ctrl Pts',(23.,38.9583333469893,-39.8371685740842));
#7172=CARTESIAN_POINT('Ctrl Pts',(33.6743371481683,38.7500000136559,-33.6743371481684));
#7173=CARTESIAN_POINT('Ctrl Pts',(39.8371685740842,38.5416666803226,-23.));
#7174=CARTESIAN_POINT('Ctrl Pts',(46.,38.3333333469893,-12.3256628518317));
#7175=CARTESIAN_POINT('Ctrl Pts',(46.,38.1250000136559,-5.63337527607782E-15));
#7176=CARTESIAN_POINT('Ctrl Pts',(46.,37.9166666803226,12.3256628518316));
#7177=CARTESIAN_POINT('Ctrl Pts',(39.8371685740842,37.7083333469893,23.));
#7178=CARTESIAN_POINT('Ctrl Pts',(33.6743371481684,37.5000000136559,33.6743371481683));
#7179=CARTESIAN_POINT('Ctrl Pts',(23.,37.2916666803226,39.8371685740842));
#7180=CARTESIAN_POINT('Ctrl Pts',(12.3256628518317,37.0833333469893,46.));
#7181=CARTESIAN_POINT('Ctrl Pts',(8.45006291411674E-15,36.8750000136559,
46.));
#7182=CARTESIAN_POINT('Ctrl Pts',(-12.3256628518316,36.6666666803226,46.));
#7183=CARTESIAN_POINT('Ctrl Pts',(-23.,36.4583333469893,39.8371685740842));
#7184=CARTESIAN_POINT('Ctrl Pts',(-33.6743371481683,36.2500000136559,33.6743371481684));
#7185=CARTESIAN_POINT('Ctrl Pts',(-39.8371685740842,36.0416666803226,23.));
#7186=CARTESIAN_POINT('Ctrl Pts',(-46.,35.8333333469893,12.3256628518317));
#7187=CARTESIAN_POINT('Ctrl Pts',(-46.,35.6250000136559,0.));
#7188=CARTESIAN_POINT('Ctrl Pts',(-46.,35.4166666803226,-12.3256628518316));
#7189=CARTESIAN_POINT('Ctrl Pts',(-39.8371685740842,35.2083333469893,-23.));
#7190=CARTESIAN_POINT('Ctrl Pts',(-33.6743371481684,35.0000000136559,-33.6743371481684));
#7191=CARTESIAN_POINT('Ctrl Pts',(-23.,34.7916666803226,-39.8371685740842));
#7192=CARTESIAN_POINT('Ctrl Pts',(-12.3256628518317,34.5833333469893,-46.));
#7193=CARTESIAN_POINT('Ctrl Pts',(-2.81668763803891E-15,34.3750000136559,
-46.));
#7194=CARTESIAN_POINT('Ctrl Pts',(12.3256628518316,34.1666666803226,-46.));
#7195=CARTESIAN_POINT('Ctrl Pts',(23.,33.9583333469893,-39.8371685740842));
#7196=CARTESIAN_POINT('Ctrl Pts',(33.6743371481683,33.7500000136559,-33.6743371481684));
#7197=CARTESIAN_POINT('Ctrl Pts',(39.8371685740842,33.5416666803226,-23.));
#7198=CARTESIAN_POINT('Ctrl Pts',(46.,33.3333333469893,-12.3256628518317));
#7199=CARTESIAN_POINT('Ctrl Pts',(46.,33.1250000136559,-5.63337527607782E-15));
#7200=CARTESIAN_POINT('Ctrl Pts',(46.,32.9166666803226,12.3256628518316));
#7201=CARTESIAN_POINT('Ctrl Pts',(39.8371685740842,32.7083333469893,23.));
#7202=CARTESIAN_POINT('Ctrl Pts',(33.6743371481684,32.5000000136559,33.6743371481683));
#7203=CARTESIAN_POINT('Ctrl Pts',(23.,32.2916666803226,39.8371685740842));
#7204=CARTESIAN_POINT('Ctrl Pts',(12.3256628518317,32.0833333469893,46.));
#7205=CARTESIAN_POINT('Ctrl Pts',(8.45006291411674E-15,31.8750000136559,
46.));
#7206=CARTESIAN_POINT('Ctrl Pts',(-12.3256628518316,31.6666666803226,46.));
#7207=CARTESIAN_POINT('Ctrl Pts',(-23.,31.4583333469893,39.8371685740842));
#7208=CARTESIAN_POINT('Ctrl Pts',(-33.6743371481683,31.2500000136559,33.6743371481684));
#7209=CARTESIAN_POINT('Ctrl Pts',(-39.8371685740842,31.0416666803226,23.));
#7210=CARTESIAN_POINT('Ctrl Pts',(-46.,30.8333333469893,12.3256628518317));
#7211=CARTESIAN_POINT('Ctrl Pts',(-46.,30.6250000136559,0.));
#7212=CARTESIAN_POINT('Ctrl Pts',(-46.,30.4166666803226,-12.3256628518316));
#7213=CARTESIAN_POINT('Ctrl Pts',(-39.8371685740842,30.2083333469893,-23.));
#7214=CARTESIAN_POINT('Ctrl Pts',(-33.6743371481684,30.0000000136559,-33.6743371481684));
#7215=CARTESIAN_POINT('Ctrl Pts',(-23.,29.7916666803226,-39.8371685740842));
#7216=CARTESIAN_POINT('Ctrl Pts',(-12.3256628518317,29.5833333469893,-46.));
#7217=CARTESIAN_POINT('Ctrl Pts',(-2.81668763803891E-15,29.3750000136559,
-46.));
#7218=CARTESIAN_POINT('Ctrl Pts',(12.3256628518316,29.1666666803226,-46.));
#7219=CARTESIAN_POINT('Ctrl Pts',(23.,28.9583333469893,-39.8371685740842));
#7220=CARTESIAN_POINT('Ctrl Pts',(33.6743371481683,28.7500000136559,-33.6743371481684));
#7221=CARTESIAN_POINT('Ctrl Pts',(39.8371685740842,28.5416666803226,-23.));
#7222=CARTESIAN_POINT('Ctrl Pts',(46.,28.3333333469893,-12.3256628518317));
#7223=CARTESIAN_POINT('Ctrl Pts',(46.,28.1250000136559,-5.63337527607782E-15));
#7224=CARTESIAN_POINT('Ctrl Pts',(46.,27.9166666803226,12.3256628518316));
#7225=CARTESIAN_POINT('Ctrl Pts',(39.8371685740842,27.7083333469893,23.));
#7226=CARTESIAN_POINT('Ctrl Pts',(33.6743371481684,27.5000000136559,33.6743371481683));
#7227=CARTESIAN_POINT('Ctrl Pts',(23.,27.2916666803226,39.8371685740842));
#7228=CARTESIAN_POINT('Ctrl Pts',(12.3256628518317,27.0833333469893,46.));
#7229=CARTESIAN_POINT('Ctrl Pts',(8.45006291411674E-15,26.8750000136559,
46.));
#7230=CARTESIAN_POINT('Ctrl Pts',(-12.3256628518316,26.6666666803226,46.));
#7231=CARTESIAN_POINT('Ctrl Pts',(-23.,26.4583333469893,39.8371685740842));
#7232=CARTESIAN_POINT('Ctrl Pts',(-33.6743371481683,26.2500000136559,33.6743371481684));
#7233=CARTESIAN_POINT('Ctrl Pts',(-39.8371685740842,26.0416666803226,23.));
#7234=CARTESIAN_POINT('Ctrl Pts',(-46.,25.8333333469893,12.3256628518317));
#7235=CARTESIAN_POINT('Ctrl Pts',(-46.,25.6250000136559,0.));
#7236=CARTESIAN_POINT('Ctrl Pts',(-48.706329375,57.187500006828,-1.8898197019151E-14));
#7237=CARTESIAN_POINT('Ctrl Pts',(-48.706329375,56.9791666734946,-13.0508216223155));
#7238=CARTESIAN_POINT('Ctrl Pts',(-42.1809185638422,56.7708333401613,-24.3531646875));
#7239=CARTESIAN_POINT('Ctrl Pts',(-35.6555077526845,56.562500006828,-35.6555077526845));
#7240=CARTESIAN_POINT('Ctrl Pts',(-24.3531646875,56.3541666734946,-42.1809185638423));
#7241=CARTESIAN_POINT('Ctrl Pts',(-13.0508216223155,56.1458333401613,-48.706329375));
#7242=CARTESIAN_POINT('Ctrl Pts',(1.59157945007855E-14,55.937500006828,
-48.706329375));
#7243=CARTESIAN_POINT('Ctrl Pts',(13.0508216223155,55.7291666734946,-48.706329375));
#7244=CARTESIAN_POINT('Ctrl Pts',(24.3531646875,55.5208333401613,-42.1809185638422));
#7245=CARTESIAN_POINT('Ctrl Pts',(35.6555077526845,55.312500006828,-35.6555077526845));
#7246=CARTESIAN_POINT('Ctrl Pts',(42.1809185638422,55.1041666734946,-24.3531646875));
#7247=CARTESIAN_POINT('Ctrl Pts',(48.706329375,54.8958333401613,-13.0508216223155));
#7248=CARTESIAN_POINT('Ctrl Pts',(48.706329375,54.687500006828,1.293339198242E-14));
#7249=CARTESIAN_POINT('Ctrl Pts',(48.706329375,54.4791666734946,13.0508216223155));
#7250=CARTESIAN_POINT('Ctrl Pts',(42.1809185638422,54.2708333401613,24.3531646875));
#7251=CARTESIAN_POINT('Ctrl Pts',(35.6555077526845,54.062500006828,35.6555077526845));
#7252=CARTESIAN_POINT('Ctrl Pts',(24.3531646875,53.8541666734946,42.1809185638422));
#7253=CARTESIAN_POINT('Ctrl Pts',(13.0508216223155,53.6458333401613,48.706329375));
#7254=CARTESIAN_POINT('Ctrl Pts',(-9.95098946405443E-15,53.437500006828,
48.706329375));
#7255=CARTESIAN_POINT('Ctrl Pts',(-13.0508216223155,53.2291666734946,48.706329375));
#7256=CARTESIAN_POINT('Ctrl Pts',(-24.3531646875,53.0208333401613,42.1809185638423));
#7257=CARTESIAN_POINT('Ctrl Pts',(-35.6555077526845,52.812500006828,35.6555077526845));
#7258=CARTESIAN_POINT('Ctrl Pts',(-42.1809185638422,52.6041666734946,24.3531646875));
#7259=CARTESIAN_POINT('Ctrl Pts',(-48.706329375,52.3958333401613,13.0508216223155));
#7260=CARTESIAN_POINT('Ctrl Pts',(-48.706329375,52.187500006828,-1.8898197019151E-14));
#7261=CARTESIAN_POINT('Ctrl Pts',(-48.706329375,51.9791666734946,-13.0508216223155));
#7262=CARTESIAN_POINT('Ctrl Pts',(-42.1809185638422,51.7708333401613,-24.3531646875));
#7263=CARTESIAN_POINT('Ctrl Pts',(-35.6555077526845,51.562500006828,-35.6555077526845));
#7264=CARTESIAN_POINT('Ctrl Pts',(-24.3531646875,51.3541666734946,-42.1809185638423));
#7265=CARTESIAN_POINT('Ctrl Pts',(-13.0508216223155,51.1458333401613,-48.706329375));
#7266=CARTESIAN_POINT('Ctrl Pts',(1.59157945007855E-14,50.937500006828,
-48.706329375));
#7267=CARTESIAN_POINT('Ctrl Pts',(13.0508216223155,50.7291666734946,-48.706329375));
#7268=CARTESIAN_POINT('Ctrl Pts',(24.3531646875,50.5208333401613,-42.1809185638422));
#7269=CARTESIAN_POINT('Ctrl Pts',(35.6555077526845,50.312500006828,-35.6555077526845));
#7270=CARTESIAN_POINT('Ctrl Pts',(42.1809185638422,50.1041666734946,-24.3531646875));
#7271=CARTESIAN_POINT('Ctrl Pts',(48.706329375,49.8958333401613,-13.0508216223155));
#7272=CARTESIAN_POINT('Ctrl Pts',(48.706329375,49.687500006828,1.293339198242E-14));
#7273=CARTESIAN_POINT('Ctrl Pts',(48.706329375,49.4791666734946,13.0508216223155));
#7274=CARTESIAN_POINT('Ctrl Pts',(42.1809185638422,49.2708333401613,24.3531646875));
#7275=CARTESIAN_POINT('Ctrl Pts',(35.6555077526845,49.062500006828,35.6555077526845));
#7276=CARTESIAN_POINT('Ctrl Pts',(24.3531646875,48.8541666734946,42.1809185638422));
#7277=CARTESIAN_POINT('Ctrl Pts',(13.0508216223155,48.6458333401613,48.706329375));
#7278=CARTESIAN_POINT('Ctrl Pts',(-9.95098946405443E-15,48.437500006828,
48.706329375));
#7279=CARTESIAN_POINT('Ctrl Pts',(-13.0508216223155,48.2291666734946,48.706329375));
#7280=CARTESIAN_POINT('Ctrl Pts',(-24.3531646875,48.0208333401613,42.1809185638423));
#7281=CARTESIAN_POINT('Ctrl Pts',(-35.6555077526845,47.812500006828,35.6555077526845));
#7282=CARTESIAN_POINT('Ctrl Pts',(-42.1809185638422,47.6041666734946,24.3531646875));
#7283=CARTESIAN_POINT('Ctrl Pts',(-48.706329375,47.3958333401613,13.0508216223155));
#7284=CARTESIAN_POINT('Ctrl Pts',(-48.706329375,47.187500006828,-1.8898197019151E-14));
#7285=CARTESIAN_POINT('Ctrl Pts',(-48.706329375,46.9791666734946,-13.0508216223155));
#7286=CARTESIAN_POINT('Ctrl Pts',(-42.1809185638422,46.7708333401613,-24.3531646875));
#7287=CARTESIAN_POINT('Ctrl Pts',(-35.6555077526845,46.562500006828,-35.6555077526845));
#7288=CARTESIAN_POINT('Ctrl Pts',(-24.3531646875,46.3541666734946,-42.1809185638423));
#7289=CARTESIAN_POINT('Ctrl Pts',(-13.0508216223155,46.1458333401613,-48.706329375));
#7290=CARTESIAN_POINT('Ctrl Pts',(1.59157945007855E-14,45.937500006828,
-48.706329375));
#7291=CARTESIAN_POINT('Ctrl Pts',(13.0508216223155,45.7291666734946,-48.706329375));
#7292=CARTESIAN_POINT('Ctrl Pts',(24.3531646875,45.5208333401613,-42.1809185638422));
#7293=CARTESIAN_POINT('Ctrl Pts',(35.6555077526845,45.312500006828,-35.6555077526845));
#7294=CARTESIAN_POINT('Ctrl Pts',(42.1809185638422,45.1041666734946,-24.3531646875));
#7295=CARTESIAN_POINT('Ctrl Pts',(48.706329375,44.8958333401613,-13.0508216223155));
#7296=CARTESIAN_POINT('Ctrl Pts',(48.706329375,44.687500006828,1.293339198242E-14));
#7297=CARTESIAN_POINT('Ctrl Pts',(48.706329375,44.4791666734946,13.0508216223155));
#7298=CARTESIAN_POINT('Ctrl Pts',(42.1809185638422,44.2708333401613,24.3531646875));
#7299=CARTESIAN_POINT('Ctrl Pts',(35.6555077526845,44.062500006828,35.6555077526845));
#7300=CARTESIAN_POINT('Ctrl Pts',(24.3531646875,43.8541666734946,42.1809185638422));
#7301=CARTESIAN_POINT('Ctrl Pts',(13.0508216223155,43.6458333401613,48.706329375));
#7302=CARTESIAN_POINT('Ctrl Pts',(-9.95098946405443E-15,43.437500006828,
48.706329375));
#7303=CARTESIAN_POINT('Ctrl Pts',(-13.0508216223155,43.2291666734946,48.706329375));
#7304=CARTESIAN_POINT('Ctrl Pts',(-24.3531646875,43.0208333401613,42.1809185638423));
#7305=CARTESIAN_POINT('Ctrl Pts',(-35.6555077526845,42.812500006828,35.6555077526845));
#7306=CARTESIAN_POINT('Ctrl Pts',(-42.1809185638422,42.6041666734946,24.3531646875));
#7307=CARTESIAN_POINT('Ctrl Pts',(-48.706329375,42.3958333401613,13.0508216223155));
#7308=CARTESIAN_POINT('Ctrl Pts',(-48.706329375,42.187500006828,-1.8898197019151E-14));
#7309=CARTESIAN_POINT('Ctrl Pts',(-48.706329375,41.9791666734946,-13.0508216223155));
#7310=CARTESIAN_POINT('Ctrl Pts',(-42.1809185638422,41.7708333401613,-24.3531646875));
#7311=CARTESIAN_POINT('Ctrl Pts',(-35.6555077526845,41.562500006828,-35.6555077526845));
#7312=CARTESIAN_POINT('Ctrl Pts',(-24.3531646875,41.3541666734946,-42.1809185638423));
#7313=CARTESIAN_POINT('Ctrl Pts',(-13.0508216223155,41.1458333401613,-48.706329375));
#7314=CARTESIAN_POINT('Ctrl Pts',(1.59157945007855E-14,40.937500006828,
-48.706329375));
#7315=CARTESIAN_POINT('Ctrl Pts',(13.0508216223155,40.7291666734946,-48.706329375));
#7316=CARTESIAN_POINT('Ctrl Pts',(24.3531646875,40.5208333401613,-42.1809185638422));
#7317=CARTESIAN_POINT('Ctrl Pts',(35.6555077526845,40.312500006828,-35.6555077526845));
#7318=CARTESIAN_POINT('Ctrl Pts',(42.1809185638422,40.1041666734946,-24.3531646875));
#7319=CARTESIAN_POINT('Ctrl Pts',(48.706329375,39.8958333401613,-13.0508216223155));
#7320=CARTESIAN_POINT('Ctrl Pts',(48.706329375,39.687500006828,1.293339198242E-14));
#7321=CARTESIAN_POINT('Ctrl Pts',(48.706329375,39.4791666734946,13.0508216223155));
#7322=CARTESIAN_POINT('Ctrl Pts',(42.1809185638422,39.2708333401613,24.3531646875));
#7323=CARTESIAN_POINT('Ctrl Pts',(35.6555077526845,39.062500006828,35.6555077526845));
#7324=CARTESIAN_POINT('Ctrl Pts',(24.3531646875,38.8541666734946,42.1809185638422));
#7325=CARTESIAN_POINT('Ctrl Pts',(13.0508216223155,38.6458333401613,48.706329375));
#7326=CARTESIAN_POINT('Ctrl Pts',(-9.95098946405443E-15,38.437500006828,
48.706329375));
#7327=CARTESIAN_POINT('Ctrl Pts',(-13.0508216223155,38.2291666734946,48.706329375));
#7328=CARTESIAN_POINT('Ctrl Pts',(-24.3531646875,38.0208333401613,42.1809185638423));
#7329=CARTESIAN_POINT('Ctrl Pts',(-35.6555077526845,37.812500006828,35.6555077526845));
#7330=CARTESIAN_POINT('Ctrl Pts',(-42.1809185638422,37.6041666734946,24.3531646875));
#7331=CARTESIAN_POINT('Ctrl Pts',(-48.706329375,37.3958333401613,13.0508216223155));
#7332=CARTESIAN_POINT('Ctrl Pts',(-48.706329375,37.187500006828,-1.8898197019151E-14));
#7333=CARTESIAN_POINT('Ctrl Pts',(-48.706329375,36.9791666734946,-13.0508216223155));
#7334=CARTESIAN_POINT('Ctrl Pts',(-42.1809185638422,36.7708333401613,-24.3531646875));
#7335=CARTESIAN_POINT('Ctrl Pts',(-35.6555077526845,36.562500006828,-35.6555077526845));
#7336=CARTESIAN_POINT('Ctrl Pts',(-24.3531646875,36.3541666734946,-42.1809185638423));
#7337=CARTESIAN_POINT('Ctrl Pts',(-13.0508216223155,36.1458333401613,-48.706329375));
#7338=CARTESIAN_POINT('Ctrl Pts',(1.59157945007855E-14,35.937500006828,
-48.706329375));
#7339=CARTESIAN_POINT('Ctrl Pts',(13.0508216223155,35.7291666734946,-48.706329375));
#7340=CARTESIAN_POINT('Ctrl Pts',(24.3531646875,35.5208333401613,-42.1809185638422));
#7341=CARTESIAN_POINT('Ctrl Pts',(35.6555077526845,35.312500006828,-35.6555077526845));
#7342=CARTESIAN_POINT('Ctrl Pts',(42.1809185638422,35.1041666734946,-24.3531646875));
#7343=CARTESIAN_POINT('Ctrl Pts',(48.706329375,34.8958333401613,-13.0508216223155));
#7344=CARTESIAN_POINT('Ctrl Pts',(48.706329375,34.687500006828,1.293339198242E-14));
#7345=CARTESIAN_POINT('Ctrl Pts',(48.706329375,34.4791666734946,13.0508216223155));
#7346=CARTESIAN_POINT('Ctrl Pts',(42.1809185638422,34.2708333401613,24.3531646875));
#7347=CARTESIAN_POINT('Ctrl Pts',(35.6555077526845,34.062500006828,35.6555077526845));
#7348=CARTESIAN_POINT('Ctrl Pts',(24.3531646875,33.8541666734946,42.1809185638422));
#7349=CARTESIAN_POINT('Ctrl Pts',(13.0508216223155,33.6458333401613,48.706329375));
#7350=CARTESIAN_POINT('Ctrl Pts',(-9.95098946405443E-15,33.437500006828,
48.706329375));
#7351=CARTESIAN_POINT('Ctrl Pts',(-13.0508216223155,33.2291666734946,48.706329375));
#7352=CARTESIAN_POINT('Ctrl Pts',(-24.3531646875,33.0208333401613,42.1809185638423));
#7353=CARTESIAN_POINT('Ctrl Pts',(-35.6555077526845,32.812500006828,35.6555077526845));
#7354=CARTESIAN_POINT('Ctrl Pts',(-42.1809185638422,32.6041666734946,24.3531646875));
#7355=CARTESIAN_POINT('Ctrl Pts',(-48.706329375,32.3958333401613,13.0508216223155));
#7356=CARTESIAN_POINT('Ctrl Pts',(-48.706329375,32.187500006828,-1.8898197019151E-14));
#7357=CARTESIAN_POINT('Ctrl Pts',(-48.706329375,31.9791666734946,-13.0508216223155));
#7358=CARTESIAN_POINT('Ctrl Pts',(-42.1809185638422,31.7708333401613,-24.3531646875));
#7359=CARTESIAN_POINT('Ctrl Pts',(-35.6555077526845,31.562500006828,-35.6555077526845));
#7360=CARTESIAN_POINT('Ctrl Pts',(-24.3531646875,31.3541666734946,-42.1809185638423));
#7361=CARTESIAN_POINT('Ctrl Pts',(-13.0508216223155,31.1458333401613,-48.706329375));
#7362=CARTESIAN_POINT('Ctrl Pts',(1.59157945007855E-14,30.937500006828,
-48.706329375));
#7363=CARTESIAN_POINT('Ctrl Pts',(13.0508216223155,30.7291666734946,-48.706329375));
#7364=CARTESIAN_POINT('Ctrl Pts',(24.3531646875,30.5208333401613,-42.1809185638422));
#7365=CARTESIAN_POINT('Ctrl Pts',(35.6555077526845,30.312500006828,-35.6555077526845));
#7366=CARTESIAN_POINT('Ctrl Pts',(42.1809185638422,30.1041666734946,-24.3531646875));
#7367=CARTESIAN_POINT('Ctrl Pts',(48.706329375,29.8958333401613,-13.0508216223155));
#7368=CARTESIAN_POINT('Ctrl Pts',(48.706329375,29.687500006828,1.293339198242E-14));
#7369=CARTESIAN_POINT('Ctrl Pts',(48.706329375,29.4791666734946,13.0508216223155));
#7370=CARTESIAN_POINT('Ctrl Pts',(42.1809185638422,29.2708333401613,24.3531646875));
#7371=CARTESIAN_POINT('Ctrl Pts',(35.6555077526845,29.062500006828,35.6555077526845));
#7372=CARTESIAN_POINT('Ctrl Pts',(24.3531646875,28.8541666734946,42.1809185638422));
#7373=CARTESIAN_POINT('Ctrl Pts',(13.0508216223155,28.6458333401613,48.706329375));
#7374=CARTESIAN_POINT('Ctrl Pts',(-9.95098946405443E-15,28.437500006828,
48.706329375));
#7375=CARTESIAN_POINT('Ctrl Pts',(-13.0508216223155,28.2291666734946,48.706329375));
#7376=CARTESIAN_POINT('Ctrl Pts',(-24.3531646875,28.0208333401613,42.1809185638423));
#7377=CARTESIAN_POINT('Ctrl Pts',(-35.6555077526845,27.812500006828,35.6555077526845));
#7378=CARTESIAN_POINT('Ctrl Pts',(-42.1809185638422,27.6041666734946,24.3531646875));
#7379=CARTESIAN_POINT('Ctrl Pts',(-48.706329375,27.3958333401613,13.0508216223155));
#7380=CARTESIAN_POINT('Ctrl Pts',(-48.706329375,27.187500006828,-1.8898197019151E-14));
#7381=CARTESIAN_POINT('',(48.5725845633798,44.6293483229262,3.60701400320328));
#7382=CARTESIAN_POINT('Ctrl Pts',(45.858362923034,43.0633913333999,3.60701400320327));
#7383=CARTESIAN_POINT('Ctrl Pts',(46.089925771934,43.1969849680263,3.60701400320324));
#7384=CARTESIAN_POINT('Ctrl Pts',(46.5530501979845,43.4641744416604,3.60701400320326));
#7385=CARTESIAN_POINT('Ctrl Pts',(47.0161721905706,43.7313681332063,3.60701400320324));
#7386=CARTESIAN_POINT('Ctrl Pts',(47.6893519862319,44.1197565257476,3.60701400320324));
#7387=CARTESIAN_POINT('Ctrl Pts',(48.1309692507095,44.3745507329179,3.60701400320328));
#7388=CARTESIAN_POINT('Ctrl Pts',(48.5725845633798,44.6293483229262,3.60701400320328));
#7389=CARTESIAN_POINT('',(3.61292728433797,43.4957479656467,48.5721450795008));
#7390=CARTESIAN_POINT('Ctrl Pts',(48.5725845633798,44.6293483229262,3.60701400320328));
#7391=CARTESIAN_POINT('Ctrl Pts',(47.7480251419552,44.4485714020251,14.7106532430575));
#7392=CARTESIAN_POINT('Ctrl Pts',(42.1809185638422,44.2708333401613,24.3531646875));
#7393=CARTESIAN_POINT('Ctrl Pts',(35.6555077526845,44.062500006828,35.6555077526845));
#7394=CARTESIAN_POINT('Ctrl Pts',(24.3531646875,43.8541666734946,42.1809185638422));
#7395=CARTESIAN_POINT('Ctrl Pts',(14.7133549689477,43.6764784118853,47.7464652997852));
#7396=CARTESIAN_POINT('Ctrl Pts',(3.61292728433797,43.4957479656467,48.5721450795008));
#7397=CARTESIAN_POINT('Ctrl Pts',(3.61292728433797,43.4957479656467,48.5721450795008));
#7398=CARTESIAN_POINT('Ctrl Pts',(3.61292728433797,43.3625660950884,48.3403451622818));
#7399=CARTESIAN_POINT('Ctrl Pts',(3.612927284338,43.2293911846469,48.1085412459393));
#7400=CARTESIAN_POINT('Ctrl Pts',(3.612927284338,42.9630558994543,47.6449250631479));
#7401=CARTESIAN_POINT('Ctrl Pts',(3.61292728433804,42.8298955244832,47.4131127965212));
#7402=CARTESIAN_POINT('Ctrl Pts',(3.61292728433804,42.6967427432646,47.1812961682826));
#7403=CARTESIAN_POINT('Ctrl Pts',(3.61292728433804,42.4433704509922,46.7401795055579));
#7404=CARTESIAN_POINT('Ctrl Pts',(3.61292728433798,42.1900256371662,46.2990470581854));
#7405=CARTESIAN_POINT('Ctrl Pts',(3.61292728433799,41.936710750803,45.8578974271399));
#7406=CARTESIAN_POINT('Ctrl Pts',(-46.,55.6250000136559,0.));
#7407=CARTESIAN_POINT('Ctrl Pts',(-46.,55.4166666803226,-12.3256628518316));
#7408=CARTESIAN_POINT('Ctrl Pts',(-39.8371685740842,55.2083333469893,-23.));
#7409=CARTESIAN_POINT('Ctrl Pts',(-33.6743371481684,55.0000000136559,-33.6743371481684));
#7410=CARTESIAN_POINT('Ctrl Pts',(-23.,54.7916666803226,-39.8371685740842));
#7411=CARTESIAN_POINT('Ctrl Pts',(-12.3256628518317,54.5833333469893,-46.));
#7412=CARTESIAN_POINT('Ctrl Pts',(-2.81668763803891E-15,54.3750000136559,
-46.));
#7413=CARTESIAN_POINT('Ctrl Pts',(12.3256628518316,54.1666666803226,-46.));
#7414=CARTESIAN_POINT('Ctrl Pts',(23.,53.9583333469893,-39.8371685740842));
#7415=CARTESIAN_POINT('Ctrl Pts',(33.6743371481683,53.7500000136559,-33.6743371481684));
#7416=CARTESIAN_POINT('Ctrl Pts',(39.8371685740842,53.5416666803226,-23.));
#7417=CARTESIAN_POINT('Ctrl Pts',(46.,53.3333333469893,-12.3256628518317));
#7418=CARTESIAN_POINT('Ctrl Pts',(46.,53.1250000136559,-5.63337527607782E-15));
#7419=CARTESIAN_POINT('Ctrl Pts',(46.,52.9166666803226,12.3256628518316));
#7420=CARTESIAN_POINT('Ctrl Pts',(39.8371685740842,52.7083333469893,23.));
#7421=CARTESIAN_POINT('Ctrl Pts',(33.6743371481684,52.5000000136559,33.6743371481683));
#7422=CARTESIAN_POINT('Ctrl Pts',(23.,52.2916666803226,39.8371685740842));
#7423=CARTESIAN_POINT('Ctrl Pts',(12.3256628518317,52.0833333469893,46.));
#7424=CARTESIAN_POINT('Ctrl Pts',(8.45006291411674E-15,51.8750000136559,
46.));
#7425=CARTESIAN_POINT('Ctrl Pts',(-12.3256628518316,51.6666666803226,46.));
#7426=CARTESIAN_POINT('Ctrl Pts',(-23.,51.4583333469893,39.8371685740842));
#7427=CARTESIAN_POINT('Ctrl Pts',(-33.6743371481683,51.2500000136559,33.6743371481684));
#7428=CARTESIAN_POINT('Ctrl Pts',(-39.8371685740842,51.0416666803226,23.));
#7429=CARTESIAN_POINT('Ctrl Pts',(-46.,50.8333333469893,12.3256628518317));
#7430=CARTESIAN_POINT('Ctrl Pts',(-46.,50.6250000136559,0.));
#7431=CARTESIAN_POINT('Ctrl Pts',(-46.,50.4166666803226,-12.3256628518316));
#7432=CARTESIAN_POINT('Ctrl Pts',(-39.8371685740842,50.2083333469893,-23.));
#7433=CARTESIAN_POINT('Ctrl Pts',(-33.6743371481684,50.0000000136559,-33.6743371481684));
#7434=CARTESIAN_POINT('Ctrl Pts',(-23.,49.7916666803226,-39.8371685740842));
#7435=CARTESIAN_POINT('Ctrl Pts',(-12.3256628518317,49.5833333469893,-46.));
#7436=CARTESIAN_POINT('Ctrl Pts',(-2.81668763803891E-15,49.3750000136559,
-46.));
#7437=CARTESIAN_POINT('Ctrl Pts',(12.3256628518316,49.1666666803226,-46.));
#7438=CARTESIAN_POINT('Ctrl Pts',(23.,48.9583333469893,-39.8371685740842));
#7439=CARTESIAN_POINT('Ctrl Pts',(33.6743371481683,48.7500000136559,-33.6743371481684));
#7440=CARTESIAN_POINT('Ctrl Pts',(39.8371685740842,48.5416666803226,-23.));
#7441=CARTESIAN_POINT('Ctrl Pts',(46.,48.3333333469893,-12.3256628518317));
#7442=CARTESIAN_POINT('Ctrl Pts',(46.,48.1250000136559,-5.63337527607782E-15));
#7443=CARTESIAN_POINT('Ctrl Pts',(46.,47.9166666803226,12.3256628518316));
#7444=CARTESIAN_POINT('Ctrl Pts',(39.8371685740842,47.7083333469893,23.));
#7445=CARTESIAN_POINT('Ctrl Pts',(33.6743371481684,47.5000000136559,33.6743371481683));
#7446=CARTESIAN_POINT('Ctrl Pts',(23.,47.2916666803226,39.8371685740842));
#7447=CARTESIAN_POINT('Ctrl Pts',(12.3256628518317,47.0833333469893,46.));
#7448=CARTESIAN_POINT('Ctrl Pts',(8.45006291411674E-15,46.8750000136559,
46.));
#7449=CARTESIAN_POINT('Ctrl Pts',(-12.3256628518316,46.6666666803226,46.));
#7450=CARTESIAN_POINT('Ctrl Pts',(-23.,46.4583333469893,39.8371685740842));
#7451=CARTESIAN_POINT('Ctrl Pts',(-33.6743371481683,46.2500000136559,33.6743371481684));
#7452=CARTESIAN_POINT('Ctrl Pts',(-39.8371685740842,46.0416666803226,23.));
#7453=CARTESIAN_POINT('Ctrl Pts',(-46.,45.8333333469892,12.3256628518317));
#7454=CARTESIAN_POINT('Ctrl Pts',(-46.,45.6250000136559,0.));
#7455=CARTESIAN_POINT('Ctrl Pts',(-46.,45.4166666803226,-12.3256628518316));
#7456=CARTESIAN_POINT('Ctrl Pts',(-39.8371685740842,45.2083333469893,-23.));
#7457=CARTESIAN_POINT('Ctrl Pts',(-33.6743371481684,45.0000000136559,-33.6743371481684));
#7458=CARTESIAN_POINT('Ctrl Pts',(-23.,44.7916666803226,-39.8371685740842));
#7459=CARTESIAN_POINT('Ctrl Pts',(-12.3256628518317,44.5833333469893,-46.));
#7460=CARTESIAN_POINT('Ctrl Pts',(-2.81668763803891E-15,44.3750000136559,
-46.));
#7461=CARTESIAN_POINT('Ctrl Pts',(12.3256628518316,44.1666666803226,-46.));
#7462=CARTESIAN_POINT('Ctrl Pts',(23.,43.9583333469893,-39.8371685740842));
#7463=CARTESIAN_POINT('Ctrl Pts',(33.6743371481683,43.7500000136559,-33.6743371481684));
#7464=CARTESIAN_POINT('Ctrl Pts',(39.8371685740842,43.5416666803226,-23.));
#7465=CARTESIAN_POINT('Ctrl Pts',(46.,43.3333333469893,-12.3256628518317));
#7466=CARTESIAN_POINT('Ctrl Pts',(46.,43.1250000136559,-5.63337527607782E-15));
#7467=CARTESIAN_POINT('Ctrl Pts',(46.,42.9166666803226,12.3256628518316));
#7468=CARTESIAN_POINT('Ctrl Pts',(39.8371685740842,42.7083333469893,23.));
#7469=CARTESIAN_POINT('Ctrl Pts',(33.6743371481684,42.5000000136559,33.6743371481683));
#7470=CARTESIAN_POINT('Ctrl Pts',(23.,42.2916666803226,39.8371685740842));
#7471=CARTESIAN_POINT('Ctrl Pts',(12.3256628518317,42.0833333469893,46.));
#7472=CARTESIAN_POINT('Ctrl Pts',(8.45006291411674E-15,41.8750000136559,
46.));
#7473=CARTESIAN_POINT('Ctrl Pts',(-12.3256628518316,41.6666666803226,46.));
#7474=CARTESIAN_POINT('Ctrl Pts',(-23.,41.4583333469893,39.8371685740842));
#7475=CARTESIAN_POINT('Ctrl Pts',(-33.6743371481683,41.2500000136559,33.6743371481684));
#7476=CARTESIAN_POINT('Ctrl Pts',(-39.8371685740842,41.0416666803226,23.));
#7477=CARTESIAN_POINT('Ctrl Pts',(-46.,40.8333333469893,12.3256628518317));
#7478=CARTESIAN_POINT('Ctrl Pts',(-46.,40.6250000136559,0.));
#7479=CARTESIAN_POINT('Ctrl Pts',(-46.,40.4166666803226,-12.3256628518316));
#7480=CARTESIAN_POINT('Ctrl Pts',(-39.8371685740842,40.2083333469893,-23.));
#7481=CARTESIAN_POINT('Ctrl Pts',(-33.6743371481684,40.0000000136559,-33.6743371481684));
#7482=CARTESIAN_POINT('Ctrl Pts',(-23.,39.7916666803226,-39.8371685740842));
#7483=CARTESIAN_POINT('Ctrl Pts',(-12.3256628518317,39.5833333469893,-46.));
#7484=CARTESIAN_POINT('Ctrl Pts',(-2.81668763803891E-15,39.3750000136559,
-46.));
#7485=CARTESIAN_POINT('Ctrl Pts',(12.3256628518316,39.1666666803226,-46.));
#7486=CARTESIAN_POINT('Ctrl Pts',(23.,38.9583333469893,-39.8371685740842));
#7487=CARTESIAN_POINT('Ctrl Pts',(33.6743371481683,38.7500000136559,-33.6743371481684));
#7488=CARTESIAN_POINT('Ctrl Pts',(39.8371685740842,38.5416666803226,-23.));
#7489=CARTESIAN_POINT('Ctrl Pts',(46.,38.3333333469893,-12.3256628518317));
#7490=CARTESIAN_POINT('Ctrl Pts',(46.,38.1250000136559,-5.63337527607782E-15));
#7491=CARTESIAN_POINT('Ctrl Pts',(46.,37.9166666803226,12.3256628518316));
#7492=CARTESIAN_POINT('Ctrl Pts',(39.8371685740842,37.7083333469893,23.));
#7493=CARTESIAN_POINT('Ctrl Pts',(33.6743371481684,37.5000000136559,33.6743371481683));
#7494=CARTESIAN_POINT('Ctrl Pts',(23.,37.2916666803226,39.8371685740842));
#7495=CARTESIAN_POINT('Ctrl Pts',(12.3256628518317,37.0833333469893,46.));
#7496=CARTESIAN_POINT('Ctrl Pts',(8.45006291411674E-15,36.8750000136559,
46.));
#7497=CARTESIAN_POINT('Ctrl Pts',(-12.3256628518316,36.6666666803226,46.));
#7498=CARTESIAN_POINT('Ctrl Pts',(-23.,36.4583333469893,39.8371685740842));
#7499=CARTESIAN_POINT('Ctrl Pts',(-33.6743371481683,36.2500000136559,33.6743371481684));
#7500=CARTESIAN_POINT('Ctrl Pts',(-39.8371685740842,36.0416666803226,23.));
#7501=CARTESIAN_POINT('Ctrl Pts',(-46.,35.8333333469893,12.3256628518317));
#7502=CARTESIAN_POINT('Ctrl Pts',(-46.,35.6250000136559,0.));
#7503=CARTESIAN_POINT('Ctrl Pts',(-46.,35.4166666803226,-12.3256628518316));
#7504=CARTESIAN_POINT('Ctrl Pts',(-39.8371685740842,35.2083333469893,-23.));
#7505=CARTESIAN_POINT('Ctrl Pts',(-33.6743371481684,35.0000000136559,-33.6743371481684));
#7506=CARTESIAN_POINT('Ctrl Pts',(-23.,34.7916666803226,-39.8371685740842));
#7507=CARTESIAN_POINT('Ctrl Pts',(-12.3256628518317,34.5833333469893,-46.));
#7508=CARTESIAN_POINT('Ctrl Pts',(-2.81668763803891E-15,34.3750000136559,
-46.));
#7509=CARTESIAN_POINT('Ctrl Pts',(12.3256628518316,34.1666666803226,-46.));
#7510=CARTESIAN_POINT('Ctrl Pts',(23.,33.9583333469893,-39.8371685740842));
#7511=CARTESIAN_POINT('Ctrl Pts',(33.6743371481683,33.7500000136559,-33.6743371481684));
#7512=CARTESIAN_POINT('Ctrl Pts',(39.8371685740842,33.5416666803226,-23.));
#7513=CARTESIAN_POINT('Ctrl Pts',(46.,33.3333333469893,-12.3256628518317));
#7514=CARTESIAN_POINT('Ctrl Pts',(46.,33.1250000136559,-5.63337527607782E-15));
#7515=CARTESIAN_POINT('Ctrl Pts',(46.,32.9166666803226,12.3256628518316));
#7516=CARTESIAN_POINT('Ctrl Pts',(39.8371685740842,32.7083333469893,23.));
#7517=CARTESIAN_POINT('Ctrl Pts',(33.6743371481684,32.5000000136559,33.6743371481683));
#7518=CARTESIAN_POINT('Ctrl Pts',(23.,32.2916666803226,39.8371685740842));
#7519=CARTESIAN_POINT('Ctrl Pts',(12.3256628518317,32.0833333469893,46.));
#7520=CARTESIAN_POINT('Ctrl Pts',(8.45006291411674E-15,31.8750000136559,
46.));
#7521=CARTESIAN_POINT('Ctrl Pts',(-12.3256628518316,31.6666666803226,46.));
#7522=CARTESIAN_POINT('Ctrl Pts',(-23.,31.4583333469893,39.8371685740842));
#7523=CARTESIAN_POINT('Ctrl Pts',(-33.6743371481683,31.2500000136559,33.6743371481684));
#7524=CARTESIAN_POINT('Ctrl Pts',(-39.8371685740842,31.0416666803226,23.));
#7525=CARTESIAN_POINT('Ctrl Pts',(-46.,30.8333333469893,12.3256628518317));
#7526=CARTESIAN_POINT('Ctrl Pts',(-46.,30.6250000136559,0.));
#7527=CARTESIAN_POINT('Ctrl Pts',(-46.,30.4166666803226,-12.3256628518316));
#7528=CARTESIAN_POINT('Ctrl Pts',(-39.8371685740842,30.2083333469893,-23.));
#7529=CARTESIAN_POINT('Ctrl Pts',(-33.6743371481684,30.0000000136559,-33.6743371481684));
#7530=CARTESIAN_POINT('Ctrl Pts',(-23.,29.7916666803226,-39.8371685740842));
#7531=CARTESIAN_POINT('Ctrl Pts',(-12.3256628518317,29.5833333469893,-46.));
#7532=CARTESIAN_POINT('Ctrl Pts',(-2.81668763803891E-15,29.3750000136559,
-46.));
#7533=CARTESIAN_POINT('Ctrl Pts',(12.3256628518316,29.1666666803226,-46.));
#7534=CARTESIAN_POINT('Ctrl Pts',(23.,28.9583333469893,-39.8371685740842));
#7535=CARTESIAN_POINT('Ctrl Pts',(33.6743371481683,28.7500000136559,-33.6743371481684));
#7536=CARTESIAN_POINT('Ctrl Pts',(39.8371685740842,28.5416666803226,-23.));
#7537=CARTESIAN_POINT('Ctrl Pts',(46.,28.3333333469893,-12.3256628518317));
#7538=CARTESIAN_POINT('Ctrl Pts',(46.,28.1250000136559,-5.63337527607782E-15));
#7539=CARTESIAN_POINT('Ctrl Pts',(46.,27.9166666803226,12.3256628518316));
#7540=CARTESIAN_POINT('Ctrl Pts',(39.8371685740842,27.7083333469893,23.));
#7541=CARTESIAN_POINT('Ctrl Pts',(33.6743371481684,27.5000000136559,33.6743371481683));
#7542=CARTESIAN_POINT('Ctrl Pts',(23.,27.2916666803226,39.8371685740842));
#7543=CARTESIAN_POINT('Ctrl Pts',(12.3256628518317,27.0833333469893,46.));
#7544=CARTESIAN_POINT('Ctrl Pts',(8.45006291411674E-15,26.8750000136559,
46.));
#7545=CARTESIAN_POINT('Ctrl Pts',(-12.3256628518316,26.6666666803226,46.));
#7546=CARTESIAN_POINT('Ctrl Pts',(-23.,26.4583333469893,39.8371685740842));
#7547=CARTESIAN_POINT('Ctrl Pts',(-33.6743371481683,26.2500000136559,33.6743371481684));
#7548=CARTESIAN_POINT('Ctrl Pts',(-39.8371685740842,26.0416666803226,23.));
#7549=CARTESIAN_POINT('Ctrl Pts',(-46.,25.8333333469893,12.3256628518317));
#7550=CARTESIAN_POINT('Ctrl Pts',(-46.,25.6250000136559,0.));
#7551=CARTESIAN_POINT('Ctrl Pts',(-48.706329375,57.187500006828,-1.8898197019151E-14));
#7552=CARTESIAN_POINT('Ctrl Pts',(-48.706329375,56.9791666734946,-13.0508216223155));
#7553=CARTESIAN_POINT('Ctrl Pts',(-42.1809185638422,56.7708333401613,-24.3531646875));
#7554=CARTESIAN_POINT('Ctrl Pts',(-35.6555077526845,56.562500006828,-35.6555077526845));
#7555=CARTESIAN_POINT('Ctrl Pts',(-24.3531646875,56.3541666734946,-42.1809185638423));
#7556=CARTESIAN_POINT('Ctrl Pts',(-13.0508216223155,56.1458333401613,-48.706329375));
#7557=CARTESIAN_POINT('Ctrl Pts',(1.59157945007855E-14,55.937500006828,
-48.706329375));
#7558=CARTESIAN_POINT('Ctrl Pts',(13.0508216223155,55.7291666734946,-48.706329375));
#7559=CARTESIAN_POINT('Ctrl Pts',(24.3531646875,55.5208333401613,-42.1809185638422));
#7560=CARTESIAN_POINT('Ctrl Pts',(35.6555077526845,55.312500006828,-35.6555077526845));
#7561=CARTESIAN_POINT('Ctrl Pts',(42.1809185638422,55.1041666734946,-24.3531646875));
#7562=CARTESIAN_POINT('Ctrl Pts',(48.706329375,54.8958333401613,-13.0508216223155));
#7563=CARTESIAN_POINT('Ctrl Pts',(48.706329375,54.687500006828,1.293339198242E-14));
#7564=CARTESIAN_POINT('Ctrl Pts',(48.706329375,54.4791666734946,13.0508216223155));
#7565=CARTESIAN_POINT('Ctrl Pts',(42.1809185638422,54.2708333401613,24.3531646875));
#7566=CARTESIAN_POINT('Ctrl Pts',(35.6555077526845,54.062500006828,35.6555077526845));
#7567=CARTESIAN_POINT('Ctrl Pts',(24.3531646875,53.8541666734946,42.1809185638422));
#7568=CARTESIAN_POINT('Ctrl Pts',(13.0508216223155,53.6458333401613,48.706329375));
#7569=CARTESIAN_POINT('Ctrl Pts',(-9.95098946405443E-15,53.437500006828,
48.706329375));
#7570=CARTESIAN_POINT('Ctrl Pts',(-13.0508216223155,53.2291666734946,48.706329375));
#7571=CARTESIAN_POINT('Ctrl Pts',(-24.3531646875,53.0208333401613,42.1809185638423));
#7572=CARTESIAN_POINT('Ctrl Pts',(-35.6555077526845,52.812500006828,35.6555077526845));
#7573=CARTESIAN_POINT('Ctrl Pts',(-42.1809185638422,52.6041666734946,24.3531646875));
#7574=CARTESIAN_POINT('Ctrl Pts',(-48.706329375,52.3958333401613,13.0508216223155));
#7575=CARTESIAN_POINT('Ctrl Pts',(-48.706329375,52.187500006828,-1.8898197019151E-14));
#7576=CARTESIAN_POINT('Ctrl Pts',(-48.706329375,51.9791666734946,-13.0508216223155));
#7577=CARTESIAN_POINT('Ctrl Pts',(-42.1809185638422,51.7708333401613,-24.3531646875));
#7578=CARTESIAN_POINT('Ctrl Pts',(-35.6555077526845,51.562500006828,-35.6555077526845));
#7579=CARTESIAN_POINT('Ctrl Pts',(-24.3531646875,51.3541666734946,-42.1809185638423));
#7580=CARTESIAN_POINT('Ctrl Pts',(-13.0508216223155,51.1458333401613,-48.706329375));
#7581=CARTESIAN_POINT('Ctrl Pts',(1.59157945007855E-14,50.937500006828,
-48.706329375));
#7582=CARTESIAN_POINT('Ctrl Pts',(13.0508216223155,50.7291666734946,-48.706329375));
#7583=CARTESIAN_POINT('Ctrl Pts',(24.3531646875,50.5208333401613,-42.1809185638422));
#7584=CARTESIAN_POINT('Ctrl Pts',(35.6555077526845,50.312500006828,-35.6555077526845));
#7585=CARTESIAN_POINT('Ctrl Pts',(42.1809185638422,50.1041666734946,-24.3531646875));
#7586=CARTESIAN_POINT('Ctrl Pts',(48.706329375,49.8958333401613,-13.0508216223155));
#7587=CARTESIAN_POINT('Ctrl Pts',(48.706329375,49.687500006828,1.293339198242E-14));
#7588=CARTESIAN_POINT('Ctrl Pts',(48.706329375,49.4791666734946,13.0508216223155));
#7589=CARTESIAN_POINT('Ctrl Pts',(42.1809185638422,49.2708333401613,24.3531646875));
#7590=CARTESIAN_POINT('Ctrl Pts',(35.6555077526845,49.062500006828,35.6555077526845));
#7591=CARTESIAN_POINT('Ctrl Pts',(24.3531646875,48.8541666734946,42.1809185638422));
#7592=CARTESIAN_POINT('Ctrl Pts',(13.0508216223155,48.6458333401613,48.706329375));
#7593=CARTESIAN_POINT('Ctrl Pts',(-9.95098946405443E-15,48.437500006828,
48.706329375));
#7594=CARTESIAN_POINT('Ctrl Pts',(-13.0508216223155,48.2291666734946,48.706329375));
#7595=CARTESIAN_POINT('Ctrl Pts',(-24.3531646875,48.0208333401613,42.1809185638423));
#7596=CARTESIAN_POINT('Ctrl Pts',(-35.6555077526845,47.812500006828,35.6555077526845));
#7597=CARTESIAN_POINT('Ctrl Pts',(-42.1809185638422,47.6041666734946,24.3531646875));
#7598=CARTESIAN_POINT('Ctrl Pts',(-48.706329375,47.3958333401613,13.0508216223155));
#7599=CARTESIAN_POINT('Ctrl Pts',(-48.706329375,47.187500006828,-1.8898197019151E-14));
#7600=CARTESIAN_POINT('Ctrl Pts',(-48.706329375,46.9791666734946,-13.0508216223155));
#7601=CARTESIAN_POINT('Ctrl Pts',(-42.1809185638422,46.7708333401613,-24.3531646875));
#7602=CARTESIAN_POINT('Ctrl Pts',(-35.6555077526845,46.562500006828,-35.6555077526845));
#7603=CARTESIAN_POINT('Ctrl Pts',(-24.3531646875,46.3541666734946,-42.1809185638423));
#7604=CARTESIAN_POINT('Ctrl Pts',(-13.0508216223155,46.1458333401613,-48.706329375));
#7605=CARTESIAN_POINT('Ctrl Pts',(1.59157945007855E-14,45.937500006828,
-48.706329375));
#7606=CARTESIAN_POINT('Ctrl Pts',(13.0508216223155,45.7291666734946,-48.706329375));
#7607=CARTESIAN_POINT('Ctrl Pts',(24.3531646875,45.5208333401613,-42.1809185638422));
#7608=CARTESIAN_POINT('Ctrl Pts',(35.6555077526845,45.312500006828,-35.6555077526845));
#7609=CARTESIAN_POINT('Ctrl Pts',(42.1809185638422,45.1041666734946,-24.3531646875));
#7610=CARTESIAN_POINT('Ctrl Pts',(48.706329375,44.8958333401613,-13.0508216223155));
#7611=CARTESIAN_POINT('Ctrl Pts',(48.706329375,44.687500006828,1.293339198242E-14));
#7612=CARTESIAN_POINT('Ctrl Pts',(48.706329375,44.4791666734946,13.0508216223155));
#7613=CARTESIAN_POINT('Ctrl Pts',(42.1809185638422,44.2708333401613,24.3531646875));
#7614=CARTESIAN_POINT('Ctrl Pts',(35.6555077526845,44.062500006828,35.6555077526845));
#7615=CARTESIAN_POINT('Ctrl Pts',(24.3531646875,43.8541666734946,42.1809185638422));
#7616=CARTESIAN_POINT('Ctrl Pts',(13.0508216223155,43.6458333401613,48.706329375));
#7617=CARTESIAN_POINT('Ctrl Pts',(-9.95098946405443E-15,43.437500006828,
48.706329375));
#7618=CARTESIAN_POINT('Ctrl Pts',(-13.0508216223155,43.2291666734946,48.706329375));
#7619=CARTESIAN_POINT('Ctrl Pts',(-24.3531646875,43.0208333401613,42.1809185638423));
#7620=CARTESIAN_POINT('Ctrl Pts',(-35.6555077526845,42.812500006828,35.6555077526845));
#7621=CARTESIAN_POINT('Ctrl Pts',(-42.1809185638422,42.6041666734946,24.3531646875));
#7622=CARTESIAN_POINT('Ctrl Pts',(-48.706329375,42.3958333401613,13.0508216223155));
#7623=CARTESIAN_POINT('Ctrl Pts',(-48.706329375,42.187500006828,-1.8898197019151E-14));
#7624=CARTESIAN_POINT('Ctrl Pts',(-48.706329375,41.9791666734946,-13.0508216223155));
#7625=CARTESIAN_POINT('Ctrl Pts',(-42.1809185638422,41.7708333401613,-24.3531646875));
#7626=CARTESIAN_POINT('Ctrl Pts',(-35.6555077526845,41.562500006828,-35.6555077526845));
#7627=CARTESIAN_POINT('Ctrl Pts',(-24.3531646875,41.3541666734946,-42.1809185638423));
#7628=CARTESIAN_POINT('Ctrl Pts',(-13.0508216223155,41.1458333401613,-48.706329375));
#7629=CARTESIAN_POINT('Ctrl Pts',(1.59157945007855E-14,40.937500006828,
-48.706329375));
#7630=CARTESIAN_POINT('Ctrl Pts',(13.0508216223155,40.7291666734946,-48.706329375));
#7631=CARTESIAN_POINT('Ctrl Pts',(24.3531646875,40.5208333401613,-42.1809185638422));
#7632=CARTESIAN_POINT('Ctrl Pts',(35.6555077526845,40.312500006828,-35.6555077526845));
#7633=CARTESIAN_POINT('Ctrl Pts',(42.1809185638422,40.1041666734946,-24.3531646875));
#7634=CARTESIAN_POINT('Ctrl Pts',(48.706329375,39.8958333401613,-13.0508216223155));
#7635=CARTESIAN_POINT('Ctrl Pts',(48.706329375,39.687500006828,1.293339198242E-14));
#7636=CARTESIAN_POINT('Ctrl Pts',(48.706329375,39.4791666734946,13.0508216223155));
#7637=CARTESIAN_POINT('Ctrl Pts',(42.1809185638422,39.2708333401613,24.3531646875));
#7638=CARTESIAN_POINT('Ctrl Pts',(35.6555077526845,39.062500006828,35.6555077526845));
#7639=CARTESIAN_POINT('Ctrl Pts',(24.3531646875,38.8541666734946,42.1809185638422));
#7640=CARTESIAN_POINT('Ctrl Pts',(13.0508216223155,38.6458333401613,48.706329375));
#7641=CARTESIAN_POINT('Ctrl Pts',(-9.95098946405443E-15,38.437500006828,
48.706329375));
#7642=CARTESIAN_POINT('Ctrl Pts',(-13.0508216223155,38.2291666734946,48.706329375));
#7643=CARTESIAN_POINT('Ctrl Pts',(-24.3531646875,38.0208333401613,42.1809185638423));
#7644=CARTESIAN_POINT('Ctrl Pts',(-35.6555077526845,37.812500006828,35.6555077526845));
#7645=CARTESIAN_POINT('Ctrl Pts',(-42.1809185638422,37.6041666734946,24.3531646875));
#7646=CARTESIAN_POINT('Ctrl Pts',(-48.706329375,37.3958333401613,13.0508216223155));
#7647=CARTESIAN_POINT('Ctrl Pts',(-48.706329375,37.187500006828,-1.8898197019151E-14));
#7648=CARTESIAN_POINT('Ctrl Pts',(-48.706329375,36.9791666734946,-13.0508216223155));
#7649=CARTESIAN_POINT('Ctrl Pts',(-42.1809185638422,36.7708333401613,-24.3531646875));
#7650=CARTESIAN_POINT('Ctrl Pts',(-35.6555077526845,36.562500006828,-35.6555077526845));
#7651=CARTESIAN_POINT('Ctrl Pts',(-24.3531646875,36.3541666734946,-42.1809185638423));
#7652=CARTESIAN_POINT('Ctrl Pts',(-13.0508216223155,36.1458333401613,-48.706329375));
#7653=CARTESIAN_POINT('Ctrl Pts',(1.59157945007855E-14,35.937500006828,
-48.706329375));
#7654=CARTESIAN_POINT('Ctrl Pts',(13.0508216223155,35.7291666734946,-48.706329375));
#7655=CARTESIAN_POINT('Ctrl Pts',(24.3531646875,35.5208333401613,-42.1809185638422));
#7656=CARTESIAN_POINT('Ctrl Pts',(35.6555077526845,35.312500006828,-35.6555077526845));
#7657=CARTESIAN_POINT('Ctrl Pts',(42.1809185638422,35.1041666734946,-24.3531646875));
#7658=CARTESIAN_POINT('Ctrl Pts',(48.706329375,34.8958333401613,-13.0508216223155));
#7659=CARTESIAN_POINT('Ctrl Pts',(48.706329375,34.687500006828,1.293339198242E-14));
#7660=CARTESIAN_POINT('Ctrl Pts',(48.706329375,34.4791666734946,13.0508216223155));
#7661=CARTESIAN_POINT('Ctrl Pts',(42.1809185638422,34.2708333401613,24.3531646875));
#7662=CARTESIAN_POINT('Ctrl Pts',(35.6555077526845,34.062500006828,35.6555077526845));
#7663=CARTESIAN_POINT('Ctrl Pts',(24.3531646875,33.8541666734946,42.1809185638422));
#7664=CARTESIAN_POINT('Ctrl Pts',(13.0508216223155,33.6458333401613,48.706329375));
#7665=CARTESIAN_POINT('Ctrl Pts',(-9.95098946405443E-15,33.437500006828,
48.706329375));
#7666=CARTESIAN_POINT('Ctrl Pts',(-13.0508216223155,33.2291666734946,48.706329375));
#7667=CARTESIAN_POINT('Ctrl Pts',(-24.3531646875,33.0208333401613,42.1809185638423));
#7668=CARTESIAN_POINT('Ctrl Pts',(-35.6555077526845,32.812500006828,35.6555077526845));
#7669=CARTESIAN_POINT('Ctrl Pts',(-42.1809185638422,32.6041666734946,24.3531646875));
#7670=CARTESIAN_POINT('Ctrl Pts',(-48.706329375,32.3958333401613,13.0508216223155));
#7671=CARTESIAN_POINT('Ctrl Pts',(-48.706329375,32.187500006828,-1.8898197019151E-14));
#7672=CARTESIAN_POINT('Ctrl Pts',(-48.706329375,31.9791666734946,-13.0508216223155));
#7673=CARTESIAN_POINT('Ctrl Pts',(-42.1809185638422,31.7708333401613,-24.3531646875));
#7674=CARTESIAN_POINT('Ctrl Pts',(-35.6555077526845,31.562500006828,-35.6555077526845));
#7675=CARTESIAN_POINT('Ctrl Pts',(-24.3531646875,31.3541666734946,-42.1809185638423));
#7676=CARTESIAN_POINT('Ctrl Pts',(-13.0508216223155,31.1458333401613,-48.706329375));
#7677=CARTESIAN_POINT('Ctrl Pts',(1.59157945007855E-14,30.937500006828,
-48.706329375));
#7678=CARTESIAN_POINT('Ctrl Pts',(13.0508216223155,30.7291666734946,-48.706329375));
#7679=CARTESIAN_POINT('Ctrl Pts',(24.3531646875,30.5208333401613,-42.1809185638422));
#7680=CARTESIAN_POINT('Ctrl Pts',(35.6555077526845,30.312500006828,-35.6555077526845));
#7681=CARTESIAN_POINT('Ctrl Pts',(42.1809185638422,30.1041666734946,-24.3531646875));
#7682=CARTESIAN_POINT('Ctrl Pts',(48.706329375,29.8958333401613,-13.0508216223155));
#7683=CARTESIAN_POINT('Ctrl Pts',(48.706329375,29.687500006828,1.293339198242E-14));
#7684=CARTESIAN_POINT('Ctrl Pts',(48.706329375,29.4791666734946,13.0508216223155));
#7685=CARTESIAN_POINT('Ctrl Pts',(42.1809185638422,29.2708333401613,24.3531646875));
#7686=CARTESIAN_POINT('Ctrl Pts',(35.6555077526845,29.062500006828,35.6555077526845));
#7687=CARTESIAN_POINT('Ctrl Pts',(24.3531646875,28.8541666734946,42.1809185638422));
#7688=CARTESIAN_POINT('Ctrl Pts',(13.0508216223155,28.6458333401613,48.706329375));
#7689=CARTESIAN_POINT('Ctrl Pts',(-9.95098946405443E-15,28.437500006828,
48.706329375));
#7690=CARTESIAN_POINT('Ctrl Pts',(-13.0508216223155,28.2291666734946,48.706329375));
#7691=CARTESIAN_POINT('Ctrl Pts',(-24.3531646875,28.0208333401613,42.1809185638423));
#7692=CARTESIAN_POINT('Ctrl Pts',(-35.6555077526845,27.812500006828,35.6555077526845));
#7693=CARTESIAN_POINT('Ctrl Pts',(-42.1809185638422,27.6041666734946,24.3531646875));
#7694=CARTESIAN_POINT('Ctrl Pts',(-48.706329375,27.3958333401613,13.0508216223155));
#7695=CARTESIAN_POINT('Ctrl Pts',(-48.706329375,27.187500006828,-1.8898197019151E-14));
#7696=CARTESIAN_POINT('',(3.61292728433798,40.8792520480093,-48.5721450795008));
#7697=CARTESIAN_POINT('',(48.5134353784345,39.7574536451604,-4.33048599679679));
#7698=CARTESIAN_POINT('Ctrl Pts',(3.61292728433798,40.8792520480092,-48.5721450795008));
#7699=CARTESIAN_POINT('Ctrl Pts',(14.7133549689477,40.6985216017706,-47.7464652997852));
#7700=CARTESIAN_POINT('Ctrl Pts',(24.3531646875,40.5208333401613,-42.1809185638422));
#7701=CARTESIAN_POINT('Ctrl Pts',(35.6555077526845,40.312500006828,-35.6555077526845));
#7702=CARTESIAN_POINT('Ctrl Pts',(42.1809185638422,40.1041666734946,-24.3531646875));
#7703=CARTESIAN_POINT('Ctrl Pts',(47.5573898704235,39.9325149229327,-15.0408432190651));
#7704=CARTESIAN_POINT('Ctrl Pts',(48.5134353784345,39.7574536451604,-4.33048599679679));
#7705=CARTESIAN_POINT('Origin',(-4513.80899746256,7993.28354997889,-4.33049059987538));
#7706=CARTESIAN_POINT('Ctrl Pts',(3.61292728433799,39.3132892765089,-45.8578974271399));
#7707=CARTESIAN_POINT('Ctrl Pts',(3.61292728433795,39.4468822859549,-46.089460636719));
#7708=CARTESIAN_POINT('Ctrl Pts',(3.61292728433823,39.7140705280013,-46.5525857733052));
#7709=CARTESIAN_POINT('Ctrl Pts',(3.61292728433805,39.9812630238615,-47.0157084557285));
#7710=CARTESIAN_POINT('Ctrl Pts',(3.61292728433805,40.3696539378594,-47.6888965792834));
#7711=CARTESIAN_POINT('Ctrl Pts',(3.61292728433798,40.624451287085,-48.1305218136162));
#7712=CARTESIAN_POINT('Ctrl Pts',(3.61292728433798,40.8792520480093,-48.5721450795008));
#7713=CARTESIAN_POINT('Ctrl Pts',(-46.,55.6250000136559,0.));
#7714=CARTESIAN_POINT('Ctrl Pts',(-46.,55.4166666803226,-12.3256628518316));
#7715=CARTESIAN_POINT('Ctrl Pts',(-39.8371685740842,55.2083333469893,-23.));
#7716=CARTESIAN_POINT('Ctrl Pts',(-33.6743371481684,55.0000000136559,-33.6743371481684));
#7717=CARTESIAN_POINT('Ctrl Pts',(-23.,54.7916666803226,-39.8371685740842));
#7718=CARTESIAN_POINT('Ctrl Pts',(-12.3256628518317,54.5833333469893,-46.));
#7719=CARTESIAN_POINT('Ctrl Pts',(-2.81668763803891E-15,54.3750000136559,
-46.));
#7720=CARTESIAN_POINT('Ctrl Pts',(12.3256628518316,54.1666666803226,-46.));
#7721=CARTESIAN_POINT('Ctrl Pts',(23.,53.9583333469893,-39.8371685740842));
#7722=CARTESIAN_POINT('Ctrl Pts',(33.6743371481683,53.7500000136559,-33.6743371481684));
#7723=CARTESIAN_POINT('Ctrl Pts',(39.8371685740842,53.5416666803226,-23.));
#7724=CARTESIAN_POINT('Ctrl Pts',(46.,53.3333333469893,-12.3256628518317));
#7725=CARTESIAN_POINT('Ctrl Pts',(46.,53.1250000136559,-5.63337527607782E-15));
#7726=CARTESIAN_POINT('Ctrl Pts',(46.,52.9166666803226,12.3256628518316));
#7727=CARTESIAN_POINT('Ctrl Pts',(39.8371685740842,52.7083333469893,23.));
#7728=CARTESIAN_POINT('Ctrl Pts',(33.6743371481684,52.5000000136559,33.6743371481683));
#7729=CARTESIAN_POINT('Ctrl Pts',(23.,52.2916666803226,39.8371685740842));
#7730=CARTESIAN_POINT('Ctrl Pts',(12.3256628518317,52.0833333469893,46.));
#7731=CARTESIAN_POINT('Ctrl Pts',(8.45006291411674E-15,51.8750000136559,
46.));
#7732=CARTESIAN_POINT('Ctrl Pts',(-12.3256628518316,51.6666666803226,46.));
#7733=CARTESIAN_POINT('Ctrl Pts',(-23.,51.4583333469893,39.8371685740842));
#7734=CARTESIAN_POINT('Ctrl Pts',(-33.6743371481683,51.2500000136559,33.6743371481684));
#7735=CARTESIAN_POINT('Ctrl Pts',(-39.8371685740842,51.0416666803226,23.));
#7736=CARTESIAN_POINT('Ctrl Pts',(-46.,50.8333333469893,12.3256628518317));
#7737=CARTESIAN_POINT('Ctrl Pts',(-46.,50.6250000136559,0.));
#7738=CARTESIAN_POINT('Ctrl Pts',(-46.,50.4166666803226,-12.3256628518316));
#7739=CARTESIAN_POINT('Ctrl Pts',(-39.8371685740842,50.2083333469893,-23.));
#7740=CARTESIAN_POINT('Ctrl Pts',(-33.6743371481684,50.0000000136559,-33.6743371481684));
#7741=CARTESIAN_POINT('Ctrl Pts',(-23.,49.7916666803226,-39.8371685740842));
#7742=CARTESIAN_POINT('Ctrl Pts',(-12.3256628518317,49.5833333469893,-46.));
#7743=CARTESIAN_POINT('Ctrl Pts',(-2.81668763803891E-15,49.3750000136559,
-46.));
#7744=CARTESIAN_POINT('Ctrl Pts',(12.3256628518316,49.1666666803226,-46.));
#7745=CARTESIAN_POINT('Ctrl Pts',(23.,48.9583333469893,-39.8371685740842));
#7746=CARTESIAN_POINT('Ctrl Pts',(33.6743371481683,48.7500000136559,-33.6743371481684));
#7747=CARTESIAN_POINT('Ctrl Pts',(39.8371685740842,48.5416666803226,-23.));
#7748=CARTESIAN_POINT('Ctrl Pts',(46.,48.3333333469893,-12.3256628518317));
#7749=CARTESIAN_POINT('Ctrl Pts',(46.,48.1250000136559,-5.63337527607782E-15));
#7750=CARTESIAN_POINT('Ctrl Pts',(46.,47.9166666803226,12.3256628518316));
#7751=CARTESIAN_POINT('Ctrl Pts',(39.8371685740842,47.7083333469893,23.));
#7752=CARTESIAN_POINT('Ctrl Pts',(33.6743371481684,47.5000000136559,33.6743371481683));
#7753=CARTESIAN_POINT('Ctrl Pts',(23.,47.2916666803226,39.8371685740842));
#7754=CARTESIAN_POINT('Ctrl Pts',(12.3256628518317,47.0833333469893,46.));
#7755=CARTESIAN_POINT('Ctrl Pts',(8.45006291411674E-15,46.8750000136559,
46.));
#7756=CARTESIAN_POINT('Ctrl Pts',(-12.3256628518316,46.6666666803226,46.));
#7757=CARTESIAN_POINT('Ctrl Pts',(-23.,46.4583333469893,39.8371685740842));
#7758=CARTESIAN_POINT('Ctrl Pts',(-33.6743371481683,46.2500000136559,33.6743371481684));
#7759=CARTESIAN_POINT('Ctrl Pts',(-39.8371685740842,46.0416666803226,23.));
#7760=CARTESIAN_POINT('Ctrl Pts',(-46.,45.8333333469892,12.3256628518317));
#7761=CARTESIAN_POINT('Ctrl Pts',(-46.,45.6250000136559,0.));
#7762=CARTESIAN_POINT('Ctrl Pts',(-46.,45.4166666803226,-12.3256628518316));
#7763=CARTESIAN_POINT('Ctrl Pts',(-39.8371685740842,45.2083333469893,-23.));
#7764=CARTESIAN_POINT('Ctrl Pts',(-33.6743371481684,45.0000000136559,-33.6743371481684));
#7765=CARTESIAN_POINT('Ctrl Pts',(-23.,44.7916666803226,-39.8371685740842));
#7766=CARTESIAN_POINT('Ctrl Pts',(-12.3256628518317,44.5833333469893,-46.));
#7767=CARTESIAN_POINT('Ctrl Pts',(-2.81668763803891E-15,44.3750000136559,
-46.));
#7768=CARTESIAN_POINT('Ctrl Pts',(12.3256628518316,44.1666666803226,-46.));
#7769=CARTESIAN_POINT('Ctrl Pts',(23.,43.9583333469893,-39.8371685740842));
#7770=CARTESIAN_POINT('Ctrl Pts',(33.6743371481683,43.7500000136559,-33.6743371481684));
#7771=CARTESIAN_POINT('Ctrl Pts',(39.8371685740842,43.5416666803226,-23.));
#7772=CARTESIAN_POINT('Ctrl Pts',(46.,43.3333333469893,-12.3256628518317));
#7773=CARTESIAN_POINT('Ctrl Pts',(46.,43.1250000136559,-5.63337527607782E-15));
#7774=CARTESIAN_POINT('Ctrl Pts',(46.,42.9166666803226,12.3256628518316));
#7775=CARTESIAN_POINT('Ctrl Pts',(39.8371685740842,42.7083333469893,23.));
#7776=CARTESIAN_POINT('Ctrl Pts',(33.6743371481684,42.5000000136559,33.6743371481683));
#7777=CARTESIAN_POINT('Ctrl Pts',(23.,42.2916666803226,39.8371685740842));
#7778=CARTESIAN_POINT('Ctrl Pts',(12.3256628518317,42.0833333469893,46.));
#7779=CARTESIAN_POINT('Ctrl Pts',(8.45006291411674E-15,41.8750000136559,
46.));
#7780=CARTESIAN_POINT('Ctrl Pts',(-12.3256628518316,41.6666666803226,46.));
#7781=CARTESIAN_POINT('Ctrl Pts',(-23.,41.4583333469893,39.8371685740842));
#7782=CARTESIAN_POINT('Ctrl Pts',(-33.6743371481683,41.2500000136559,33.6743371481684));
#7783=CARTESIAN_POINT('Ctrl Pts',(-39.8371685740842,41.0416666803226,23.));
#7784=CARTESIAN_POINT('Ctrl Pts',(-46.,40.8333333469893,12.3256628518317));
#7785=CARTESIAN_POINT('Ctrl Pts',(-46.,40.6250000136559,0.));
#7786=CARTESIAN_POINT('Ctrl Pts',(-46.,40.4166666803226,-12.3256628518316));
#7787=CARTESIAN_POINT('Ctrl Pts',(-39.8371685740842,40.2083333469893,-23.));
#7788=CARTESIAN_POINT('Ctrl Pts',(-33.6743371481684,40.0000000136559,-33.6743371481684));
#7789=CARTESIAN_POINT('Ctrl Pts',(-23.,39.7916666803226,-39.8371685740842));
#7790=CARTESIAN_POINT('Ctrl Pts',(-12.3256628518317,39.5833333469893,-46.));
#7791=CARTESIAN_POINT('Ctrl Pts',(-2.81668763803891E-15,39.3750000136559,
-46.));
#7792=CARTESIAN_POINT('Ctrl Pts',(12.3256628518316,39.1666666803226,-46.));
#7793=CARTESIAN_POINT('Ctrl Pts',(23.,38.9583333469893,-39.8371685740842));
#7794=CARTESIAN_POINT('Ctrl Pts',(33.6743371481683,38.7500000136559,-33.6743371481684));
#7795=CARTESIAN_POINT('Ctrl Pts',(39.8371685740842,38.5416666803226,-23.));
#7796=CARTESIAN_POINT('Ctrl Pts',(46.,38.3333333469893,-12.3256628518317));
#7797=CARTESIAN_POINT('Ctrl Pts',(46.,38.1250000136559,-5.63337527607782E-15));
#7798=CARTESIAN_POINT('Ctrl Pts',(46.,37.9166666803226,12.3256628518316));
#7799=CARTESIAN_POINT('Ctrl Pts',(39.8371685740842,37.7083333469893,23.));
#7800=CARTESIAN_POINT('Ctrl Pts',(33.6743371481684,37.5000000136559,33.6743371481683));
#7801=CARTESIAN_POINT('Ctrl Pts',(23.,37.2916666803226,39.8371685740842));
#7802=CARTESIAN_POINT('Ctrl Pts',(12.3256628518317,37.0833333469893,46.));
#7803=CARTESIAN_POINT('Ctrl Pts',(8.45006291411674E-15,36.8750000136559,
46.));
#7804=CARTESIAN_POINT('Ctrl Pts',(-12.3256628518316,36.6666666803226,46.));
#7805=CARTESIAN_POINT('Ctrl Pts',(-23.,36.4583333469893,39.8371685740842));
#7806=CARTESIAN_POINT('Ctrl Pts',(-33.6743371481683,36.2500000136559,33.6743371481684));
#7807=CARTESIAN_POINT('Ctrl Pts',(-39.8371685740842,36.0416666803226,23.));
#7808=CARTESIAN_POINT('Ctrl Pts',(-46.,35.8333333469893,12.3256628518317));
#7809=CARTESIAN_POINT('Ctrl Pts',(-46.,35.6250000136559,0.));
#7810=CARTESIAN_POINT('Ctrl Pts',(-46.,35.4166666803226,-12.3256628518316));
#7811=CARTESIAN_POINT('Ctrl Pts',(-39.8371685740842,35.2083333469893,-23.));
#7812=CARTESIAN_POINT('Ctrl Pts',(-33.6743371481684,35.0000000136559,-33.6743371481684));
#7813=CARTESIAN_POINT('Ctrl Pts',(-23.,34.7916666803226,-39.8371685740842));
#7814=CARTESIAN_POINT('Ctrl Pts',(-12.3256628518317,34.5833333469893,-46.));
#7815=CARTESIAN_POINT('Ctrl Pts',(-2.81668763803891E-15,34.3750000136559,
-46.));
#7816=CARTESIAN_POINT('Ctrl Pts',(12.3256628518316,34.1666666803226,-46.));
#7817=CARTESIAN_POINT('Ctrl Pts',(23.,33.9583333469893,-39.8371685740842));
#7818=CARTESIAN_POINT('Ctrl Pts',(33.6743371481683,33.7500000136559,-33.6743371481684));
#7819=CARTESIAN_POINT('Ctrl Pts',(39.8371685740842,33.5416666803226,-23.));
#7820=CARTESIAN_POINT('Ctrl Pts',(46.,33.3333333469893,-12.3256628518317));
#7821=CARTESIAN_POINT('Ctrl Pts',(46.,33.1250000136559,-5.63337527607782E-15));
#7822=CARTESIAN_POINT('Ctrl Pts',(46.,32.9166666803226,12.3256628518316));
#7823=CARTESIAN_POINT('Ctrl Pts',(39.8371685740842,32.7083333469893,23.));
#7824=CARTESIAN_POINT('Ctrl Pts',(33.6743371481684,32.5000000136559,33.6743371481683));
#7825=CARTESIAN_POINT('Ctrl Pts',(23.,32.2916666803226,39.8371685740842));
#7826=CARTESIAN_POINT('Ctrl Pts',(12.3256628518317,32.0833333469893,46.));
#7827=CARTESIAN_POINT('Ctrl Pts',(8.45006291411674E-15,31.8750000136559,
46.));
#7828=CARTESIAN_POINT('Ctrl Pts',(-12.3256628518316,31.6666666803226,46.));
#7829=CARTESIAN_POINT('Ctrl Pts',(-23.,31.4583333469893,39.8371685740842));
#7830=CARTESIAN_POINT('Ctrl Pts',(-33.6743371481683,31.2500000136559,33.6743371481684));
#7831=CARTESIAN_POINT('Ctrl Pts',(-39.8371685740842,31.0416666803226,23.));
#7832=CARTESIAN_POINT('Ctrl Pts',(-46.,30.8333333469893,12.3256628518317));
#7833=CARTESIAN_POINT('Ctrl Pts',(-46.,30.6250000136559,0.));
#7834=CARTESIAN_POINT('Ctrl Pts',(-46.,30.4166666803226,-12.3256628518316));
#7835=CARTESIAN_POINT('Ctrl Pts',(-39.8371685740842,30.2083333469893,-23.));
#7836=CARTESIAN_POINT('Ctrl Pts',(-33.6743371481684,30.0000000136559,-33.6743371481684));
#7837=CARTESIAN_POINT('Ctrl Pts',(-23.,29.7916666803226,-39.8371685740842));
#7838=CARTESIAN_POINT('Ctrl Pts',(-12.3256628518317,29.5833333469893,-46.));
#7839=CARTESIAN_POINT('Ctrl Pts',(-2.81668763803891E-15,29.3750000136559,
-46.));
#7840=CARTESIAN_POINT('Ctrl Pts',(12.3256628518316,29.1666666803226,-46.));
#7841=CARTESIAN_POINT('Ctrl Pts',(23.,28.9583333469893,-39.8371685740842));
#7842=CARTESIAN_POINT('Ctrl Pts',(33.6743371481683,28.7500000136559,-33.6743371481684));
#7843=CARTESIAN_POINT('Ctrl Pts',(39.8371685740842,28.5416666803226,-23.));
#7844=CARTESIAN_POINT('Ctrl Pts',(46.,28.3333333469893,-12.3256628518317));
#7845=CARTESIAN_POINT('Ctrl Pts',(46.,28.1250000136559,-5.63337527607782E-15));
#7846=CARTESIAN_POINT('Ctrl Pts',(46.,27.9166666803226,12.3256628518316));
#7847=CARTESIAN_POINT('Ctrl Pts',(39.8371685740842,27.7083333469893,23.));
#7848=CARTESIAN_POINT('Ctrl Pts',(33.6743371481684,27.5000000136559,33.6743371481683));
#7849=CARTESIAN_POINT('Ctrl Pts',(23.,27.2916666803226,39.8371685740842));
#7850=CARTESIAN_POINT('Ctrl Pts',(12.3256628518317,27.0833333469893,46.));
#7851=CARTESIAN_POINT('Ctrl Pts',(8.45006291411674E-15,26.8750000136559,
46.));
#7852=CARTESIAN_POINT('Ctrl Pts',(-12.3256628518316,26.6666666803226,46.));
#7853=CARTESIAN_POINT('Ctrl Pts',(-23.,26.4583333469893,39.8371685740842));
#7854=CARTESIAN_POINT('Ctrl Pts',(-33.6743371481683,26.2500000136559,33.6743371481684));
#7855=CARTESIAN_POINT('Ctrl Pts',(-39.8371685740842,26.0416666803226,23.));
#7856=CARTESIAN_POINT('Ctrl Pts',(-46.,25.8333333469893,12.3256628518317));
#7857=CARTESIAN_POINT('Ctrl Pts',(-46.,25.6250000136559,0.));
#7858=CARTESIAN_POINT('Ctrl Pts',(-48.706329375,57.187500006828,-1.8898197019151E-14));
#7859=CARTESIAN_POINT('Ctrl Pts',(-48.706329375,56.9791666734946,-13.0508216223155));
#7860=CARTESIAN_POINT('Ctrl Pts',(-42.1809185638422,56.7708333401613,-24.3531646875));
#7861=CARTESIAN_POINT('Ctrl Pts',(-35.6555077526845,56.562500006828,-35.6555077526845));
#7862=CARTESIAN_POINT('Ctrl Pts',(-24.3531646875,56.3541666734946,-42.1809185638423));
#7863=CARTESIAN_POINT('Ctrl Pts',(-13.0508216223155,56.1458333401613,-48.706329375));
#7864=CARTESIAN_POINT('Ctrl Pts',(1.59157945007855E-14,55.937500006828,
-48.706329375));
#7865=CARTESIAN_POINT('Ctrl Pts',(13.0508216223155,55.7291666734946,-48.706329375));
#7866=CARTESIAN_POINT('Ctrl Pts',(24.3531646875,55.5208333401613,-42.1809185638422));
#7867=CARTESIAN_POINT('Ctrl Pts',(35.6555077526845,55.312500006828,-35.6555077526845));
#7868=CARTESIAN_POINT('Ctrl Pts',(42.1809185638422,55.1041666734946,-24.3531646875));
#7869=CARTESIAN_POINT('Ctrl Pts',(48.706329375,54.8958333401613,-13.0508216223155));
#7870=CARTESIAN_POINT('Ctrl Pts',(48.706329375,54.687500006828,1.293339198242E-14));
#7871=CARTESIAN_POINT('Ctrl Pts',(48.706329375,54.4791666734946,13.0508216223155));
#7872=CARTESIAN_POINT('Ctrl Pts',(42.1809185638422,54.2708333401613,24.3531646875));
#7873=CARTESIAN_POINT('Ctrl Pts',(35.6555077526845,54.062500006828,35.6555077526845));
#7874=CARTESIAN_POINT('Ctrl Pts',(24.3531646875,53.8541666734946,42.1809185638422));
#7875=CARTESIAN_POINT('Ctrl Pts',(13.0508216223155,53.6458333401613,48.706329375));
#7876=CARTESIAN_POINT('Ctrl Pts',(-9.95098946405443E-15,53.437500006828,
48.706329375));
#7877=CARTESIAN_POINT('Ctrl Pts',(-13.0508216223155,53.2291666734946,48.706329375));
#7878=CARTESIAN_POINT('Ctrl Pts',(-24.3531646875,53.0208333401613,42.1809185638423));
#7879=CARTESIAN_POINT('Ctrl Pts',(-35.6555077526845,52.812500006828,35.6555077526845));
#7880=CARTESIAN_POINT('Ctrl Pts',(-42.1809185638422,52.6041666734946,24.3531646875));
#7881=CARTESIAN_POINT('Ctrl Pts',(-48.706329375,52.3958333401613,13.0508216223155));
#7882=CARTESIAN_POINT('Ctrl Pts',(-48.706329375,52.187500006828,-1.8898197019151E-14));
#7883=CARTESIAN_POINT('Ctrl Pts',(-48.706329375,51.9791666734946,-13.0508216223155));
#7884=CARTESIAN_POINT('Ctrl Pts',(-42.1809185638422,51.7708333401613,-24.3531646875));
#7885=CARTESIAN_POINT('Ctrl Pts',(-35.6555077526845,51.562500006828,-35.6555077526845));
#7886=CARTESIAN_POINT('Ctrl Pts',(-24.3531646875,51.3541666734946,-42.1809185638423));
#7887=CARTESIAN_POINT('Ctrl Pts',(-13.0508216223155,51.1458333401613,-48.706329375));
#7888=CARTESIAN_POINT('Ctrl Pts',(1.59157945007855E-14,50.937500006828,
-48.706329375));
#7889=CARTESIAN_POINT('Ctrl Pts',(13.0508216223155,50.7291666734946,-48.706329375));
#7890=CARTESIAN_POINT('Ctrl Pts',(24.3531646875,50.5208333401613,-42.1809185638422));
#7891=CARTESIAN_POINT('Ctrl Pts',(35.6555077526845,50.312500006828,-35.6555077526845));
#7892=CARTESIAN_POINT('Ctrl Pts',(42.1809185638422,50.1041666734946,-24.3531646875));
#7893=CARTESIAN_POINT('Ctrl Pts',(48.706329375,49.8958333401613,-13.0508216223155));
#7894=CARTESIAN_POINT('Ctrl Pts',(48.706329375,49.687500006828,1.293339198242E-14));
#7895=CARTESIAN_POINT('Ctrl Pts',(48.706329375,49.4791666734946,13.0508216223155));
#7896=CARTESIAN_POINT('Ctrl Pts',(42.1809185638422,49.2708333401613,24.3531646875));
#7897=CARTESIAN_POINT('Ctrl Pts',(35.6555077526845,49.062500006828,35.6555077526845));
#7898=CARTESIAN_POINT('Ctrl Pts',(24.3531646875,48.8541666734946,42.1809185638422));
#7899=CARTESIAN_POINT('Ctrl Pts',(13.0508216223155,48.6458333401613,48.706329375));
#7900=CARTESIAN_POINT('Ctrl Pts',(-9.95098946405443E-15,48.437500006828,
48.706329375));
#7901=CARTESIAN_POINT('Ctrl Pts',(-13.0508216223155,48.2291666734946,48.706329375));
#7902=CARTESIAN_POINT('Ctrl Pts',(-24.3531646875,48.0208333401613,42.1809185638423));
#7903=CARTESIAN_POINT('Ctrl Pts',(-35.6555077526845,47.812500006828,35.6555077526845));
#7904=CARTESIAN_POINT('Ctrl Pts',(-42.1809185638422,47.6041666734946,24.3531646875));
#7905=CARTESIAN_POINT('Ctrl Pts',(-48.706329375,47.3958333401613,13.0508216223155));
#7906=CARTESIAN_POINT('Ctrl Pts',(-48.706329375,47.187500006828,-1.8898197019151E-14));
#7907=CARTESIAN_POINT('Ctrl Pts',(-48.706329375,46.9791666734946,-13.0508216223155));
#7908=CARTESIAN_POINT('Ctrl Pts',(-42.1809185638422,46.7708333401613,-24.3531646875));
#7909=CARTESIAN_POINT('Ctrl Pts',(-35.6555077526845,46.562500006828,-35.6555077526845));
#7910=CARTESIAN_POINT('Ctrl Pts',(-24.3531646875,46.3541666734946,-42.1809185638423));
#7911=CARTESIAN_POINT('Ctrl Pts',(-13.0508216223155,46.1458333401613,-48.706329375));
#7912=CARTESIAN_POINT('Ctrl Pts',(1.59157945007855E-14,45.937500006828,
-48.706329375));
#7913=CARTESIAN_POINT('Ctrl Pts',(13.0508216223155,45.7291666734946,-48.706329375));
#7914=CARTESIAN_POINT('Ctrl Pts',(24.3531646875,45.5208333401613,-42.1809185638422));
#7915=CARTESIAN_POINT('Ctrl Pts',(35.6555077526845,45.312500006828,-35.6555077526845));
#7916=CARTESIAN_POINT('Ctrl Pts',(42.1809185638422,45.1041666734946,-24.3531646875));
#7917=CARTESIAN_POINT('Ctrl Pts',(48.706329375,44.8958333401613,-13.0508216223155));
#7918=CARTESIAN_POINT('Ctrl Pts',(48.706329375,44.687500006828,1.293339198242E-14));
#7919=CARTESIAN_POINT('Ctrl Pts',(48.706329375,44.4791666734946,13.0508216223155));
#7920=CARTESIAN_POINT('Ctrl Pts',(42.1809185638422,44.2708333401613,24.3531646875));
#7921=CARTESIAN_POINT('Ctrl Pts',(35.6555077526845,44.062500006828,35.6555077526845));
#7922=CARTESIAN_POINT('Ctrl Pts',(24.3531646875,43.8541666734946,42.1809185638422));
#7923=CARTESIAN_POINT('Ctrl Pts',(13.0508216223155,43.6458333401613,48.706329375));
#7924=CARTESIAN_POINT('Ctrl Pts',(-9.95098946405443E-15,43.437500006828,
48.706329375));
#7925=CARTESIAN_POINT('Ctrl Pts',(-13.0508216223155,43.2291666734946,48.706329375));
#7926=CARTESIAN_POINT('Ctrl Pts',(-24.3531646875,43.0208333401613,42.1809185638423));
#7927=CARTESIAN_POINT('Ctrl Pts',(-35.6555077526845,42.812500006828,35.6555077526845));
#7928=CARTESIAN_POINT('Ctrl Pts',(-42.1809185638422,42.6041666734946,24.3531646875));
#7929=CARTESIAN_POINT('Ctrl Pts',(-48.706329375,42.3958333401613,13.0508216223155));
#7930=CARTESIAN_POINT('Ctrl Pts',(-48.706329375,42.187500006828,-1.8898197019151E-14));
#7931=CARTESIAN_POINT('Ctrl Pts',(-48.706329375,41.9791666734946,-13.0508216223155));
#7932=CARTESIAN_POINT('Ctrl Pts',(-42.1809185638422,41.7708333401613,-24.3531646875));
#7933=CARTESIAN_POINT('Ctrl Pts',(-35.6555077526845,41.562500006828,-35.6555077526845));
#7934=CARTESIAN_POINT('Ctrl Pts',(-24.3531646875,41.3541666734946,-42.1809185638423));
#7935=CARTESIAN_POINT('Ctrl Pts',(-13.0508216223155,41.1458333401613,-48.706329375));
#7936=CARTESIAN_POINT('Ctrl Pts',(1.59157945007855E-14,40.937500006828,
-48.706329375));
#7937=CARTESIAN_POINT('Ctrl Pts',(13.0508216223155,40.7291666734946,-48.706329375));
#7938=CARTESIAN_POINT('Ctrl Pts',(24.3531646875,40.5208333401613,-42.1809185638422));
#7939=CARTESIAN_POINT('Ctrl Pts',(35.6555077526845,40.312500006828,-35.6555077526845));
#7940=CARTESIAN_POINT('Ctrl Pts',(42.1809185638422,40.1041666734946,-24.3531646875));
#7941=CARTESIAN_POINT('Ctrl Pts',(48.706329375,39.8958333401613,-13.0508216223155));
#7942=CARTESIAN_POINT('Ctrl Pts',(48.706329375,39.687500006828,1.293339198242E-14));
#7943=CARTESIAN_POINT('Ctrl Pts',(48.706329375,39.4791666734946,13.0508216223155));
#7944=CARTESIAN_POINT('Ctrl Pts',(42.1809185638422,39.2708333401613,24.3531646875));
#7945=CARTESIAN_POINT('Ctrl Pts',(35.6555077526845,39.062500006828,35.6555077526845));
#7946=CARTESIAN_POINT('Ctrl Pts',(24.3531646875,38.8541666734946,42.1809185638422));
#7947=CARTESIAN_POINT('Ctrl Pts',(13.0508216223155,38.6458333401613,48.706329375));
#7948=CARTESIAN_POINT('Ctrl Pts',(-9.95098946405443E-15,38.437500006828,
48.706329375));
#7949=CARTESIAN_POINT('Ctrl Pts',(-13.0508216223155,38.2291666734946,48.706329375));
#7950=CARTESIAN_POINT('Ctrl Pts',(-24.3531646875,38.0208333401613,42.1809185638423));
#7951=CARTESIAN_POINT('Ctrl Pts',(-35.6555077526845,37.812500006828,35.6555077526845));
#7952=CARTESIAN_POINT('Ctrl Pts',(-42.1809185638422,37.6041666734946,24.3531646875));
#7953=CARTESIAN_POINT('Ctrl Pts',(-48.706329375,37.3958333401613,13.0508216223155));
#7954=CARTESIAN_POINT('Ctrl Pts',(-48.706329375,37.187500006828,-1.8898197019151E-14));
#7955=CARTESIAN_POINT('Ctrl Pts',(-48.706329375,36.9791666734946,-13.0508216223155));
#7956=CARTESIAN_POINT('Ctrl Pts',(-42.1809185638422,36.7708333401613,-24.3531646875));
#7957=CARTESIAN_POINT('Ctrl Pts',(-35.6555077526845,36.562500006828,-35.6555077526845));
#7958=CARTESIAN_POINT('Ctrl Pts',(-24.3531646875,36.3541666734946,-42.1809185638423));
#7959=CARTESIAN_POINT('Ctrl Pts',(-13.0508216223155,36.1458333401613,-48.706329375));
#7960=CARTESIAN_POINT('Ctrl Pts',(1.59157945007855E-14,35.937500006828,
-48.706329375));
#7961=CARTESIAN_POINT('Ctrl Pts',(13.0508216223155,35.7291666734946,-48.706329375));
#7962=CARTESIAN_POINT('Ctrl Pts',(24.3531646875,35.5208333401613,-42.1809185638422));
#7963=CARTESIAN_POINT('Ctrl Pts',(35.6555077526845,35.312500006828,-35.6555077526845));
#7964=CARTESIAN_POINT('Ctrl Pts',(42.1809185638422,35.1041666734946,-24.3531646875));
#7965=CARTESIAN_POINT('Ctrl Pts',(48.706329375,34.8958333401613,-13.0508216223155));
#7966=CARTESIAN_POINT('Ctrl Pts',(48.706329375,34.687500006828,1.293339198242E-14));
#7967=CARTESIAN_POINT('Ctrl Pts',(48.706329375,34.4791666734946,13.0508216223155));
#7968=CARTESIAN_POINT('Ctrl Pts',(42.1809185638422,34.2708333401613,24.3531646875));
#7969=CARTESIAN_POINT('Ctrl Pts',(35.6555077526845,34.062500006828,35.6555077526845));
#7970=CARTESIAN_POINT('Ctrl Pts',(24.3531646875,33.8541666734946,42.1809185638422));
#7971=CARTESIAN_POINT('Ctrl Pts',(13.0508216223155,33.6458333401613,48.706329375));
#7972=CARTESIAN_POINT('Ctrl Pts',(-9.95098946405443E-15,33.437500006828,
48.706329375));
#7973=CARTESIAN_POINT('Ctrl Pts',(-13.0508216223155,33.2291666734946,48.706329375));
#7974=CARTESIAN_POINT('Ctrl Pts',(-24.3531646875,33.0208333401613,42.1809185638423));
#7975=CARTESIAN_POINT('Ctrl Pts',(-35.6555077526845,32.812500006828,35.6555077526845));
#7976=CARTESIAN_POINT('Ctrl Pts',(-42.1809185638422,32.6041666734946,24.3531646875));
#7977=CARTESIAN_POINT('Ctrl Pts',(-48.706329375,32.3958333401613,13.0508216223155));
#7978=CARTESIAN_POINT('Ctrl Pts',(-48.706329375,32.187500006828,-1.8898197019151E-14));
#7979=CARTESIAN_POINT('Ctrl Pts',(-48.706329375,31.9791666734946,-13.0508216223155));
#7980=CARTESIAN_POINT('Ctrl Pts',(-42.1809185638422,31.7708333401613,-24.3531646875));
#7981=CARTESIAN_POINT('Ctrl Pts',(-35.6555077526845,31.562500006828,-35.6555077526845));
#7982=CARTESIAN_POINT('Ctrl Pts',(-24.3531646875,31.3541666734946,-42.1809185638423));
#7983=CARTESIAN_POINT('Ctrl Pts',(-13.0508216223155,31.1458333401613,-48.706329375));
#7984=CARTESIAN_POINT('Ctrl Pts',(1.59157945007855E-14,30.937500006828,
-48.706329375));
#7985=CARTESIAN_POINT('Ctrl Pts',(13.0508216223155,30.7291666734946,-48.706329375));
#7986=CARTESIAN_POINT('Ctrl Pts',(24.3531646875,30.5208333401613,-42.1809185638422));
#7987=CARTESIAN_POINT('Ctrl Pts',(35.6555077526845,30.312500006828,-35.6555077526845));
#7988=CARTESIAN_POINT('Ctrl Pts',(42.1809185638422,30.1041666734946,-24.3531646875));
#7989=CARTESIAN_POINT('Ctrl Pts',(48.706329375,29.8958333401613,-13.0508216223155));
#7990=CARTESIAN_POINT('Ctrl Pts',(48.706329375,29.687500006828,1.293339198242E-14));
#7991=CARTESIAN_POINT('Ctrl Pts',(48.706329375,29.4791666734946,13.0508216223155));
#7992=CARTESIAN_POINT('Ctrl Pts',(42.1809185638422,29.2708333401613,24.3531646875));
#7993=CARTESIAN_POINT('Ctrl Pts',(35.6555077526845,29.062500006828,35.6555077526845));
#7994=CARTESIAN_POINT('Ctrl Pts',(24.3531646875,28.8541666734946,42.1809185638422));
#7995=CARTESIAN_POINT('Ctrl Pts',(13.0508216223155,28.6458333401613,48.706329375));
#7996=CARTESIAN_POINT('Ctrl Pts',(-9.95098946405443E-15,28.437500006828,
48.706329375));
#7997=CARTESIAN_POINT('Ctrl Pts',(-13.0508216223155,28.2291666734946,48.706329375));
#7998=CARTESIAN_POINT('Ctrl Pts',(-24.3531646875,28.0208333401613,42.1809185638423));
#7999=CARTESIAN_POINT('Ctrl Pts',(-35.6555077526845,27.812500006828,35.6555077526845));
#8000=CARTESIAN_POINT('Ctrl Pts',(-42.1809185638422,27.6041666734946,24.3531646875));
#8001=CARTESIAN_POINT('Ctrl Pts',(-48.706329375,27.3958333401613,13.0508216223155));
#8002=CARTESIAN_POINT('Ctrl Pts',(-48.706329375,27.187500006828,-1.8898197019151E-14));
#8003=CARTESIAN_POINT('',(48.5725845633798,39.6293483229262,3.60701400320329));
#8004=CARTESIAN_POINT('Ctrl Pts',(45.858362923034,38.0633913333999,3.60701400320327));
#8005=CARTESIAN_POINT('Ctrl Pts',(46.0899257719339,38.1969849680263,3.60701400320326));
#8006=CARTESIAN_POINT('Ctrl Pts',(46.5530501979845,38.4641744416604,3.60701400320347));
#8007=CARTESIAN_POINT('Ctrl Pts',(47.0161721905706,38.7313681332063,3.60701400320335));
#8008=CARTESIAN_POINT('Ctrl Pts',(47.6893519862319,39.1197565257476,3.60701400320335));
#8009=CARTESIAN_POINT('Ctrl Pts',(48.1309692507095,39.3745507329179,3.60701400320329));
#8010=CARTESIAN_POINT('Ctrl Pts',(48.5725845633798,39.6293483229262,3.60701400320329));
#8011=CARTESIAN_POINT('',(3.61292728433799,38.4957479656467,48.5721450795008));
#8012=CARTESIAN_POINT('Ctrl Pts',(48.5725845633798,39.6293483229262,3.60701400320329));
#8013=CARTESIAN_POINT('Ctrl Pts',(47.7480251419552,39.4485714020251,14.7106532430575));
#8014=CARTESIAN_POINT('Ctrl Pts',(42.1809185638422,39.2708333401613,24.3531646875));
#8015=CARTESIAN_POINT('Ctrl Pts',(35.6555077526845,39.062500006828,35.6555077526845));
#8016=CARTESIAN_POINT('Ctrl Pts',(24.3531646875,38.8541666734946,42.1809185638422));
#8017=CARTESIAN_POINT('Ctrl Pts',(14.7133549689477,38.6764784118853,47.7464652997852));
#8018=CARTESIAN_POINT('Ctrl Pts',(3.61292728433799,38.4957479656467,48.5721450795008));
#8019=CARTESIAN_POINT('',(3.61293045337837,36.9438035980764,45.8702489620438));
#8020=CARTESIAN_POINT('Ctrl Pts',(3.61292728433799,38.4957479656467,48.5721450795008));
#8021=CARTESIAN_POINT('Ctrl Pts',(3.61292728433799,38.3625660950884,48.3403451622817));
#8022=CARTESIAN_POINT('Ctrl Pts',(3.61292728433799,38.2293911846469,48.1085412459393));
#8023=CARTESIAN_POINT('Ctrl Pts',(3.61292728433799,38.0962235420553,47.8767331545518));
#8024=CARTESIAN_POINT('Ctrl Pts',(3.61292728433799,37.9630558994543,47.6449250631479));
#8025=CARTESIAN_POINT('Ctrl Pts',(3.61292728433799,37.8298955244832,47.4131127965212));
#8026=CARTESIAN_POINT('Ctrl Pts',(3.61292728433799,37.6967427432646,47.1812961682826));
#8027=CARTESIAN_POINT('Ctrl Pts',(3.61292728433799,37.4457351673773,46.7442964348035));
#8028=CARTESIAN_POINT('Ctrl Pts',(3.61292728433799,37.1947545598528,46.3072812097023));
#8029=CARTESIAN_POINT('Ctrl Pts',(3.61292728433799,36.9438035983105,45.8702489624514));
#8030=CARTESIAN_POINT('',(3.61293362241916,36.9438035983105,45.8702489624514));
#8031=CARTESIAN_POINT('Ctrl Pts',(-46.,55.6250000136559,0.));
#8032=CARTESIAN_POINT('Ctrl Pts',(-46.,55.4166666803226,-12.3256628518316));
#8033=CARTESIAN_POINT('Ctrl Pts',(-39.8371685740842,55.2083333469893,-23.));
#8034=CARTESIAN_POINT('Ctrl Pts',(-33.6743371481684,55.0000000136559,-33.6743371481684));
#8035=CARTESIAN_POINT('Ctrl Pts',(-23.,54.7916666803226,-39.8371685740842));
#8036=CARTESIAN_POINT('Ctrl Pts',(-12.3256628518317,54.5833333469893,-46.));
#8037=CARTESIAN_POINT('Ctrl Pts',(-2.81668763803891E-15,54.3750000136559,
-46.));
#8038=CARTESIAN_POINT('Ctrl Pts',(12.3256628518316,54.1666666803226,-46.));
#8039=CARTESIAN_POINT('Ctrl Pts',(23.,53.9583333469893,-39.8371685740842));
#8040=CARTESIAN_POINT('Ctrl Pts',(33.6743371481683,53.7500000136559,-33.6743371481684));
#8041=CARTESIAN_POINT('Ctrl Pts',(39.8371685740842,53.5416666803226,-23.));
#8042=CARTESIAN_POINT('Ctrl Pts',(46.,53.3333333469893,-12.3256628518317));
#8043=CARTESIAN_POINT('Ctrl Pts',(46.,53.1250000136559,-5.63337527607782E-15));
#8044=CARTESIAN_POINT('Ctrl Pts',(46.,52.9166666803226,12.3256628518316));
#8045=CARTESIAN_POINT('Ctrl Pts',(39.8371685740842,52.7083333469893,23.));
#8046=CARTESIAN_POINT('Ctrl Pts',(33.6743371481684,52.5000000136559,33.6743371481683));
#8047=CARTESIAN_POINT('Ctrl Pts',(23.,52.2916666803226,39.8371685740842));
#8048=CARTESIAN_POINT('Ctrl Pts',(12.3256628518317,52.0833333469893,46.));
#8049=CARTESIAN_POINT('Ctrl Pts',(8.45006291411674E-15,51.8750000136559,
46.));
#8050=CARTESIAN_POINT('Ctrl Pts',(-12.3256628518316,51.6666666803226,46.));
#8051=CARTESIAN_POINT('Ctrl Pts',(-23.,51.4583333469893,39.8371685740842));
#8052=CARTESIAN_POINT('Ctrl Pts',(-33.6743371481683,51.2500000136559,33.6743371481684));
#8053=CARTESIAN_POINT('Ctrl Pts',(-39.8371685740842,51.0416666803226,23.));
#8054=CARTESIAN_POINT('Ctrl Pts',(-46.,50.8333333469893,12.3256628518317));
#8055=CARTESIAN_POINT('Ctrl Pts',(-46.,50.6250000136559,0.));
#8056=CARTESIAN_POINT('Ctrl Pts',(-46.,50.4166666803226,-12.3256628518316));
#8057=CARTESIAN_POINT('Ctrl Pts',(-39.8371685740842,50.2083333469893,-23.));
#8058=CARTESIAN_POINT('Ctrl Pts',(-33.6743371481684,50.0000000136559,-33.6743371481684));
#8059=CARTESIAN_POINT('Ctrl Pts',(-23.,49.7916666803226,-39.8371685740842));
#8060=CARTESIAN_POINT('Ctrl Pts',(-12.3256628518317,49.5833333469893,-46.));
#8061=CARTESIAN_POINT('Ctrl Pts',(-2.81668763803891E-15,49.3750000136559,
-46.));
#8062=CARTESIAN_POINT('Ctrl Pts',(12.3256628518316,49.1666666803226,-46.));
#8063=CARTESIAN_POINT('Ctrl Pts',(23.,48.9583333469893,-39.8371685740842));
#8064=CARTESIAN_POINT('Ctrl Pts',(33.6743371481683,48.7500000136559,-33.6743371481684));
#8065=CARTESIAN_POINT('Ctrl Pts',(39.8371685740842,48.5416666803226,-23.));
#8066=CARTESIAN_POINT('Ctrl Pts',(46.,48.3333333469893,-12.3256628518317));
#8067=CARTESIAN_POINT('Ctrl Pts',(46.,48.1250000136559,-5.63337527607782E-15));
#8068=CARTESIAN_POINT('Ctrl Pts',(46.,47.9166666803226,12.3256628518316));
#8069=CARTESIAN_POINT('Ctrl Pts',(39.8371685740842,47.7083333469893,23.));
#8070=CARTESIAN_POINT('Ctrl Pts',(33.6743371481684,47.5000000136559,33.6743371481683));
#8071=CARTESIAN_POINT('Ctrl Pts',(23.,47.2916666803226,39.8371685740842));
#8072=CARTESIAN_POINT('Ctrl Pts',(12.3256628518317,47.0833333469893,46.));
#8073=CARTESIAN_POINT('Ctrl Pts',(8.45006291411674E-15,46.8750000136559,
46.));
#8074=CARTESIAN_POINT('Ctrl Pts',(-12.3256628518316,46.6666666803226,46.));
#8075=CARTESIAN_POINT('Ctrl Pts',(-23.,46.4583333469893,39.8371685740842));
#8076=CARTESIAN_POINT('Ctrl Pts',(-33.6743371481683,46.2500000136559,33.6743371481684));
#8077=CARTESIAN_POINT('Ctrl Pts',(-39.8371685740842,46.0416666803226,23.));
#8078=CARTESIAN_POINT('Ctrl Pts',(-46.,45.8333333469892,12.3256628518317));
#8079=CARTESIAN_POINT('Ctrl Pts',(-46.,45.6250000136559,0.));
#8080=CARTESIAN_POINT('Ctrl Pts',(-46.,45.4166666803226,-12.3256628518316));
#8081=CARTESIAN_POINT('Ctrl Pts',(-39.8371685740842,45.2083333469893,-23.));
#8082=CARTESIAN_POINT('Ctrl Pts',(-33.6743371481684,45.0000000136559,-33.6743371481684));
#8083=CARTESIAN_POINT('Ctrl Pts',(-23.,44.7916666803226,-39.8371685740842));
#8084=CARTESIAN_POINT('Ctrl Pts',(-12.3256628518317,44.5833333469893,-46.));
#8085=CARTESIAN_POINT('Ctrl Pts',(-2.81668763803891E-15,44.3750000136559,
-46.));
#8086=CARTESIAN_POINT('Ctrl Pts',(12.3256628518316,44.1666666803226,-46.));
#8087=CARTESIAN_POINT('Ctrl Pts',(23.,43.9583333469893,-39.8371685740842));
#8088=CARTESIAN_POINT('Ctrl Pts',(33.6743371481683,43.7500000136559,-33.6743371481684));
#8089=CARTESIAN_POINT('Ctrl Pts',(39.8371685740842,43.5416666803226,-23.));
#8090=CARTESIAN_POINT('Ctrl Pts',(46.,43.3333333469893,-12.3256628518317));
#8091=CARTESIAN_POINT('Ctrl Pts',(46.,43.1250000136559,-5.63337527607782E-15));
#8092=CARTESIAN_POINT('Ctrl Pts',(46.,42.9166666803226,12.3256628518316));
#8093=CARTESIAN_POINT('Ctrl Pts',(39.8371685740842,42.7083333469893,23.));
#8094=CARTESIAN_POINT('Ctrl Pts',(33.6743371481684,42.5000000136559,33.6743371481683));
#8095=CARTESIAN_POINT('Ctrl Pts',(23.,42.2916666803226,39.8371685740842));
#8096=CARTESIAN_POINT('Ctrl Pts',(12.3256628518317,42.0833333469893,46.));
#8097=CARTESIAN_POINT('Ctrl Pts',(8.45006291411674E-15,41.8750000136559,
46.));
#8098=CARTESIAN_POINT('Ctrl Pts',(-12.3256628518316,41.6666666803226,46.));
#8099=CARTESIAN_POINT('Ctrl Pts',(-23.,41.4583333469893,39.8371685740842));
#8100=CARTESIAN_POINT('Ctrl Pts',(-33.6743371481683,41.2500000136559,33.6743371481684));
#8101=CARTESIAN_POINT('Ctrl Pts',(-39.8371685740842,41.0416666803226,23.));
#8102=CARTESIAN_POINT('Ctrl Pts',(-46.,40.8333333469893,12.3256628518317));
#8103=CARTESIAN_POINT('Ctrl Pts',(-46.,40.6250000136559,0.));
#8104=CARTESIAN_POINT('Ctrl Pts',(-46.,40.4166666803226,-12.3256628518316));
#8105=CARTESIAN_POINT('Ctrl Pts',(-39.8371685740842,40.2083333469893,-23.));
#8106=CARTESIAN_POINT('Ctrl Pts',(-33.6743371481684,40.0000000136559,-33.6743371481684));
#8107=CARTESIAN_POINT('Ctrl Pts',(-23.,39.7916666803226,-39.8371685740842));
#8108=CARTESIAN_POINT('Ctrl Pts',(-12.3256628518317,39.5833333469893,-46.));
#8109=CARTESIAN_POINT('Ctrl Pts',(-2.81668763803891E-15,39.3750000136559,
-46.));
#8110=CARTESIAN_POINT('Ctrl Pts',(12.3256628518316,39.1666666803226,-46.));
#8111=CARTESIAN_POINT('Ctrl Pts',(23.,38.9583333469893,-39.8371685740842));
#8112=CARTESIAN_POINT('Ctrl Pts',(33.6743371481683,38.7500000136559,-33.6743371481684));
#8113=CARTESIAN_POINT('Ctrl Pts',(39.8371685740842,38.5416666803226,-23.));
#8114=CARTESIAN_POINT('Ctrl Pts',(46.,38.3333333469893,-12.3256628518317));
#8115=CARTESIAN_POINT('Ctrl Pts',(46.,38.1250000136559,-5.63337527607782E-15));
#8116=CARTESIAN_POINT('Ctrl Pts',(46.,37.9166666803226,12.3256628518316));
#8117=CARTESIAN_POINT('Ctrl Pts',(39.8371685740842,37.7083333469893,23.));
#8118=CARTESIAN_POINT('Ctrl Pts',(33.6743371481684,37.5000000136559,33.6743371481683));
#8119=CARTESIAN_POINT('Ctrl Pts',(23.,37.2916666803226,39.8371685740842));
#8120=CARTESIAN_POINT('Ctrl Pts',(12.3256628518317,37.0833333469893,46.));
#8121=CARTESIAN_POINT('Ctrl Pts',(8.45006291411674E-15,36.8750000136559,
46.));
#8122=CARTESIAN_POINT('Ctrl Pts',(-12.3256628518316,36.6666666803226,46.));
#8123=CARTESIAN_POINT('Ctrl Pts',(-23.,36.4583333469893,39.8371685740842));
#8124=CARTESIAN_POINT('Ctrl Pts',(-33.6743371481683,36.2500000136559,33.6743371481684));
#8125=CARTESIAN_POINT('Ctrl Pts',(-39.8371685740842,36.0416666803226,23.));
#8126=CARTESIAN_POINT('Ctrl Pts',(-46.,35.8333333469893,12.3256628518317));
#8127=CARTESIAN_POINT('Ctrl Pts',(-46.,35.6250000136559,0.));
#8128=CARTESIAN_POINT('Ctrl Pts',(-46.,35.4166666803226,-12.3256628518316));
#8129=CARTESIAN_POINT('Ctrl Pts',(-39.8371685740842,35.2083333469893,-23.));
#8130=CARTESIAN_POINT('Ctrl Pts',(-33.6743371481684,35.0000000136559,-33.6743371481684));
#8131=CARTESIAN_POINT('Ctrl Pts',(-23.,34.7916666803226,-39.8371685740842));
#8132=CARTESIAN_POINT('Ctrl Pts',(-12.3256628518317,34.5833333469893,-46.));
#8133=CARTESIAN_POINT('Ctrl Pts',(-2.81668763803891E-15,34.3750000136559,
-46.));
#8134=CARTESIAN_POINT('Ctrl Pts',(12.3256628518316,34.1666666803226,-46.));
#8135=CARTESIAN_POINT('Ctrl Pts',(23.,33.9583333469893,-39.8371685740842));
#8136=CARTESIAN_POINT('Ctrl Pts',(33.6743371481683,33.7500000136559,-33.6743371481684));
#8137=CARTESIAN_POINT('Ctrl Pts',(39.8371685740842,33.5416666803226,-23.));
#8138=CARTESIAN_POINT('Ctrl Pts',(46.,33.3333333469893,-12.3256628518317));
#8139=CARTESIAN_POINT('Ctrl Pts',(46.,33.1250000136559,-5.63337527607782E-15));
#8140=CARTESIAN_POINT('Ctrl Pts',(46.,32.9166666803226,12.3256628518316));
#8141=CARTESIAN_POINT('Ctrl Pts',(39.8371685740842,32.7083333469893,23.));
#8142=CARTESIAN_POINT('Ctrl Pts',(33.6743371481684,32.5000000136559,33.6743371481683));
#8143=CARTESIAN_POINT('Ctrl Pts',(23.,32.2916666803226,39.8371685740842));
#8144=CARTESIAN_POINT('Ctrl Pts',(12.3256628518317,32.0833333469893,46.));
#8145=CARTESIAN_POINT('Ctrl Pts',(8.45006291411674E-15,31.8750000136559,
46.));
#8146=CARTESIAN_POINT('Ctrl Pts',(-12.3256628518316,31.6666666803226,46.));
#8147=CARTESIAN_POINT('Ctrl Pts',(-23.,31.4583333469893,39.8371685740842));
#8148=CARTESIAN_POINT('Ctrl Pts',(-33.6743371481683,31.2500000136559,33.6743371481684));
#8149=CARTESIAN_POINT('Ctrl Pts',(-39.8371685740842,31.0416666803226,23.));
#8150=CARTESIAN_POINT('Ctrl Pts',(-46.,30.8333333469893,12.3256628518317));
#8151=CARTESIAN_POINT('Ctrl Pts',(-46.,30.6250000136559,0.));
#8152=CARTESIAN_POINT('Ctrl Pts',(-46.,30.4166666803226,-12.3256628518316));
#8153=CARTESIAN_POINT('Ctrl Pts',(-39.8371685740842,30.2083333469893,-23.));
#8154=CARTESIAN_POINT('Ctrl Pts',(-33.6743371481684,30.0000000136559,-33.6743371481684));
#8155=CARTESIAN_POINT('Ctrl Pts',(-23.,29.7916666803226,-39.8371685740842));
#8156=CARTESIAN_POINT('Ctrl Pts',(-12.3256628518317,29.5833333469893,-46.));
#8157=CARTESIAN_POINT('Ctrl Pts',(-2.81668763803891E-15,29.3750000136559,
-46.));
#8158=CARTESIAN_POINT('Ctrl Pts',(12.3256628518316,29.1666666803226,-46.));
#8159=CARTESIAN_POINT('Ctrl Pts',(23.,28.9583333469893,-39.8371685740842));
#8160=CARTESIAN_POINT('Ctrl Pts',(33.6743371481683,28.7500000136559,-33.6743371481684));
#8161=CARTESIAN_POINT('Ctrl Pts',(39.8371685740842,28.5416666803226,-23.));
#8162=CARTESIAN_POINT('Ctrl Pts',(46.,28.3333333469893,-12.3256628518317));
#8163=CARTESIAN_POINT('Ctrl Pts',(46.,28.1250000136559,-5.63337527607782E-15));
#8164=CARTESIAN_POINT('Ctrl Pts',(46.,27.9166666803226,12.3256628518316));
#8165=CARTESIAN_POINT('Ctrl Pts',(39.8371685740842,27.7083333469893,23.));
#8166=CARTESIAN_POINT('Ctrl Pts',(33.6743371481684,27.5000000136559,33.6743371481683));
#8167=CARTESIAN_POINT('Ctrl Pts',(23.,27.2916666803226,39.8371685740842));
#8168=CARTESIAN_POINT('Ctrl Pts',(12.3256628518317,27.0833333469893,46.));
#8169=CARTESIAN_POINT('Ctrl Pts',(8.45006291411674E-15,26.8750000136559,
46.));
#8170=CARTESIAN_POINT('Ctrl Pts',(-12.3256628518316,26.6666666803226,46.));
#8171=CARTESIAN_POINT('Ctrl Pts',(-23.,26.4583333469893,39.8371685740842));
#8172=CARTESIAN_POINT('Ctrl Pts',(-33.6743371481683,26.2500000136559,33.6743371481684));
#8173=CARTESIAN_POINT('Ctrl Pts',(-39.8371685740842,26.0416666803226,23.));
#8174=CARTESIAN_POINT('Ctrl Pts',(-46.,25.8333333469893,12.3256628518317));
#8175=CARTESIAN_POINT('Ctrl Pts',(-46.,25.6250000136559,0.));
#8176=CARTESIAN_POINT('Ctrl Pts',(-48.706329375,57.187500006828,-1.8898197019151E-14));
#8177=CARTESIAN_POINT('Ctrl Pts',(-48.706329375,56.9791666734946,-13.0508216223155));
#8178=CARTESIAN_POINT('Ctrl Pts',(-42.1809185638422,56.7708333401613,-24.3531646875));
#8179=CARTESIAN_POINT('Ctrl Pts',(-35.6555077526845,56.562500006828,-35.6555077526845));
#8180=CARTESIAN_POINT('Ctrl Pts',(-24.3531646875,56.3541666734946,-42.1809185638423));
#8181=CARTESIAN_POINT('Ctrl Pts',(-13.0508216223155,56.1458333401613,-48.706329375));
#8182=CARTESIAN_POINT('Ctrl Pts',(1.59157945007855E-14,55.937500006828,
-48.706329375));
#8183=CARTESIAN_POINT('Ctrl Pts',(13.0508216223155,55.7291666734946,-48.706329375));
#8184=CARTESIAN_POINT('Ctrl Pts',(24.3531646875,55.5208333401613,-42.1809185638422));
#8185=CARTESIAN_POINT('Ctrl Pts',(35.6555077526845,55.312500006828,-35.6555077526845));
#8186=CARTESIAN_POINT('Ctrl Pts',(42.1809185638422,55.1041666734946,-24.3531646875));
#8187=CARTESIAN_POINT('Ctrl Pts',(48.706329375,54.8958333401613,-13.0508216223155));
#8188=CARTESIAN_POINT('Ctrl Pts',(48.706329375,54.687500006828,1.293339198242E-14));
#8189=CARTESIAN_POINT('Ctrl Pts',(48.706329375,54.4791666734946,13.0508216223155));
#8190=CARTESIAN_POINT('Ctrl Pts',(42.1809185638422,54.2708333401613,24.3531646875));
#8191=CARTESIAN_POINT('Ctrl Pts',(35.6555077526845,54.062500006828,35.6555077526845));
#8192=CARTESIAN_POINT('Ctrl Pts',(24.3531646875,53.8541666734946,42.1809185638422));
#8193=CARTESIAN_POINT('Ctrl Pts',(13.0508216223155,53.6458333401613,48.706329375));
#8194=CARTESIAN_POINT('Ctrl Pts',(-9.95098946405443E-15,53.437500006828,
48.706329375));
#8195=CARTESIAN_POINT('Ctrl Pts',(-13.0508216223155,53.2291666734946,48.706329375));
#8196=CARTESIAN_POINT('Ctrl Pts',(-24.3531646875,53.0208333401613,42.1809185638423));
#8197=CARTESIAN_POINT('Ctrl Pts',(-35.6555077526845,52.812500006828,35.6555077526845));
#8198=CARTESIAN_POINT('Ctrl Pts',(-42.1809185638422,52.6041666734946,24.3531646875));
#8199=CARTESIAN_POINT('Ctrl Pts',(-48.706329375,52.3958333401613,13.0508216223155));
#8200=CARTESIAN_POINT('Ctrl Pts',(-48.706329375,52.187500006828,-1.8898197019151E-14));
#8201=CARTESIAN_POINT('Ctrl Pts',(-48.706329375,51.9791666734946,-13.0508216223155));
#8202=CARTESIAN_POINT('Ctrl Pts',(-42.1809185638422,51.7708333401613,-24.3531646875));
#8203=CARTESIAN_POINT('Ctrl Pts',(-35.6555077526845,51.562500006828,-35.6555077526845));
#8204=CARTESIAN_POINT('Ctrl Pts',(-24.3531646875,51.3541666734946,-42.1809185638423));
#8205=CARTESIAN_POINT('Ctrl Pts',(-13.0508216223155,51.1458333401613,-48.706329375));
#8206=CARTESIAN_POINT('Ctrl Pts',(1.59157945007855E-14,50.937500006828,
-48.706329375));
#8207=CARTESIAN_POINT('Ctrl Pts',(13.0508216223155,50.7291666734946,-48.706329375));
#8208=CARTESIAN_POINT('Ctrl Pts',(24.3531646875,50.5208333401613,-42.1809185638422));
#8209=CARTESIAN_POINT('Ctrl Pts',(35.6555077526845,50.312500006828,-35.6555077526845));
#8210=CARTESIAN_POINT('Ctrl Pts',(42.1809185638422,50.1041666734946,-24.3531646875));
#8211=CARTESIAN_POINT('Ctrl Pts',(48.706329375,49.8958333401613,-13.0508216223155));
#8212=CARTESIAN_POINT('Ctrl Pts',(48.706329375,49.687500006828,1.293339198242E-14));
#8213=CARTESIAN_POINT('Ctrl Pts',(48.706329375,49.4791666734946,13.0508216223155));
#8214=CARTESIAN_POINT('Ctrl Pts',(42.1809185638422,49.2708333401613,24.3531646875));
#8215=CARTESIAN_POINT('Ctrl Pts',(35.6555077526845,49.062500006828,35.6555077526845));
#8216=CARTESIAN_POINT('Ctrl Pts',(24.3531646875,48.8541666734946,42.1809185638422));
#8217=CARTESIAN_POINT('Ctrl Pts',(13.0508216223155,48.6458333401613,48.706329375));
#8218=CARTESIAN_POINT('Ctrl Pts',(-9.95098946405443E-15,48.437500006828,
48.706329375));
#8219=CARTESIAN_POINT('Ctrl Pts',(-13.0508216223155,48.2291666734946,48.706329375));
#8220=CARTESIAN_POINT('Ctrl Pts',(-24.3531646875,48.0208333401613,42.1809185638423));
#8221=CARTESIAN_POINT('Ctrl Pts',(-35.6555077526845,47.812500006828,35.6555077526845));
#8222=CARTESIAN_POINT('Ctrl Pts',(-42.1809185638422,47.6041666734946,24.3531646875));
#8223=CARTESIAN_POINT('Ctrl Pts',(-48.706329375,47.3958333401613,13.0508216223155));
#8224=CARTESIAN_POINT('Ctrl Pts',(-48.706329375,47.187500006828,-1.8898197019151E-14));
#8225=CARTESIAN_POINT('Ctrl Pts',(-48.706329375,46.9791666734946,-13.0508216223155));
#8226=CARTESIAN_POINT('Ctrl Pts',(-42.1809185638422,46.7708333401613,-24.3531646875));
#8227=CARTESIAN_POINT('Ctrl Pts',(-35.6555077526845,46.562500006828,-35.6555077526845));
#8228=CARTESIAN_POINT('Ctrl Pts',(-24.3531646875,46.3541666734946,-42.1809185638423));
#8229=CARTESIAN_POINT('Ctrl Pts',(-13.0508216223155,46.1458333401613,-48.706329375));
#8230=CARTESIAN_POINT('Ctrl Pts',(1.59157945007855E-14,45.937500006828,
-48.706329375));
#8231=CARTESIAN_POINT('Ctrl Pts',(13.0508216223155,45.7291666734946,-48.706329375));
#8232=CARTESIAN_POINT('Ctrl Pts',(24.3531646875,45.5208333401613,-42.1809185638422));
#8233=CARTESIAN_POINT('Ctrl Pts',(35.6555077526845,45.312500006828,-35.6555077526845));
#8234=CARTESIAN_POINT('Ctrl Pts',(42.1809185638422,45.1041666734946,-24.3531646875));
#8235=CARTESIAN_POINT('Ctrl Pts',(48.706329375,44.8958333401613,-13.0508216223155));
#8236=CARTESIAN_POINT('Ctrl Pts',(48.706329375,44.687500006828,1.293339198242E-14));
#8237=CARTESIAN_POINT('Ctrl Pts',(48.706329375,44.4791666734946,13.0508216223155));
#8238=CARTESIAN_POINT('Ctrl Pts',(42.1809185638422,44.2708333401613,24.3531646875));
#8239=CARTESIAN_POINT('Ctrl Pts',(35.6555077526845,44.062500006828,35.6555077526845));
#8240=CARTESIAN_POINT('Ctrl Pts',(24.3531646875,43.8541666734946,42.1809185638422));
#8241=CARTESIAN_POINT('Ctrl Pts',(13.0508216223155,43.6458333401613,48.706329375));
#8242=CARTESIAN_POINT('Ctrl Pts',(-9.95098946405443E-15,43.437500006828,
48.706329375));
#8243=CARTESIAN_POINT('Ctrl Pts',(-13.0508216223155,43.2291666734946,48.706329375));
#8244=CARTESIAN_POINT('Ctrl Pts',(-24.3531646875,43.0208333401613,42.1809185638423));
#8245=CARTESIAN_POINT('Ctrl Pts',(-35.6555077526845,42.812500006828,35.6555077526845));
#8246=CARTESIAN_POINT('Ctrl Pts',(-42.1809185638422,42.6041666734946,24.3531646875));
#8247=CARTESIAN_POINT('Ctrl Pts',(-48.706329375,42.3958333401613,13.0508216223155));
#8248=CARTESIAN_POINT('Ctrl Pts',(-48.706329375,42.187500006828,-1.8898197019151E-14));
#8249=CARTESIAN_POINT('Ctrl Pts',(-48.706329375,41.9791666734946,-13.0508216223155));
#8250=CARTESIAN_POINT('Ctrl Pts',(-42.1809185638422,41.7708333401613,-24.3531646875));
#8251=CARTESIAN_POINT('Ctrl Pts',(-35.6555077526845,41.562500006828,-35.6555077526845));
#8252=CARTESIAN_POINT('Ctrl Pts',(-24.3531646875,41.3541666734946,-42.1809185638423));
#8253=CARTESIAN_POINT('Ctrl Pts',(-13.0508216223155,41.1458333401613,-48.706329375));
#8254=CARTESIAN_POINT('Ctrl Pts',(1.59157945007855E-14,40.937500006828,
-48.706329375));
#8255=CARTESIAN_POINT('Ctrl Pts',(13.0508216223155,40.7291666734946,-48.706329375));
#8256=CARTESIAN_POINT('Ctrl Pts',(24.3531646875,40.5208333401613,-42.1809185638422));
#8257=CARTESIAN_POINT('Ctrl Pts',(35.6555077526845,40.312500006828,-35.6555077526845));
#8258=CARTESIAN_POINT('Ctrl Pts',(42.1809185638422,40.1041666734946,-24.3531646875));
#8259=CARTESIAN_POINT('Ctrl Pts',(48.706329375,39.8958333401613,-13.0508216223155));
#8260=CARTESIAN_POINT('Ctrl Pts',(48.706329375,39.687500006828,1.293339198242E-14));
#8261=CARTESIAN_POINT('Ctrl Pts',(48.706329375,39.4791666734946,13.0508216223155));
#8262=CARTESIAN_POINT('Ctrl Pts',(42.1809185638422,39.2708333401613,24.3531646875));
#8263=CARTESIAN_POINT('Ctrl Pts',(35.6555077526845,39.062500006828,35.6555077526845));
#8264=CARTESIAN_POINT('Ctrl Pts',(24.3531646875,38.8541666734946,42.1809185638422));
#8265=CARTESIAN_POINT('Ctrl Pts',(13.0508216223155,38.6458333401613,48.706329375));
#8266=CARTESIAN_POINT('Ctrl Pts',(-9.95098946405443E-15,38.437500006828,
48.706329375));
#8267=CARTESIAN_POINT('Ctrl Pts',(-13.0508216223155,38.2291666734946,48.706329375));
#8268=CARTESIAN_POINT('Ctrl Pts',(-24.3531646875,38.0208333401613,42.1809185638423));
#8269=CARTESIAN_POINT('Ctrl Pts',(-35.6555077526845,37.812500006828,35.6555077526845));
#8270=CARTESIAN_POINT('Ctrl Pts',(-42.1809185638422,37.6041666734946,24.3531646875));
#8271=CARTESIAN_POINT('Ctrl Pts',(-48.706329375,37.3958333401613,13.0508216223155));
#8272=CARTESIAN_POINT('Ctrl Pts',(-48.706329375,37.187500006828,-1.8898197019151E-14));
#8273=CARTESIAN_POINT('Ctrl Pts',(-48.706329375,36.9791666734946,-13.0508216223155));
#8274=CARTESIAN_POINT('Ctrl Pts',(-42.1809185638422,36.7708333401613,-24.3531646875));
#8275=CARTESIAN_POINT('Ctrl Pts',(-35.6555077526845,36.562500006828,-35.6555077526845));
#8276=CARTESIAN_POINT('Ctrl Pts',(-24.3531646875,36.3541666734946,-42.1809185638423));
#8277=CARTESIAN_POINT('Ctrl Pts',(-13.0508216223155,36.1458333401613,-48.706329375));
#8278=CARTESIAN_POINT('Ctrl Pts',(1.59157945007855E-14,35.937500006828,
-48.706329375));
#8279=CARTESIAN_POINT('Ctrl Pts',(13.0508216223155,35.7291666734946,-48.706329375));
#8280=CARTESIAN_POINT('Ctrl Pts',(24.3531646875,35.5208333401613,-42.1809185638422));
#8281=CARTESIAN_POINT('Ctrl Pts',(35.6555077526845,35.312500006828,-35.6555077526845));
#8282=CARTESIAN_POINT('Ctrl Pts',(42.1809185638422,35.1041666734946,-24.3531646875));
#8283=CARTESIAN_POINT('Ctrl Pts',(48.706329375,34.8958333401613,-13.0508216223155));
#8284=CARTESIAN_POINT('Ctrl Pts',(48.706329375,34.687500006828,1.293339198242E-14));
#8285=CARTESIAN_POINT('Ctrl Pts',(48.706329375,34.4791666734946,13.0508216223155));
#8286=CARTESIAN_POINT('Ctrl Pts',(42.1809185638422,34.2708333401613,24.3531646875));
#8287=CARTESIAN_POINT('Ctrl Pts',(35.6555077526845,34.062500006828,35.6555077526845));
#8288=CARTESIAN_POINT('Ctrl Pts',(24.3531646875,33.8541666734946,42.1809185638422));
#8289=CARTESIAN_POINT('Ctrl Pts',(13.0508216223155,33.6458333401613,48.706329375));
#8290=CARTESIAN_POINT('Ctrl Pts',(-9.95098946405443E-15,33.437500006828,
48.706329375));
#8291=CARTESIAN_POINT('Ctrl Pts',(-13.0508216223155,33.2291666734946,48.706329375));
#8292=CARTESIAN_POINT('Ctrl Pts',(-24.3531646875,33.0208333401613,42.1809185638423));
#8293=CARTESIAN_POINT('Ctrl Pts',(-35.6555077526845,32.812500006828,35.6555077526845));
#8294=CARTESIAN_POINT('Ctrl Pts',(-42.1809185638422,32.6041666734946,24.3531646875));
#8295=CARTESIAN_POINT('Ctrl Pts',(-48.706329375,32.3958333401613,13.0508216223155));
#8296=CARTESIAN_POINT('Ctrl Pts',(-48.706329375,32.187500006828,-1.8898197019151E-14));
#8297=CARTESIAN_POINT('Ctrl Pts',(-48.706329375,31.9791666734946,-13.0508216223155));
#8298=CARTESIAN_POINT('Ctrl Pts',(-42.1809185638422,31.7708333401613,-24.3531646875));
#8299=CARTESIAN_POINT('Ctrl Pts',(-35.6555077526845,31.562500006828,-35.6555077526845));
#8300=CARTESIAN_POINT('Ctrl Pts',(-24.3531646875,31.3541666734946,-42.1809185638423));
#8301=CARTESIAN_POINT('Ctrl Pts',(-13.0508216223155,31.1458333401613,-48.706329375));
#8302=CARTESIAN_POINT('Ctrl Pts',(1.59157945007855E-14,30.937500006828,
-48.706329375));
#8303=CARTESIAN_POINT('Ctrl Pts',(13.0508216223155,30.7291666734946,-48.706329375));
#8304=CARTESIAN_POINT('Ctrl Pts',(24.3531646875,30.5208333401613,-42.1809185638422));
#8305=CARTESIAN_POINT('Ctrl Pts',(35.6555077526845,30.312500006828,-35.6555077526845));
#8306=CARTESIAN_POINT('Ctrl Pts',(42.1809185638422,30.1041666734946,-24.3531646875));
#8307=CARTESIAN_POINT('Ctrl Pts',(48.706329375,29.8958333401613,-13.0508216223155));
#8308=CARTESIAN_POINT('Ctrl Pts',(48.706329375,29.687500006828,1.293339198242E-14));
#8309=CARTESIAN_POINT('Ctrl Pts',(48.706329375,29.4791666734946,13.0508216223155));
#8310=CARTESIAN_POINT('Ctrl Pts',(42.1809185638422,29.2708333401613,24.3531646875));
#8311=CARTESIAN_POINT('Ctrl Pts',(35.6555077526845,29.062500006828,35.6555077526845));
#8312=CARTESIAN_POINT('Ctrl Pts',(24.3531646875,28.8541666734946,42.1809185638422));
#8313=CARTESIAN_POINT('Ctrl Pts',(13.0508216223155,28.6458333401613,48.706329375));
#8314=CARTESIAN_POINT('Ctrl Pts',(-9.95098946405443E-15,28.437500006828,
48.706329375));
#8315=CARTESIAN_POINT('Ctrl Pts',(-13.0508216223155,28.2291666734946,48.706329375));
#8316=CARTESIAN_POINT('Ctrl Pts',(-24.3531646875,28.0208333401613,42.1809185638423));
#8317=CARTESIAN_POINT('Ctrl Pts',(-35.6555077526845,27.812500006828,35.6555077526845));
#8318=CARTESIAN_POINT('Ctrl Pts',(-42.1809185638422,27.6041666734946,24.3531646875));
#8319=CARTESIAN_POINT('Ctrl Pts',(-48.706329375,27.3958333401613,13.0508216223155));
#8320=CARTESIAN_POINT('Ctrl Pts',(-48.706329375,27.187500006828,-1.8898197019151E-14));
#8321=CARTESIAN_POINT('',(-48.3095415605567,56.9999999999858,-4.33048599679673));
#8322=CARTESIAN_POINT('Ctrl Pts',(-45.7957082162897,55.5508791552084,-4.33048599679673));
#8323=CARTESIAN_POINT('Ctrl Pts',(-46.027322302781,55.6843839384496,-4.33048599679673));
#8324=CARTESIAN_POINT('Ctrl Pts',(-46.4905476657728,55.9513983799647,-4.33048599679673));
#8325=CARTESIAN_POINT('Ctrl Pts',(-46.9537676533565,56.2184221466352,-4.33048599679673));
#8326=CARTESIAN_POINT('Ctrl Pts',(-47.5601013844768,56.5679517997618,-4.33048599679673));
#8327=CARTESIAN_POINT('Ctrl Pts',(-47.9348230422494,56.7839731770798,-4.33048599679673));
#8328=CARTESIAN_POINT('Ctrl Pts',(-48.3095415605567,56.9999999999858,-4.33048599679673));
#8329=CARTESIAN_POINT('',(-48.0678199532544,57.,-7.03922488851235));
#8330=CARTESIAN_POINT('Origin',(0.322758650769908,56.9999468614787,-1.35580654760172));
#8331=CARTESIAN_POINT('',(-48.3871149493437,57.0447214927916,-4.33048599679673));
#8332=CARTESIAN_POINT('Origin',(0.0124715173034229,56.9065257752989,0.00338253564322266));
#8333=CARTESIAN_POINT('',(-48.5134353784345,57.1175463684955,-4.33048599679673));
#8334=CARTESIAN_POINT('',(-48.3871149493437,57.0447214927916,-4.33048599679673));
#8335=CARTESIAN_POINT('',(-4.32456003949879,56.0073567866782,-48.5139639861634));
#8336=CARTESIAN_POINT('Ctrl Pts',(-48.5134353784344,57.1175463684955,-4.33048599679673));
#8337=CARTESIAN_POINT('Ctrl Pts',(-47.5573898704235,56.9424850907232,-15.0408432190651));
#8338=CARTESIAN_POINT('Ctrl Pts',(-42.1809185638422,56.7708333401613,-24.3531646875));
#8339=CARTESIAN_POINT('Ctrl Pts',(-35.6555077526845,56.562500006828,-35.6555077526845));
#8340=CARTESIAN_POINT('Ctrl Pts',(-24.3531646875,56.3541666734946,-42.1809185638423));
#8341=CARTESIAN_POINT('Ctrl Pts',(-15.038141415499,56.1824651212465,-47.5589497574396));
#8342=CARTESIAN_POINT('Ctrl Pts',(-4.32456003949879,56.0073567866783,-48.5139639861634));
#8343=CARTESIAN_POINT('Origin',(-4.32456007771086,8027.20453909234,4524.01087309897));
#8344=CARTESIAN_POINT('Ctrl Pts',(-46.,55.6250000136559,0.));
#8345=CARTESIAN_POINT('Ctrl Pts',(-46.,55.4166666803226,-12.3256628518316));
#8346=CARTESIAN_POINT('Ctrl Pts',(-39.8371685740842,55.2083333469893,-23.));
#8347=CARTESIAN_POINT('Ctrl Pts',(-33.6743371481684,55.0000000136559,-33.6743371481684));
#8348=CARTESIAN_POINT('Ctrl Pts',(-23.,54.7916666803226,-39.8371685740842));
#8349=CARTESIAN_POINT('Ctrl Pts',(-12.3256628518317,54.5833333469893,-46.));
#8350=CARTESIAN_POINT('Ctrl Pts',(-2.81668763803891E-15,54.3750000136559,
-46.));
#8351=CARTESIAN_POINT('Ctrl Pts',(12.3256628518316,54.1666666803226,-46.));
#8352=CARTESIAN_POINT('Ctrl Pts',(23.,53.9583333469893,-39.8371685740842));
#8353=CARTESIAN_POINT('Ctrl Pts',(33.6743371481683,53.7500000136559,-33.6743371481684));
#8354=CARTESIAN_POINT('Ctrl Pts',(39.8371685740842,53.5416666803226,-23.));
#8355=CARTESIAN_POINT('Ctrl Pts',(46.,53.3333333469893,-12.3256628518317));
#8356=CARTESIAN_POINT('Ctrl Pts',(46.,53.1250000136559,-5.63337527607782E-15));
#8357=CARTESIAN_POINT('Ctrl Pts',(46.,52.9166666803226,12.3256628518316));
#8358=CARTESIAN_POINT('Ctrl Pts',(39.8371685740842,52.7083333469893,23.));
#8359=CARTESIAN_POINT('Ctrl Pts',(33.6743371481684,52.5000000136559,33.6743371481683));
#8360=CARTESIAN_POINT('Ctrl Pts',(23.,52.2916666803226,39.8371685740842));
#8361=CARTESIAN_POINT('Ctrl Pts',(12.3256628518317,52.0833333469893,46.));
#8362=CARTESIAN_POINT('Ctrl Pts',(8.45006291411674E-15,51.8750000136559,
46.));
#8363=CARTESIAN_POINT('Ctrl Pts',(-12.3256628518316,51.6666666803226,46.));
#8364=CARTESIAN_POINT('Ctrl Pts',(-23.,51.4583333469893,39.8371685740842));
#8365=CARTESIAN_POINT('Ctrl Pts',(-33.6743371481683,51.2500000136559,33.6743371481684));
#8366=CARTESIAN_POINT('Ctrl Pts',(-39.8371685740842,51.0416666803226,23.));
#8367=CARTESIAN_POINT('Ctrl Pts',(-46.,50.8333333469893,12.3256628518317));
#8368=CARTESIAN_POINT('Ctrl Pts',(-46.,50.6250000136559,0.));
#8369=CARTESIAN_POINT('Ctrl Pts',(-46.,50.4166666803226,-12.3256628518316));
#8370=CARTESIAN_POINT('Ctrl Pts',(-39.8371685740842,50.2083333469893,-23.));
#8371=CARTESIAN_POINT('Ctrl Pts',(-33.6743371481684,50.0000000136559,-33.6743371481684));
#8372=CARTESIAN_POINT('Ctrl Pts',(-23.,49.7916666803226,-39.8371685740842));
#8373=CARTESIAN_POINT('Ctrl Pts',(-12.3256628518317,49.5833333469893,-46.));
#8374=CARTESIAN_POINT('Ctrl Pts',(-2.81668763803891E-15,49.3750000136559,
-46.));
#8375=CARTESIAN_POINT('Ctrl Pts',(12.3256628518316,49.1666666803226,-46.));
#8376=CARTESIAN_POINT('Ctrl Pts',(23.,48.9583333469893,-39.8371685740842));
#8377=CARTESIAN_POINT('Ctrl Pts',(33.6743371481683,48.7500000136559,-33.6743371481684));
#8378=CARTESIAN_POINT('Ctrl Pts',(39.8371685740842,48.5416666803226,-23.));
#8379=CARTESIAN_POINT('Ctrl Pts',(46.,48.3333333469893,-12.3256628518317));
#8380=CARTESIAN_POINT('Ctrl Pts',(46.,48.1250000136559,-5.63337527607782E-15));
#8381=CARTESIAN_POINT('Ctrl Pts',(46.,47.9166666803226,12.3256628518316));
#8382=CARTESIAN_POINT('Ctrl Pts',(39.8371685740842,47.7083333469893,23.));
#8383=CARTESIAN_POINT('Ctrl Pts',(33.6743371481684,47.5000000136559,33.6743371481683));
#8384=CARTESIAN_POINT('Ctrl Pts',(23.,47.2916666803226,39.8371685740842));
#8385=CARTESIAN_POINT('Ctrl Pts',(12.3256628518317,47.0833333469893,46.));
#8386=CARTESIAN_POINT('Ctrl Pts',(8.45006291411674E-15,46.8750000136559,
46.));
#8387=CARTESIAN_POINT('Ctrl Pts',(-12.3256628518316,46.6666666803226,46.));
#8388=CARTESIAN_POINT('Ctrl Pts',(-23.,46.4583333469893,39.8371685740842));
#8389=CARTESIAN_POINT('Ctrl Pts',(-33.6743371481683,46.2500000136559,33.6743371481684));
#8390=CARTESIAN_POINT('Ctrl Pts',(-39.8371685740842,46.0416666803226,23.));
#8391=CARTESIAN_POINT('Ctrl Pts',(-46.,45.8333333469892,12.3256628518317));
#8392=CARTESIAN_POINT('Ctrl Pts',(-46.,45.6250000136559,0.));
#8393=CARTESIAN_POINT('Ctrl Pts',(-46.,45.4166666803226,-12.3256628518316));
#8394=CARTESIAN_POINT('Ctrl Pts',(-39.8371685740842,45.2083333469893,-23.));
#8395=CARTESIAN_POINT('Ctrl Pts',(-33.6743371481684,45.0000000136559,-33.6743371481684));
#8396=CARTESIAN_POINT('Ctrl Pts',(-23.,44.7916666803226,-39.8371685740842));
#8397=CARTESIAN_POINT('Ctrl Pts',(-12.3256628518317,44.5833333469893,-46.));
#8398=CARTESIAN_POINT('Ctrl Pts',(-2.81668763803891E-15,44.3750000136559,
-46.));
#8399=CARTESIAN_POINT('Ctrl Pts',(12.3256628518316,44.1666666803226,-46.));
#8400=CARTESIAN_POINT('Ctrl Pts',(23.,43.9583333469893,-39.8371685740842));
#8401=CARTESIAN_POINT('Ctrl Pts',(33.6743371481683,43.7500000136559,-33.6743371481684));
#8402=CARTESIAN_POINT('Ctrl Pts',(39.8371685740842,43.5416666803226,-23.));
#8403=CARTESIAN_POINT('Ctrl Pts',(46.,43.3333333469893,-12.3256628518317));
#8404=CARTESIAN_POINT('Ctrl Pts',(46.,43.1250000136559,-5.63337527607782E-15));
#8405=CARTESIAN_POINT('Ctrl Pts',(46.,42.9166666803226,12.3256628518316));
#8406=CARTESIAN_POINT('Ctrl Pts',(39.8371685740842,42.7083333469893,23.));
#8407=CARTESIAN_POINT('Ctrl Pts',(33.6743371481684,42.5000000136559,33.6743371481683));
#8408=CARTESIAN_POINT('Ctrl Pts',(23.,42.2916666803226,39.8371685740842));
#8409=CARTESIAN_POINT('Ctrl Pts',(12.3256628518317,42.0833333469893,46.));
#8410=CARTESIAN_POINT('Ctrl Pts',(8.45006291411674E-15,41.8750000136559,
46.));
#8411=CARTESIAN_POINT('Ctrl Pts',(-12.3256628518316,41.6666666803226,46.));
#8412=CARTESIAN_POINT('Ctrl Pts',(-23.,41.4583333469893,39.8371685740842));
#8413=CARTESIAN_POINT('Ctrl Pts',(-33.6743371481683,41.2500000136559,33.6743371481684));
#8414=CARTESIAN_POINT('Ctrl Pts',(-39.8371685740842,41.0416666803226,23.));
#8415=CARTESIAN_POINT('Ctrl Pts',(-46.,40.8333333469893,12.3256628518317));
#8416=CARTESIAN_POINT('Ctrl Pts',(-46.,40.6250000136559,0.));
#8417=CARTESIAN_POINT('Ctrl Pts',(-46.,40.4166666803226,-12.3256628518316));
#8418=CARTESIAN_POINT('Ctrl Pts',(-39.8371685740842,40.2083333469893,-23.));
#8419=CARTESIAN_POINT('Ctrl Pts',(-33.6743371481684,40.0000000136559,-33.6743371481684));
#8420=CARTESIAN_POINT('Ctrl Pts',(-23.,39.7916666803226,-39.8371685740842));
#8421=CARTESIAN_POINT('Ctrl Pts',(-12.3256628518317,39.5833333469893,-46.));
#8422=CARTESIAN_POINT('Ctrl Pts',(-2.81668763803891E-15,39.3750000136559,
-46.));
#8423=CARTESIAN_POINT('Ctrl Pts',(12.3256628518316,39.1666666803226,-46.));
#8424=CARTESIAN_POINT('Ctrl Pts',(23.,38.9583333469893,-39.8371685740842));
#8425=CARTESIAN_POINT('Ctrl Pts',(33.6743371481683,38.7500000136559,-33.6743371481684));
#8426=CARTESIAN_POINT('Ctrl Pts',(39.8371685740842,38.5416666803226,-23.));
#8427=CARTESIAN_POINT('Ctrl Pts',(46.,38.3333333469893,-12.3256628518317));
#8428=CARTESIAN_POINT('Ctrl Pts',(46.,38.1250000136559,-5.63337527607782E-15));
#8429=CARTESIAN_POINT('Ctrl Pts',(46.,37.9166666803226,12.3256628518316));
#8430=CARTESIAN_POINT('Ctrl Pts',(39.8371685740842,37.7083333469893,23.));
#8431=CARTESIAN_POINT('Ctrl Pts',(33.6743371481684,37.5000000136559,33.6743371481683));
#8432=CARTESIAN_POINT('Ctrl Pts',(23.,37.2916666803226,39.8371685740842));
#8433=CARTESIAN_POINT('Ctrl Pts',(12.3256628518317,37.0833333469893,46.));
#8434=CARTESIAN_POINT('Ctrl Pts',(8.45006291411674E-15,36.8750000136559,
46.));
#8435=CARTESIAN_POINT('Ctrl Pts',(-12.3256628518316,36.6666666803226,46.));
#8436=CARTESIAN_POINT('Ctrl Pts',(-23.,36.4583333469893,39.8371685740842));
#8437=CARTESIAN_POINT('Ctrl Pts',(-33.6743371481683,36.2500000136559,33.6743371481684));
#8438=CARTESIAN_POINT('Ctrl Pts',(-39.8371685740842,36.0416666803226,23.));
#8439=CARTESIAN_POINT('Ctrl Pts',(-46.,35.8333333469893,12.3256628518317));
#8440=CARTESIAN_POINT('Ctrl Pts',(-46.,35.6250000136559,0.));
#8441=CARTESIAN_POINT('Ctrl Pts',(-46.,35.4166666803226,-12.3256628518316));
#8442=CARTESIAN_POINT('Ctrl Pts',(-39.8371685740842,35.2083333469893,-23.));
#8443=CARTESIAN_POINT('Ctrl Pts',(-33.6743371481684,35.0000000136559,-33.6743371481684));
#8444=CARTESIAN_POINT('Ctrl Pts',(-23.,34.7916666803226,-39.8371685740842));
#8445=CARTESIAN_POINT('Ctrl Pts',(-12.3256628518317,34.5833333469893,-46.));
#8446=CARTESIAN_POINT('Ctrl Pts',(-2.81668763803891E-15,34.3750000136559,
-46.));
#8447=CARTESIAN_POINT('Ctrl Pts',(12.3256628518316,34.1666666803226,-46.));
#8448=CARTESIAN_POINT('Ctrl Pts',(23.,33.9583333469893,-39.8371685740842));
#8449=CARTESIAN_POINT('Ctrl Pts',(33.6743371481683,33.7500000136559,-33.6743371481684));
#8450=CARTESIAN_POINT('Ctrl Pts',(39.8371685740842,33.5416666803226,-23.));
#8451=CARTESIAN_POINT('Ctrl Pts',(46.,33.3333333469893,-12.3256628518317));
#8452=CARTESIAN_POINT('Ctrl Pts',(46.,33.1250000136559,-5.63337527607782E-15));
#8453=CARTESIAN_POINT('Ctrl Pts',(46.,32.9166666803226,12.3256628518316));
#8454=CARTESIAN_POINT('Ctrl Pts',(39.8371685740842,32.7083333469893,23.));
#8455=CARTESIAN_POINT('Ctrl Pts',(33.6743371481684,32.5000000136559,33.6743371481683));
#8456=CARTESIAN_POINT('Ctrl Pts',(23.,32.2916666803226,39.8371685740842));
#8457=CARTESIAN_POINT('Ctrl Pts',(12.3256628518317,32.0833333469893,46.));
#8458=CARTESIAN_POINT('Ctrl Pts',(8.45006291411674E-15,31.8750000136559,
46.));
#8459=CARTESIAN_POINT('Ctrl Pts',(-12.3256628518316,31.6666666803226,46.));
#8460=CARTESIAN_POINT('Ctrl Pts',(-23.,31.4583333469893,39.8371685740842));
#8461=CARTESIAN_POINT('Ctrl Pts',(-33.6743371481683,31.2500000136559,33.6743371481684));
#8462=CARTESIAN_POINT('Ctrl Pts',(-39.8371685740842,31.0416666803226,23.));
#8463=CARTESIAN_POINT('Ctrl Pts',(-46.,30.8333333469893,12.3256628518317));
#8464=CARTESIAN_POINT('Ctrl Pts',(-46.,30.6250000136559,0.));
#8465=CARTESIAN_POINT('Ctrl Pts',(-46.,30.4166666803226,-12.3256628518316));
#8466=CARTESIAN_POINT('Ctrl Pts',(-39.8371685740842,30.2083333469893,-23.));
#8467=CARTESIAN_POINT('Ctrl Pts',(-33.6743371481684,30.0000000136559,-33.6743371481684));
#8468=CARTESIAN_POINT('Ctrl Pts',(-23.,29.7916666803226,-39.8371685740842));
#8469=CARTESIAN_POINT('Ctrl Pts',(-12.3256628518317,29.5833333469893,-46.));
#8470=CARTESIAN_POINT('Ctrl Pts',(-2.81668763803891E-15,29.3750000136559,
-46.));
#8471=CARTESIAN_POINT('Ctrl Pts',(12.3256628518316,29.1666666803226,-46.));
#8472=CARTESIAN_POINT('Ctrl Pts',(23.,28.9583333469893,-39.8371685740842));
#8473=CARTESIAN_POINT('Ctrl Pts',(33.6743371481683,28.7500000136559,-33.6743371481684));
#8474=CARTESIAN_POINT('Ctrl Pts',(39.8371685740842,28.5416666803226,-23.));
#8475=CARTESIAN_POINT('Ctrl Pts',(46.,28.3333333469893,-12.3256628518317));
#8476=CARTESIAN_POINT('Ctrl Pts',(46.,28.1250000136559,-5.63337527607782E-15));
#8477=CARTESIAN_POINT('Ctrl Pts',(46.,27.9166666803226,12.3256628518316));
#8478=CARTESIAN_POINT('Ctrl Pts',(39.8371685740842,27.7083333469893,23.));
#8479=CARTESIAN_POINT('Ctrl Pts',(33.6743371481684,27.5000000136559,33.6743371481683));
#8480=CARTESIAN_POINT('Ctrl Pts',(23.,27.2916666803226,39.8371685740842));
#8481=CARTESIAN_POINT('Ctrl Pts',(12.3256628518317,27.0833333469893,46.));
#8482=CARTESIAN_POINT('Ctrl Pts',(8.45006291411674E-15,26.8750000136559,
46.));
#8483=CARTESIAN_POINT('Ctrl Pts',(-12.3256628518316,26.6666666803226,46.));
#8484=CARTESIAN_POINT('Ctrl Pts',(-23.,26.4583333469893,39.8371685740842));
#8485=CARTESIAN_POINT('Ctrl Pts',(-33.6743371481683,26.2500000136559,33.6743371481684));
#8486=CARTESIAN_POINT('Ctrl Pts',(-39.8371685740842,26.0416666803226,23.));
#8487=CARTESIAN_POINT('Ctrl Pts',(-46.,25.8333333469893,12.3256628518317));
#8488=CARTESIAN_POINT('Ctrl Pts',(-46.,25.6250000136559,0.));
#8489=CARTESIAN_POINT('Ctrl Pts',(-48.706329375,57.187500006828,-1.8898197019151E-14));
#8490=CARTESIAN_POINT('Ctrl Pts',(-48.706329375,56.9791666734946,-13.0508216223155));
#8491=CARTESIAN_POINT('Ctrl Pts',(-42.1809185638422,56.7708333401613,-24.3531646875));
#8492=CARTESIAN_POINT('Ctrl Pts',(-35.6555077526845,56.562500006828,-35.6555077526845));
#8493=CARTESIAN_POINT('Ctrl Pts',(-24.3531646875,56.3541666734946,-42.1809185638423));
#8494=CARTESIAN_POINT('Ctrl Pts',(-13.0508216223155,56.1458333401613,-48.706329375));
#8495=CARTESIAN_POINT('Ctrl Pts',(1.59157945007855E-14,55.937500006828,
-48.706329375));
#8496=CARTESIAN_POINT('Ctrl Pts',(13.0508216223155,55.7291666734946,-48.706329375));
#8497=CARTESIAN_POINT('Ctrl Pts',(24.3531646875,55.5208333401613,-42.1809185638422));
#8498=CARTESIAN_POINT('Ctrl Pts',(35.6555077526845,55.312500006828,-35.6555077526845));
#8499=CARTESIAN_POINT('Ctrl Pts',(42.1809185638422,55.1041666734946,-24.3531646875));
#8500=CARTESIAN_POINT('Ctrl Pts',(48.706329375,54.8958333401613,-13.0508216223155));
#8501=CARTESIAN_POINT('Ctrl Pts',(48.706329375,54.687500006828,1.293339198242E-14));
#8502=CARTESIAN_POINT('Ctrl Pts',(48.706329375,54.4791666734946,13.0508216223155));
#8503=CARTESIAN_POINT('Ctrl Pts',(42.1809185638422,54.2708333401613,24.3531646875));
#8504=CARTESIAN_POINT('Ctrl Pts',(35.6555077526845,54.062500006828,35.6555077526845));
#8505=CARTESIAN_POINT('Ctrl Pts',(24.3531646875,53.8541666734946,42.1809185638422));
#8506=CARTESIAN_POINT('Ctrl Pts',(13.0508216223155,53.6458333401613,48.706329375));
#8507=CARTESIAN_POINT('Ctrl Pts',(-9.95098946405443E-15,53.437500006828,
48.706329375));
#8508=CARTESIAN_POINT('Ctrl Pts',(-13.0508216223155,53.2291666734946,48.706329375));
#8509=CARTESIAN_POINT('Ctrl Pts',(-24.3531646875,53.0208333401613,42.1809185638423));
#8510=CARTESIAN_POINT('Ctrl Pts',(-35.6555077526845,52.812500006828,35.6555077526845));
#8511=CARTESIAN_POINT('Ctrl Pts',(-42.1809185638422,52.6041666734946,24.3531646875));
#8512=CARTESIAN_POINT('Ctrl Pts',(-48.706329375,52.3958333401613,13.0508216223155));
#8513=CARTESIAN_POINT('Ctrl Pts',(-48.706329375,52.187500006828,-1.8898197019151E-14));
#8514=CARTESIAN_POINT('Ctrl Pts',(-48.706329375,51.9791666734946,-13.0508216223155));
#8515=CARTESIAN_POINT('Ctrl Pts',(-42.1809185638422,51.7708333401613,-24.3531646875));
#8516=CARTESIAN_POINT('Ctrl Pts',(-35.6555077526845,51.562500006828,-35.6555077526845));
#8517=CARTESIAN_POINT('Ctrl Pts',(-24.3531646875,51.3541666734946,-42.1809185638423));
#8518=CARTESIAN_POINT('Ctrl Pts',(-13.0508216223155,51.1458333401613,-48.706329375));
#8519=CARTESIAN_POINT('Ctrl Pts',(1.59157945007855E-14,50.937500006828,
-48.706329375));
#8520=CARTESIAN_POINT('Ctrl Pts',(13.0508216223155,50.7291666734946,-48.706329375));
#8521=CARTESIAN_POINT('Ctrl Pts',(24.3531646875,50.5208333401613,-42.1809185638422));
#8522=CARTESIAN_POINT('Ctrl Pts',(35.6555077526845,50.312500006828,-35.6555077526845));
#8523=CARTESIAN_POINT('Ctrl Pts',(42.1809185638422,50.1041666734946,-24.3531646875));
#8524=CARTESIAN_POINT('Ctrl Pts',(48.706329375,49.8958333401613,-13.0508216223155));
#8525=CARTESIAN_POINT('Ctrl Pts',(48.706329375,49.687500006828,1.293339198242E-14));
#8526=CARTESIAN_POINT('Ctrl Pts',(48.706329375,49.4791666734946,13.0508216223155));
#8527=CARTESIAN_POINT('Ctrl Pts',(42.1809185638422,49.2708333401613,24.3531646875));
#8528=CARTESIAN_POINT('Ctrl Pts',(35.6555077526845,49.062500006828,35.6555077526845));
#8529=CARTESIAN_POINT('Ctrl Pts',(24.3531646875,48.8541666734946,42.1809185638422));
#8530=CARTESIAN_POINT('Ctrl Pts',(13.0508216223155,48.6458333401613,48.706329375));
#8531=CARTESIAN_POINT('Ctrl Pts',(-9.95098946405443E-15,48.437500006828,
48.706329375));
#8532=CARTESIAN_POINT('Ctrl Pts',(-13.0508216223155,48.2291666734946,48.706329375));
#8533=CARTESIAN_POINT('Ctrl Pts',(-24.3531646875,48.0208333401613,42.1809185638423));
#8534=CARTESIAN_POINT('Ctrl Pts',(-35.6555077526845,47.812500006828,35.6555077526845));
#8535=CARTESIAN_POINT('Ctrl Pts',(-42.1809185638422,47.6041666734946,24.3531646875));
#8536=CARTESIAN_POINT('Ctrl Pts',(-48.706329375,47.3958333401613,13.0508216223155));
#8537=CARTESIAN_POINT('Ctrl Pts',(-48.706329375,47.187500006828,-1.8898197019151E-14));
#8538=CARTESIAN_POINT('Ctrl Pts',(-48.706329375,46.9791666734946,-13.0508216223155));
#8539=CARTESIAN_POINT('Ctrl Pts',(-42.1809185638422,46.7708333401613,-24.3531646875));
#8540=CARTESIAN_POINT('Ctrl Pts',(-35.6555077526845,46.562500006828,-35.6555077526845));
#8541=CARTESIAN_POINT('Ctrl Pts',(-24.3531646875,46.3541666734946,-42.1809185638423));
#8542=CARTESIAN_POINT('Ctrl Pts',(-13.0508216223155,46.1458333401613,-48.706329375));
#8543=CARTESIAN_POINT('Ctrl Pts',(1.59157945007855E-14,45.937500006828,
-48.706329375));
#8544=CARTESIAN_POINT('Ctrl Pts',(13.0508216223155,45.7291666734946,-48.706329375));
#8545=CARTESIAN_POINT('Ctrl Pts',(24.3531646875,45.5208333401613,-42.1809185638422));
#8546=CARTESIAN_POINT('Ctrl Pts',(35.6555077526845,45.312500006828,-35.6555077526845));
#8547=CARTESIAN_POINT('Ctrl Pts',(42.1809185638422,45.1041666734946,-24.3531646875));
#8548=CARTESIAN_POINT('Ctrl Pts',(48.706329375,44.8958333401613,-13.0508216223155));
#8549=CARTESIAN_POINT('Ctrl Pts',(48.706329375,44.687500006828,1.293339198242E-14));
#8550=CARTESIAN_POINT('Ctrl Pts',(48.706329375,44.4791666734946,13.0508216223155));
#8551=CARTESIAN_POINT('Ctrl Pts',(42.1809185638422,44.2708333401613,24.3531646875));
#8552=CARTESIAN_POINT('Ctrl Pts',(35.6555077526845,44.062500006828,35.6555077526845));
#8553=CARTESIAN_POINT('Ctrl Pts',(24.3531646875,43.8541666734946,42.1809185638422));
#8554=CARTESIAN_POINT('Ctrl Pts',(13.0508216223155,43.6458333401613,48.706329375));
#8555=CARTESIAN_POINT('Ctrl Pts',(-9.95098946405443E-15,43.437500006828,
48.706329375));
#8556=CARTESIAN_POINT('Ctrl Pts',(-13.0508216223155,43.2291666734946,48.706329375));
#8557=CARTESIAN_POINT('Ctrl Pts',(-24.3531646875,43.0208333401613,42.1809185638423));
#8558=CARTESIAN_POINT('Ctrl Pts',(-35.6555077526845,42.812500006828,35.6555077526845));
#8559=CARTESIAN_POINT('Ctrl Pts',(-42.1809185638422,42.6041666734946,24.3531646875));
#8560=CARTESIAN_POINT('Ctrl Pts',(-48.706329375,42.3958333401613,13.0508216223155));
#8561=CARTESIAN_POINT('Ctrl Pts',(-48.706329375,42.187500006828,-1.8898197019151E-14));
#8562=CARTESIAN_POINT('Ctrl Pts',(-48.706329375,41.9791666734946,-13.0508216223155));
#8563=CARTESIAN_POINT('Ctrl Pts',(-42.1809185638422,41.7708333401613,-24.3531646875));
#8564=CARTESIAN_POINT('Ctrl Pts',(-35.6555077526845,41.562500006828,-35.6555077526845));
#8565=CARTESIAN_POINT('Ctrl Pts',(-24.3531646875,41.3541666734946,-42.1809185638423));
#8566=CARTESIAN_POINT('Ctrl Pts',(-13.0508216223155,41.1458333401613,-48.706329375));
#8567=CARTESIAN_POINT('Ctrl Pts',(1.59157945007855E-14,40.937500006828,
-48.706329375));
#8568=CARTESIAN_POINT('Ctrl Pts',(13.0508216223155,40.7291666734946,-48.706329375));
#8569=CARTESIAN_POINT('Ctrl Pts',(24.3531646875,40.5208333401613,-42.1809185638422));
#8570=CARTESIAN_POINT('Ctrl Pts',(35.6555077526845,40.312500006828,-35.6555077526845));
#8571=CARTESIAN_POINT('Ctrl Pts',(42.1809185638422,40.1041666734946,-24.3531646875));
#8572=CARTESIAN_POINT('Ctrl Pts',(48.706329375,39.8958333401613,-13.0508216223155));
#8573=CARTESIAN_POINT('Ctrl Pts',(48.706329375,39.687500006828,1.293339198242E-14));
#8574=CARTESIAN_POINT('Ctrl Pts',(48.706329375,39.4791666734946,13.0508216223155));
#8575=CARTESIAN_POINT('Ctrl Pts',(42.1809185638422,39.2708333401613,24.3531646875));
#8576=CARTESIAN_POINT('Ctrl Pts',(35.6555077526845,39.062500006828,35.6555077526845));
#8577=CARTESIAN_POINT('Ctrl Pts',(24.3531646875,38.8541666734946,42.1809185638422));
#8578=CARTESIAN_POINT('Ctrl Pts',(13.0508216223155,38.6458333401613,48.706329375));
#8579=CARTESIAN_POINT('Ctrl Pts',(-9.95098946405443E-15,38.437500006828,
48.706329375));
#8580=CARTESIAN_POINT('Ctrl Pts',(-13.0508216223155,38.2291666734946,48.706329375));
#8581=CARTESIAN_POINT('Ctrl Pts',(-24.3531646875,38.0208333401613,42.1809185638423));
#8582=CARTESIAN_POINT('Ctrl Pts',(-35.6555077526845,37.812500006828,35.6555077526845));
#8583=CARTESIAN_POINT('Ctrl Pts',(-42.1809185638422,37.6041666734946,24.3531646875));
#8584=CARTESIAN_POINT('Ctrl Pts',(-48.706329375,37.3958333401613,13.0508216223155));
#8585=CARTESIAN_POINT('Ctrl Pts',(-48.706329375,37.187500006828,-1.8898197019151E-14));
#8586=CARTESIAN_POINT('Ctrl Pts',(-48.706329375,36.9791666734946,-13.0508216223155));
#8587=CARTESIAN_POINT('Ctrl Pts',(-42.1809185638422,36.7708333401613,-24.3531646875));
#8588=CARTESIAN_POINT('Ctrl Pts',(-35.6555077526845,36.562500006828,-35.6555077526845));
#8589=CARTESIAN_POINT('Ctrl Pts',(-24.3531646875,36.3541666734946,-42.1809185638423));
#8590=CARTESIAN_POINT('Ctrl Pts',(-13.0508216223155,36.1458333401613,-48.706329375));
#8591=CARTESIAN_POINT('Ctrl Pts',(1.59157945007855E-14,35.937500006828,
-48.706329375));
#8592=CARTESIAN_POINT('Ctrl Pts',(13.0508216223155,35.7291666734946,-48.706329375));
#8593=CARTESIAN_POINT('Ctrl Pts',(24.3531646875,35.5208333401613,-42.1809185638422));
#8594=CARTESIAN_POINT('Ctrl Pts',(35.6555077526845,35.312500006828,-35.6555077526845));
#8595=CARTESIAN_POINT('Ctrl Pts',(42.1809185638422,35.1041666734946,-24.3531646875));
#8596=CARTESIAN_POINT('Ctrl Pts',(48.706329375,34.8958333401613,-13.0508216223155));
#8597=CARTESIAN_POINT('Ctrl Pts',(48.706329375,34.687500006828,1.293339198242E-14));
#8598=CARTESIAN_POINT('Ctrl Pts',(48.706329375,34.4791666734946,13.0508216223155));
#8599=CARTESIAN_POINT('Ctrl Pts',(42.1809185638422,34.2708333401613,24.3531646875));
#8600=CARTESIAN_POINT('Ctrl Pts',(35.6555077526845,34.062500006828,35.6555077526845));
#8601=CARTESIAN_POINT('Ctrl Pts',(24.3531646875,33.8541666734946,42.1809185638422));
#8602=CARTESIAN_POINT('Ctrl Pts',(13.0508216223155,33.6458333401613,48.706329375));
#8603=CARTESIAN_POINT('Ctrl Pts',(-9.95098946405443E-15,33.437500006828,
48.706329375));
#8604=CARTESIAN_POINT('Ctrl Pts',(-13.0508216223155,33.2291666734946,48.706329375));
#8605=CARTESIAN_POINT('Ctrl Pts',(-24.3531646875,33.0208333401613,42.1809185638423));
#8606=CARTESIAN_POINT('Ctrl Pts',(-35.6555077526845,32.812500006828,35.6555077526845));
#8607=CARTESIAN_POINT('Ctrl Pts',(-42.1809185638422,32.6041666734946,24.3531646875));
#8608=CARTESIAN_POINT('Ctrl Pts',(-48.706329375,32.3958333401613,13.0508216223155));
#8609=CARTESIAN_POINT('Ctrl Pts',(-48.706329375,32.187500006828,-1.8898197019151E-14));
#8610=CARTESIAN_POINT('Ctrl Pts',(-48.706329375,31.9791666734946,-13.0508216223155));
#8611=CARTESIAN_POINT('Ctrl Pts',(-42.1809185638422,31.7708333401613,-24.3531646875));
#8612=CARTESIAN_POINT('Ctrl Pts',(-35.6555077526845,31.562500006828,-35.6555077526845));
#8613=CARTESIAN_POINT('Ctrl Pts',(-24.3531646875,31.3541666734946,-42.1809185638423));
#8614=CARTESIAN_POINT('Ctrl Pts',(-13.0508216223155,31.1458333401613,-48.706329375));
#8615=CARTESIAN_POINT('Ctrl Pts',(1.59157945007855E-14,30.937500006828,
-48.706329375));
#8616=CARTESIAN_POINT('Ctrl Pts',(13.0508216223155,30.7291666734946,-48.706329375));
#8617=CARTESIAN_POINT('Ctrl Pts',(24.3531646875,30.5208333401613,-42.1809185638422));
#8618=CARTESIAN_POINT('Ctrl Pts',(35.6555077526845,30.312500006828,-35.6555077526845));
#8619=CARTESIAN_POINT('Ctrl Pts',(42.1809185638422,30.1041666734946,-24.3531646875));
#8620=CARTESIAN_POINT('Ctrl Pts',(48.706329375,29.8958333401613,-13.0508216223155));
#8621=CARTESIAN_POINT('Ctrl Pts',(48.706329375,29.687500006828,1.293339198242E-14));
#8622=CARTESIAN_POINT('Ctrl Pts',(48.706329375,29.4791666734946,13.0508216223155));
#8623=CARTESIAN_POINT('Ctrl Pts',(42.1809185638422,29.2708333401613,24.3531646875));
#8624=CARTESIAN_POINT('Ctrl Pts',(35.6555077526845,29.062500006828,35.6555077526845));
#8625=CARTESIAN_POINT('Ctrl Pts',(24.3531646875,28.8541666734946,42.1809185638422));
#8626=CARTESIAN_POINT('Ctrl Pts',(13.0508216223155,28.6458333401613,48.706329375));
#8627=CARTESIAN_POINT('Ctrl Pts',(-9.95098946405443E-15,28.437500006828,
48.706329375));
#8628=CARTESIAN_POINT('Ctrl Pts',(-13.0508216223155,28.2291666734946,48.706329375));
#8629=CARTESIAN_POINT('Ctrl Pts',(-24.3531646875,28.0208333401613,42.1809185638423));
#8630=CARTESIAN_POINT('Ctrl Pts',(-35.6555077526845,27.812500006828,35.6555077526845));
#8631=CARTESIAN_POINT('Ctrl Pts',(-42.1809185638422,27.6041666734946,24.3531646875));
#8632=CARTESIAN_POINT('Ctrl Pts',(-48.706329375,27.3958333401613,13.0508216223155));
#8633=CARTESIAN_POINT('Ctrl Pts',(-48.706329375,27.187500006828,-1.8898197019151E-14));
#8634=CARTESIAN_POINT('',(-48.5134353784345,52.1175463684955,-4.33048599679673));
#8635=CARTESIAN_POINT('Ctrl Pts',(-45.7957082162897,50.5508791552084,-4.33048599679673));
#8636=CARTESIAN_POINT('Ctrl Pts',(-46.027322302781,50.6843839384496,-4.33048599679671));
#8637=CARTESIAN_POINT('Ctrl Pts',(-46.4905476657728,50.9513983799648,-4.33048599679678));
#8638=CARTESIAN_POINT('Ctrl Pts',(-46.9537676533565,51.2184221466352,-4.33048599679674));
#8639=CARTESIAN_POINT('Ctrl Pts',(-47.6280672732222,51.6071316973962,-4.33048599679674));
#8640=CARTESIAN_POINT('Ctrl Pts',(-48.0707534890442,51.8623352807796,-4.33048599679674));
#8641=CARTESIAN_POINT('Ctrl Pts',(-48.5134353784345,52.1175463684955,-4.33048599679673));
#8642=CARTESIAN_POINT('',(-4.32456003949876,51.0073567866782,-48.5139639861634));
#8643=CARTESIAN_POINT('Ctrl Pts',(-48.5134353784345,52.1175463684955,-4.33048599679674));
#8644=CARTESIAN_POINT('Ctrl Pts',(-47.5573898704235,51.9424850907232,-15.0408432190651));
#8645=CARTESIAN_POINT('Ctrl Pts',(-42.1809185638422,51.7708333401613,-24.3531646875));
#8646=CARTESIAN_POINT('Ctrl Pts',(-35.6555077526845,51.562500006828,-35.6555077526845));
#8647=CARTESIAN_POINT('Ctrl Pts',(-24.3531646875,51.3541666734946,-42.1809185638423));
#8648=CARTESIAN_POINT('Ctrl Pts',(-15.038141415499,51.1824651212465,-47.5589497574396));
#8649=CARTESIAN_POINT('Ctrl Pts',(-4.32456003949876,51.0073567866782,-48.5139639861634));
#8650=CARTESIAN_POINT('Origin',(-4.32455765124451,8022.20454033029,4524.01087378963));
#8651=CARTESIAN_POINT('Ctrl Pts',(-46.,55.6250000136559,0.));
#8652=CARTESIAN_POINT('Ctrl Pts',(-46.,55.4166666803226,-12.3256628518316));
#8653=CARTESIAN_POINT('Ctrl Pts',(-39.8371685740842,55.2083333469893,-23.));
#8654=CARTESIAN_POINT('Ctrl Pts',(-33.6743371481684,55.0000000136559,-33.6743371481684));
#8655=CARTESIAN_POINT('Ctrl Pts',(-23.,54.7916666803226,-39.8371685740842));
#8656=CARTESIAN_POINT('Ctrl Pts',(-12.3256628518317,54.5833333469893,-46.));
#8657=CARTESIAN_POINT('Ctrl Pts',(-2.81668763803891E-15,54.3750000136559,
-46.));
#8658=CARTESIAN_POINT('Ctrl Pts',(12.3256628518316,54.1666666803226,-46.));
#8659=CARTESIAN_POINT('Ctrl Pts',(23.,53.9583333469893,-39.8371685740842));
#8660=CARTESIAN_POINT('Ctrl Pts',(33.6743371481683,53.7500000136559,-33.6743371481684));
#8661=CARTESIAN_POINT('Ctrl Pts',(39.8371685740842,53.5416666803226,-23.));
#8662=CARTESIAN_POINT('Ctrl Pts',(46.,53.3333333469893,-12.3256628518317));
#8663=CARTESIAN_POINT('Ctrl Pts',(46.,53.1250000136559,-5.63337527607782E-15));
#8664=CARTESIAN_POINT('Ctrl Pts',(46.,52.9166666803226,12.3256628518316));
#8665=CARTESIAN_POINT('Ctrl Pts',(39.8371685740842,52.7083333469893,23.));
#8666=CARTESIAN_POINT('Ctrl Pts',(33.6743371481684,52.5000000136559,33.6743371481683));
#8667=CARTESIAN_POINT('Ctrl Pts',(23.,52.2916666803226,39.8371685740842));
#8668=CARTESIAN_POINT('Ctrl Pts',(12.3256628518317,52.0833333469893,46.));
#8669=CARTESIAN_POINT('Ctrl Pts',(8.45006291411674E-15,51.8750000136559,
46.));
#8670=CARTESIAN_POINT('Ctrl Pts',(-12.3256628518316,51.6666666803226,46.));
#8671=CARTESIAN_POINT('Ctrl Pts',(-23.,51.4583333469893,39.8371685740842));
#8672=CARTESIAN_POINT('Ctrl Pts',(-33.6743371481683,51.2500000136559,33.6743371481684));
#8673=CARTESIAN_POINT('Ctrl Pts',(-39.8371685740842,51.0416666803226,23.));
#8674=CARTESIAN_POINT('Ctrl Pts',(-46.,50.8333333469893,12.3256628518317));
#8675=CARTESIAN_POINT('Ctrl Pts',(-46.,50.6250000136559,0.));
#8676=CARTESIAN_POINT('Ctrl Pts',(-46.,50.4166666803226,-12.3256628518316));
#8677=CARTESIAN_POINT('Ctrl Pts',(-39.8371685740842,50.2083333469893,-23.));
#8678=CARTESIAN_POINT('Ctrl Pts',(-33.6743371481684,50.0000000136559,-33.6743371481684));
#8679=CARTESIAN_POINT('Ctrl Pts',(-23.,49.7916666803226,-39.8371685740842));
#8680=CARTESIAN_POINT('Ctrl Pts',(-12.3256628518317,49.5833333469893,-46.));
#8681=CARTESIAN_POINT('Ctrl Pts',(-2.81668763803891E-15,49.3750000136559,
-46.));
#8682=CARTESIAN_POINT('Ctrl Pts',(12.3256628518316,49.1666666803226,-46.));
#8683=CARTESIAN_POINT('Ctrl Pts',(23.,48.9583333469893,-39.8371685740842));
#8684=CARTESIAN_POINT('Ctrl Pts',(33.6743371481683,48.7500000136559,-33.6743371481684));
#8685=CARTESIAN_POINT('Ctrl Pts',(39.8371685740842,48.5416666803226,-23.));
#8686=CARTESIAN_POINT('Ctrl Pts',(46.,48.3333333469893,-12.3256628518317));
#8687=CARTESIAN_POINT('Ctrl Pts',(46.,48.1250000136559,-5.63337527607782E-15));
#8688=CARTESIAN_POINT('Ctrl Pts',(46.,47.9166666803226,12.3256628518316));
#8689=CARTESIAN_POINT('Ctrl Pts',(39.8371685740842,47.7083333469893,23.));
#8690=CARTESIAN_POINT('Ctrl Pts',(33.6743371481684,47.5000000136559,33.6743371481683));
#8691=CARTESIAN_POINT('Ctrl Pts',(23.,47.2916666803226,39.8371685740842));
#8692=CARTESIAN_POINT('Ctrl Pts',(12.3256628518317,47.0833333469893,46.));
#8693=CARTESIAN_POINT('Ctrl Pts',(8.45006291411674E-15,46.8750000136559,
46.));
#8694=CARTESIAN_POINT('Ctrl Pts',(-12.3256628518316,46.6666666803226,46.));
#8695=CARTESIAN_POINT('Ctrl Pts',(-23.,46.4583333469893,39.8371685740842));
#8696=CARTESIAN_POINT('Ctrl Pts',(-33.6743371481683,46.2500000136559,33.6743371481684));
#8697=CARTESIAN_POINT('Ctrl Pts',(-39.8371685740842,46.0416666803226,23.));
#8698=CARTESIAN_POINT('Ctrl Pts',(-46.,45.8333333469892,12.3256628518317));
#8699=CARTESIAN_POINT('Ctrl Pts',(-46.,45.6250000136559,0.));
#8700=CARTESIAN_POINT('Ctrl Pts',(-46.,45.4166666803226,-12.3256628518316));
#8701=CARTESIAN_POINT('Ctrl Pts',(-39.8371685740842,45.2083333469893,-23.));
#8702=CARTESIAN_POINT('Ctrl Pts',(-33.6743371481684,45.0000000136559,-33.6743371481684));
#8703=CARTESIAN_POINT('Ctrl Pts',(-23.,44.7916666803226,-39.8371685740842));
#8704=CARTESIAN_POINT('Ctrl Pts',(-12.3256628518317,44.5833333469893,-46.));
#8705=CARTESIAN_POINT('Ctrl Pts',(-2.81668763803891E-15,44.3750000136559,
-46.));
#8706=CARTESIAN_POINT('Ctrl Pts',(12.3256628518316,44.1666666803226,-46.));
#8707=CARTESIAN_POINT('Ctrl Pts',(23.,43.9583333469893,-39.8371685740842));
#8708=CARTESIAN_POINT('Ctrl Pts',(33.6743371481683,43.7500000136559,-33.6743371481684));
#8709=CARTESIAN_POINT('Ctrl Pts',(39.8371685740842,43.5416666803226,-23.));
#8710=CARTESIAN_POINT('Ctrl Pts',(46.,43.3333333469893,-12.3256628518317));
#8711=CARTESIAN_POINT('Ctrl Pts',(46.,43.1250000136559,-5.63337527607782E-15));
#8712=CARTESIAN_POINT('Ctrl Pts',(46.,42.9166666803226,12.3256628518316));
#8713=CARTESIAN_POINT('Ctrl Pts',(39.8371685740842,42.7083333469893,23.));
#8714=CARTESIAN_POINT('Ctrl Pts',(33.6743371481684,42.5000000136559,33.6743371481683));
#8715=CARTESIAN_POINT('Ctrl Pts',(23.,42.2916666803226,39.8371685740842));
#8716=CARTESIAN_POINT('Ctrl Pts',(12.3256628518317,42.0833333469893,46.));
#8717=CARTESIAN_POINT('Ctrl Pts',(8.45006291411674E-15,41.8750000136559,
46.));
#8718=CARTESIAN_POINT('Ctrl Pts',(-12.3256628518316,41.6666666803226,46.));
#8719=CARTESIAN_POINT('Ctrl Pts',(-23.,41.4583333469893,39.8371685740842));
#8720=CARTESIAN_POINT('Ctrl Pts',(-33.6743371481683,41.2500000136559,33.6743371481684));
#8721=CARTESIAN_POINT('Ctrl Pts',(-39.8371685740842,41.0416666803226,23.));
#8722=CARTESIAN_POINT('Ctrl Pts',(-46.,40.8333333469893,12.3256628518317));
#8723=CARTESIAN_POINT('Ctrl Pts',(-46.,40.6250000136559,0.));
#8724=CARTESIAN_POINT('Ctrl Pts',(-46.,40.4166666803226,-12.3256628518316));
#8725=CARTESIAN_POINT('Ctrl Pts',(-39.8371685740842,40.2083333469893,-23.));
#8726=CARTESIAN_POINT('Ctrl Pts',(-33.6743371481684,40.0000000136559,-33.6743371481684));
#8727=CARTESIAN_POINT('Ctrl Pts',(-23.,39.7916666803226,-39.8371685740842));
#8728=CARTESIAN_POINT('Ctrl Pts',(-12.3256628518317,39.5833333469893,-46.));
#8729=CARTESIAN_POINT('Ctrl Pts',(-2.81668763803891E-15,39.3750000136559,
-46.));
#8730=CARTESIAN_POINT('Ctrl Pts',(12.3256628518316,39.1666666803226,-46.));
#8731=CARTESIAN_POINT('Ctrl Pts',(23.,38.9583333469893,-39.8371685740842));
#8732=CARTESIAN_POINT('Ctrl Pts',(33.6743371481683,38.7500000136559,-33.6743371481684));
#8733=CARTESIAN_POINT('Ctrl Pts',(39.8371685740842,38.5416666803226,-23.));
#8734=CARTESIAN_POINT('Ctrl Pts',(46.,38.3333333469893,-12.3256628518317));
#8735=CARTESIAN_POINT('Ctrl Pts',(46.,38.1250000136559,-5.63337527607782E-15));
#8736=CARTESIAN_POINT('Ctrl Pts',(46.,37.9166666803226,12.3256628518316));
#8737=CARTESIAN_POINT('Ctrl Pts',(39.8371685740842,37.7083333469893,23.));
#8738=CARTESIAN_POINT('Ctrl Pts',(33.6743371481684,37.5000000136559,33.6743371481683));
#8739=CARTESIAN_POINT('Ctrl Pts',(23.,37.2916666803226,39.8371685740842));
#8740=CARTESIAN_POINT('Ctrl Pts',(12.3256628518317,37.0833333469893,46.));
#8741=CARTESIAN_POINT('Ctrl Pts',(8.45006291411674E-15,36.8750000136559,
46.));
#8742=CARTESIAN_POINT('Ctrl Pts',(-12.3256628518316,36.6666666803226,46.));
#8743=CARTESIAN_POINT('Ctrl Pts',(-23.,36.4583333469893,39.8371685740842));
#8744=CARTESIAN_POINT('Ctrl Pts',(-33.6743371481683,36.2500000136559,33.6743371481684));
#8745=CARTESIAN_POINT('Ctrl Pts',(-39.8371685740842,36.0416666803226,23.));
#8746=CARTESIAN_POINT('Ctrl Pts',(-46.,35.8333333469893,12.3256628518317));
#8747=CARTESIAN_POINT('Ctrl Pts',(-46.,35.6250000136559,0.));
#8748=CARTESIAN_POINT('Ctrl Pts',(-46.,35.4166666803226,-12.3256628518316));
#8749=CARTESIAN_POINT('Ctrl Pts',(-39.8371685740842,35.2083333469893,-23.));
#8750=CARTESIAN_POINT('Ctrl Pts',(-33.6743371481684,35.0000000136559,-33.6743371481684));
#8751=CARTESIAN_POINT('Ctrl Pts',(-23.,34.7916666803226,-39.8371685740842));
#8752=CARTESIAN_POINT('Ctrl Pts',(-12.3256628518317,34.5833333469893,-46.));
#8753=CARTESIAN_POINT('Ctrl Pts',(-2.81668763803891E-15,34.3750000136559,
-46.));
#8754=CARTESIAN_POINT('Ctrl Pts',(12.3256628518316,34.1666666803226,-46.));
#8755=CARTESIAN_POINT('Ctrl Pts',(23.,33.9583333469893,-39.8371685740842));
#8756=CARTESIAN_POINT('Ctrl Pts',(33.6743371481683,33.7500000136559,-33.6743371481684));
#8757=CARTESIAN_POINT('Ctrl Pts',(39.8371685740842,33.5416666803226,-23.));
#8758=CARTESIAN_POINT('Ctrl Pts',(46.,33.3333333469893,-12.3256628518317));
#8759=CARTESIAN_POINT('Ctrl Pts',(46.,33.1250000136559,-5.63337527607782E-15));
#8760=CARTESIAN_POINT('Ctrl Pts',(46.,32.9166666803226,12.3256628518316));
#8761=CARTESIAN_POINT('Ctrl Pts',(39.8371685740842,32.7083333469893,23.));
#8762=CARTESIAN_POINT('Ctrl Pts',(33.6743371481684,32.5000000136559,33.6743371481683));
#8763=CARTESIAN_POINT('Ctrl Pts',(23.,32.2916666803226,39.8371685740842));
#8764=CARTESIAN_POINT('Ctrl Pts',(12.3256628518317,32.0833333469893,46.));
#8765=CARTESIAN_POINT('Ctrl Pts',(8.45006291411674E-15,31.8750000136559,
46.));
#8766=CARTESIAN_POINT('Ctrl Pts',(-12.3256628518316,31.6666666803226,46.));
#8767=CARTESIAN_POINT('Ctrl Pts',(-23.,31.4583333469893,39.8371685740842));
#8768=CARTESIAN_POINT('Ctrl Pts',(-33.6743371481683,31.2500000136559,33.6743371481684));
#8769=CARTESIAN_POINT('Ctrl Pts',(-39.8371685740842,31.0416666803226,23.));
#8770=CARTESIAN_POINT('Ctrl Pts',(-46.,30.8333333469893,12.3256628518317));
#8771=CARTESIAN_POINT('Ctrl Pts',(-46.,30.6250000136559,0.));
#8772=CARTESIAN_POINT('Ctrl Pts',(-46.,30.4166666803226,-12.3256628518316));
#8773=CARTESIAN_POINT('Ctrl Pts',(-39.8371685740842,30.2083333469893,-23.));
#8774=CARTESIAN_POINT('Ctrl Pts',(-33.6743371481684,30.0000000136559,-33.6743371481684));
#8775=CARTESIAN_POINT('Ctrl Pts',(-23.,29.7916666803226,-39.8371685740842));
#8776=CARTESIAN_POINT('Ctrl Pts',(-12.3256628518317,29.5833333469893,-46.));
#8777=CARTESIAN_POINT('Ctrl Pts',(-2.81668763803891E-15,29.3750000136559,
-46.));
#8778=CARTESIAN_POINT('Ctrl Pts',(12.3256628518316,29.1666666803226,-46.));
#8779=CARTESIAN_POINT('Ctrl Pts',(23.,28.9583333469893,-39.8371685740842));
#8780=CARTESIAN_POINT('Ctrl Pts',(33.6743371481683,28.7500000136559,-33.6743371481684));
#8781=CARTESIAN_POINT('Ctrl Pts',(39.8371685740842,28.5416666803226,-23.));
#8782=CARTESIAN_POINT('Ctrl Pts',(46.,28.3333333469893,-12.3256628518317));
#8783=CARTESIAN_POINT('Ctrl Pts',(46.,28.1250000136559,-5.63337527607782E-15));
#8784=CARTESIAN_POINT('Ctrl Pts',(46.,27.9166666803226,12.3256628518316));
#8785=CARTESIAN_POINT('Ctrl Pts',(39.8371685740842,27.7083333469893,23.));
#8786=CARTESIAN_POINT('Ctrl Pts',(33.6743371481684,27.5000000136559,33.6743371481683));
#8787=CARTESIAN_POINT('Ctrl Pts',(23.,27.2916666803226,39.8371685740842));
#8788=CARTESIAN_POINT('Ctrl Pts',(12.3256628518317,27.0833333469893,46.));
#8789=CARTESIAN_POINT('Ctrl Pts',(8.45006291411674E-15,26.8750000136559,
46.));
#8790=CARTESIAN_POINT('Ctrl Pts',(-12.3256628518316,26.6666666803226,46.));
#8791=CARTESIAN_POINT('Ctrl Pts',(-23.,26.4583333469893,39.8371685740842));
#8792=CARTESIAN_POINT('Ctrl Pts',(-33.6743371481683,26.2500000136559,33.6743371481684));
#8793=CARTESIAN_POINT('Ctrl Pts',(-39.8371685740842,26.0416666803226,23.));
#8794=CARTESIAN_POINT('Ctrl Pts',(-46.,25.8333333469893,12.3256628518317));
#8795=CARTESIAN_POINT('Ctrl Pts',(-46.,25.6250000136559,0.));
#8796=CARTESIAN_POINT('Ctrl Pts',(-48.706329375,57.187500006828,-1.8898197019151E-14));
#8797=CARTESIAN_POINT('Ctrl Pts',(-48.706329375,56.9791666734946,-13.0508216223155));
#8798=CARTESIAN_POINT('Ctrl Pts',(-42.1809185638422,56.7708333401613,-24.3531646875));
#8799=CARTESIAN_POINT('Ctrl Pts',(-35.6555077526845,56.562500006828,-35.6555077526845));
#8800=CARTESIAN_POINT('Ctrl Pts',(-24.3531646875,56.3541666734946,-42.1809185638423));
#8801=CARTESIAN_POINT('Ctrl Pts',(-13.0508216223155,56.1458333401613,-48.706329375));
#8802=CARTESIAN_POINT('Ctrl Pts',(1.59157945007855E-14,55.937500006828,
-48.706329375));
#8803=CARTESIAN_POINT('Ctrl Pts',(13.0508216223155,55.7291666734946,-48.706329375));
#8804=CARTESIAN_POINT('Ctrl Pts',(24.3531646875,55.5208333401613,-42.1809185638422));
#8805=CARTESIAN_POINT('Ctrl Pts',(35.6555077526845,55.312500006828,-35.6555077526845));
#8806=CARTESIAN_POINT('Ctrl Pts',(42.1809185638422,55.1041666734946,-24.3531646875));
#8807=CARTESIAN_POINT('Ctrl Pts',(48.706329375,54.8958333401613,-13.0508216223155));
#8808=CARTESIAN_POINT('Ctrl Pts',(48.706329375,54.687500006828,1.293339198242E-14));
#8809=CARTESIAN_POINT('Ctrl Pts',(48.706329375,54.4791666734946,13.0508216223155));
#8810=CARTESIAN_POINT('Ctrl Pts',(42.1809185638422,54.2708333401613,24.3531646875));
#8811=CARTESIAN_POINT('Ctrl Pts',(35.6555077526845,54.062500006828,35.6555077526845));
#8812=CARTESIAN_POINT('Ctrl Pts',(24.3531646875,53.8541666734946,42.1809185638422));
#8813=CARTESIAN_POINT('Ctrl Pts',(13.0508216223155,53.6458333401613,48.706329375));
#8814=CARTESIAN_POINT('Ctrl Pts',(-9.95098946405443E-15,53.437500006828,
48.706329375));
#8815=CARTESIAN_POINT('Ctrl Pts',(-13.0508216223155,53.2291666734946,48.706329375));
#8816=CARTESIAN_POINT('Ctrl Pts',(-24.3531646875,53.0208333401613,42.1809185638423));
#8817=CARTESIAN_POINT('Ctrl Pts',(-35.6555077526845,52.812500006828,35.6555077526845));
#8818=CARTESIAN_POINT('Ctrl Pts',(-42.1809185638422,52.6041666734946,24.3531646875));
#8819=CARTESIAN_POINT('Ctrl Pts',(-48.706329375,52.3958333401613,13.0508216223155));
#8820=CARTESIAN_POINT('Ctrl Pts',(-48.706329375,52.187500006828,-1.8898197019151E-14));
#8821=CARTESIAN_POINT('Ctrl Pts',(-48.706329375,51.9791666734946,-13.0508216223155));
#8822=CARTESIAN_POINT('Ctrl Pts',(-42.1809185638422,51.7708333401613,-24.3531646875));
#8823=CARTESIAN_POINT('Ctrl Pts',(-35.6555077526845,51.562500006828,-35.6555077526845));
#8824=CARTESIAN_POINT('Ctrl Pts',(-24.3531646875,51.3541666734946,-42.1809185638423));
#8825=CARTESIAN_POINT('Ctrl Pts',(-13.0508216223155,51.1458333401613,-48.706329375));
#8826=CARTESIAN_POINT('Ctrl Pts',(1.59157945007855E-14,50.937500006828,
-48.706329375));
#8827=CARTESIAN_POINT('Ctrl Pts',(13.0508216223155,50.7291666734946,-48.706329375));
#8828=CARTESIAN_POINT('Ctrl Pts',(24.3531646875,50.5208333401613,-42.1809185638422));
#8829=CARTESIAN_POINT('Ctrl Pts',(35.6555077526845,50.312500006828,-35.6555077526845));
#8830=CARTESIAN_POINT('Ctrl Pts',(42.1809185638422,50.1041666734946,-24.3531646875));
#8831=CARTESIAN_POINT('Ctrl Pts',(48.706329375,49.8958333401613,-13.0508216223155));
#8832=CARTESIAN_POINT('Ctrl Pts',(48.706329375,49.687500006828,1.293339198242E-14));
#8833=CARTESIAN_POINT('Ctrl Pts',(48.706329375,49.4791666734946,13.0508216223155));
#8834=CARTESIAN_POINT('Ctrl Pts',(42.1809185638422,49.2708333401613,24.3531646875));
#8835=CARTESIAN_POINT('Ctrl Pts',(35.6555077526845,49.062500006828,35.6555077526845));
#8836=CARTESIAN_POINT('Ctrl Pts',(24.3531646875,48.8541666734946,42.1809185638422));
#8837=CARTESIAN_POINT('Ctrl Pts',(13.0508216223155,48.6458333401613,48.706329375));
#8838=CARTESIAN_POINT('Ctrl Pts',(-9.95098946405443E-15,48.437500006828,
48.706329375));
#8839=CARTESIAN_POINT('Ctrl Pts',(-13.0508216223155,48.2291666734946,48.706329375));
#8840=CARTESIAN_POINT('Ctrl Pts',(-24.3531646875,48.0208333401613,42.1809185638423));
#8841=CARTESIAN_POINT('Ctrl Pts',(-35.6555077526845,47.812500006828,35.6555077526845));
#8842=CARTESIAN_POINT('Ctrl Pts',(-42.1809185638422,47.6041666734946,24.3531646875));
#8843=CARTESIAN_POINT('Ctrl Pts',(-48.706329375,47.3958333401613,13.0508216223155));
#8844=CARTESIAN_POINT('Ctrl Pts',(-48.706329375,47.187500006828,-1.8898197019151E-14));
#8845=CARTESIAN_POINT('Ctrl Pts',(-48.706329375,46.9791666734946,-13.0508216223155));
#8846=CARTESIAN_POINT('Ctrl Pts',(-42.1809185638422,46.7708333401613,-24.3531646875));
#8847=CARTESIAN_POINT('Ctrl Pts',(-35.6555077526845,46.562500006828,-35.6555077526845));
#8848=CARTESIAN_POINT('Ctrl Pts',(-24.3531646875,46.3541666734946,-42.1809185638423));
#8849=CARTESIAN_POINT('Ctrl Pts',(-13.0508216223155,46.1458333401613,-48.706329375));
#8850=CARTESIAN_POINT('Ctrl Pts',(1.59157945007855E-14,45.937500006828,
-48.706329375));
#8851=CARTESIAN_POINT('Ctrl Pts',(13.0508216223155,45.7291666734946,-48.706329375));
#8852=CARTESIAN_POINT('Ctrl Pts',(24.3531646875,45.5208333401613,-42.1809185638422));
#8853=CARTESIAN_POINT('Ctrl Pts',(35.6555077526845,45.312500006828,-35.6555077526845));
#8854=CARTESIAN_POINT('Ctrl Pts',(42.1809185638422,45.1041666734946,-24.3531646875));
#8855=CARTESIAN_POINT('Ctrl Pts',(48.706329375,44.8958333401613,-13.0508216223155));
#8856=CARTESIAN_POINT('Ctrl Pts',(48.706329375,44.687500006828,1.293339198242E-14));
#8857=CARTESIAN_POINT('Ctrl Pts',(48.706329375,44.4791666734946,13.0508216223155));
#8858=CARTESIAN_POINT('Ctrl Pts',(42.1809185638422,44.2708333401613,24.3531646875));
#8859=CARTESIAN_POINT('Ctrl Pts',(35.6555077526845,44.062500006828,35.6555077526845));
#8860=CARTESIAN_POINT('Ctrl Pts',(24.3531646875,43.8541666734946,42.1809185638422));
#8861=CARTESIAN_POINT('Ctrl Pts',(13.0508216223155,43.6458333401613,48.706329375));
#8862=CARTESIAN_POINT('Ctrl Pts',(-9.95098946405443E-15,43.437500006828,
48.706329375));
#8863=CARTESIAN_POINT('Ctrl Pts',(-13.0508216223155,43.2291666734946,48.706329375));
#8864=CARTESIAN_POINT('Ctrl Pts',(-24.3531646875,43.0208333401613,42.1809185638423));
#8865=CARTESIAN_POINT('Ctrl Pts',(-35.6555077526845,42.812500006828,35.6555077526845));
#8866=CARTESIAN_POINT('Ctrl Pts',(-42.1809185638422,42.6041666734946,24.3531646875));
#8867=CARTESIAN_POINT('Ctrl Pts',(-48.706329375,42.3958333401613,13.0508216223155));
#8868=CARTESIAN_POINT('Ctrl Pts',(-48.706329375,42.187500006828,-1.8898197019151E-14));
#8869=CARTESIAN_POINT('Ctrl Pts',(-48.706329375,41.9791666734946,-13.0508216223155));
#8870=CARTESIAN_POINT('Ctrl Pts',(-42.1809185638422,41.7708333401613,-24.3531646875));
#8871=CARTESIAN_POINT('Ctrl Pts',(-35.6555077526845,41.562500006828,-35.6555077526845));
#8872=CARTESIAN_POINT('Ctrl Pts',(-24.3531646875,41.3541666734946,-42.1809185638423));
#8873=CARTESIAN_POINT('Ctrl Pts',(-13.0508216223155,41.1458333401613,-48.706329375));
#8874=CARTESIAN_POINT('Ctrl Pts',(1.59157945007855E-14,40.937500006828,
-48.706329375));
#8875=CARTESIAN_POINT('Ctrl Pts',(13.0508216223155,40.7291666734946,-48.706329375));
#8876=CARTESIAN_POINT('Ctrl Pts',(24.3531646875,40.5208333401613,-42.1809185638422));
#8877=CARTESIAN_POINT('Ctrl Pts',(35.6555077526845,40.312500006828,-35.6555077526845));
#8878=CARTESIAN_POINT('Ctrl Pts',(42.1809185638422,40.1041666734946,-24.3531646875));
#8879=CARTESIAN_POINT('Ctrl Pts',(48.706329375,39.8958333401613,-13.0508216223155));
#8880=CARTESIAN_POINT('Ctrl Pts',(48.706329375,39.687500006828,1.293339198242E-14));
#8881=CARTESIAN_POINT('Ctrl Pts',(48.706329375,39.4791666734946,13.0508216223155));
#8882=CARTESIAN_POINT('Ctrl Pts',(42.1809185638422,39.2708333401613,24.3531646875));
#8883=CARTESIAN_POINT('Ctrl Pts',(35.6555077526845,39.062500006828,35.6555077526845));
#8884=CARTESIAN_POINT('Ctrl Pts',(24.3531646875,38.8541666734946,42.1809185638422));
#8885=CARTESIAN_POINT('Ctrl Pts',(13.0508216223155,38.6458333401613,48.706329375));
#8886=CARTESIAN_POINT('Ctrl Pts',(-9.95098946405443E-15,38.437500006828,
48.706329375));
#8887=CARTESIAN_POINT('Ctrl Pts',(-13.0508216223155,38.2291666734946,48.706329375));
#8888=CARTESIAN_POINT('Ctrl Pts',(-24.3531646875,38.0208333401613,42.1809185638423));
#8889=CARTESIAN_POINT('Ctrl Pts',(-35.6555077526845,37.812500006828,35.6555077526845));
#8890=CARTESIAN_POINT('Ctrl Pts',(-42.1809185638422,37.6041666734946,24.3531646875));
#8891=CARTESIAN_POINT('Ctrl Pts',(-48.706329375,37.3958333401613,13.0508216223155));
#8892=CARTESIAN_POINT('Ctrl Pts',(-48.706329375,37.187500006828,-1.8898197019151E-14));
#8893=CARTESIAN_POINT('Ctrl Pts',(-48.706329375,36.9791666734946,-13.0508216223155));
#8894=CARTESIAN_POINT('Ctrl Pts',(-42.1809185638422,36.7708333401613,-24.3531646875));
#8895=CARTESIAN_POINT('Ctrl Pts',(-35.6555077526845,36.562500006828,-35.6555077526845));
#8896=CARTESIAN_POINT('Ctrl Pts',(-24.3531646875,36.3541666734946,-42.1809185638423));
#8897=CARTESIAN_POINT('Ctrl Pts',(-13.0508216223155,36.1458333401613,-48.706329375));
#8898=CARTESIAN_POINT('Ctrl Pts',(1.59157945007855E-14,35.937500006828,
-48.706329375));
#8899=CARTESIAN_POINT('Ctrl Pts',(13.0508216223155,35.7291666734946,-48.706329375));
#8900=CARTESIAN_POINT('Ctrl Pts',(24.3531646875,35.5208333401613,-42.1809185638422));
#8901=CARTESIAN_POINT('Ctrl Pts',(35.6555077526845,35.312500006828,-35.6555077526845));
#8902=CARTESIAN_POINT('Ctrl Pts',(42.1809185638422,35.1041666734946,-24.3531646875));
#8903=CARTESIAN_POINT('Ctrl Pts',(48.706329375,34.8958333401613,-13.0508216223155));
#8904=CARTESIAN_POINT('Ctrl Pts',(48.706329375,34.687500006828,1.293339198242E-14));
#8905=CARTESIAN_POINT('Ctrl Pts',(48.706329375,34.4791666734946,13.0508216223155));
#8906=CARTESIAN_POINT('Ctrl Pts',(42.1809185638422,34.2708333401613,24.3531646875));
#8907=CARTESIAN_POINT('Ctrl Pts',(35.6555077526845,34.062500006828,35.6555077526845));
#8908=CARTESIAN_POINT('Ctrl Pts',(24.3531646875,33.8541666734946,42.1809185638422));
#8909=CARTESIAN_POINT('Ctrl Pts',(13.0508216223155,33.6458333401613,48.706329375));
#8910=CARTESIAN_POINT('Ctrl Pts',(-9.95098946405443E-15,33.437500006828,
48.706329375));
#8911=CARTESIAN_POINT('Ctrl Pts',(-13.0508216223155,33.2291666734946,48.706329375));
#8912=CARTESIAN_POINT('Ctrl Pts',(-24.3531646875,33.0208333401613,42.1809185638423));
#8913=CARTESIAN_POINT('Ctrl Pts',(-35.6555077526845,32.812500006828,35.6555077526845));
#8914=CARTESIAN_POINT('Ctrl Pts',(-42.1809185638422,32.6041666734946,24.3531646875));
#8915=CARTESIAN_POINT('Ctrl Pts',(-48.706329375,32.3958333401613,13.0508216223155));
#8916=CARTESIAN_POINT('Ctrl Pts',(-48.706329375,32.187500006828,-1.8898197019151E-14));
#8917=CARTESIAN_POINT('Ctrl Pts',(-48.706329375,31.9791666734946,-13.0508216223155));
#8918=CARTESIAN_POINT('Ctrl Pts',(-42.1809185638422,31.7708333401613,-24.3531646875));
#8919=CARTESIAN_POINT('Ctrl Pts',(-35.6555077526845,31.562500006828,-35.6555077526845));
#8920=CARTESIAN_POINT('Ctrl Pts',(-24.3531646875,31.3541666734946,-42.1809185638423));
#8921=CARTESIAN_POINT('Ctrl Pts',(-13.0508216223155,31.1458333401613,-48.706329375));
#8922=CARTESIAN_POINT('Ctrl Pts',(1.59157945007855E-14,30.937500006828,
-48.706329375));
#8923=CARTESIAN_POINT('Ctrl Pts',(13.0508216223155,30.7291666734946,-48.706329375));
#8924=CARTESIAN_POINT('Ctrl Pts',(24.3531646875,30.5208333401613,-42.1809185638422));
#8925=CARTESIAN_POINT('Ctrl Pts',(35.6555077526845,30.312500006828,-35.6555077526845));
#8926=CARTESIAN_POINT('Ctrl Pts',(42.1809185638422,30.1041666734946,-24.3531646875));
#8927=CARTESIAN_POINT('Ctrl Pts',(48.706329375,29.8958333401613,-13.0508216223155));
#8928=CARTESIAN_POINT('Ctrl Pts',(48.706329375,29.687500006828,1.293339198242E-14));
#8929=CARTESIAN_POINT('Ctrl Pts',(48.706329375,29.4791666734946,13.0508216223155));
#8930=CARTESIAN_POINT('Ctrl Pts',(42.1809185638422,29.2708333401613,24.3531646875));
#8931=CARTESIAN_POINT('Ctrl Pts',(35.6555077526845,29.062500006828,35.6555077526845));
#8932=CARTESIAN_POINT('Ctrl Pts',(24.3531646875,28.8541666734946,42.1809185638422));
#8933=CARTESIAN_POINT('Ctrl Pts',(13.0508216223155,28.6458333401613,48.706329375));
#8934=CARTESIAN_POINT('Ctrl Pts',(-9.95098946405443E-15,28.437500006828,
48.706329375));
#8935=CARTESIAN_POINT('Ctrl Pts',(-13.0508216223155,28.2291666734946,48.706329375));
#8936=CARTESIAN_POINT('Ctrl Pts',(-24.3531646875,28.0208333401613,42.1809185638423));
#8937=CARTESIAN_POINT('Ctrl Pts',(-35.6555077526845,27.812500006828,35.6555077526845));
#8938=CARTESIAN_POINT('Ctrl Pts',(-42.1809185638422,27.6041666734946,24.3531646875));
#8939=CARTESIAN_POINT('Ctrl Pts',(-48.706329375,27.3958333401613,13.0508216223155));
#8940=CARTESIAN_POINT('Ctrl Pts',(-48.706329375,27.187500006828,-1.8898197019151E-14));
#8941=CARTESIAN_POINT('',(-4.32456003949878,53.3676432269777,48.5139639861634));
#8942=CARTESIAN_POINT('',(-48.5725845633798,52.2456516907297,3.60701400320327));
#8943=CARTESIAN_POINT('Ctrl Pts',(-4.32456003949878,53.3676432269777,48.5139639861634));
#8944=CARTESIAN_POINT('Ctrl Pts',(-15.038141415499,53.1925348924095,47.5589497574396));
#8945=CARTESIAN_POINT('Ctrl Pts',(-24.3531646875,53.0208333401613,42.1809185638423));
#8946=CARTESIAN_POINT('Ctrl Pts',(-35.6555077526845,52.812500006828,35.6555077526845));
#8947=CARTESIAN_POINT('Ctrl Pts',(-42.1809185638422,52.6041666734946,24.3531646875));
#8948=CARTESIAN_POINT('Ctrl Pts',(-47.7480251419551,52.4264286116309,14.7106532430575));
#8949=CARTESIAN_POINT('Ctrl Pts',(-48.5725845633798,52.2456516907297,3.60701400320327));
#8950=CARTESIAN_POINT('Ctrl Pts',(-48.5725845633798,52.2456516907297,3.60701400320327));
#8951=CARTESIAN_POINT('Ctrl Pts',(-48.3407853679392,52.1124685639422,3.60701400320327));
#8952=CARTESIAN_POINT('Ctrl Pts',(-48.1089821836664,51.9792923792741,3.60701400320327));
#8953=CARTESIAN_POINT('Ctrl Pts',(-47.6453674864979,51.7129545080418,3.60701400320327));
#8954=CARTESIAN_POINT('Ctrl Pts',(-47.4135559734253,51.5797928212585,3.60701400320325));
#8955=CARTESIAN_POINT('Ctrl Pts',(-47.1817401099609,51.4466387085919,3.60701400320325));
#8956=CARTESIAN_POINT('Ctrl Pts',(-46.7406305897488,51.1932671494809,3.60701400320325));
#8957=CARTESIAN_POINT('Ctrl Pts',(-46.2995053259033,50.9399229970588,3.60701400320327));
#8958=CARTESIAN_POINT('Ctrl Pts',(-45.858362923034,50.686608693912,3.60701400320327));
#8959=CARTESIAN_POINT('Ctrl Pts',(-4.32456003949877,51.8009818542622,45.7962681936506));
#8960=CARTESIAN_POINT('Ctrl Pts',(-4.32456003949877,51.9344874667937,46.0278818021281));
#8961=CARTESIAN_POINT('Ctrl Pts',(-4.32456003949885,52.2015035419424,46.4911062234486));
#8962=CARTESIAN_POINT('Ctrl Pts',(-4.32456003949878,52.4685288945405,46.954325296818));
#8963=CARTESIAN_POINT('Ctrl Pts',(-4.32456003949878,52.8572357107336,47.6286149142205));
#8964=CARTESIAN_POINT('Ctrl Pts',(-4.32456003949878,53.1124357360102,48.0712916022845));
#8965=CARTESIAN_POINT('Ctrl Pts',(-4.32456003949878,53.3676432269777,48.5139639861634));
#8966=CARTESIAN_POINT('Ctrl Pts',(-46.,55.6250000136559,0.));
#8967=CARTESIAN_POINT('Ctrl Pts',(-46.,55.4166666803226,-12.3256628518316));
#8968=CARTESIAN_POINT('Ctrl Pts',(-39.8371685740842,55.2083333469893,-23.));
#8969=CARTESIAN_POINT('Ctrl Pts',(-33.6743371481684,55.0000000136559,-33.6743371481684));
#8970=CARTESIAN_POINT('Ctrl Pts',(-23.,54.7916666803226,-39.8371685740842));
#8971=CARTESIAN_POINT('Ctrl Pts',(-12.3256628518317,54.5833333469893,-46.));
#8972=CARTESIAN_POINT('Ctrl Pts',(-2.81668763803891E-15,54.3750000136559,
-46.));
#8973=CARTESIAN_POINT('Ctrl Pts',(12.3256628518316,54.1666666803226,-46.));
#8974=CARTESIAN_POINT('Ctrl Pts',(23.,53.9583333469893,-39.8371685740842));
#8975=CARTESIAN_POINT('Ctrl Pts',(33.6743371481683,53.7500000136559,-33.6743371481684));
#8976=CARTESIAN_POINT('Ctrl Pts',(39.8371685740842,53.5416666803226,-23.));
#8977=CARTESIAN_POINT('Ctrl Pts',(46.,53.3333333469893,-12.3256628518317));
#8978=CARTESIAN_POINT('Ctrl Pts',(46.,53.1250000136559,-5.63337527607782E-15));
#8979=CARTESIAN_POINT('Ctrl Pts',(46.,52.9166666803226,12.3256628518316));
#8980=CARTESIAN_POINT('Ctrl Pts',(39.8371685740842,52.7083333469893,23.));
#8981=CARTESIAN_POINT('Ctrl Pts',(33.6743371481684,52.5000000136559,33.6743371481683));
#8982=CARTESIAN_POINT('Ctrl Pts',(23.,52.2916666803226,39.8371685740842));
#8983=CARTESIAN_POINT('Ctrl Pts',(12.3256628518317,52.0833333469893,46.));
#8984=CARTESIAN_POINT('Ctrl Pts',(8.45006291411674E-15,51.8750000136559,
46.));
#8985=CARTESIAN_POINT('Ctrl Pts',(-12.3256628518316,51.6666666803226,46.));
#8986=CARTESIAN_POINT('Ctrl Pts',(-23.,51.4583333469893,39.8371685740842));
#8987=CARTESIAN_POINT('Ctrl Pts',(-33.6743371481683,51.2500000136559,33.6743371481684));
#8988=CARTESIAN_POINT('Ctrl Pts',(-39.8371685740842,51.0416666803226,23.));
#8989=CARTESIAN_POINT('Ctrl Pts',(-46.,50.8333333469893,12.3256628518317));
#8990=CARTESIAN_POINT('Ctrl Pts',(-46.,50.6250000136559,0.));
#8991=CARTESIAN_POINT('Ctrl Pts',(-46.,50.4166666803226,-12.3256628518316));
#8992=CARTESIAN_POINT('Ctrl Pts',(-39.8371685740842,50.2083333469893,-23.));
#8993=CARTESIAN_POINT('Ctrl Pts',(-33.6743371481684,50.0000000136559,-33.6743371481684));
#8994=CARTESIAN_POINT('Ctrl Pts',(-23.,49.7916666803226,-39.8371685740842));
#8995=CARTESIAN_POINT('Ctrl Pts',(-12.3256628518317,49.5833333469893,-46.));
#8996=CARTESIAN_POINT('Ctrl Pts',(-2.81668763803891E-15,49.3750000136559,
-46.));
#8997=CARTESIAN_POINT('Ctrl Pts',(12.3256628518316,49.1666666803226,-46.));
#8998=CARTESIAN_POINT('Ctrl Pts',(23.,48.9583333469893,-39.8371685740842));
#8999=CARTESIAN_POINT('Ctrl Pts',(33.6743371481683,48.7500000136559,-33.6743371481684));
#9000=CARTESIAN_POINT('Ctrl Pts',(39.8371685740842,48.5416666803226,-23.));
#9001=CARTESIAN_POINT('Ctrl Pts',(46.,48.3333333469893,-12.3256628518317));
#9002=CARTESIAN_POINT('Ctrl Pts',(46.,48.1250000136559,-5.63337527607782E-15));
#9003=CARTESIAN_POINT('Ctrl Pts',(46.,47.9166666803226,12.3256628518316));
#9004=CARTESIAN_POINT('Ctrl Pts',(39.8371685740842,47.7083333469893,23.));
#9005=CARTESIAN_POINT('Ctrl Pts',(33.6743371481684,47.5000000136559,33.6743371481683));
#9006=CARTESIAN_POINT('Ctrl Pts',(23.,47.2916666803226,39.8371685740842));
#9007=CARTESIAN_POINT('Ctrl Pts',(12.3256628518317,47.0833333469893,46.));
#9008=CARTESIAN_POINT('Ctrl Pts',(8.45006291411674E-15,46.8750000136559,
46.));
#9009=CARTESIAN_POINT('Ctrl Pts',(-12.3256628518316,46.6666666803226,46.));
#9010=CARTESIAN_POINT('Ctrl Pts',(-23.,46.4583333469893,39.8371685740842));
#9011=CARTESIAN_POINT('Ctrl Pts',(-33.6743371481683,46.2500000136559,33.6743371481684));
#9012=CARTESIAN_POINT('Ctrl Pts',(-39.8371685740842,46.0416666803226,23.));
#9013=CARTESIAN_POINT('Ctrl Pts',(-46.,45.8333333469892,12.3256628518317));
#9014=CARTESIAN_POINT('Ctrl Pts',(-46.,45.6250000136559,0.));
#9015=CARTESIAN_POINT('Ctrl Pts',(-46.,45.4166666803226,-12.3256628518316));
#9016=CARTESIAN_POINT('Ctrl Pts',(-39.8371685740842,45.2083333469893,-23.));
#9017=CARTESIAN_POINT('Ctrl Pts',(-33.6743371481684,45.0000000136559,-33.6743371481684));
#9018=CARTESIAN_POINT('Ctrl Pts',(-23.,44.7916666803226,-39.8371685740842));
#9019=CARTESIAN_POINT('Ctrl Pts',(-12.3256628518317,44.5833333469893,-46.));
#9020=CARTESIAN_POINT('Ctrl Pts',(-2.81668763803891E-15,44.3750000136559,
-46.));
#9021=CARTESIAN_POINT('Ctrl Pts',(12.3256628518316,44.1666666803226,-46.));
#9022=CARTESIAN_POINT('Ctrl Pts',(23.,43.9583333469893,-39.8371685740842));
#9023=CARTESIAN_POINT('Ctrl Pts',(33.6743371481683,43.7500000136559,-33.6743371481684));
#9024=CARTESIAN_POINT('Ctrl Pts',(39.8371685740842,43.5416666803226,-23.));
#9025=CARTESIAN_POINT('Ctrl Pts',(46.,43.3333333469893,-12.3256628518317));
#9026=CARTESIAN_POINT('Ctrl Pts',(46.,43.1250000136559,-5.63337527607782E-15));
#9027=CARTESIAN_POINT('Ctrl Pts',(46.,42.9166666803226,12.3256628518316));
#9028=CARTESIAN_POINT('Ctrl Pts',(39.8371685740842,42.7083333469893,23.));
#9029=CARTESIAN_POINT('Ctrl Pts',(33.6743371481684,42.5000000136559,33.6743371481683));
#9030=CARTESIAN_POINT('Ctrl Pts',(23.,42.2916666803226,39.8371685740842));
#9031=CARTESIAN_POINT('Ctrl Pts',(12.3256628518317,42.0833333469893,46.));
#9032=CARTESIAN_POINT('Ctrl Pts',(8.45006291411674E-15,41.8750000136559,
46.));
#9033=CARTESIAN_POINT('Ctrl Pts',(-12.3256628518316,41.6666666803226,46.));
#9034=CARTESIAN_POINT('Ctrl Pts',(-23.,41.4583333469893,39.8371685740842));
#9035=CARTESIAN_POINT('Ctrl Pts',(-33.6743371481683,41.2500000136559,33.6743371481684));
#9036=CARTESIAN_POINT('Ctrl Pts',(-39.8371685740842,41.0416666803226,23.));
#9037=CARTESIAN_POINT('Ctrl Pts',(-46.,40.8333333469893,12.3256628518317));
#9038=CARTESIAN_POINT('Ctrl Pts',(-46.,40.6250000136559,0.));
#9039=CARTESIAN_POINT('Ctrl Pts',(-46.,40.4166666803226,-12.3256628518316));
#9040=CARTESIAN_POINT('Ctrl Pts',(-39.8371685740842,40.2083333469893,-23.));
#9041=CARTESIAN_POINT('Ctrl Pts',(-33.6743371481684,40.0000000136559,-33.6743371481684));
#9042=CARTESIAN_POINT('Ctrl Pts',(-23.,39.7916666803226,-39.8371685740842));
#9043=CARTESIAN_POINT('Ctrl Pts',(-12.3256628518317,39.5833333469893,-46.));
#9044=CARTESIAN_POINT('Ctrl Pts',(-2.81668763803891E-15,39.3750000136559,
-46.));
#9045=CARTESIAN_POINT('Ctrl Pts',(12.3256628518316,39.1666666803226,-46.));
#9046=CARTESIAN_POINT('Ctrl Pts',(23.,38.9583333469893,-39.8371685740842));
#9047=CARTESIAN_POINT('Ctrl Pts',(33.6743371481683,38.7500000136559,-33.6743371481684));
#9048=CARTESIAN_POINT('Ctrl Pts',(39.8371685740842,38.5416666803226,-23.));
#9049=CARTESIAN_POINT('Ctrl Pts',(46.,38.3333333469893,-12.3256628518317));
#9050=CARTESIAN_POINT('Ctrl Pts',(46.,38.1250000136559,-5.63337527607782E-15));
#9051=CARTESIAN_POINT('Ctrl Pts',(46.,37.9166666803226,12.3256628518316));
#9052=CARTESIAN_POINT('Ctrl Pts',(39.8371685740842,37.7083333469893,23.));
#9053=CARTESIAN_POINT('Ctrl Pts',(33.6743371481684,37.5000000136559,33.6743371481683));
#9054=CARTESIAN_POINT('Ctrl Pts',(23.,37.2916666803226,39.8371685740842));
#9055=CARTESIAN_POINT('Ctrl Pts',(12.3256628518317,37.0833333469893,46.));
#9056=CARTESIAN_POINT('Ctrl Pts',(8.45006291411674E-15,36.8750000136559,
46.));
#9057=CARTESIAN_POINT('Ctrl Pts',(-12.3256628518316,36.6666666803226,46.));
#9058=CARTESIAN_POINT('Ctrl Pts',(-23.,36.4583333469893,39.8371685740842));
#9059=CARTESIAN_POINT('Ctrl Pts',(-33.6743371481683,36.2500000136559,33.6743371481684));
#9060=CARTESIAN_POINT('Ctrl Pts',(-39.8371685740842,36.0416666803226,23.));
#9061=CARTESIAN_POINT('Ctrl Pts',(-46.,35.8333333469893,12.3256628518317));
#9062=CARTESIAN_POINT('Ctrl Pts',(-46.,35.6250000136559,0.));
#9063=CARTESIAN_POINT('Ctrl Pts',(-46.,35.4166666803226,-12.3256628518316));
#9064=CARTESIAN_POINT('Ctrl Pts',(-39.8371685740842,35.2083333469893,-23.));
#9065=CARTESIAN_POINT('Ctrl Pts',(-33.6743371481684,35.0000000136559,-33.6743371481684));
#9066=CARTESIAN_POINT('Ctrl Pts',(-23.,34.7916666803226,-39.8371685740842));
#9067=CARTESIAN_POINT('Ctrl Pts',(-12.3256628518317,34.5833333469893,-46.));
#9068=CARTESIAN_POINT('Ctrl Pts',(-2.81668763803891E-15,34.3750000136559,
-46.));
#9069=CARTESIAN_POINT('Ctrl Pts',(12.3256628518316,34.1666666803226,-46.));
#9070=CARTESIAN_POINT('Ctrl Pts',(23.,33.9583333469893,-39.8371685740842));
#9071=CARTESIAN_POINT('Ctrl Pts',(33.6743371481683,33.7500000136559,-33.6743371481684));
#9072=CARTESIAN_POINT('Ctrl Pts',(39.8371685740842,33.5416666803226,-23.));
#9073=CARTESIAN_POINT('Ctrl Pts',(46.,33.3333333469893,-12.3256628518317));
#9074=CARTESIAN_POINT('Ctrl Pts',(46.,33.1250000136559,-5.63337527607782E-15));
#9075=CARTESIAN_POINT('Ctrl Pts',(46.,32.9166666803226,12.3256628518316));
#9076=CARTESIAN_POINT('Ctrl Pts',(39.8371685740842,32.7083333469893,23.));
#9077=CARTESIAN_POINT('Ctrl Pts',(33.6743371481684,32.5000000136559,33.6743371481683));
#9078=CARTESIAN_POINT('Ctrl Pts',(23.,32.2916666803226,39.8371685740842));
#9079=CARTESIAN_POINT('Ctrl Pts',(12.3256628518317,32.0833333469893,46.));
#9080=CARTESIAN_POINT('Ctrl Pts',(8.45006291411674E-15,31.8750000136559,
46.));
#9081=CARTESIAN_POINT('Ctrl Pts',(-12.3256628518316,31.6666666803226,46.));
#9082=CARTESIAN_POINT('Ctrl Pts',(-23.,31.4583333469893,39.8371685740842));
#9083=CARTESIAN_POINT('Ctrl Pts',(-33.6743371481683,31.2500000136559,33.6743371481684));
#9084=CARTESIAN_POINT('Ctrl Pts',(-39.8371685740842,31.0416666803226,23.));
#9085=CARTESIAN_POINT('Ctrl Pts',(-46.,30.8333333469893,12.3256628518317));
#9086=CARTESIAN_POINT('Ctrl Pts',(-46.,30.6250000136559,0.));
#9087=CARTESIAN_POINT('Ctrl Pts',(-46.,30.4166666803226,-12.3256628518316));
#9088=CARTESIAN_POINT('Ctrl Pts',(-39.8371685740842,30.2083333469893,-23.));
#9089=CARTESIAN_POINT('Ctrl Pts',(-33.6743371481684,30.0000000136559,-33.6743371481684));
#9090=CARTESIAN_POINT('Ctrl Pts',(-23.,29.7916666803226,-39.8371685740842));
#9091=CARTESIAN_POINT('Ctrl Pts',(-12.3256628518317,29.5833333469893,-46.));
#9092=CARTESIAN_POINT('Ctrl Pts',(-2.81668763803891E-15,29.3750000136559,
-46.));
#9093=CARTESIAN_POINT('Ctrl Pts',(12.3256628518316,29.1666666803226,-46.));
#9094=CARTESIAN_POINT('Ctrl Pts',(23.,28.9583333469893,-39.8371685740842));
#9095=CARTESIAN_POINT('Ctrl Pts',(33.6743371481683,28.7500000136559,-33.6743371481684));
#9096=CARTESIAN_POINT('Ctrl Pts',(39.8371685740842,28.5416666803226,-23.));
#9097=CARTESIAN_POINT('Ctrl Pts',(46.,28.3333333469893,-12.3256628518317));
#9098=CARTESIAN_POINT('Ctrl Pts',(46.,28.1250000136559,-5.63337527607782E-15));
#9099=CARTESIAN_POINT('Ctrl Pts',(46.,27.9166666803226,12.3256628518316));
#9100=CARTESIAN_POINT('Ctrl Pts',(39.8371685740842,27.7083333469893,23.));
#9101=CARTESIAN_POINT('Ctrl Pts',(33.6743371481684,27.5000000136559,33.6743371481683));
#9102=CARTESIAN_POINT('Ctrl Pts',(23.,27.2916666803226,39.8371685740842));
#9103=CARTESIAN_POINT('Ctrl Pts',(12.3256628518317,27.0833333469893,46.));
#9104=CARTESIAN_POINT('Ctrl Pts',(8.45006291411674E-15,26.8750000136559,
46.));
#9105=CARTESIAN_POINT('Ctrl Pts',(-12.3256628518316,26.6666666803226,46.));
#9106=CARTESIAN_POINT('Ctrl Pts',(-23.,26.4583333469893,39.8371685740842));
#9107=CARTESIAN_POINT('Ctrl Pts',(-33.6743371481683,26.2500000136559,33.6743371481684));
#9108=CARTESIAN_POINT('Ctrl Pts',(-39.8371685740842,26.0416666803226,23.));
#9109=CARTESIAN_POINT('Ctrl Pts',(-46.,25.8333333469893,12.3256628518317));
#9110=CARTESIAN_POINT('Ctrl Pts',(-46.,25.6250000136559,0.));
#9111=CARTESIAN_POINT('Ctrl Pts',(-48.706329375,57.187500006828,-1.8898197019151E-14));
#9112=CARTESIAN_POINT('Ctrl Pts',(-48.706329375,56.9791666734946,-13.0508216223155));
#9113=CARTESIAN_POINT('Ctrl Pts',(-42.1809185638422,56.7708333401613,-24.3531646875));
#9114=CARTESIAN_POINT('Ctrl Pts',(-35.6555077526845,56.562500006828,-35.6555077526845));
#9115=CARTESIAN_POINT('Ctrl Pts',(-24.3531646875,56.3541666734946,-42.1809185638423));
#9116=CARTESIAN_POINT('Ctrl Pts',(-13.0508216223155,56.1458333401613,-48.706329375));
#9117=CARTESIAN_POINT('Ctrl Pts',(1.59157945007855E-14,55.937500006828,
-48.706329375));
#9118=CARTESIAN_POINT('Ctrl Pts',(13.0508216223155,55.7291666734946,-48.706329375));
#9119=CARTESIAN_POINT('Ctrl Pts',(24.3531646875,55.5208333401613,-42.1809185638422));
#9120=CARTESIAN_POINT('Ctrl Pts',(35.6555077526845,55.312500006828,-35.6555077526845));
#9121=CARTESIAN_POINT('Ctrl Pts',(42.1809185638422,55.1041666734946,-24.3531646875));
#9122=CARTESIAN_POINT('Ctrl Pts',(48.706329375,54.8958333401613,-13.0508216223155));
#9123=CARTESIAN_POINT('Ctrl Pts',(48.706329375,54.687500006828,1.293339198242E-14));
#9124=CARTESIAN_POINT('Ctrl Pts',(48.706329375,54.4791666734946,13.0508216223155));
#9125=CARTESIAN_POINT('Ctrl Pts',(42.1809185638422,54.2708333401613,24.3531646875));
#9126=CARTESIAN_POINT('Ctrl Pts',(35.6555077526845,54.062500006828,35.6555077526845));
#9127=CARTESIAN_POINT('Ctrl Pts',(24.3531646875,53.8541666734946,42.1809185638422));
#9128=CARTESIAN_POINT('Ctrl Pts',(13.0508216223155,53.6458333401613,48.706329375));
#9129=CARTESIAN_POINT('Ctrl Pts',(-9.95098946405443E-15,53.437500006828,
48.706329375));
#9130=CARTESIAN_POINT('Ctrl Pts',(-13.0508216223155,53.2291666734946,48.706329375));
#9131=CARTESIAN_POINT('Ctrl Pts',(-24.3531646875,53.0208333401613,42.1809185638423));
#9132=CARTESIAN_POINT('Ctrl Pts',(-35.6555077526845,52.812500006828,35.6555077526845));
#9133=CARTESIAN_POINT('Ctrl Pts',(-42.1809185638422,52.6041666734946,24.3531646875));
#9134=CARTESIAN_POINT('Ctrl Pts',(-48.706329375,52.3958333401613,13.0508216223155));
#9135=CARTESIAN_POINT('Ctrl Pts',(-48.706329375,52.187500006828,-1.8898197019151E-14));
#9136=CARTESIAN_POINT('Ctrl Pts',(-48.706329375,51.9791666734946,-13.0508216223155));
#9137=CARTESIAN_POINT('Ctrl Pts',(-42.1809185638422,51.7708333401613,-24.3531646875));
#9138=CARTESIAN_POINT('Ctrl Pts',(-35.6555077526845,51.562500006828,-35.6555077526845));
#9139=CARTESIAN_POINT('Ctrl Pts',(-24.3531646875,51.3541666734946,-42.1809185638423));
#9140=CARTESIAN_POINT('Ctrl Pts',(-13.0508216223155,51.1458333401613,-48.706329375));
#9141=CARTESIAN_POINT('Ctrl Pts',(1.59157945007855E-14,50.937500006828,
-48.706329375));
#9142=CARTESIAN_POINT('Ctrl Pts',(13.0508216223155,50.7291666734946,-48.706329375));
#9143=CARTESIAN_POINT('Ctrl Pts',(24.3531646875,50.5208333401613,-42.1809185638422));
#9144=CARTESIAN_POINT('Ctrl Pts',(35.6555077526845,50.312500006828,-35.6555077526845));
#9145=CARTESIAN_POINT('Ctrl Pts',(42.1809185638422,50.1041666734946,-24.3531646875));
#9146=CARTESIAN_POINT('Ctrl Pts',(48.706329375,49.8958333401613,-13.0508216223155));
#9147=CARTESIAN_POINT('Ctrl Pts',(48.706329375,49.687500006828,1.293339198242E-14));
#9148=CARTESIAN_POINT('Ctrl Pts',(48.706329375,49.4791666734946,13.0508216223155));
#9149=CARTESIAN_POINT('Ctrl Pts',(42.1809185638422,49.2708333401613,24.3531646875));
#9150=CARTESIAN_POINT('Ctrl Pts',(35.6555077526845,49.062500006828,35.6555077526845));
#9151=CARTESIAN_POINT('Ctrl Pts',(24.3531646875,48.8541666734946,42.1809185638422));
#9152=CARTESIAN_POINT('Ctrl Pts',(13.0508216223155,48.6458333401613,48.706329375));
#9153=CARTESIAN_POINT('Ctrl Pts',(-9.95098946405443E-15,48.437500006828,
48.706329375));
#9154=CARTESIAN_POINT('Ctrl Pts',(-13.0508216223155,48.2291666734946,48.706329375));
#9155=CARTESIAN_POINT('Ctrl Pts',(-24.3531646875,48.0208333401613,42.1809185638423));
#9156=CARTESIAN_POINT('Ctrl Pts',(-35.6555077526845,47.812500006828,35.6555077526845));
#9157=CARTESIAN_POINT('Ctrl Pts',(-42.1809185638422,47.6041666734946,24.3531646875));
#9158=CARTESIAN_POINT('Ctrl Pts',(-48.706329375,47.3958333401613,13.0508216223155));
#9159=CARTESIAN_POINT('Ctrl Pts',(-48.706329375,47.187500006828,-1.8898197019151E-14));
#9160=CARTESIAN_POINT('Ctrl Pts',(-48.706329375,46.9791666734946,-13.0508216223155));
#9161=CARTESIAN_POINT('Ctrl Pts',(-42.1809185638422,46.7708333401613,-24.3531646875));
#9162=CARTESIAN_POINT('Ctrl Pts',(-35.6555077526845,46.562500006828,-35.6555077526845));
#9163=CARTESIAN_POINT('Ctrl Pts',(-24.3531646875,46.3541666734946,-42.1809185638423));
#9164=CARTESIAN_POINT('Ctrl Pts',(-13.0508216223155,46.1458333401613,-48.706329375));
#9165=CARTESIAN_POINT('Ctrl Pts',(1.59157945007855E-14,45.937500006828,
-48.706329375));
#9166=CARTESIAN_POINT('Ctrl Pts',(13.0508216223155,45.7291666734946,-48.706329375));
#9167=CARTESIAN_POINT('Ctrl Pts',(24.3531646875,45.5208333401613,-42.1809185638422));
#9168=CARTESIAN_POINT('Ctrl Pts',(35.6555077526845,45.312500006828,-35.6555077526845));
#9169=CARTESIAN_POINT('Ctrl Pts',(42.1809185638422,45.1041666734946,-24.3531646875));
#9170=CARTESIAN_POINT('Ctrl Pts',(48.706329375,44.8958333401613,-13.0508216223155));
#9171=CARTESIAN_POINT('Ctrl Pts',(48.706329375,44.687500006828,1.293339198242E-14));
#9172=CARTESIAN_POINT('Ctrl Pts',(48.706329375,44.4791666734946,13.0508216223155));
#9173=CARTESIAN_POINT('Ctrl Pts',(42.1809185638422,44.2708333401613,24.3531646875));
#9174=CARTESIAN_POINT('Ctrl Pts',(35.6555077526845,44.062500006828,35.6555077526845));
#9175=CARTESIAN_POINT('Ctrl Pts',(24.3531646875,43.8541666734946,42.1809185638422));
#9176=CARTESIAN_POINT('Ctrl Pts',(13.0508216223155,43.6458333401613,48.706329375));
#9177=CARTESIAN_POINT('Ctrl Pts',(-9.95098946405443E-15,43.437500006828,
48.706329375));
#9178=CARTESIAN_POINT('Ctrl Pts',(-13.0508216223155,43.2291666734946,48.706329375));
#9179=CARTESIAN_POINT('Ctrl Pts',(-24.3531646875,43.0208333401613,42.1809185638423));
#9180=CARTESIAN_POINT('Ctrl Pts',(-35.6555077526845,42.812500006828,35.6555077526845));
#9181=CARTESIAN_POINT('Ctrl Pts',(-42.1809185638422,42.6041666734946,24.3531646875));
#9182=CARTESIAN_POINT('Ctrl Pts',(-48.706329375,42.3958333401613,13.0508216223155));
#9183=CARTESIAN_POINT('Ctrl Pts',(-48.706329375,42.187500006828,-1.8898197019151E-14));
#9184=CARTESIAN_POINT('Ctrl Pts',(-48.706329375,41.9791666734946,-13.0508216223155));
#9185=CARTESIAN_POINT('Ctrl Pts',(-42.1809185638422,41.7708333401613,-24.3531646875));
#9186=CARTESIAN_POINT('Ctrl Pts',(-35.6555077526845,41.562500006828,-35.6555077526845));
#9187=CARTESIAN_POINT('Ctrl Pts',(-24.3531646875,41.3541666734946,-42.1809185638423));
#9188=CARTESIAN_POINT('Ctrl Pts',(-13.0508216223155,41.1458333401613,-48.706329375));
#9189=CARTESIAN_POINT('Ctrl Pts',(1.59157945007855E-14,40.937500006828,
-48.706329375));
#9190=CARTESIAN_POINT('Ctrl Pts',(13.0508216223155,40.7291666734946,-48.706329375));
#9191=CARTESIAN_POINT('Ctrl Pts',(24.3531646875,40.5208333401613,-42.1809185638422));
#9192=CARTESIAN_POINT('Ctrl Pts',(35.6555077526845,40.312500006828,-35.6555077526845));
#9193=CARTESIAN_POINT('Ctrl Pts',(42.1809185638422,40.1041666734946,-24.3531646875));
#9194=CARTESIAN_POINT('Ctrl Pts',(48.706329375,39.8958333401613,-13.0508216223155));
#9195=CARTESIAN_POINT('Ctrl Pts',(48.706329375,39.687500006828,1.293339198242E-14));
#9196=CARTESIAN_POINT('Ctrl Pts',(48.706329375,39.4791666734946,13.0508216223155));
#9197=CARTESIAN_POINT('Ctrl Pts',(42.1809185638422,39.2708333401613,24.3531646875));
#9198=CARTESIAN_POINT('Ctrl Pts',(35.6555077526845,39.062500006828,35.6555077526845));
#9199=CARTESIAN_POINT('Ctrl Pts',(24.3531646875,38.8541666734946,42.1809185638422));
#9200=CARTESIAN_POINT('Ctrl Pts',(13.0508216223155,38.6458333401613,48.706329375));
#9201=CARTESIAN_POINT('Ctrl Pts',(-9.95098946405443E-15,38.437500006828,
48.706329375));
#9202=CARTESIAN_POINT('Ctrl Pts',(-13.0508216223155,38.2291666734946,48.706329375));
#9203=CARTESIAN_POINT('Ctrl Pts',(-24.3531646875,38.0208333401613,42.1809185638423));
#9204=CARTESIAN_POINT('Ctrl Pts',(-35.6555077526845,37.812500006828,35.6555077526845));
#9205=CARTESIAN_POINT('Ctrl Pts',(-42.1809185638422,37.6041666734946,24.3531646875));
#9206=CARTESIAN_POINT('Ctrl Pts',(-48.706329375,37.3958333401613,13.0508216223155));
#9207=CARTESIAN_POINT('Ctrl Pts',(-48.706329375,37.187500006828,-1.8898197019151E-14));
#9208=CARTESIAN_POINT('Ctrl Pts',(-48.706329375,36.9791666734946,-13.0508216223155));
#9209=CARTESIAN_POINT('Ctrl Pts',(-42.1809185638422,36.7708333401613,-24.3531646875));
#9210=CARTESIAN_POINT('Ctrl Pts',(-35.6555077526845,36.562500006828,-35.6555077526845));
#9211=CARTESIAN_POINT('Ctrl Pts',(-24.3531646875,36.3541666734946,-42.1809185638423));
#9212=CARTESIAN_POINT('Ctrl Pts',(-13.0508216223155,36.1458333401613,-48.706329375));
#9213=CARTESIAN_POINT('Ctrl Pts',(1.59157945007855E-14,35.937500006828,
-48.706329375));
#9214=CARTESIAN_POINT('Ctrl Pts',(13.0508216223155,35.7291666734946,-48.706329375));
#9215=CARTESIAN_POINT('Ctrl Pts',(24.3531646875,35.5208333401613,-42.1809185638422));
#9216=CARTESIAN_POINT('Ctrl Pts',(35.6555077526845,35.312500006828,-35.6555077526845));
#9217=CARTESIAN_POINT('Ctrl Pts',(42.1809185638422,35.1041666734946,-24.3531646875));
#9218=CARTESIAN_POINT('Ctrl Pts',(48.706329375,34.8958333401613,-13.0508216223155));
#9219=CARTESIAN_POINT('Ctrl Pts',(48.706329375,34.687500006828,1.293339198242E-14));
#9220=CARTESIAN_POINT('Ctrl Pts',(48.706329375,34.4791666734946,13.0508216223155));
#9221=CARTESIAN_POINT('Ctrl Pts',(42.1809185638422,34.2708333401613,24.3531646875));
#9222=CARTESIAN_POINT('Ctrl Pts',(35.6555077526845,34.062500006828,35.6555077526845));
#9223=CARTESIAN_POINT('Ctrl Pts',(24.3531646875,33.8541666734946,42.1809185638422));
#9224=CARTESIAN_POINT('Ctrl Pts',(13.0508216223155,33.6458333401613,48.706329375));
#9225=CARTESIAN_POINT('Ctrl Pts',(-9.95098946405443E-15,33.437500006828,
48.706329375));
#9226=CARTESIAN_POINT('Ctrl Pts',(-13.0508216223155,33.2291666734946,48.706329375));
#9227=CARTESIAN_POINT('Ctrl Pts',(-24.3531646875,33.0208333401613,42.1809185638423));
#9228=CARTESIAN_POINT('Ctrl Pts',(-35.6555077526845,32.812500006828,35.6555077526845));
#9229=CARTESIAN_POINT('Ctrl Pts',(-42.1809185638422,32.6041666734946,24.3531646875));
#9230=CARTESIAN_POINT('Ctrl Pts',(-48.706329375,32.3958333401613,13.0508216223155));
#9231=CARTESIAN_POINT('Ctrl Pts',(-48.706329375,32.187500006828,-1.8898197019151E-14));
#9232=CARTESIAN_POINT('Ctrl Pts',(-48.706329375,31.9791666734946,-13.0508216223155));
#9233=CARTESIAN_POINT('Ctrl Pts',(-42.1809185638422,31.7708333401613,-24.3531646875));
#9234=CARTESIAN_POINT('Ctrl Pts',(-35.6555077526845,31.562500006828,-35.6555077526845));
#9235=CARTESIAN_POINT('Ctrl Pts',(-24.3531646875,31.3541666734946,-42.1809185638423));
#9236=CARTESIAN_POINT('Ctrl Pts',(-13.0508216223155,31.1458333401613,-48.706329375));
#9237=CARTESIAN_POINT('Ctrl Pts',(1.59157945007855E-14,30.937500006828,
-48.706329375));
#9238=CARTESIAN_POINT('Ctrl Pts',(13.0508216223155,30.7291666734946,-48.706329375));
#9239=CARTESIAN_POINT('Ctrl Pts',(24.3531646875,30.5208333401613,-42.1809185638422));
#9240=CARTESIAN_POINT('Ctrl Pts',(35.6555077526845,30.312500006828,-35.6555077526845));
#9241=CARTESIAN_POINT('Ctrl Pts',(42.1809185638422,30.1041666734946,-24.3531646875));
#9242=CARTESIAN_POINT('Ctrl Pts',(48.706329375,29.8958333401613,-13.0508216223155));
#9243=CARTESIAN_POINT('Ctrl Pts',(48.706329375,29.687500006828,1.293339198242E-14));
#9244=CARTESIAN_POINT('Ctrl Pts',(48.706329375,29.4791666734946,13.0508216223155));
#9245=CARTESIAN_POINT('Ctrl Pts',(42.1809185638422,29.2708333401613,24.3531646875));
#9246=CARTESIAN_POINT('Ctrl Pts',(35.6555077526845,29.062500006828,35.6555077526845));
#9247=CARTESIAN_POINT('Ctrl Pts',(24.3531646875,28.8541666734946,42.1809185638422));
#9248=CARTESIAN_POINT('Ctrl Pts',(13.0508216223155,28.6458333401613,48.706329375));
#9249=CARTESIAN_POINT('Ctrl Pts',(-9.95098946405443E-15,28.437500006828,
48.706329375));
#9250=CARTESIAN_POINT('Ctrl Pts',(-13.0508216223155,28.2291666734946,48.706329375));
#9251=CARTESIAN_POINT('Ctrl Pts',(-24.3531646875,28.0208333401613,42.1809185638423));
#9252=CARTESIAN_POINT('Ctrl Pts',(-35.6555077526845,27.812500006828,35.6555077526845));
#9253=CARTESIAN_POINT('Ctrl Pts',(-42.1809185638422,27.6041666734946,24.3531646875));
#9254=CARTESIAN_POINT('Ctrl Pts',(-48.706329375,27.3958333401613,13.0508216223155));
#9255=CARTESIAN_POINT('Ctrl Pts',(-48.706329375,27.187500006828,-1.8898197019151E-14));
#9256=CARTESIAN_POINT('',(-48.5134353784345,47.1175463684955,-4.33048599679673));
#9257=CARTESIAN_POINT('Ctrl Pts',(-45.7957082162897,45.5508791552084,-4.33048599679673));
#9258=CARTESIAN_POINT('Ctrl Pts',(-46.027322302781,45.6843839384496,-4.33048599679671));
#9259=CARTESIAN_POINT('Ctrl Pts',(-46.4905476657728,45.9513983799647,-4.33048599679668));
#9260=CARTESIAN_POINT('Ctrl Pts',(-46.9537676533565,46.2184221466352,-4.33048599679674));
#9261=CARTESIAN_POINT('Ctrl Pts',(-47.6280672732222,46.6071316973962,-4.33048599679674));
#9262=CARTESIAN_POINT('Ctrl Pts',(-48.0707534890442,46.8623352807796,-4.33048599679674));
#9263=CARTESIAN_POINT('Ctrl Pts',(-48.5134353784345,47.1175463684955,-4.33048599679673));
#9264=CARTESIAN_POINT('',(-4.32456003949881,46.0073567866782,-48.5139639861634));
#9265=CARTESIAN_POINT('Ctrl Pts',(-48.5134353784345,47.1175463684955,-4.33048599679674));
#9266=CARTESIAN_POINT('Ctrl Pts',(-47.5573898704235,46.9424850907233,-15.0408432190651));
#9267=CARTESIAN_POINT('Ctrl Pts',(-42.1809185638422,46.7708333401613,-24.3531646875));
#9268=CARTESIAN_POINT('Ctrl Pts',(-35.6555077526845,46.562500006828,-35.6555077526845));
#9269=CARTESIAN_POINT('Ctrl Pts',(-24.3531646875,46.3541666734946,-42.1809185638423));
#9270=CARTESIAN_POINT('Ctrl Pts',(-15.0381414154991,46.1824651212465,-47.5589497574396));
#9271=CARTESIAN_POINT('Ctrl Pts',(-4.32456003949881,46.0073567866782,-48.5139639861634));
#9272=CARTESIAN_POINT('Origin',(-4.32455753660831,8017.20454015463,4524.01087370844));
#9273=CARTESIAN_POINT('Ctrl Pts',(-46.,55.6250000136559,0.));
#9274=CARTESIAN_POINT('Ctrl Pts',(-46.,55.4166666803226,-12.3256628518316));
#9275=CARTESIAN_POINT('Ctrl Pts',(-39.8371685740842,55.2083333469893,-23.));
#9276=CARTESIAN_POINT('Ctrl Pts',(-33.6743371481684,55.0000000136559,-33.6743371481684));
#9277=CARTESIAN_POINT('Ctrl Pts',(-23.,54.7916666803226,-39.8371685740842));
#9278=CARTESIAN_POINT('Ctrl Pts',(-12.3256628518317,54.5833333469893,-46.));
#9279=CARTESIAN_POINT('Ctrl Pts',(-2.81668763803891E-15,54.3750000136559,
-46.));
#9280=CARTESIAN_POINT('Ctrl Pts',(12.3256628518316,54.1666666803226,-46.));
#9281=CARTESIAN_POINT('Ctrl Pts',(23.,53.9583333469893,-39.8371685740842));
#9282=CARTESIAN_POINT('Ctrl Pts',(33.6743371481683,53.7500000136559,-33.6743371481684));
#9283=CARTESIAN_POINT('Ctrl Pts',(39.8371685740842,53.5416666803226,-23.));
#9284=CARTESIAN_POINT('Ctrl Pts',(46.,53.3333333469893,-12.3256628518317));
#9285=CARTESIAN_POINT('Ctrl Pts',(46.,53.1250000136559,-5.63337527607782E-15));
#9286=CARTESIAN_POINT('Ctrl Pts',(46.,52.9166666803226,12.3256628518316));
#9287=CARTESIAN_POINT('Ctrl Pts',(39.8371685740842,52.7083333469893,23.));
#9288=CARTESIAN_POINT('Ctrl Pts',(33.6743371481684,52.5000000136559,33.6743371481683));
#9289=CARTESIAN_POINT('Ctrl Pts',(23.,52.2916666803226,39.8371685740842));
#9290=CARTESIAN_POINT('Ctrl Pts',(12.3256628518317,52.0833333469893,46.));
#9291=CARTESIAN_POINT('Ctrl Pts',(8.45006291411674E-15,51.8750000136559,
46.));
#9292=CARTESIAN_POINT('Ctrl Pts',(-12.3256628518316,51.6666666803226,46.));
#9293=CARTESIAN_POINT('Ctrl Pts',(-23.,51.4583333469893,39.8371685740842));
#9294=CARTESIAN_POINT('Ctrl Pts',(-33.6743371481683,51.2500000136559,33.6743371481684));
#9295=CARTESIAN_POINT('Ctrl Pts',(-39.8371685740842,51.0416666803226,23.));
#9296=CARTESIAN_POINT('Ctrl Pts',(-46.,50.8333333469893,12.3256628518317));
#9297=CARTESIAN_POINT('Ctrl Pts',(-46.,50.6250000136559,0.));
#9298=CARTESIAN_POINT('Ctrl Pts',(-46.,50.4166666803226,-12.3256628518316));
#9299=CARTESIAN_POINT('Ctrl Pts',(-39.8371685740842,50.2083333469893,-23.));
#9300=CARTESIAN_POINT('Ctrl Pts',(-33.6743371481684,50.0000000136559,-33.6743371481684));
#9301=CARTESIAN_POINT('Ctrl Pts',(-23.,49.7916666803226,-39.8371685740842));
#9302=CARTESIAN_POINT('Ctrl Pts',(-12.3256628518317,49.5833333469893,-46.));
#9303=CARTESIAN_POINT('Ctrl Pts',(-2.81668763803891E-15,49.3750000136559,
-46.));
#9304=CARTESIAN_POINT('Ctrl Pts',(12.3256628518316,49.1666666803226,-46.));
#9305=CARTESIAN_POINT('Ctrl Pts',(23.,48.9583333469893,-39.8371685740842));
#9306=CARTESIAN_POINT('Ctrl Pts',(33.6743371481683,48.7500000136559,-33.6743371481684));
#9307=CARTESIAN_POINT('Ctrl Pts',(39.8371685740842,48.5416666803226,-23.));
#9308=CARTESIAN_POINT('Ctrl Pts',(46.,48.3333333469893,-12.3256628518317));
#9309=CARTESIAN_POINT('Ctrl Pts',(46.,48.1250000136559,-5.63337527607782E-15));
#9310=CARTESIAN_POINT('Ctrl Pts',(46.,47.9166666803226,12.3256628518316));
#9311=CARTESIAN_POINT('Ctrl Pts',(39.8371685740842,47.7083333469893,23.));
#9312=CARTESIAN_POINT('Ctrl Pts',(33.6743371481684,47.5000000136559,33.6743371481683));
#9313=CARTESIAN_POINT('Ctrl Pts',(23.,47.2916666803226,39.8371685740842));
#9314=CARTESIAN_POINT('Ctrl Pts',(12.3256628518317,47.0833333469893,46.));
#9315=CARTESIAN_POINT('Ctrl Pts',(8.45006291411674E-15,46.8750000136559,
46.));
#9316=CARTESIAN_POINT('Ctrl Pts',(-12.3256628518316,46.6666666803226,46.));
#9317=CARTESIAN_POINT('Ctrl Pts',(-23.,46.4583333469893,39.8371685740842));
#9318=CARTESIAN_POINT('Ctrl Pts',(-33.6743371481683,46.2500000136559,33.6743371481684));
#9319=CARTESIAN_POINT('Ctrl Pts',(-39.8371685740842,46.0416666803226,23.));
#9320=CARTESIAN_POINT('Ctrl Pts',(-46.,45.8333333469892,12.3256628518317));
#9321=CARTESIAN_POINT('Ctrl Pts',(-46.,45.6250000136559,0.));
#9322=CARTESIAN_POINT('Ctrl Pts',(-46.,45.4166666803226,-12.3256628518316));
#9323=CARTESIAN_POINT('Ctrl Pts',(-39.8371685740842,45.2083333469893,-23.));
#9324=CARTESIAN_POINT('Ctrl Pts',(-33.6743371481684,45.0000000136559,-33.6743371481684));
#9325=CARTESIAN_POINT('Ctrl Pts',(-23.,44.7916666803226,-39.8371685740842));
#9326=CARTESIAN_POINT('Ctrl Pts',(-12.3256628518317,44.5833333469893,-46.));
#9327=CARTESIAN_POINT('Ctrl Pts',(-2.81668763803891E-15,44.3750000136559,
-46.));
#9328=CARTESIAN_POINT('Ctrl Pts',(12.3256628518316,44.1666666803226,-46.));
#9329=CARTESIAN_POINT('Ctrl Pts',(23.,43.9583333469893,-39.8371685740842));
#9330=CARTESIAN_POINT('Ctrl Pts',(33.6743371481683,43.7500000136559,-33.6743371481684));
#9331=CARTESIAN_POINT('Ctrl Pts',(39.8371685740842,43.5416666803226,-23.));
#9332=CARTESIAN_POINT('Ctrl Pts',(46.,43.3333333469893,-12.3256628518317));
#9333=CARTESIAN_POINT('Ctrl Pts',(46.,43.1250000136559,-5.63337527607782E-15));
#9334=CARTESIAN_POINT('Ctrl Pts',(46.,42.9166666803226,12.3256628518316));
#9335=CARTESIAN_POINT('Ctrl Pts',(39.8371685740842,42.7083333469893,23.));
#9336=CARTESIAN_POINT('Ctrl Pts',(33.6743371481684,42.5000000136559,33.6743371481683));
#9337=CARTESIAN_POINT('Ctrl Pts',(23.,42.2916666803226,39.8371685740842));
#9338=CARTESIAN_POINT('Ctrl Pts',(12.3256628518317,42.0833333469893,46.));
#9339=CARTESIAN_POINT('Ctrl Pts',(8.45006291411674E-15,41.8750000136559,
46.));
#9340=CARTESIAN_POINT('Ctrl Pts',(-12.3256628518316,41.6666666803226,46.));
#9341=CARTESIAN_POINT('Ctrl Pts',(-23.,41.4583333469893,39.8371685740842));
#9342=CARTESIAN_POINT('Ctrl Pts',(-33.6743371481683,41.2500000136559,33.6743371481684));
#9343=CARTESIAN_POINT('Ctrl Pts',(-39.8371685740842,41.0416666803226,23.));
#9344=CARTESIAN_POINT('Ctrl Pts',(-46.,40.8333333469893,12.3256628518317));
#9345=CARTESIAN_POINT('Ctrl Pts',(-46.,40.6250000136559,0.));
#9346=CARTESIAN_POINT('Ctrl Pts',(-46.,40.4166666803226,-12.3256628518316));
#9347=CARTESIAN_POINT('Ctrl Pts',(-39.8371685740842,40.2083333469893,-23.));
#9348=CARTESIAN_POINT('Ctrl Pts',(-33.6743371481684,40.0000000136559,-33.6743371481684));
#9349=CARTESIAN_POINT('Ctrl Pts',(-23.,39.7916666803226,-39.8371685740842));
#9350=CARTESIAN_POINT('Ctrl Pts',(-12.3256628518317,39.5833333469893,-46.));
#9351=CARTESIAN_POINT('Ctrl Pts',(-2.81668763803891E-15,39.3750000136559,
-46.));
#9352=CARTESIAN_POINT('Ctrl Pts',(12.3256628518316,39.1666666803226,-46.));
#9353=CARTESIAN_POINT('Ctrl Pts',(23.,38.9583333469893,-39.8371685740842));
#9354=CARTESIAN_POINT('Ctrl Pts',(33.6743371481683,38.7500000136559,-33.6743371481684));
#9355=CARTESIAN_POINT('Ctrl Pts',(39.8371685740842,38.5416666803226,-23.));
#9356=CARTESIAN_POINT('Ctrl Pts',(46.,38.3333333469893,-12.3256628518317));
#9357=CARTESIAN_POINT('Ctrl Pts',(46.,38.1250000136559,-5.63337527607782E-15));
#9358=CARTESIAN_POINT('Ctrl Pts',(46.,37.9166666803226,12.3256628518316));
#9359=CARTESIAN_POINT('Ctrl Pts',(39.8371685740842,37.7083333469893,23.));
#9360=CARTESIAN_POINT('Ctrl Pts',(33.6743371481684,37.5000000136559,33.6743371481683));
#9361=CARTESIAN_POINT('Ctrl Pts',(23.,37.2916666803226,39.8371685740842));
#9362=CARTESIAN_POINT('Ctrl Pts',(12.3256628518317,37.0833333469893,46.));
#9363=CARTESIAN_POINT('Ctrl Pts',(8.45006291411674E-15,36.8750000136559,
46.));
#9364=CARTESIAN_POINT('Ctrl Pts',(-12.3256628518316,36.6666666803226,46.));
#9365=CARTESIAN_POINT('Ctrl Pts',(-23.,36.4583333469893,39.8371685740842));
#9366=CARTESIAN_POINT('Ctrl Pts',(-33.6743371481683,36.2500000136559,33.6743371481684));
#9367=CARTESIAN_POINT('Ctrl Pts',(-39.8371685740842,36.0416666803226,23.));
#9368=CARTESIAN_POINT('Ctrl Pts',(-46.,35.8333333469893,12.3256628518317));
#9369=CARTESIAN_POINT('Ctrl Pts',(-46.,35.6250000136559,0.));
#9370=CARTESIAN_POINT('Ctrl Pts',(-46.,35.4166666803226,-12.3256628518316));
#9371=CARTESIAN_POINT('Ctrl Pts',(-39.8371685740842,35.2083333469893,-23.));
#9372=CARTESIAN_POINT('Ctrl Pts',(-33.6743371481684,35.0000000136559,-33.6743371481684));
#9373=CARTESIAN_POINT('Ctrl Pts',(-23.,34.7916666803226,-39.8371685740842));
#9374=CARTESIAN_POINT('Ctrl Pts',(-12.3256628518317,34.5833333469893,-46.));
#9375=CARTESIAN_POINT('Ctrl Pts',(-2.81668763803891E-15,34.3750000136559,
-46.));
#9376=CARTESIAN_POINT('Ctrl Pts',(12.3256628518316,34.1666666803226,-46.));
#9377=CARTESIAN_POINT('Ctrl Pts',(23.,33.9583333469893,-39.8371685740842));
#9378=CARTESIAN_POINT('Ctrl Pts',(33.6743371481683,33.7500000136559,-33.6743371481684));
#9379=CARTESIAN_POINT('Ctrl Pts',(39.8371685740842,33.5416666803226,-23.));
#9380=CARTESIAN_POINT('Ctrl Pts',(46.,33.3333333469893,-12.3256628518317));
#9381=CARTESIAN_POINT('Ctrl Pts',(46.,33.1250000136559,-5.63337527607782E-15));
#9382=CARTESIAN_POINT('Ctrl Pts',(46.,32.9166666803226,12.3256628518316));
#9383=CARTESIAN_POINT('Ctrl Pts',(39.8371685740842,32.7083333469893,23.));
#9384=CARTESIAN_POINT('Ctrl Pts',(33.6743371481684,32.5000000136559,33.6743371481683));
#9385=CARTESIAN_POINT('Ctrl Pts',(23.,32.2916666803226,39.8371685740842));
#9386=CARTESIAN_POINT('Ctrl Pts',(12.3256628518317,32.0833333469893,46.));
#9387=CARTESIAN_POINT('Ctrl Pts',(8.45006291411674E-15,31.8750000136559,
46.));
#9388=CARTESIAN_POINT('Ctrl Pts',(-12.3256628518316,31.6666666803226,46.));
#9389=CARTESIAN_POINT('Ctrl Pts',(-23.,31.4583333469893,39.8371685740842));
#9390=CARTESIAN_POINT('Ctrl Pts',(-33.6743371481683,31.2500000136559,33.6743371481684));
#9391=CARTESIAN_POINT('Ctrl Pts',(-39.8371685740842,31.0416666803226,23.));
#9392=CARTESIAN_POINT('Ctrl Pts',(-46.,30.8333333469893,12.3256628518317));
#9393=CARTESIAN_POINT('Ctrl Pts',(-46.,30.6250000136559,0.));
#9394=CARTESIAN_POINT('Ctrl Pts',(-46.,30.4166666803226,-12.3256628518316));
#9395=CARTESIAN_POINT('Ctrl Pts',(-39.8371685740842,30.2083333469893,-23.));
#9396=CARTESIAN_POINT('Ctrl Pts',(-33.6743371481684,30.0000000136559,-33.6743371481684));
#9397=CARTESIAN_POINT('Ctrl Pts',(-23.,29.7916666803226,-39.8371685740842));
#9398=CARTESIAN_POINT('Ctrl Pts',(-12.3256628518317,29.5833333469893,-46.));
#9399=CARTESIAN_POINT('Ctrl Pts',(-2.81668763803891E-15,29.3750000136559,
-46.));
#9400=CARTESIAN_POINT('Ctrl Pts',(12.3256628518316,29.1666666803226,-46.));
#9401=CARTESIAN_POINT('Ctrl Pts',(23.,28.9583333469893,-39.8371685740842));
#9402=CARTESIAN_POINT('Ctrl Pts',(33.6743371481683,28.7500000136559,-33.6743371481684));
#9403=CARTESIAN_POINT('Ctrl Pts',(39.8371685740842,28.5416666803226,-23.));
#9404=CARTESIAN_POINT('Ctrl Pts',(46.,28.3333333469893,-12.3256628518317));
#9405=CARTESIAN_POINT('Ctrl Pts',(46.,28.1250000136559,-5.63337527607782E-15));
#9406=CARTESIAN_POINT('Ctrl Pts',(46.,27.9166666803226,12.3256628518316));
#9407=CARTESIAN_POINT('Ctrl Pts',(39.8371685740842,27.7083333469893,23.));
#9408=CARTESIAN_POINT('Ctrl Pts',(33.6743371481684,27.5000000136559,33.6743371481683));
#9409=CARTESIAN_POINT('Ctrl Pts',(23.,27.2916666803226,39.8371685740842));
#9410=CARTESIAN_POINT('Ctrl Pts',(12.3256628518317,27.0833333469893,46.));
#9411=CARTESIAN_POINT('Ctrl Pts',(8.45006291411674E-15,26.8750000136559,
46.));
#9412=CARTESIAN_POINT('Ctrl Pts',(-12.3256628518316,26.6666666803226,46.));
#9413=CARTESIAN_POINT('Ctrl Pts',(-23.,26.4583333469893,39.8371685740842));
#9414=CARTESIAN_POINT('Ctrl Pts',(-33.6743371481683,26.2500000136559,33.6743371481684));
#9415=CARTESIAN_POINT('Ctrl Pts',(-39.8371685740842,26.0416666803226,23.));
#9416=CARTESIAN_POINT('Ctrl Pts',(-46.,25.8333333469893,12.3256628518317));
#9417=CARTESIAN_POINT('Ctrl Pts',(-46.,25.6250000136559,0.));
#9418=CARTESIAN_POINT('Ctrl Pts',(-48.706329375,57.187500006828,-1.8898197019151E-14));
#9419=CARTESIAN_POINT('Ctrl Pts',(-48.706329375,56.9791666734946,-13.0508216223155));
#9420=CARTESIAN_POINT('Ctrl Pts',(-42.1809185638422,56.7708333401613,-24.3531646875));
#9421=CARTESIAN_POINT('Ctrl Pts',(-35.6555077526845,56.562500006828,-35.6555077526845));
#9422=CARTESIAN_POINT('Ctrl Pts',(-24.3531646875,56.3541666734946,-42.1809185638423));
#9423=CARTESIAN_POINT('Ctrl Pts',(-13.0508216223155,56.1458333401613,-48.706329375));
#9424=CARTESIAN_POINT('Ctrl Pts',(1.59157945007855E-14,55.937500006828,
-48.706329375));
#9425=CARTESIAN_POINT('Ctrl Pts',(13.0508216223155,55.7291666734946,-48.706329375));
#9426=CARTESIAN_POINT('Ctrl Pts',(24.3531646875,55.5208333401613,-42.1809185638422));
#9427=CARTESIAN_POINT('Ctrl Pts',(35.6555077526845,55.312500006828,-35.6555077526845));
#9428=CARTESIAN_POINT('Ctrl Pts',(42.1809185638422,55.1041666734946,-24.3531646875));
#9429=CARTESIAN_POINT('Ctrl Pts',(48.706329375,54.8958333401613,-13.0508216223155));
#9430=CARTESIAN_POINT('Ctrl Pts',(48.706329375,54.687500006828,1.293339198242E-14));
#9431=CARTESIAN_POINT('Ctrl Pts',(48.706329375,54.4791666734946,13.0508216223155));
#9432=CARTESIAN_POINT('Ctrl Pts',(42.1809185638422,54.2708333401613,24.3531646875));
#9433=CARTESIAN_POINT('Ctrl Pts',(35.6555077526845,54.062500006828,35.6555077526845));
#9434=CARTESIAN_POINT('Ctrl Pts',(24.3531646875,53.8541666734946,42.1809185638422));
#9435=CARTESIAN_POINT('Ctrl Pts',(13.0508216223155,53.6458333401613,48.706329375));
#9436=CARTESIAN_POINT('Ctrl Pts',(-9.95098946405443E-15,53.437500006828,
48.706329375));
#9437=CARTESIAN_POINT('Ctrl Pts',(-13.0508216223155,53.2291666734946,48.706329375));
#9438=CARTESIAN_POINT('Ctrl Pts',(-24.3531646875,53.0208333401613,42.1809185638423));
#9439=CARTESIAN_POINT('Ctrl Pts',(-35.6555077526845,52.812500006828,35.6555077526845));
#9440=CARTESIAN_POINT('Ctrl Pts',(-42.1809185638422,52.6041666734946,24.3531646875));
#9441=CARTESIAN_POINT('Ctrl Pts',(-48.706329375,52.3958333401613,13.0508216223155));
#9442=CARTESIAN_POINT('Ctrl Pts',(-48.706329375,52.187500006828,-1.8898197019151E-14));
#9443=CARTESIAN_POINT('Ctrl Pts',(-48.706329375,51.9791666734946,-13.0508216223155));
#9444=CARTESIAN_POINT('Ctrl Pts',(-42.1809185638422,51.7708333401613,-24.3531646875));
#9445=CARTESIAN_POINT('Ctrl Pts',(-35.6555077526845,51.562500006828,-35.6555077526845));
#9446=CARTESIAN_POINT('Ctrl Pts',(-24.3531646875,51.3541666734946,-42.1809185638423));
#9447=CARTESIAN_POINT('Ctrl Pts',(-13.0508216223155,51.1458333401613,-48.706329375));
#9448=CARTESIAN_POINT('Ctrl Pts',(1.59157945007855E-14,50.937500006828,
-48.706329375));
#9449=CARTESIAN_POINT('Ctrl Pts',(13.0508216223155,50.7291666734946,-48.706329375));
#9450=CARTESIAN_POINT('Ctrl Pts',(24.3531646875,50.5208333401613,-42.1809185638422));
#9451=CARTESIAN_POINT('Ctrl Pts',(35.6555077526845,50.312500006828,-35.6555077526845));
#9452=CARTESIAN_POINT('Ctrl Pts',(42.1809185638422,50.1041666734946,-24.3531646875));
#9453=CARTESIAN_POINT('Ctrl Pts',(48.706329375,49.8958333401613,-13.0508216223155));
#9454=CARTESIAN_POINT('Ctrl Pts',(48.706329375,49.687500006828,1.293339198242E-14));
#9455=CARTESIAN_POINT('Ctrl Pts',(48.706329375,49.4791666734946,13.0508216223155));
#9456=CARTESIAN_POINT('Ctrl Pts',(42.1809185638422,49.2708333401613,24.3531646875));
#9457=CARTESIAN_POINT('Ctrl Pts',(35.6555077526845,49.062500006828,35.6555077526845));
#9458=CARTESIAN_POINT('Ctrl Pts',(24.3531646875,48.8541666734946,42.1809185638422));
#9459=CARTESIAN_POINT('Ctrl Pts',(13.0508216223155,48.6458333401613,48.706329375));
#9460=CARTESIAN_POINT('Ctrl Pts',(-9.95098946405443E-15,48.437500006828,
48.706329375));
#9461=CARTESIAN_POINT('Ctrl Pts',(-13.0508216223155,48.2291666734946,48.706329375));
#9462=CARTESIAN_POINT('Ctrl Pts',(-24.3531646875,48.0208333401613,42.1809185638423));
#9463=CARTESIAN_POINT('Ctrl Pts',(-35.6555077526845,47.812500006828,35.6555077526845));
#9464=CARTESIAN_POINT('Ctrl Pts',(-42.1809185638422,47.6041666734946,24.3531646875));
#9465=CARTESIAN_POINT('Ctrl Pts',(-48.706329375,47.3958333401613,13.0508216223155));
#9466=CARTESIAN_POINT('Ctrl Pts',(-48.706329375,47.187500006828,-1.8898197019151E-14));
#9467=CARTESIAN_POINT('Ctrl Pts',(-48.706329375,46.9791666734946,-13.0508216223155));
#9468=CARTESIAN_POINT('Ctrl Pts',(-42.1809185638422,46.7708333401613,-24.3531646875));
#9469=CARTESIAN_POINT('Ctrl Pts',(-35.6555077526845,46.562500006828,-35.6555077526845));
#9470=CARTESIAN_POINT('Ctrl Pts',(-24.3531646875,46.3541666734946,-42.1809185638423));
#9471=CARTESIAN_POINT('Ctrl Pts',(-13.0508216223155,46.1458333401613,-48.706329375));
#9472=CARTESIAN_POINT('Ctrl Pts',(1.59157945007855E-14,45.937500006828,
-48.706329375));
#9473=CARTESIAN_POINT('Ctrl Pts',(13.0508216223155,45.7291666734946,-48.706329375));
#9474=CARTESIAN_POINT('Ctrl Pts',(24.3531646875,45.5208333401613,-42.1809185638422));
#9475=CARTESIAN_POINT('Ctrl Pts',(35.6555077526845,45.312500006828,-35.6555077526845));
#9476=CARTESIAN_POINT('Ctrl Pts',(42.1809185638422,45.1041666734946,-24.3531646875));
#9477=CARTESIAN_POINT('Ctrl Pts',(48.706329375,44.8958333401613,-13.0508216223155));
#9478=CARTESIAN_POINT('Ctrl Pts',(48.706329375,44.687500006828,1.293339198242E-14));
#9479=CARTESIAN_POINT('Ctrl Pts',(48.706329375,44.4791666734946,13.0508216223155));
#9480=CARTESIAN_POINT('Ctrl Pts',(42.1809185638422,44.2708333401613,24.3531646875));
#9481=CARTESIAN_POINT('Ctrl Pts',(35.6555077526845,44.062500006828,35.6555077526845));
#9482=CARTESIAN_POINT('Ctrl Pts',(24.3531646875,43.8541666734946,42.1809185638422));
#9483=CARTESIAN_POINT('Ctrl Pts',(13.0508216223155,43.6458333401613,48.706329375));
#9484=CARTESIAN_POINT('Ctrl Pts',(-9.95098946405443E-15,43.437500006828,
48.706329375));
#9485=CARTESIAN_POINT('Ctrl Pts',(-13.0508216223155,43.2291666734946,48.706329375));
#9486=CARTESIAN_POINT('Ctrl Pts',(-24.3531646875,43.0208333401613,42.1809185638423));
#9487=CARTESIAN_POINT('Ctrl Pts',(-35.6555077526845,42.812500006828,35.6555077526845));
#9488=CARTESIAN_POINT('Ctrl Pts',(-42.1809185638422,42.6041666734946,24.3531646875));
#9489=CARTESIAN_POINT('Ctrl Pts',(-48.706329375,42.3958333401613,13.0508216223155));
#9490=CARTESIAN_POINT('Ctrl Pts',(-48.706329375,42.187500006828,-1.8898197019151E-14));
#9491=CARTESIAN_POINT('Ctrl Pts',(-48.706329375,41.9791666734946,-13.0508216223155));
#9492=CARTESIAN_POINT('Ctrl Pts',(-42.1809185638422,41.7708333401613,-24.3531646875));
#9493=CARTESIAN_POINT('Ctrl Pts',(-35.6555077526845,41.562500006828,-35.6555077526845));
#9494=CARTESIAN_POINT('Ctrl Pts',(-24.3531646875,41.3541666734946,-42.1809185638423));
#9495=CARTESIAN_POINT('Ctrl Pts',(-13.0508216223155,41.1458333401613,-48.706329375));
#9496=CARTESIAN_POINT('Ctrl Pts',(1.59157945007855E-14,40.937500006828,
-48.706329375));
#9497=CARTESIAN_POINT('Ctrl Pts',(13.0508216223155,40.7291666734946,-48.706329375));
#9498=CARTESIAN_POINT('Ctrl Pts',(24.3531646875,40.5208333401613,-42.1809185638422));
#9499=CARTESIAN_POINT('Ctrl Pts',(35.6555077526845,40.312500006828,-35.6555077526845));
#9500=CARTESIAN_POINT('Ctrl Pts',(42.1809185638422,40.1041666734946,-24.3531646875));
#9501=CARTESIAN_POINT('Ctrl Pts',(48.706329375,39.8958333401613,-13.0508216223155));
#9502=CARTESIAN_POINT('Ctrl Pts',(48.706329375,39.687500006828,1.293339198242E-14));
#9503=CARTESIAN_POINT('Ctrl Pts',(48.706329375,39.4791666734946,13.0508216223155));
#9504=CARTESIAN_POINT('Ctrl Pts',(42.1809185638422,39.2708333401613,24.3531646875));
#9505=CARTESIAN_POINT('Ctrl Pts',(35.6555077526845,39.062500006828,35.6555077526845));
#9506=CARTESIAN_POINT('Ctrl Pts',(24.3531646875,38.8541666734946,42.1809185638422));
#9507=CARTESIAN_POINT('Ctrl Pts',(13.0508216223155,38.6458333401613,48.706329375));
#9508=CARTESIAN_POINT('Ctrl Pts',(-9.95098946405443E-15,38.437500006828,
48.706329375));
#9509=CARTESIAN_POINT('Ctrl Pts',(-13.0508216223155,38.2291666734946,48.706329375));
#9510=CARTESIAN_POINT('Ctrl Pts',(-24.3531646875,38.0208333401613,42.1809185638423));
#9511=CARTESIAN_POINT('Ctrl Pts',(-35.6555077526845,37.812500006828,35.6555077526845));
#9512=CARTESIAN_POINT('Ctrl Pts',(-42.1809185638422,37.6041666734946,24.3531646875));
#9513=CARTESIAN_POINT('Ctrl Pts',(-48.706329375,37.3958333401613,13.0508216223155));
#9514=CARTESIAN_POINT('Ctrl Pts',(-48.706329375,37.187500006828,-1.8898197019151E-14));
#9515=CARTESIAN_POINT('Ctrl Pts',(-48.706329375,36.9791666734946,-13.0508216223155));
#9516=CARTESIAN_POINT('Ctrl Pts',(-42.1809185638422,36.7708333401613,-24.3531646875));
#9517=CARTESIAN_POINT('Ctrl Pts',(-35.6555077526845,36.562500006828,-35.6555077526845));
#9518=CARTESIAN_POINT('Ctrl Pts',(-24.3531646875,36.3541666734946,-42.1809185638423));
#9519=CARTESIAN_POINT('Ctrl Pts',(-13.0508216223155,36.1458333401613,-48.706329375));
#9520=CARTESIAN_POINT('Ctrl Pts',(1.59157945007855E-14,35.937500006828,
-48.706329375));
#9521=CARTESIAN_POINT('Ctrl Pts',(13.0508216223155,35.7291666734946,-48.706329375));
#9522=CARTESIAN_POINT('Ctrl Pts',(24.3531646875,35.5208333401613,-42.1809185638422));
#9523=CARTESIAN_POINT('Ctrl Pts',(35.6555077526845,35.312500006828,-35.6555077526845));
#9524=CARTESIAN_POINT('Ctrl Pts',(42.1809185638422,35.1041666734946,-24.3531646875));
#9525=CARTESIAN_POINT('Ctrl Pts',(48.706329375,34.8958333401613,-13.0508216223155));
#9526=CARTESIAN_POINT('Ctrl Pts',(48.706329375,34.687500006828,1.293339198242E-14));
#9527=CARTESIAN_POINT('Ctrl Pts',(48.706329375,34.4791666734946,13.0508216223155));
#9528=CARTESIAN_POINT('Ctrl Pts',(42.1809185638422,34.2708333401613,24.3531646875));
#9529=CARTESIAN_POINT('Ctrl Pts',(35.6555077526845,34.062500006828,35.6555077526845));
#9530=CARTESIAN_POINT('Ctrl Pts',(24.3531646875,33.8541666734946,42.1809185638422));
#9531=CARTESIAN_POINT('Ctrl Pts',(13.0508216223155,33.6458333401613,48.706329375));
#9532=CARTESIAN_POINT('Ctrl Pts',(-9.95098946405443E-15,33.437500006828,
48.706329375));
#9533=CARTESIAN_POINT('Ctrl Pts',(-13.0508216223155,33.2291666734946,48.706329375));
#9534=CARTESIAN_POINT('Ctrl Pts',(-24.3531646875,33.0208333401613,42.1809185638423));
#9535=CARTESIAN_POINT('Ctrl Pts',(-35.6555077526845,32.812500006828,35.6555077526845));
#9536=CARTESIAN_POINT('Ctrl Pts',(-42.1809185638422,32.6041666734946,24.3531646875));
#9537=CARTESIAN_POINT('Ctrl Pts',(-48.706329375,32.3958333401613,13.0508216223155));
#9538=CARTESIAN_POINT('Ctrl Pts',(-48.706329375,32.187500006828,-1.8898197019151E-14));
#9539=CARTESIAN_POINT('Ctrl Pts',(-48.706329375,31.9791666734946,-13.0508216223155));
#9540=CARTESIAN_POINT('Ctrl Pts',(-42.1809185638422,31.7708333401613,-24.3531646875));
#9541=CARTESIAN_POINT('Ctrl Pts',(-35.6555077526845,31.562500006828,-35.6555077526845));
#9542=CARTESIAN_POINT('Ctrl Pts',(-24.3531646875,31.3541666734946,-42.1809185638423));
#9543=CARTESIAN_POINT('Ctrl Pts',(-13.0508216223155,31.1458333401613,-48.706329375));
#9544=CARTESIAN_POINT('Ctrl Pts',(1.59157945007855E-14,30.937500006828,
-48.706329375));
#9545=CARTESIAN_POINT('Ctrl Pts',(13.0508216223155,30.7291666734946,-48.706329375));
#9546=CARTESIAN_POINT('Ctrl Pts',(24.3531646875,30.5208333401613,-42.1809185638422));
#9547=CARTESIAN_POINT('Ctrl Pts',(35.6555077526845,30.312500006828,-35.6555077526845));
#9548=CARTESIAN_POINT('Ctrl Pts',(42.1809185638422,30.1041666734946,-24.3531646875));
#9549=CARTESIAN_POINT('Ctrl Pts',(48.706329375,29.8958333401613,-13.0508216223155));
#9550=CARTESIAN_POINT('Ctrl Pts',(48.706329375,29.687500006828,1.293339198242E-14));
#9551=CARTESIAN_POINT('Ctrl Pts',(48.706329375,29.4791666734946,13.0508216223155));
#9552=CARTESIAN_POINT('Ctrl Pts',(42.1809185638422,29.2708333401613,24.3531646875));
#9553=CARTESIAN_POINT('Ctrl Pts',(35.6555077526845,29.062500006828,35.6555077526845));
#9554=CARTESIAN_POINT('Ctrl Pts',(24.3531646875,28.8541666734946,42.1809185638422));
#9555=CARTESIAN_POINT('Ctrl Pts',(13.0508216223155,28.6458333401613,48.706329375));
#9556=CARTESIAN_POINT('Ctrl Pts',(-9.95098946405443E-15,28.437500006828,
48.706329375));
#9557=CARTESIAN_POINT('Ctrl Pts',(-13.0508216223155,28.2291666734946,48.706329375));
#9558=CARTESIAN_POINT('Ctrl Pts',(-24.3531646875,28.0208333401613,42.1809185638423));
#9559=CARTESIAN_POINT('Ctrl Pts',(-35.6555077526845,27.812500006828,35.6555077526845));
#9560=CARTESIAN_POINT('Ctrl Pts',(-42.1809185638422,27.6041666734946,24.3531646875));
#9561=CARTESIAN_POINT('Ctrl Pts',(-48.706329375,27.3958333401613,13.0508216223155));
#9562=CARTESIAN_POINT('Ctrl Pts',(-48.706329375,27.187500006828,-1.8898197019151E-14));
#9563=CARTESIAN_POINT('',(-4.32456003949883,48.3676432269777,48.5139639861634));
#9564=CARTESIAN_POINT('',(-48.5725845633798,47.2456516907297,3.60701400320326));
#9565=CARTESIAN_POINT('Ctrl Pts',(-4.32456003949883,48.3676432269777,48.5139639861634));
#9566=CARTESIAN_POINT('Ctrl Pts',(-15.0381414154991,48.1925348924095,47.5589497574396));
#9567=CARTESIAN_POINT('Ctrl Pts',(-24.3531646875,48.0208333401613,42.1809185638423));
#9568=CARTESIAN_POINT('Ctrl Pts',(-35.6555077526845,47.812500006828,35.6555077526845));
#9569=CARTESIAN_POINT('Ctrl Pts',(-42.1809185638422,47.6041666734946,24.3531646875));
#9570=CARTESIAN_POINT('Ctrl Pts',(-47.7480251419552,47.4264286116308,14.7106532430575));
#9571=CARTESIAN_POINT('Ctrl Pts',(-48.5725845633798,47.2456516907297,3.60701400320326));
#9572=CARTESIAN_POINT('Ctrl Pts',(-48.5725845633798,47.2456516907297,3.60701400320326));
#9573=CARTESIAN_POINT('Ctrl Pts',(-48.3407853679392,47.1124685639422,3.60701400320326));
#9574=CARTESIAN_POINT('Ctrl Pts',(-48.1089821836664,46.9792923792741,3.60701400320326));
#9575=CARTESIAN_POINT('Ctrl Pts',(-47.6453674864979,46.7129545080418,3.60701400320326));
#9576=CARTESIAN_POINT('Ctrl Pts',(-47.4135559734253,46.5797928212585,3.60701400320325));
#9577=CARTESIAN_POINT('Ctrl Pts',(-47.1817401099609,46.4466387085919,3.60701400320325));
#9578=CARTESIAN_POINT('Ctrl Pts',(-46.7406305897488,46.1932671494809,3.60701400320325));
#9579=CARTESIAN_POINT('Ctrl Pts',(-46.2995053259033,45.9399229970588,3.60701400320326));
#9580=CARTESIAN_POINT('Ctrl Pts',(-45.858362923034,45.686608693912,3.60701400320327));
#9581=CARTESIAN_POINT('Ctrl Pts',(-4.32456003949882,46.8009818542622,45.7962681936506));
#9582=CARTESIAN_POINT('Ctrl Pts',(-4.32456003949882,46.9344874667937,46.0278818021281));
#9583=CARTESIAN_POINT('Ctrl Pts',(-4.32456003949869,47.2015035419424,46.4911062234486));
#9584=CARTESIAN_POINT('Ctrl Pts',(-4.32456003949883,47.4685288945405,46.954325296818));
#9585=CARTESIAN_POINT('Ctrl Pts',(-4.32456003949883,47.8572357107336,47.6286149142205));
#9586=CARTESIAN_POINT('Ctrl Pts',(-4.32456003949883,48.1124357360102,48.0712916022845));
#9587=CARTESIAN_POINT('Ctrl Pts',(-4.32456003949883,48.3676432269777,48.5139639861634));
#9588=CARTESIAN_POINT('Ctrl Pts',(-46.,55.6250000136559,0.));
#9589=CARTESIAN_POINT('Ctrl Pts',(-46.,55.4166666803226,-12.3256628518316));
#9590=CARTESIAN_POINT('Ctrl Pts',(-39.8371685740842,55.2083333469893,-23.));
#9591=CARTESIAN_POINT('Ctrl Pts',(-33.6743371481684,55.0000000136559,-33.6743371481684));
#9592=CARTESIAN_POINT('Ctrl Pts',(-23.,54.7916666803226,-39.8371685740842));
#9593=CARTESIAN_POINT('Ctrl Pts',(-12.3256628518317,54.5833333469893,-46.));
#9594=CARTESIAN_POINT('Ctrl Pts',(-2.81668763803891E-15,54.3750000136559,
-46.));
#9595=CARTESIAN_POINT('Ctrl Pts',(12.3256628518316,54.1666666803226,-46.));
#9596=CARTESIAN_POINT('Ctrl Pts',(23.,53.9583333469893,-39.8371685740842));
#9597=CARTESIAN_POINT('Ctrl Pts',(33.6743371481683,53.7500000136559,-33.6743371481684));
#9598=CARTESIAN_POINT('Ctrl Pts',(39.8371685740842,53.5416666803226,-23.));
#9599=CARTESIAN_POINT('Ctrl Pts',(46.,53.3333333469893,-12.3256628518317));
#9600=CARTESIAN_POINT('Ctrl Pts',(46.,53.1250000136559,-5.63337527607782E-15));
#9601=CARTESIAN_POINT('Ctrl Pts',(46.,52.9166666803226,12.3256628518316));
#9602=CARTESIAN_POINT('Ctrl Pts',(39.8371685740842,52.7083333469893,23.));
#9603=CARTESIAN_POINT('Ctrl Pts',(33.6743371481684,52.5000000136559,33.6743371481683));
#9604=CARTESIAN_POINT('Ctrl Pts',(23.,52.2916666803226,39.8371685740842));
#9605=CARTESIAN_POINT('Ctrl Pts',(12.3256628518317,52.0833333469893,46.));
#9606=CARTESIAN_POINT('Ctrl Pts',(8.45006291411674E-15,51.8750000136559,
46.));
#9607=CARTESIAN_POINT('Ctrl Pts',(-12.3256628518316,51.6666666803226,46.));
#9608=CARTESIAN_POINT('Ctrl Pts',(-23.,51.4583333469893,39.8371685740842));
#9609=CARTESIAN_POINT('Ctrl Pts',(-33.6743371481683,51.2500000136559,33.6743371481684));
#9610=CARTESIAN_POINT('Ctrl Pts',(-39.8371685740842,51.0416666803226,23.));
#9611=CARTESIAN_POINT('Ctrl Pts',(-46.,50.8333333469893,12.3256628518317));
#9612=CARTESIAN_POINT('Ctrl Pts',(-46.,50.6250000136559,0.));
#9613=CARTESIAN_POINT('Ctrl Pts',(-46.,50.4166666803226,-12.3256628518316));
#9614=CARTESIAN_POINT('Ctrl Pts',(-39.8371685740842,50.2083333469893,-23.));
#9615=CARTESIAN_POINT('Ctrl Pts',(-33.6743371481684,50.0000000136559,-33.6743371481684));
#9616=CARTESIAN_POINT('Ctrl Pts',(-23.,49.7916666803226,-39.8371685740842));
#9617=CARTESIAN_POINT('Ctrl Pts',(-12.3256628518317,49.5833333469893,-46.));
#9618=CARTESIAN_POINT('Ctrl Pts',(-2.81668763803891E-15,49.3750000136559,
-46.));
#9619=CARTESIAN_POINT('Ctrl Pts',(12.3256628518316,49.1666666803226,-46.));
#9620=CARTESIAN_POINT('Ctrl Pts',(23.,48.9583333469893,-39.8371685740842));
#9621=CARTESIAN_POINT('Ctrl Pts',(33.6743371481683,48.7500000136559,-33.6743371481684));
#9622=CARTESIAN_POINT('Ctrl Pts',(39.8371685740842,48.5416666803226,-23.));
#9623=CARTESIAN_POINT('Ctrl Pts',(46.,48.3333333469893,-12.3256628518317));
#9624=CARTESIAN_POINT('Ctrl Pts',(46.,48.1250000136559,-5.63337527607782E-15));
#9625=CARTESIAN_POINT('Ctrl Pts',(46.,47.9166666803226,12.3256628518316));
#9626=CARTESIAN_POINT('Ctrl Pts',(39.8371685740842,47.7083333469893,23.));
#9627=CARTESIAN_POINT('Ctrl Pts',(33.6743371481684,47.5000000136559,33.6743371481683));
#9628=CARTESIAN_POINT('Ctrl Pts',(23.,47.2916666803226,39.8371685740842));
#9629=CARTESIAN_POINT('Ctrl Pts',(12.3256628518317,47.0833333469893,46.));
#9630=CARTESIAN_POINT('Ctrl Pts',(8.45006291411674E-15,46.8750000136559,
46.));
#9631=CARTESIAN_POINT('Ctrl Pts',(-12.3256628518316,46.6666666803226,46.));
#9632=CARTESIAN_POINT('Ctrl Pts',(-23.,46.4583333469893,39.8371685740842));
#9633=CARTESIAN_POINT('Ctrl Pts',(-33.6743371481683,46.2500000136559,33.6743371481684));
#9634=CARTESIAN_POINT('Ctrl Pts',(-39.8371685740842,46.0416666803226,23.));
#9635=CARTESIAN_POINT('Ctrl Pts',(-46.,45.8333333469892,12.3256628518317));
#9636=CARTESIAN_POINT('Ctrl Pts',(-46.,45.6250000136559,0.));
#9637=CARTESIAN_POINT('Ctrl Pts',(-46.,45.4166666803226,-12.3256628518316));
#9638=CARTESIAN_POINT('Ctrl Pts',(-39.8371685740842,45.2083333469893,-23.));
#9639=CARTESIAN_POINT('Ctrl Pts',(-33.6743371481684,45.0000000136559,-33.6743371481684));
#9640=CARTESIAN_POINT('Ctrl Pts',(-23.,44.7916666803226,-39.8371685740842));
#9641=CARTESIAN_POINT('Ctrl Pts',(-12.3256628518317,44.5833333469893,-46.));
#9642=CARTESIAN_POINT('Ctrl Pts',(-2.81668763803891E-15,44.3750000136559,
-46.));
#9643=CARTESIAN_POINT('Ctrl Pts',(12.3256628518316,44.1666666803226,-46.));
#9644=CARTESIAN_POINT('Ctrl Pts',(23.,43.9583333469893,-39.8371685740842));
#9645=CARTESIAN_POINT('Ctrl Pts',(33.6743371481683,43.7500000136559,-33.6743371481684));
#9646=CARTESIAN_POINT('Ctrl Pts',(39.8371685740842,43.5416666803226,-23.));
#9647=CARTESIAN_POINT('Ctrl Pts',(46.,43.3333333469893,-12.3256628518317));
#9648=CARTESIAN_POINT('Ctrl Pts',(46.,43.1250000136559,-5.63337527607782E-15));
#9649=CARTESIAN_POINT('Ctrl Pts',(46.,42.9166666803226,12.3256628518316));
#9650=CARTESIAN_POINT('Ctrl Pts',(39.8371685740842,42.7083333469893,23.));
#9651=CARTESIAN_POINT('Ctrl Pts',(33.6743371481684,42.5000000136559,33.6743371481683));
#9652=CARTESIAN_POINT('Ctrl Pts',(23.,42.2916666803226,39.8371685740842));
#9653=CARTESIAN_POINT('Ctrl Pts',(12.3256628518317,42.0833333469893,46.));
#9654=CARTESIAN_POINT('Ctrl Pts',(8.45006291411674E-15,41.8750000136559,
46.));
#9655=CARTESIAN_POINT('Ctrl Pts',(-12.3256628518316,41.6666666803226,46.));
#9656=CARTESIAN_POINT('Ctrl Pts',(-23.,41.4583333469893,39.8371685740842));
#9657=CARTESIAN_POINT('Ctrl Pts',(-33.6743371481683,41.2500000136559,33.6743371481684));
#9658=CARTESIAN_POINT('Ctrl Pts',(-39.8371685740842,41.0416666803226,23.));
#9659=CARTESIAN_POINT('Ctrl Pts',(-46.,40.8333333469893,12.3256628518317));
#9660=CARTESIAN_POINT('Ctrl Pts',(-46.,40.6250000136559,0.));
#9661=CARTESIAN_POINT('Ctrl Pts',(-46.,40.4166666803226,-12.3256628518316));
#9662=CARTESIAN_POINT('Ctrl Pts',(-39.8371685740842,40.2083333469893,-23.));
#9663=CARTESIAN_POINT('Ctrl Pts',(-33.6743371481684,40.0000000136559,-33.6743371481684));
#9664=CARTESIAN_POINT('Ctrl Pts',(-23.,39.7916666803226,-39.8371685740842));
#9665=CARTESIAN_POINT('Ctrl Pts',(-12.3256628518317,39.5833333469893,-46.));
#9666=CARTESIAN_POINT('Ctrl Pts',(-2.81668763803891E-15,39.3750000136559,
-46.));
#9667=CARTESIAN_POINT('Ctrl Pts',(12.3256628518316,39.1666666803226,-46.));
#9668=CARTESIAN_POINT('Ctrl Pts',(23.,38.9583333469893,-39.8371685740842));
#9669=CARTESIAN_POINT('Ctrl Pts',(33.6743371481683,38.7500000136559,-33.6743371481684));
#9670=CARTESIAN_POINT('Ctrl Pts',(39.8371685740842,38.5416666803226,-23.));
#9671=CARTESIAN_POINT('Ctrl Pts',(46.,38.3333333469893,-12.3256628518317));
#9672=CARTESIAN_POINT('Ctrl Pts',(46.,38.1250000136559,-5.63337527607782E-15));
#9673=CARTESIAN_POINT('Ctrl Pts',(46.,37.9166666803226,12.3256628518316));
#9674=CARTESIAN_POINT('Ctrl Pts',(39.8371685740842,37.7083333469893,23.));
#9675=CARTESIAN_POINT('Ctrl Pts',(33.6743371481684,37.5000000136559,33.6743371481683));
#9676=CARTESIAN_POINT('Ctrl Pts',(23.,37.2916666803226,39.8371685740842));
#9677=CARTESIAN_POINT('Ctrl Pts',(12.3256628518317,37.0833333469893,46.));
#9678=CARTESIAN_POINT('Ctrl Pts',(8.45006291411674E-15,36.8750000136559,
46.));
#9679=CARTESIAN_POINT('Ctrl Pts',(-12.3256628518316,36.6666666803226,46.));
#9680=CARTESIAN_POINT('Ctrl Pts',(-23.,36.4583333469893,39.8371685740842));
#9681=CARTESIAN_POINT('Ctrl Pts',(-33.6743371481683,36.2500000136559,33.6743371481684));
#9682=CARTESIAN_POINT('Ctrl Pts',(-39.8371685740842,36.0416666803226,23.));
#9683=CARTESIAN_POINT('Ctrl Pts',(-46.,35.8333333469893,12.3256628518317));
#9684=CARTESIAN_POINT('Ctrl Pts',(-46.,35.6250000136559,0.));
#9685=CARTESIAN_POINT('Ctrl Pts',(-46.,35.4166666803226,-12.3256628518316));
#9686=CARTESIAN_POINT('Ctrl Pts',(-39.8371685740842,35.2083333469893,-23.));
#9687=CARTESIAN_POINT('Ctrl Pts',(-33.6743371481684,35.0000000136559,-33.6743371481684));
#9688=CARTESIAN_POINT('Ctrl Pts',(-23.,34.7916666803226,-39.8371685740842));
#9689=CARTESIAN_POINT('Ctrl Pts',(-12.3256628518317,34.5833333469893,-46.));
#9690=CARTESIAN_POINT('Ctrl Pts',(-2.81668763803891E-15,34.3750000136559,
-46.));
#9691=CARTESIAN_POINT('Ctrl Pts',(12.3256628518316,34.1666666803226,-46.));
#9692=CARTESIAN_POINT('Ctrl Pts',(23.,33.9583333469893,-39.8371685740842));
#9693=CARTESIAN_POINT('Ctrl Pts',(33.6743371481683,33.7500000136559,-33.6743371481684));
#9694=CARTESIAN_POINT('Ctrl Pts',(39.8371685740842,33.5416666803226,-23.));
#9695=CARTESIAN_POINT('Ctrl Pts',(46.,33.3333333469893,-12.3256628518317));
#9696=CARTESIAN_POINT('Ctrl Pts',(46.,33.1250000136559,-5.63337527607782E-15));
#9697=CARTESIAN_POINT('Ctrl Pts',(46.,32.9166666803226,12.3256628518316));
#9698=CARTESIAN_POINT('Ctrl Pts',(39.8371685740842,32.7083333469893,23.));
#9699=CARTESIAN_POINT('Ctrl Pts',(33.6743371481684,32.5000000136559,33.6743371481683));
#9700=CARTESIAN_POINT('Ctrl Pts',(23.,32.2916666803226,39.8371685740842));
#9701=CARTESIAN_POINT('Ctrl Pts',(12.3256628518317,32.0833333469893,46.));
#9702=CARTESIAN_POINT('Ctrl Pts',(8.45006291411674E-15,31.8750000136559,
46.));
#9703=CARTESIAN_POINT('Ctrl Pts',(-12.3256628518316,31.6666666803226,46.));
#9704=CARTESIAN_POINT('Ctrl Pts',(-23.,31.4583333469893,39.8371685740842));
#9705=CARTESIAN_POINT('Ctrl Pts',(-33.6743371481683,31.2500000136559,33.6743371481684));
#9706=CARTESIAN_POINT('Ctrl Pts',(-39.8371685740842,31.0416666803226,23.));
#9707=CARTESIAN_POINT('Ctrl Pts',(-46.,30.8333333469893,12.3256628518317));
#9708=CARTESIAN_POINT('Ctrl Pts',(-46.,30.6250000136559,0.));
#9709=CARTESIAN_POINT('Ctrl Pts',(-46.,30.4166666803226,-12.3256628518316));
#9710=CARTESIAN_POINT('Ctrl Pts',(-39.8371685740842,30.2083333469893,-23.));
#9711=CARTESIAN_POINT('Ctrl Pts',(-33.6743371481684,30.0000000136559,-33.6743371481684));
#9712=CARTESIAN_POINT('Ctrl Pts',(-23.,29.7916666803226,-39.8371685740842));
#9713=CARTESIAN_POINT('Ctrl Pts',(-12.3256628518317,29.5833333469893,-46.));
#9714=CARTESIAN_POINT('Ctrl Pts',(-2.81668763803891E-15,29.3750000136559,
-46.));
#9715=CARTESIAN_POINT('Ctrl Pts',(12.3256628518316,29.1666666803226,-46.));
#9716=CARTESIAN_POINT('Ctrl Pts',(23.,28.9583333469893,-39.8371685740842));
#9717=CARTESIAN_POINT('Ctrl Pts',(33.6743371481683,28.7500000136559,-33.6743371481684));
#9718=CARTESIAN_POINT('Ctrl Pts',(39.8371685740842,28.5416666803226,-23.));
#9719=CARTESIAN_POINT('Ctrl Pts',(46.,28.3333333469893,-12.3256628518317));
#9720=CARTESIAN_POINT('Ctrl Pts',(46.,28.1250000136559,-5.63337527607782E-15));
#9721=CARTESIAN_POINT('Ctrl Pts',(46.,27.9166666803226,12.3256628518316));
#9722=CARTESIAN_POINT('Ctrl Pts',(39.8371685740842,27.7083333469893,23.));
#9723=CARTESIAN_POINT('Ctrl Pts',(33.6743371481684,27.5000000136559,33.6743371481683));
#9724=CARTESIAN_POINT('Ctrl Pts',(23.,27.2916666803226,39.8371685740842));
#9725=CARTESIAN_POINT('Ctrl Pts',(12.3256628518317,27.0833333469893,46.));
#9726=CARTESIAN_POINT('Ctrl Pts',(8.45006291411674E-15,26.8750000136559,
46.));
#9727=CARTESIAN_POINT('Ctrl Pts',(-12.3256628518316,26.6666666803226,46.));
#9728=CARTESIAN_POINT('Ctrl Pts',(-23.,26.4583333469893,39.8371685740842));
#9729=CARTESIAN_POINT('Ctrl Pts',(-33.6743371481683,26.2500000136559,33.6743371481684));
#9730=CARTESIAN_POINT('Ctrl Pts',(-39.8371685740842,26.0416666803226,23.));
#9731=CARTESIAN_POINT('Ctrl Pts',(-46.,25.8333333469893,12.3256628518317));
#9732=CARTESIAN_POINT('Ctrl Pts',(-46.,25.6250000136559,0.));
#9733=CARTESIAN_POINT('Ctrl Pts',(-48.706329375,57.187500006828,-1.8898197019151E-14));
#9734=CARTESIAN_POINT('Ctrl Pts',(-48.706329375,56.9791666734946,-13.0508216223155));
#9735=CARTESIAN_POINT('Ctrl Pts',(-42.1809185638422,56.7708333401613,-24.3531646875));
#9736=CARTESIAN_POINT('Ctrl Pts',(-35.6555077526845,56.562500006828,-35.6555077526845));
#9737=CARTESIAN_POINT('Ctrl Pts',(-24.3531646875,56.3541666734946,-42.1809185638423));
#9738=CARTESIAN_POINT('Ctrl Pts',(-13.0508216223155,56.1458333401613,-48.706329375));
#9739=CARTESIAN_POINT('Ctrl Pts',(1.59157945007855E-14,55.937500006828,
-48.706329375));
#9740=CARTESIAN_POINT('Ctrl Pts',(13.0508216223155,55.7291666734946,-48.706329375));
#9741=CARTESIAN_POINT('Ctrl Pts',(24.3531646875,55.5208333401613,-42.1809185638422));
#9742=CARTESIAN_POINT('Ctrl Pts',(35.6555077526845,55.312500006828,-35.6555077526845));
#9743=CARTESIAN_POINT('Ctrl Pts',(42.1809185638422,55.1041666734946,-24.3531646875));
#9744=CARTESIAN_POINT('Ctrl Pts',(48.706329375,54.8958333401613,-13.0508216223155));
#9745=CARTESIAN_POINT('Ctrl Pts',(48.706329375,54.687500006828,1.293339198242E-14));
#9746=CARTESIAN_POINT('Ctrl Pts',(48.706329375,54.4791666734946,13.0508216223155));
#9747=CARTESIAN_POINT('Ctrl Pts',(42.1809185638422,54.2708333401613,24.3531646875));
#9748=CARTESIAN_POINT('Ctrl Pts',(35.6555077526845,54.062500006828,35.6555077526845));
#9749=CARTESIAN_POINT('Ctrl Pts',(24.3531646875,53.8541666734946,42.1809185638422));
#9750=CARTESIAN_POINT('Ctrl Pts',(13.0508216223155,53.6458333401613,48.706329375));
#9751=CARTESIAN_POINT('Ctrl Pts',(-9.95098946405443E-15,53.437500006828,
48.706329375));
#9752=CARTESIAN_POINT('Ctrl Pts',(-13.0508216223155,53.2291666734946,48.706329375));
#9753=CARTESIAN_POINT('Ctrl Pts',(-24.3531646875,53.0208333401613,42.1809185638423));
#9754=CARTESIAN_POINT('Ctrl Pts',(-35.6555077526845,52.812500006828,35.6555077526845));
#9755=CARTESIAN_POINT('Ctrl Pts',(-42.1809185638422,52.6041666734946,24.3531646875));
#9756=CARTESIAN_POINT('Ctrl Pts',(-48.706329375,52.3958333401613,13.0508216223155));
#9757=CARTESIAN_POINT('Ctrl Pts',(-48.706329375,52.187500006828,-1.8898197019151E-14));
#9758=CARTESIAN_POINT('Ctrl Pts',(-48.706329375,51.9791666734946,-13.0508216223155));
#9759=CARTESIAN_POINT('Ctrl Pts',(-42.1809185638422,51.7708333401613,-24.3531646875));
#9760=CARTESIAN_POINT('Ctrl Pts',(-35.6555077526845,51.562500006828,-35.6555077526845));
#9761=CARTESIAN_POINT('Ctrl Pts',(-24.3531646875,51.3541666734946,-42.1809185638423));
#9762=CARTESIAN_POINT('Ctrl Pts',(-13.0508216223155,51.1458333401613,-48.706329375));
#9763=CARTESIAN_POINT('Ctrl Pts',(1.59157945007855E-14,50.937500006828,
-48.706329375));
#9764=CARTESIAN_POINT('Ctrl Pts',(13.0508216223155,50.7291666734946,-48.706329375));
#9765=CARTESIAN_POINT('Ctrl Pts',(24.3531646875,50.5208333401613,-42.1809185638422));
#9766=CARTESIAN_POINT('Ctrl Pts',(35.6555077526845,50.312500006828,-35.6555077526845));
#9767=CARTESIAN_POINT('Ctrl Pts',(42.1809185638422,50.1041666734946,-24.3531646875));
#9768=CARTESIAN_POINT('Ctrl Pts',(48.706329375,49.8958333401613,-13.0508216223155));
#9769=CARTESIAN_POINT('Ctrl Pts',(48.706329375,49.687500006828,1.293339198242E-14));
#9770=CARTESIAN_POINT('Ctrl Pts',(48.706329375,49.4791666734946,13.0508216223155));
#9771=CARTESIAN_POINT('Ctrl Pts',(42.1809185638422,49.2708333401613,24.3531646875));
#9772=CARTESIAN_POINT('Ctrl Pts',(35.6555077526845,49.062500006828,35.6555077526845));
#9773=CARTESIAN_POINT('Ctrl Pts',(24.3531646875,48.8541666734946,42.1809185638422));
#9774=CARTESIAN_POINT('Ctrl Pts',(13.0508216223155,48.6458333401613,48.706329375));
#9775=CARTESIAN_POINT('Ctrl Pts',(-9.95098946405443E-15,48.437500006828,
48.706329375));
#9776=CARTESIAN_POINT('Ctrl Pts',(-13.0508216223155,48.2291666734946,48.706329375));
#9777=CARTESIAN_POINT('Ctrl Pts',(-24.3531646875,48.0208333401613,42.1809185638423));
#9778=CARTESIAN_POINT('Ctrl Pts',(-35.6555077526845,47.812500006828,35.6555077526845));
#9779=CARTESIAN_POINT('Ctrl Pts',(-42.1809185638422,47.6041666734946,24.3531646875));
#9780=CARTESIAN_POINT('Ctrl Pts',(-48.706329375,47.3958333401613,13.0508216223155));
#9781=CARTESIAN_POINT('Ctrl Pts',(-48.706329375,47.187500006828,-1.8898197019151E-14));
#9782=CARTESIAN_POINT('Ctrl Pts',(-48.706329375,46.9791666734946,-13.0508216223155));
#9783=CARTESIAN_POINT('Ctrl Pts',(-42.1809185638422,46.7708333401613,-24.3531646875));
#9784=CARTESIAN_POINT('Ctrl Pts',(-35.6555077526845,46.562500006828,-35.6555077526845));
#9785=CARTESIAN_POINT('Ctrl Pts',(-24.3531646875,46.3541666734946,-42.1809185638423));
#9786=CARTESIAN_POINT('Ctrl Pts',(-13.0508216223155,46.1458333401613,-48.706329375));
#9787=CARTESIAN_POINT('Ctrl Pts',(1.59157945007855E-14,45.937500006828,
-48.706329375));
#9788=CARTESIAN_POINT('Ctrl Pts',(13.0508216223155,45.7291666734946,-48.706329375));
#9789=CARTESIAN_POINT('Ctrl Pts',(24.3531646875,45.5208333401613,-42.1809185638422));
#9790=CARTESIAN_POINT('Ctrl Pts',(35.6555077526845,45.312500006828,-35.6555077526845));
#9791=CARTESIAN_POINT('Ctrl Pts',(42.1809185638422,45.1041666734946,-24.3531646875));
#9792=CARTESIAN_POINT('Ctrl Pts',(48.706329375,44.8958333401613,-13.0508216223155));
#9793=CARTESIAN_POINT('Ctrl Pts',(48.706329375,44.687500006828,1.293339198242E-14));
#9794=CARTESIAN_POINT('Ctrl Pts',(48.706329375,44.4791666734946,13.0508216223155));
#9795=CARTESIAN_POINT('Ctrl Pts',(42.1809185638422,44.2708333401613,24.3531646875));
#9796=CARTESIAN_POINT('Ctrl Pts',(35.6555077526845,44.062500006828,35.6555077526845));
#9797=CARTESIAN_POINT('Ctrl Pts',(24.3531646875,43.8541666734946,42.1809185638422));
#9798=CARTESIAN_POINT('Ctrl Pts',(13.0508216223155,43.6458333401613,48.706329375));
#9799=CARTESIAN_POINT('Ctrl Pts',(-9.95098946405443E-15,43.437500006828,
48.706329375));
#9800=CARTESIAN_POINT('Ctrl Pts',(-13.0508216223155,43.2291666734946,48.706329375));
#9801=CARTESIAN_POINT('Ctrl Pts',(-24.3531646875,43.0208333401613,42.1809185638423));
#9802=CARTESIAN_POINT('Ctrl Pts',(-35.6555077526845,42.812500006828,35.6555077526845));
#9803=CARTESIAN_POINT('Ctrl Pts',(-42.1809185638422,42.6041666734946,24.3531646875));
#9804=CARTESIAN_POINT('Ctrl Pts',(-48.706329375,42.3958333401613,13.0508216223155));
#9805=CARTESIAN_POINT('Ctrl Pts',(-48.706329375,42.187500006828,-1.8898197019151E-14));
#9806=CARTESIAN_POINT('Ctrl Pts',(-48.706329375,41.9791666734946,-13.0508216223155));
#9807=CARTESIAN_POINT('Ctrl Pts',(-42.1809185638422,41.7708333401613,-24.3531646875));
#9808=CARTESIAN_POINT('Ctrl Pts',(-35.6555077526845,41.562500006828,-35.6555077526845));
#9809=CARTESIAN_POINT('Ctrl Pts',(-24.3531646875,41.3541666734946,-42.1809185638423));
#9810=CARTESIAN_POINT('Ctrl Pts',(-13.0508216223155,41.1458333401613,-48.706329375));
#9811=CARTESIAN_POINT('Ctrl Pts',(1.59157945007855E-14,40.937500006828,
-48.706329375));
#9812=CARTESIAN_POINT('Ctrl Pts',(13.0508216223155,40.7291666734946,-48.706329375));
#9813=CARTESIAN_POINT('Ctrl Pts',(24.3531646875,40.5208333401613,-42.1809185638422));
#9814=CARTESIAN_POINT('Ctrl Pts',(35.6555077526845,40.312500006828,-35.6555077526845));
#9815=CARTESIAN_POINT('Ctrl Pts',(42.1809185638422,40.1041666734946,-24.3531646875));
#9816=CARTESIAN_POINT('Ctrl Pts',(48.706329375,39.8958333401613,-13.0508216223155));
#9817=CARTESIAN_POINT('Ctrl Pts',(48.706329375,39.687500006828,1.293339198242E-14));
#9818=CARTESIAN_POINT('Ctrl Pts',(48.706329375,39.4791666734946,13.0508216223155));
#9819=CARTESIAN_POINT('Ctrl Pts',(42.1809185638422,39.2708333401613,24.3531646875));
#9820=CARTESIAN_POINT('Ctrl Pts',(35.6555077526845,39.062500006828,35.6555077526845));
#9821=CARTESIAN_POINT('Ctrl Pts',(24.3531646875,38.8541666734946,42.1809185638422));
#9822=CARTESIAN_POINT('Ctrl Pts',(13.0508216223155,38.6458333401613,48.706329375));
#9823=CARTESIAN_POINT('Ctrl Pts',(-9.95098946405443E-15,38.437500006828,
48.706329375));
#9824=CARTESIAN_POINT('Ctrl Pts',(-13.0508216223155,38.2291666734946,48.706329375));
#9825=CARTESIAN_POINT('Ctrl Pts',(-24.3531646875,38.0208333401613,42.1809185638423));
#9826=CARTESIAN_POINT('Ctrl Pts',(-35.6555077526845,37.812500006828,35.6555077526845));
#9827=CARTESIAN_POINT('Ctrl Pts',(-42.1809185638422,37.6041666734946,24.3531646875));
#9828=CARTESIAN_POINT('Ctrl Pts',(-48.706329375,37.3958333401613,13.0508216223155));
#9829=CARTESIAN_POINT('Ctrl Pts',(-48.706329375,37.187500006828,-1.8898197019151E-14));
#9830=CARTESIAN_POINT('Ctrl Pts',(-48.706329375,36.9791666734946,-13.0508216223155));
#9831=CARTESIAN_POINT('Ctrl Pts',(-42.1809185638422,36.7708333401613,-24.3531646875));
#9832=CARTESIAN_POINT('Ctrl Pts',(-35.6555077526845,36.562500006828,-35.6555077526845));
#9833=CARTESIAN_POINT('Ctrl Pts',(-24.3531646875,36.3541666734946,-42.1809185638423));
#9834=CARTESIAN_POINT('Ctrl Pts',(-13.0508216223155,36.1458333401613,-48.706329375));
#9835=CARTESIAN_POINT('Ctrl Pts',(1.59157945007855E-14,35.937500006828,
-48.706329375));
#9836=CARTESIAN_POINT('Ctrl Pts',(13.0508216223155,35.7291666734946,-48.706329375));
#9837=CARTESIAN_POINT('Ctrl Pts',(24.3531646875,35.5208333401613,-42.1809185638422));
#9838=CARTESIAN_POINT('Ctrl Pts',(35.6555077526845,35.312500006828,-35.6555077526845));
#9839=CARTESIAN_POINT('Ctrl Pts',(42.1809185638422,35.1041666734946,-24.3531646875));
#9840=CARTESIAN_POINT('Ctrl Pts',(48.706329375,34.8958333401613,-13.0508216223155));
#9841=CARTESIAN_POINT('Ctrl Pts',(48.706329375,34.687500006828,1.293339198242E-14));
#9842=CARTESIAN_POINT('Ctrl Pts',(48.706329375,34.4791666734946,13.0508216223155));
#9843=CARTESIAN_POINT('Ctrl Pts',(42.1809185638422,34.2708333401613,24.3531646875));
#9844=CARTESIAN_POINT('Ctrl Pts',(35.6555077526845,34.062500006828,35.6555077526845));
#9845=CARTESIAN_POINT('Ctrl Pts',(24.3531646875,33.8541666734946,42.1809185638422));
#9846=CARTESIAN_POINT('Ctrl Pts',(13.0508216223155,33.6458333401613,48.706329375));
#9847=CARTESIAN_POINT('Ctrl Pts',(-9.95098946405443E-15,33.437500006828,
48.706329375));
#9848=CARTESIAN_POINT('Ctrl Pts',(-13.0508216223155,33.2291666734946,48.706329375));
#9849=CARTESIAN_POINT('Ctrl Pts',(-24.3531646875,33.0208333401613,42.1809185638423));
#9850=CARTESIAN_POINT('Ctrl Pts',(-35.6555077526845,32.812500006828,35.6555077526845));
#9851=CARTESIAN_POINT('Ctrl Pts',(-42.1809185638422,32.6041666734946,24.3531646875));
#9852=CARTESIAN_POINT('Ctrl Pts',(-48.706329375,32.3958333401613,13.0508216223155));
#9853=CARTESIAN_POINT('Ctrl Pts',(-48.706329375,32.187500006828,-1.8898197019151E-14));
#9854=CARTESIAN_POINT('Ctrl Pts',(-48.706329375,31.9791666734946,-13.0508216223155));
#9855=CARTESIAN_POINT('Ctrl Pts',(-42.1809185638422,31.7708333401613,-24.3531646875));
#9856=CARTESIAN_POINT('Ctrl Pts',(-35.6555077526845,31.562500006828,-35.6555077526845));
#9857=CARTESIAN_POINT('Ctrl Pts',(-24.3531646875,31.3541666734946,-42.1809185638423));
#9858=CARTESIAN_POINT('Ctrl Pts',(-13.0508216223155,31.1458333401613,-48.706329375));
#9859=CARTESIAN_POINT('Ctrl Pts',(1.59157945007855E-14,30.937500006828,
-48.706329375));
#9860=CARTESIAN_POINT('Ctrl Pts',(13.0508216223155,30.7291666734946,-48.706329375));
#9861=CARTESIAN_POINT('Ctrl Pts',(24.3531646875,30.5208333401613,-42.1809185638422));
#9862=CARTESIAN_POINT('Ctrl Pts',(35.6555077526845,30.312500006828,-35.6555077526845));
#9863=CARTESIAN_POINT('Ctrl Pts',(42.1809185638422,30.1041666734946,-24.3531646875));
#9864=CARTESIAN_POINT('Ctrl Pts',(48.706329375,29.8958333401613,-13.0508216223155));
#9865=CARTESIAN_POINT('Ctrl Pts',(48.706329375,29.687500006828,1.293339198242E-14));
#9866=CARTESIAN_POINT('Ctrl Pts',(48.706329375,29.4791666734946,13.0508216223155));
#9867=CARTESIAN_POINT('Ctrl Pts',(42.1809185638422,29.2708333401613,24.3531646875));
#9868=CARTESIAN_POINT('Ctrl Pts',(35.6555077526845,29.062500006828,35.6555077526845));
#9869=CARTESIAN_POINT('Ctrl Pts',(24.3531646875,28.8541666734946,42.1809185638422));
#9870=CARTESIAN_POINT('Ctrl Pts',(13.0508216223155,28.6458333401613,48.706329375));
#9871=CARTESIAN_POINT('Ctrl Pts',(-9.95098946405443E-15,28.437500006828,
48.706329375));
#9872=CARTESIAN_POINT('Ctrl Pts',(-13.0508216223155,28.2291666734946,48.706329375));
#9873=CARTESIAN_POINT('Ctrl Pts',(-24.3531646875,28.0208333401613,42.1809185638423));
#9874=CARTESIAN_POINT('Ctrl Pts',(-35.6555077526845,27.812500006828,35.6555077526845));
#9875=CARTESIAN_POINT('Ctrl Pts',(-42.1809185638422,27.6041666734946,24.3531646875));
#9876=CARTESIAN_POINT('Ctrl Pts',(-48.706329375,27.3958333401613,13.0508216223155));
#9877=CARTESIAN_POINT('Ctrl Pts',(-48.706329375,27.187500006828,-1.8898197019151E-14));
#9878=CARTESIAN_POINT('',(-48.5134353784345,42.1175463684955,-4.33048599679665));
#9879=CARTESIAN_POINT('Ctrl Pts',(-45.7957082162897,40.5508791552084,-4.33048599679673));
#9880=CARTESIAN_POINT('Ctrl Pts',(-46.027322302781,40.6843839384496,-4.33048599679682));
#9881=CARTESIAN_POINT('Ctrl Pts',(-46.4905476657728,40.9513983799648,-4.33048599679661));
#9882=CARTESIAN_POINT('Ctrl Pts',(-46.9537676533565,41.2184221466352,-4.33048599679666));
#9883=CARTESIAN_POINT('Ctrl Pts',(-47.6280672732222,41.6071316973962,-4.33048599679666));
#9884=CARTESIAN_POINT('Ctrl Pts',(-48.0707534890442,41.8623352807796,-4.33048599679665));
#9885=CARTESIAN_POINT('Ctrl Pts',(-48.5134353784345,42.1175463684955,-4.33048599679665));
#9886=CARTESIAN_POINT('',(-4.32456003949873,41.0073567866782,-48.5139639861634));
#9887=CARTESIAN_POINT('Ctrl Pts',(-48.5134353784345,42.1175463684955,-4.33048599679665));
#9888=CARTESIAN_POINT('Ctrl Pts',(-47.5573898704235,41.9424850907233,-15.040843219065));
#9889=CARTESIAN_POINT('Ctrl Pts',(-42.1809185638422,41.7708333401613,-24.3531646875));
#9890=CARTESIAN_POINT('Ctrl Pts',(-35.6555077526845,41.562500006828,-35.6555077526845));
#9891=CARTESIAN_POINT('Ctrl Pts',(-24.3531646875,41.3541666734946,-42.1809185638423));
#9892=CARTESIAN_POINT('Ctrl Pts',(-15.038141415499,41.1824651212465,-47.5589497574396));
#9893=CARTESIAN_POINT('Ctrl Pts',(-4.32456003949873,41.0073567866782,-48.5139639861634));
#9894=CARTESIAN_POINT('Origin',(-4.32456091837631,8012.2045409659,4524.01087410016));
#9895=CARTESIAN_POINT('Ctrl Pts',(-46.,55.6250000136559,0.));
#9896=CARTESIAN_POINT('Ctrl Pts',(-46.,55.4166666803226,-12.3256628518316));
#9897=CARTESIAN_POINT('Ctrl Pts',(-39.8371685740842,55.2083333469893,-23.));
#9898=CARTESIAN_POINT('Ctrl Pts',(-33.6743371481684,55.0000000136559,-33.6743371481684));
#9899=CARTESIAN_POINT('Ctrl Pts',(-23.,54.7916666803226,-39.8371685740842));
#9900=CARTESIAN_POINT('Ctrl Pts',(-12.3256628518317,54.5833333469893,-46.));
#9901=CARTESIAN_POINT('Ctrl Pts',(-2.81668763803891E-15,54.3750000136559,
-46.));
#9902=CARTESIAN_POINT('Ctrl Pts',(12.3256628518316,54.1666666803226,-46.));
#9903=CARTESIAN_POINT('Ctrl Pts',(23.,53.9583333469893,-39.8371685740842));
#9904=CARTESIAN_POINT('Ctrl Pts',(33.6743371481683,53.7500000136559,-33.6743371481684));
#9905=CARTESIAN_POINT('Ctrl Pts',(39.8371685740842,53.5416666803226,-23.));
#9906=CARTESIAN_POINT('Ctrl Pts',(46.,53.3333333469893,-12.3256628518317));
#9907=CARTESIAN_POINT('Ctrl Pts',(46.,53.1250000136559,-5.63337527607782E-15));
#9908=CARTESIAN_POINT('Ctrl Pts',(46.,52.9166666803226,12.3256628518316));
#9909=CARTESIAN_POINT('Ctrl Pts',(39.8371685740842,52.7083333469893,23.));
#9910=CARTESIAN_POINT('Ctrl Pts',(33.6743371481684,52.5000000136559,33.6743371481683));
#9911=CARTESIAN_POINT('Ctrl Pts',(23.,52.2916666803226,39.8371685740842));
#9912=CARTESIAN_POINT('Ctrl Pts',(12.3256628518317,52.0833333469893,46.));
#9913=CARTESIAN_POINT('Ctrl Pts',(8.45006291411674E-15,51.8750000136559,
46.));
#9914=CARTESIAN_POINT('Ctrl Pts',(-12.3256628518316,51.6666666803226,46.));
#9915=CARTESIAN_POINT('Ctrl Pts',(-23.,51.4583333469893,39.8371685740842));
#9916=CARTESIAN_POINT('Ctrl Pts',(-33.6743371481683,51.2500000136559,33.6743371481684));
#9917=CARTESIAN_POINT('Ctrl Pts',(-39.8371685740842,51.0416666803226,23.));
#9918=CARTESIAN_POINT('Ctrl Pts',(-46.,50.8333333469893,12.3256628518317));
#9919=CARTESIAN_POINT('Ctrl Pts',(-46.,50.6250000136559,0.));
#9920=CARTESIAN_POINT('Ctrl Pts',(-46.,50.4166666803226,-12.3256628518316));
#9921=CARTESIAN_POINT('Ctrl Pts',(-39.8371685740842,50.2083333469893,-23.));
#9922=CARTESIAN_POINT('Ctrl Pts',(-33.6743371481684,50.0000000136559,-33.6743371481684));
#9923=CARTESIAN_POINT('Ctrl Pts',(-23.,49.7916666803226,-39.8371685740842));
#9924=CARTESIAN_POINT('Ctrl Pts',(-12.3256628518317,49.5833333469893,-46.));
#9925=CARTESIAN_POINT('Ctrl Pts',(-2.81668763803891E-15,49.3750000136559,
-46.));
#9926=CARTESIAN_POINT('Ctrl Pts',(12.3256628518316,49.1666666803226,-46.));
#9927=CARTESIAN_POINT('Ctrl Pts',(23.,48.9583333469893,-39.8371685740842));
#9928=CARTESIAN_POINT('Ctrl Pts',(33.6743371481683,48.7500000136559,-33.6743371481684));
#9929=CARTESIAN_POINT('Ctrl Pts',(39.8371685740842,48.5416666803226,-23.));
#9930=CARTESIAN_POINT('Ctrl Pts',(46.,48.3333333469893,-12.3256628518317));
#9931=CARTESIAN_POINT('Ctrl Pts',(46.,48.1250000136559,-5.63337527607782E-15));
#9932=CARTESIAN_POINT('Ctrl Pts',(46.,47.9166666803226,12.3256628518316));
#9933=CARTESIAN_POINT('Ctrl Pts',(39.8371685740842,47.7083333469893,23.));
#9934=CARTESIAN_POINT('Ctrl Pts',(33.6743371481684,47.5000000136559,33.6743371481683));
#9935=CARTESIAN_POINT('Ctrl Pts',(23.,47.2916666803226,39.8371685740842));
#9936=CARTESIAN_POINT('Ctrl Pts',(12.3256628518317,47.0833333469893,46.));
#9937=CARTESIAN_POINT('Ctrl Pts',(8.45006291411674E-15,46.8750000136559,
46.));
#9938=CARTESIAN_POINT('Ctrl Pts',(-12.3256628518316,46.6666666803226,46.));
#9939=CARTESIAN_POINT('Ctrl Pts',(-23.,46.4583333469893,39.8371685740842));
#9940=CARTESIAN_POINT('Ctrl Pts',(-33.6743371481683,46.2500000136559,33.6743371481684));
#9941=CARTESIAN_POINT('Ctrl Pts',(-39.8371685740842,46.0416666803226,23.));
#9942=CARTESIAN_POINT('Ctrl Pts',(-46.,45.8333333469892,12.3256628518317));
#9943=CARTESIAN_POINT('Ctrl Pts',(-46.,45.6250000136559,0.));
#9944=CARTESIAN_POINT('Ctrl Pts',(-46.,45.4166666803226,-12.3256628518316));
#9945=CARTESIAN_POINT('Ctrl Pts',(-39.8371685740842,45.2083333469893,-23.));
#9946=CARTESIAN_POINT('Ctrl Pts',(-33.6743371481684,45.0000000136559,-33.6743371481684));
#9947=CARTESIAN_POINT('Ctrl Pts',(-23.,44.7916666803226,-39.8371685740842));
#9948=CARTESIAN_POINT('Ctrl Pts',(-12.3256628518317,44.5833333469893,-46.));
#9949=CARTESIAN_POINT('Ctrl Pts',(-2.81668763803891E-15,44.3750000136559,
-46.));
#9950=CARTESIAN_POINT('Ctrl Pts',(12.3256628518316,44.1666666803226,-46.));
#9951=CARTESIAN_POINT('Ctrl Pts',(23.,43.9583333469893,-39.8371685740842));
#9952=CARTESIAN_POINT('Ctrl Pts',(33.6743371481683,43.7500000136559,-33.6743371481684));
#9953=CARTESIAN_POINT('Ctrl Pts',(39.8371685740842,43.5416666803226,-23.));
#9954=CARTESIAN_POINT('Ctrl Pts',(46.,43.3333333469893,-12.3256628518317));
#9955=CARTESIAN_POINT('Ctrl Pts',(46.,43.1250000136559,-5.63337527607782E-15));
#9956=CARTESIAN_POINT('Ctrl Pts',(46.,42.9166666803226,12.3256628518316));
#9957=CARTESIAN_POINT('Ctrl Pts',(39.8371685740842,42.7083333469893,23.));
#9958=CARTESIAN_POINT('Ctrl Pts',(33.6743371481684,42.5000000136559,33.6743371481683));
#9959=CARTESIAN_POINT('Ctrl Pts',(23.,42.2916666803226,39.8371685740842));
#9960=CARTESIAN_POINT('Ctrl Pts',(12.3256628518317,42.0833333469893,46.));
#9961=CARTESIAN_POINT('Ctrl Pts',(8.45006291411674E-15,41.8750000136559,
46.));
#9962=CARTESIAN_POINT('Ctrl Pts',(-12.3256628518316,41.6666666803226,46.));
#9963=CARTESIAN_POINT('Ctrl Pts',(-23.,41.4583333469893,39.8371685740842));
#9964=CARTESIAN_POINT('Ctrl Pts',(-33.6743371481683,41.2500000136559,33.6743371481684));
#9965=CARTESIAN_POINT('Ctrl Pts',(-39.8371685740842,41.0416666803226,23.));
#9966=CARTESIAN_POINT('Ctrl Pts',(-46.,40.8333333469893,12.3256628518317));
#9967=CARTESIAN_POINT('Ctrl Pts',(-46.,40.6250000136559,0.));
#9968=CARTESIAN_POINT('Ctrl Pts',(-46.,40.4166666803226,-12.3256628518316));
#9969=CARTESIAN_POINT('Ctrl Pts',(-39.8371685740842,40.2083333469893,-23.));
#9970=CARTESIAN_POINT('Ctrl Pts',(-33.6743371481684,40.0000000136559,-33.6743371481684));
#9971=CARTESIAN_POINT('Ctrl Pts',(-23.,39.7916666803226,-39.8371685740842));
#9972=CARTESIAN_POINT('Ctrl Pts',(-12.3256628518317,39.5833333469893,-46.));
#9973=CARTESIAN_POINT('Ctrl Pts',(-2.81668763803891E-15,39.3750000136559,
-46.));
#9974=CARTESIAN_POINT('Ctrl Pts',(12.3256628518316,39.1666666803226,-46.));
#9975=CARTESIAN_POINT('Ctrl Pts',(23.,38.9583333469893,-39.8371685740842));
#9976=CARTESIAN_POINT('Ctrl Pts',(33.6743371481683,38.7500000136559,-33.6743371481684));
#9977=CARTESIAN_POINT('Ctrl Pts',(39.8371685740842,38.5416666803226,-23.));
#9978=CARTESIAN_POINT('Ctrl Pts',(46.,38.3333333469893,-12.3256628518317));
#9979=CARTESIAN_POINT('Ctrl Pts',(46.,38.1250000136559,-5.63337527607782E-15));
#9980=CARTESIAN_POINT('Ctrl Pts',(46.,37.9166666803226,12.3256628518316));
#9981=CARTESIAN_POINT('Ctrl Pts',(39.8371685740842,37.7083333469893,23.));
#9982=CARTESIAN_POINT('Ctrl Pts',(33.6743371481684,37.5000000136559,33.6743371481683));
#9983=CARTESIAN_POINT('Ctrl Pts',(23.,37.2916666803226,39.8371685740842));
#9984=CARTESIAN_POINT('Ctrl Pts',(12.3256628518317,37.0833333469893,46.));
#9985=CARTESIAN_POINT('Ctrl Pts',(8.45006291411674E-15,36.8750000136559,
46.));
#9986=CARTESIAN_POINT('Ctrl Pts',(-12.3256628518316,36.6666666803226,46.));
#9987=CARTESIAN_POINT('Ctrl Pts',(-23.,36.4583333469893,39.8371685740842));
#9988=CARTESIAN_POINT('Ctrl Pts',(-33.6743371481683,36.2500000136559,33.6743371481684));
#9989=CARTESIAN_POINT('Ctrl Pts',(-39.8371685740842,36.0416666803226,23.));
#9990=CARTESIAN_POINT('Ctrl Pts',(-46.,35.8333333469893,12.3256628518317));
#9991=CARTESIAN_POINT('Ctrl Pts',(-46.,35.6250000136559,0.));
#9992=CARTESIAN_POINT('Ctrl Pts',(-46.,35.4166666803226,-12.3256628518316));
#9993=CARTESIAN_POINT('Ctrl Pts',(-39.8371685740842,35.2083333469893,-23.));
#9994=CARTESIAN_POINT('Ctrl Pts',(-33.6743371481684,35.0000000136559,-33.6743371481684));
#9995=CARTESIAN_POINT('Ctrl Pts',(-23.,34.7916666803226,-39.8371685740842));
#9996=CARTESIAN_POINT('Ctrl Pts',(-12.3256628518317,34.5833333469893,-46.));
#9997=CARTESIAN_POINT('Ctrl Pts',(-2.81668763803891E-15,34.3750000136559,
-46.));
#9998=CARTESIAN_POINT('Ctrl Pts',(12.3256628518316,34.1666666803226,-46.));
#9999=CARTESIAN_POINT('Ctrl Pts',(23.,33.9583333469893,-39.8371685740842));
#10000=CARTESIAN_POINT('Ctrl Pts',(33.6743371481683,33.7500000136559,-33.6743371481684));
#10001=CARTESIAN_POINT('Ctrl Pts',(39.8371685740842,33.5416666803226,-23.));
#10002=CARTESIAN_POINT('Ctrl Pts',(46.,33.3333333469893,-12.3256628518317));
#10003=CARTESIAN_POINT('Ctrl Pts',(46.,33.1250000136559,-5.63337527607782E-15));
#10004=CARTESIAN_POINT('Ctrl Pts',(46.,32.9166666803226,12.3256628518316));
#10005=CARTESIAN_POINT('Ctrl Pts',(39.8371685740842,32.7083333469893,23.));
#10006=CARTESIAN_POINT('Ctrl Pts',(33.6743371481684,32.5000000136559,33.6743371481683));
#10007=CARTESIAN_POINT('Ctrl Pts',(23.,32.2916666803226,39.8371685740842));
#10008=CARTESIAN_POINT('Ctrl Pts',(12.3256628518317,32.0833333469893,46.));
#10009=CARTESIAN_POINT('Ctrl Pts',(8.45006291411674E-15,31.8750000136559,
46.));
#10010=CARTESIAN_POINT('Ctrl Pts',(-12.3256628518316,31.6666666803226,46.));
#10011=CARTESIAN_POINT('Ctrl Pts',(-23.,31.4583333469893,39.8371685740842));
#10012=CARTESIAN_POINT('Ctrl Pts',(-33.6743371481683,31.2500000136559,33.6743371481684));
#10013=CARTESIAN_POINT('Ctrl Pts',(-39.8371685740842,31.0416666803226,23.));
#10014=CARTESIAN_POINT('Ctrl Pts',(-46.,30.8333333469893,12.3256628518317));
#10015=CARTESIAN_POINT('Ctrl Pts',(-46.,30.6250000136559,0.));
#10016=CARTESIAN_POINT('Ctrl Pts',(-46.,30.4166666803226,-12.3256628518316));
#10017=CARTESIAN_POINT('Ctrl Pts',(-39.8371685740842,30.2083333469893,-23.));
#10018=CARTESIAN_POINT('Ctrl Pts',(-33.6743371481684,30.0000000136559,-33.6743371481684));
#10019=CARTESIAN_POINT('Ctrl Pts',(-23.,29.7916666803226,-39.8371685740842));
#10020=CARTESIAN_POINT('Ctrl Pts',(-12.3256628518317,29.5833333469893,-46.));
#10021=CARTESIAN_POINT('Ctrl Pts',(-2.81668763803891E-15,29.3750000136559,
-46.));
#10022=CARTESIAN_POINT('Ctrl Pts',(12.3256628518316,29.1666666803226,-46.));
#10023=CARTESIAN_POINT('Ctrl Pts',(23.,28.9583333469893,-39.8371685740842));
#10024=CARTESIAN_POINT('Ctrl Pts',(33.6743371481683,28.7500000136559,-33.6743371481684));
#10025=CARTESIAN_POINT('Ctrl Pts',(39.8371685740842,28.5416666803226,-23.));
#10026=CARTESIAN_POINT('Ctrl Pts',(46.,28.3333333469893,-12.3256628518317));
#10027=CARTESIAN_POINT('Ctrl Pts',(46.,28.1250000136559,-5.63337527607782E-15));
#10028=CARTESIAN_POINT('Ctrl Pts',(46.,27.9166666803226,12.3256628518316));
#10029=CARTESIAN_POINT('Ctrl Pts',(39.8371685740842,27.7083333469893,23.));
#10030=CARTESIAN_POINT('Ctrl Pts',(33.6743371481684,27.5000000136559,33.6743371481683));
#10031=CARTESIAN_POINT('Ctrl Pts',(23.,27.2916666803226,39.8371685740842));
#10032=CARTESIAN_POINT('Ctrl Pts',(12.3256628518317,27.0833333469893,46.));
#10033=CARTESIAN_POINT('Ctrl Pts',(8.45006291411674E-15,26.8750000136559,
46.));
#10034=CARTESIAN_POINT('Ctrl Pts',(-12.3256628518316,26.6666666803226,46.));
#10035=CARTESIAN_POINT('Ctrl Pts',(-23.,26.4583333469893,39.8371685740842));
#10036=CARTESIAN_POINT('Ctrl Pts',(-33.6743371481683,26.2500000136559,33.6743371481684));
#10037=CARTESIAN_POINT('Ctrl Pts',(-39.8371685740842,26.0416666803226,23.));
#10038=CARTESIAN_POINT('Ctrl Pts',(-46.,25.8333333469893,12.3256628518317));
#10039=CARTESIAN_POINT('Ctrl Pts',(-46.,25.6250000136559,0.));
#10040=CARTESIAN_POINT('Ctrl Pts',(-48.706329375,57.187500006828,-1.8898197019151E-14));
#10041=CARTESIAN_POINT('Ctrl Pts',(-48.706329375,56.9791666734946,-13.0508216223155));
#10042=CARTESIAN_POINT('Ctrl Pts',(-42.1809185638422,56.7708333401613,-24.3531646875));
#10043=CARTESIAN_POINT('Ctrl Pts',(-35.6555077526845,56.562500006828,-35.6555077526845));
#10044=CARTESIAN_POINT('Ctrl Pts',(-24.3531646875,56.3541666734946,-42.1809185638423));
#10045=CARTESIAN_POINT('Ctrl Pts',(-13.0508216223155,56.1458333401613,-48.706329375));
#10046=CARTESIAN_POINT('Ctrl Pts',(1.59157945007855E-14,55.937500006828,
-48.706329375));
#10047=CARTESIAN_POINT('Ctrl Pts',(13.0508216223155,55.7291666734946,-48.706329375));
#10048=CARTESIAN_POINT('Ctrl Pts',(24.3531646875,55.5208333401613,-42.1809185638422));
#10049=CARTESIAN_POINT('Ctrl Pts',(35.6555077526845,55.312500006828,-35.6555077526845));
#10050=CARTESIAN_POINT('Ctrl Pts',(42.1809185638422,55.1041666734946,-24.3531646875));
#10051=CARTESIAN_POINT('Ctrl Pts',(48.706329375,54.8958333401613,-13.0508216223155));
#10052=CARTESIAN_POINT('Ctrl Pts',(48.706329375,54.687500006828,1.293339198242E-14));
#10053=CARTESIAN_POINT('Ctrl Pts',(48.706329375,54.4791666734946,13.0508216223155));
#10054=CARTESIAN_POINT('Ctrl Pts',(42.1809185638422,54.2708333401613,24.3531646875));
#10055=CARTESIAN_POINT('Ctrl Pts',(35.6555077526845,54.062500006828,35.6555077526845));
#10056=CARTESIAN_POINT('Ctrl Pts',(24.3531646875,53.8541666734946,42.1809185638422));
#10057=CARTESIAN_POINT('Ctrl Pts',(13.0508216223155,53.6458333401613,48.706329375));
#10058=CARTESIAN_POINT('Ctrl Pts',(-9.95098946405443E-15,53.437500006828,
48.706329375));
#10059=CARTESIAN_POINT('Ctrl Pts',(-13.0508216223155,53.2291666734946,48.706329375));
#10060=CARTESIAN_POINT('Ctrl Pts',(-24.3531646875,53.0208333401613,42.1809185638423));
#10061=CARTESIAN_POINT('Ctrl Pts',(-35.6555077526845,52.812500006828,35.6555077526845));
#10062=CARTESIAN_POINT('Ctrl Pts',(-42.1809185638422,52.6041666734946,24.3531646875));
#10063=CARTESIAN_POINT('Ctrl Pts',(-48.706329375,52.3958333401613,13.0508216223155));
#10064=CARTESIAN_POINT('Ctrl Pts',(-48.706329375,52.187500006828,-1.8898197019151E-14));
#10065=CARTESIAN_POINT('Ctrl Pts',(-48.706329375,51.9791666734946,-13.0508216223155));
#10066=CARTESIAN_POINT('Ctrl Pts',(-42.1809185638422,51.7708333401613,-24.3531646875));
#10067=CARTESIAN_POINT('Ctrl Pts',(-35.6555077526845,51.562500006828,-35.6555077526845));
#10068=CARTESIAN_POINT('Ctrl Pts',(-24.3531646875,51.3541666734946,-42.1809185638423));
#10069=CARTESIAN_POINT('Ctrl Pts',(-13.0508216223155,51.1458333401613,-48.706329375));
#10070=CARTESIAN_POINT('Ctrl Pts',(1.59157945007855E-14,50.937500006828,
-48.706329375));
#10071=CARTESIAN_POINT('Ctrl Pts',(13.0508216223155,50.7291666734946,-48.706329375));
#10072=CARTESIAN_POINT('Ctrl Pts',(24.3531646875,50.5208333401613,-42.1809185638422));
#10073=CARTESIAN_POINT('Ctrl Pts',(35.6555077526845,50.312500006828,-35.6555077526845));
#10074=CARTESIAN_POINT('Ctrl Pts',(42.1809185638422,50.1041666734946,-24.3531646875));
#10075=CARTESIAN_POINT('Ctrl Pts',(48.706329375,49.8958333401613,-13.0508216223155));
#10076=CARTESIAN_POINT('Ctrl Pts',(48.706329375,49.687500006828,1.293339198242E-14));
#10077=CARTESIAN_POINT('Ctrl Pts',(48.706329375,49.4791666734946,13.0508216223155));
#10078=CARTESIAN_POINT('Ctrl Pts',(42.1809185638422,49.2708333401613,24.3531646875));
#10079=CARTESIAN_POINT('Ctrl Pts',(35.6555077526845,49.062500006828,35.6555077526845));
#10080=CARTESIAN_POINT('Ctrl Pts',(24.3531646875,48.8541666734946,42.1809185638422));
#10081=CARTESIAN_POINT('Ctrl Pts',(13.0508216223155,48.6458333401613,48.706329375));
#10082=CARTESIAN_POINT('Ctrl Pts',(-9.95098946405443E-15,48.437500006828,
48.706329375));
#10083=CARTESIAN_POINT('Ctrl Pts',(-13.0508216223155,48.2291666734946,48.706329375));
#10084=CARTESIAN_POINT('Ctrl Pts',(-24.3531646875,48.0208333401613,42.1809185638423));
#10085=CARTESIAN_POINT('Ctrl Pts',(-35.6555077526845,47.812500006828,35.6555077526845));
#10086=CARTESIAN_POINT('Ctrl Pts',(-42.1809185638422,47.6041666734946,24.3531646875));
#10087=CARTESIAN_POINT('Ctrl Pts',(-48.706329375,47.3958333401613,13.0508216223155));
#10088=CARTESIAN_POINT('Ctrl Pts',(-48.706329375,47.187500006828,-1.8898197019151E-14));
#10089=CARTESIAN_POINT('Ctrl Pts',(-48.706329375,46.9791666734946,-13.0508216223155));
#10090=CARTESIAN_POINT('Ctrl Pts',(-42.1809185638422,46.7708333401613,-24.3531646875));
#10091=CARTESIAN_POINT('Ctrl Pts',(-35.6555077526845,46.562500006828,-35.6555077526845));
#10092=CARTESIAN_POINT('Ctrl Pts',(-24.3531646875,46.3541666734946,-42.1809185638423));
#10093=CARTESIAN_POINT('Ctrl Pts',(-13.0508216223155,46.1458333401613,-48.706329375));
#10094=CARTESIAN_POINT('Ctrl Pts',(1.59157945007855E-14,45.937500006828,
-48.706329375));
#10095=CARTESIAN_POINT('Ctrl Pts',(13.0508216223155,45.7291666734946,-48.706329375));
#10096=CARTESIAN_POINT('Ctrl Pts',(24.3531646875,45.5208333401613,-42.1809185638422));
#10097=CARTESIAN_POINT('Ctrl Pts',(35.6555077526845,45.312500006828,-35.6555077526845));
#10098=CARTESIAN_POINT('Ctrl Pts',(42.1809185638422,45.1041666734946,-24.3531646875));
#10099=CARTESIAN_POINT('Ctrl Pts',(48.706329375,44.8958333401613,-13.0508216223155));
#10100=CARTESIAN_POINT('Ctrl Pts',(48.706329375,44.687500006828,1.293339198242E-14));
#10101=CARTESIAN_POINT('Ctrl Pts',(48.706329375,44.4791666734946,13.0508216223155));
#10102=CARTESIAN_POINT('Ctrl Pts',(42.1809185638422,44.2708333401613,24.3531646875));
#10103=CARTESIAN_POINT('Ctrl Pts',(35.6555077526845,44.062500006828,35.6555077526845));
#10104=CARTESIAN_POINT('Ctrl Pts',(24.3531646875,43.8541666734946,42.1809185638422));
#10105=CARTESIAN_POINT('Ctrl Pts',(13.0508216223155,43.6458333401613,48.706329375));
#10106=CARTESIAN_POINT('Ctrl Pts',(-9.95098946405443E-15,43.437500006828,
48.706329375));
#10107=CARTESIAN_POINT('Ctrl Pts',(-13.0508216223155,43.2291666734946,48.706329375));
#10108=CARTESIAN_POINT('Ctrl Pts',(-24.3531646875,43.0208333401613,42.1809185638423));
#10109=CARTESIAN_POINT('Ctrl Pts',(-35.6555077526845,42.812500006828,35.6555077526845));
#10110=CARTESIAN_POINT('Ctrl Pts',(-42.1809185638422,42.6041666734946,24.3531646875));
#10111=CARTESIAN_POINT('Ctrl Pts',(-48.706329375,42.3958333401613,13.0508216223155));
#10112=CARTESIAN_POINT('Ctrl Pts',(-48.706329375,42.187500006828,-1.8898197019151E-14));
#10113=CARTESIAN_POINT('Ctrl Pts',(-48.706329375,41.9791666734946,-13.0508216223155));
#10114=CARTESIAN_POINT('Ctrl Pts',(-42.1809185638422,41.7708333401613,-24.3531646875));
#10115=CARTESIAN_POINT('Ctrl Pts',(-35.6555077526845,41.562500006828,-35.6555077526845));
#10116=CARTESIAN_POINT('Ctrl Pts',(-24.3531646875,41.3541666734946,-42.1809185638423));
#10117=CARTESIAN_POINT('Ctrl Pts',(-13.0508216223155,41.1458333401613,-48.706329375));
#10118=CARTESIAN_POINT('Ctrl Pts',(1.59157945007855E-14,40.937500006828,
-48.706329375));
#10119=CARTESIAN_POINT('Ctrl Pts',(13.0508216223155,40.7291666734946,-48.706329375));
#10120=CARTESIAN_POINT('Ctrl Pts',(24.3531646875,40.5208333401613,-42.1809185638422));
#10121=CARTESIAN_POINT('Ctrl Pts',(35.6555077526845,40.312500006828,-35.6555077526845));
#10122=CARTESIAN_POINT('Ctrl Pts',(42.1809185638422,40.1041666734946,-24.3531646875));
#10123=CARTESIAN_POINT('Ctrl Pts',(48.706329375,39.8958333401613,-13.0508216223155));
#10124=CARTESIAN_POINT('Ctrl Pts',(48.706329375,39.687500006828,1.293339198242E-14));
#10125=CARTESIAN_POINT('Ctrl Pts',(48.706329375,39.4791666734946,13.0508216223155));
#10126=CARTESIAN_POINT('Ctrl Pts',(42.1809185638422,39.2708333401613,24.3531646875));
#10127=CARTESIAN_POINT('Ctrl Pts',(35.6555077526845,39.062500006828,35.6555077526845));
#10128=CARTESIAN_POINT('Ctrl Pts',(24.3531646875,38.8541666734946,42.1809185638422));
#10129=CARTESIAN_POINT('Ctrl Pts',(13.0508216223155,38.6458333401613,48.706329375));
#10130=CARTESIAN_POINT('Ctrl Pts',(-9.95098946405443E-15,38.437500006828,
48.706329375));
#10131=CARTESIAN_POINT('Ctrl Pts',(-13.0508216223155,38.2291666734946,48.706329375));
#10132=CARTESIAN_POINT('Ctrl Pts',(-24.3531646875,38.0208333401613,42.1809185638423));
#10133=CARTESIAN_POINT('Ctrl Pts',(-35.6555077526845,37.812500006828,35.6555077526845));
#10134=CARTESIAN_POINT('Ctrl Pts',(-42.1809185638422,37.6041666734946,24.3531646875));
#10135=CARTESIAN_POINT('Ctrl Pts',(-48.706329375,37.3958333401613,13.0508216223155));
#10136=CARTESIAN_POINT('Ctrl Pts',(-48.706329375,37.187500006828,-1.8898197019151E-14));
#10137=CARTESIAN_POINT('Ctrl Pts',(-48.706329375,36.9791666734946,-13.0508216223155));
#10138=CARTESIAN_POINT('Ctrl Pts',(-42.1809185638422,36.7708333401613,-24.3531646875));
#10139=CARTESIAN_POINT('Ctrl Pts',(-35.6555077526845,36.562500006828,-35.6555077526845));
#10140=CARTESIAN_POINT('Ctrl Pts',(-24.3531646875,36.3541666734946,-42.1809185638423));
#10141=CARTESIAN_POINT('Ctrl Pts',(-13.0508216223155,36.1458333401613,-48.706329375));
#10142=CARTESIAN_POINT('Ctrl Pts',(1.59157945007855E-14,35.937500006828,
-48.706329375));
#10143=CARTESIAN_POINT('Ctrl Pts',(13.0508216223155,35.7291666734946,-48.706329375));
#10144=CARTESIAN_POINT('Ctrl Pts',(24.3531646875,35.5208333401613,-42.1809185638422));
#10145=CARTESIAN_POINT('Ctrl Pts',(35.6555077526845,35.312500006828,-35.6555077526845));
#10146=CARTESIAN_POINT('Ctrl Pts',(42.1809185638422,35.1041666734946,-24.3531646875));
#10147=CARTESIAN_POINT('Ctrl Pts',(48.706329375,34.8958333401613,-13.0508216223155));
#10148=CARTESIAN_POINT('Ctrl Pts',(48.706329375,34.687500006828,1.293339198242E-14));
#10149=CARTESIAN_POINT('Ctrl Pts',(48.706329375,34.4791666734946,13.0508216223155));
#10150=CARTESIAN_POINT('Ctrl Pts',(42.1809185638422,34.2708333401613,24.3531646875));
#10151=CARTESIAN_POINT('Ctrl Pts',(35.6555077526845,34.062500006828,35.6555077526845));
#10152=CARTESIAN_POINT('Ctrl Pts',(24.3531646875,33.8541666734946,42.1809185638422));
#10153=CARTESIAN_POINT('Ctrl Pts',(13.0508216223155,33.6458333401613,48.706329375));
#10154=CARTESIAN_POINT('Ctrl Pts',(-9.95098946405443E-15,33.437500006828,
48.706329375));
#10155=CARTESIAN_POINT('Ctrl Pts',(-13.0508216223155,33.2291666734946,48.706329375));
#10156=CARTESIAN_POINT('Ctrl Pts',(-24.3531646875,33.0208333401613,42.1809185638423));
#10157=CARTESIAN_POINT('Ctrl Pts',(-35.6555077526845,32.812500006828,35.6555077526845));
#10158=CARTESIAN_POINT('Ctrl Pts',(-42.1809185638422,32.6041666734946,24.3531646875));
#10159=CARTESIAN_POINT('Ctrl Pts',(-48.706329375,32.3958333401613,13.0508216223155));
#10160=CARTESIAN_POINT('Ctrl Pts',(-48.706329375,32.187500006828,-1.8898197019151E-14));
#10161=CARTESIAN_POINT('Ctrl Pts',(-48.706329375,31.9791666734946,-13.0508216223155));
#10162=CARTESIAN_POINT('Ctrl Pts',(-42.1809185638422,31.7708333401613,-24.3531646875));
#10163=CARTESIAN_POINT('Ctrl Pts',(-35.6555077526845,31.562500006828,-35.6555077526845));
#10164=CARTESIAN_POINT('Ctrl Pts',(-24.3531646875,31.3541666734946,-42.1809185638423));
#10165=CARTESIAN_POINT('Ctrl Pts',(-13.0508216223155,31.1458333401613,-48.706329375));
#10166=CARTESIAN_POINT('Ctrl Pts',(1.59157945007855E-14,30.937500006828,
-48.706329375));
#10167=CARTESIAN_POINT('Ctrl Pts',(13.0508216223155,30.7291666734946,-48.706329375));
#10168=CARTESIAN_POINT('Ctrl Pts',(24.3531646875,30.5208333401613,-42.1809185638422));
#10169=CARTESIAN_POINT('Ctrl Pts',(35.6555077526845,30.312500006828,-35.6555077526845));
#10170=CARTESIAN_POINT('Ctrl Pts',(42.1809185638422,30.1041666734946,-24.3531646875));
#10171=CARTESIAN_POINT('Ctrl Pts',(48.706329375,29.8958333401613,-13.0508216223155));
#10172=CARTESIAN_POINT('Ctrl Pts',(48.706329375,29.687500006828,1.293339198242E-14));
#10173=CARTESIAN_POINT('Ctrl Pts',(48.706329375,29.4791666734946,13.0508216223155));
#10174=CARTESIAN_POINT('Ctrl Pts',(42.1809185638422,29.2708333401613,24.3531646875));
#10175=CARTESIAN_POINT('Ctrl Pts',(35.6555077526845,29.062500006828,35.6555077526845));
#10176=CARTESIAN_POINT('Ctrl Pts',(24.3531646875,28.8541666734946,42.1809185638422));
#10177=CARTESIAN_POINT('Ctrl Pts',(13.0508216223155,28.6458333401613,48.706329375));
#10178=CARTESIAN_POINT('Ctrl Pts',(-9.95098946405443E-15,28.437500006828,
48.706329375));
#10179=CARTESIAN_POINT('Ctrl Pts',(-13.0508216223155,28.2291666734946,48.706329375));
#10180=CARTESIAN_POINT('Ctrl Pts',(-24.3531646875,28.0208333401613,42.1809185638423));
#10181=CARTESIAN_POINT('Ctrl Pts',(-35.6555077526845,27.812500006828,35.6555077526845));
#10182=CARTESIAN_POINT('Ctrl Pts',(-42.1809185638422,27.6041666734946,24.3531646875));
#10183=CARTESIAN_POINT('Ctrl Pts',(-48.706329375,27.3958333401613,13.0508216223155));
#10184=CARTESIAN_POINT('Ctrl Pts',(-48.706329375,27.187500006828,-1.8898197019151E-14));
#10185=CARTESIAN_POINT('',(-4.32456003949883,43.3676432269777,48.5139639861634));
#10186=CARTESIAN_POINT('',(-48.5725845633798,42.2456516907297,3.60701400320326));
#10187=CARTESIAN_POINT('Ctrl Pts',(-4.32456003949883,43.3676432269777,48.5139639861634));
#10188=CARTESIAN_POINT('Ctrl Pts',(-15.0381414154991,43.1925348924095,47.5589497574396));
#10189=CARTESIAN_POINT('Ctrl Pts',(-24.3531646875,43.0208333401613,42.1809185638423));
#10190=CARTESIAN_POINT('Ctrl Pts',(-35.6555077526845,42.812500006828,35.6555077526845));
#10191=CARTESIAN_POINT('Ctrl Pts',(-42.1809185638422,42.6041666734946,24.3531646875));
#10192=CARTESIAN_POINT('Ctrl Pts',(-47.7480251419552,42.4264286116308,14.7106532430575));
#10193=CARTESIAN_POINT('Ctrl Pts',(-48.5725845633798,42.2456516907297,3.60701400320326));
#10194=CARTESIAN_POINT('Ctrl Pts',(-48.5725845633798,42.2456516907297,3.60701400320326));
#10195=CARTESIAN_POINT('Ctrl Pts',(-48.3407853679392,42.1124685639422,3.60701400320326));
#10196=CARTESIAN_POINT('Ctrl Pts',(-48.1089821836664,41.9792923792741,3.60701400320326));
#10197=CARTESIAN_POINT('Ctrl Pts',(-47.6453674864979,41.7129545080418,3.60701400320326));
#10198=CARTESIAN_POINT('Ctrl Pts',(-47.4135559734253,41.5797928212585,3.60701400320325));
#10199=CARTESIAN_POINT('Ctrl Pts',(-47.1817401099609,41.4466387085919,3.60701400320325));
#10200=CARTESIAN_POINT('Ctrl Pts',(-46.7406305897488,41.1932671494809,3.60701400320325));
#10201=CARTESIAN_POINT('Ctrl Pts',(-46.2995053259033,40.9399229970588,3.60701400320326));
#10202=CARTESIAN_POINT('Ctrl Pts',(-45.858362923034,40.686608693912,3.60701400320327));
#10203=CARTESIAN_POINT('Ctrl Pts',(-4.32456003949882,41.8009818542622,45.7962681936506));
#10204=CARTESIAN_POINT('Ctrl Pts',(-4.32456003949882,41.9344874667937,46.0278818021281));
#10205=CARTESIAN_POINT('Ctrl Pts',(-4.3245600394987,42.2015035419424,46.4911062234486));
#10206=CARTESIAN_POINT('Ctrl Pts',(-4.32456003949883,42.4685288945405,46.954325296818));
#10207=CARTESIAN_POINT('Ctrl Pts',(-4.32456003949883,42.8572357107336,47.6286149142205));
#10208=CARTESIAN_POINT('Ctrl Pts',(-4.32456003949883,43.1124357360102,48.0712916022845));
#10209=CARTESIAN_POINT('Ctrl Pts',(-4.32456003949883,43.3676432269777,48.5139639861634));
#10210=CARTESIAN_POINT('Ctrl Pts',(-46.,55.6250000136559,0.));
#10211=CARTESIAN_POINT('Ctrl Pts',(-46.,55.4166666803226,-12.3256628518316));
#10212=CARTESIAN_POINT('Ctrl Pts',(-39.8371685740842,55.2083333469893,-23.));
#10213=CARTESIAN_POINT('Ctrl Pts',(-33.6743371481684,55.0000000136559,-33.6743371481684));
#10214=CARTESIAN_POINT('Ctrl Pts',(-23.,54.7916666803226,-39.8371685740842));
#10215=CARTESIAN_POINT('Ctrl Pts',(-12.3256628518317,54.5833333469893,-46.));
#10216=CARTESIAN_POINT('Ctrl Pts',(-2.81668763803891E-15,54.3750000136559,
-46.));
#10217=CARTESIAN_POINT('Ctrl Pts',(12.3256628518316,54.1666666803226,-46.));
#10218=CARTESIAN_POINT('Ctrl Pts',(23.,53.9583333469893,-39.8371685740842));
#10219=CARTESIAN_POINT('Ctrl Pts',(33.6743371481683,53.7500000136559,-33.6743371481684));
#10220=CARTESIAN_POINT('Ctrl Pts',(39.8371685740842,53.5416666803226,-23.));
#10221=CARTESIAN_POINT('Ctrl Pts',(46.,53.3333333469893,-12.3256628518317));
#10222=CARTESIAN_POINT('Ctrl Pts',(46.,53.1250000136559,-5.63337527607782E-15));
#10223=CARTESIAN_POINT('Ctrl Pts',(46.,52.9166666803226,12.3256628518316));
#10224=CARTESIAN_POINT('Ctrl Pts',(39.8371685740842,52.7083333469893,23.));
#10225=CARTESIAN_POINT('Ctrl Pts',(33.6743371481684,52.5000000136559,33.6743371481683));
#10226=CARTESIAN_POINT('Ctrl Pts',(23.,52.2916666803226,39.8371685740842));
#10227=CARTESIAN_POINT('Ctrl Pts',(12.3256628518317,52.0833333469893,46.));
#10228=CARTESIAN_POINT('Ctrl Pts',(8.45006291411674E-15,51.8750000136559,
46.));
#10229=CARTESIAN_POINT('Ctrl Pts',(-12.3256628518316,51.6666666803226,46.));
#10230=CARTESIAN_POINT('Ctrl Pts',(-23.,51.4583333469893,39.8371685740842));
#10231=CARTESIAN_POINT('Ctrl Pts',(-33.6743371481683,51.2500000136559,33.6743371481684));
#10232=CARTESIAN_POINT('Ctrl Pts',(-39.8371685740842,51.0416666803226,23.));
#10233=CARTESIAN_POINT('Ctrl Pts',(-46.,50.8333333469893,12.3256628518317));
#10234=CARTESIAN_POINT('Ctrl Pts',(-46.,50.6250000136559,0.));
#10235=CARTESIAN_POINT('Ctrl Pts',(-46.,50.4166666803226,-12.3256628518316));
#10236=CARTESIAN_POINT('Ctrl Pts',(-39.8371685740842,50.2083333469893,-23.));
#10237=CARTESIAN_POINT('Ctrl Pts',(-33.6743371481684,50.0000000136559,-33.6743371481684));
#10238=CARTESIAN_POINT('Ctrl Pts',(-23.,49.7916666803226,-39.8371685740842));
#10239=CARTESIAN_POINT('Ctrl Pts',(-12.3256628518317,49.5833333469893,-46.));
#10240=CARTESIAN_POINT('Ctrl Pts',(-2.81668763803891E-15,49.3750000136559,
-46.));
#10241=CARTESIAN_POINT('Ctrl Pts',(12.3256628518316,49.1666666803226,-46.));
#10242=CARTESIAN_POINT('Ctrl Pts',(23.,48.9583333469893,-39.8371685740842));
#10243=CARTESIAN_POINT('Ctrl Pts',(33.6743371481683,48.7500000136559,-33.6743371481684));
#10244=CARTESIAN_POINT('Ctrl Pts',(39.8371685740842,48.5416666803226,-23.));
#10245=CARTESIAN_POINT('Ctrl Pts',(46.,48.3333333469893,-12.3256628518317));
#10246=CARTESIAN_POINT('Ctrl Pts',(46.,48.1250000136559,-5.63337527607782E-15));
#10247=CARTESIAN_POINT('Ctrl Pts',(46.,47.9166666803226,12.3256628518316));
#10248=CARTESIAN_POINT('Ctrl Pts',(39.8371685740842,47.7083333469893,23.));
#10249=CARTESIAN_POINT('Ctrl Pts',(33.6743371481684,47.5000000136559,33.6743371481683));
#10250=CARTESIAN_POINT('Ctrl Pts',(23.,47.2916666803226,39.8371685740842));
#10251=CARTESIAN_POINT('Ctrl Pts',(12.3256628518317,47.0833333469893,46.));
#10252=CARTESIAN_POINT('Ctrl Pts',(8.45006291411674E-15,46.8750000136559,
46.));
#10253=CARTESIAN_POINT('Ctrl Pts',(-12.3256628518316,46.6666666803226,46.));
#10254=CARTESIAN_POINT('Ctrl Pts',(-23.,46.4583333469893,39.8371685740842));
#10255=CARTESIAN_POINT('Ctrl Pts',(-33.6743371481683,46.2500000136559,33.6743371481684));
#10256=CARTESIAN_POINT('Ctrl Pts',(-39.8371685740842,46.0416666803226,23.));
#10257=CARTESIAN_POINT('Ctrl Pts',(-46.,45.8333333469892,12.3256628518317));
#10258=CARTESIAN_POINT('Ctrl Pts',(-46.,45.6250000136559,0.));
#10259=CARTESIAN_POINT('Ctrl Pts',(-46.,45.4166666803226,-12.3256628518316));
#10260=CARTESIAN_POINT('Ctrl Pts',(-39.8371685740842,45.2083333469893,-23.));
#10261=CARTESIAN_POINT('Ctrl Pts',(-33.6743371481684,45.0000000136559,-33.6743371481684));
#10262=CARTESIAN_POINT('Ctrl Pts',(-23.,44.7916666803226,-39.8371685740842));
#10263=CARTESIAN_POINT('Ctrl Pts',(-12.3256628518317,44.5833333469893,-46.));
#10264=CARTESIAN_POINT('Ctrl Pts',(-2.81668763803891E-15,44.3750000136559,
-46.));
#10265=CARTESIAN_POINT('Ctrl Pts',(12.3256628518316,44.1666666803226,-46.));
#10266=CARTESIAN_POINT('Ctrl Pts',(23.,43.9583333469893,-39.8371685740842));
#10267=CARTESIAN_POINT('Ctrl Pts',(33.6743371481683,43.7500000136559,-33.6743371481684));
#10268=CARTESIAN_POINT('Ctrl Pts',(39.8371685740842,43.5416666803226,-23.));
#10269=CARTESIAN_POINT('Ctrl Pts',(46.,43.3333333469893,-12.3256628518317));
#10270=CARTESIAN_POINT('Ctrl Pts',(46.,43.1250000136559,-5.63337527607782E-15));
#10271=CARTESIAN_POINT('Ctrl Pts',(46.,42.9166666803226,12.3256628518316));
#10272=CARTESIAN_POINT('Ctrl Pts',(39.8371685740842,42.7083333469893,23.));
#10273=CARTESIAN_POINT('Ctrl Pts',(33.6743371481684,42.5000000136559,33.6743371481683));
#10274=CARTESIAN_POINT('Ctrl Pts',(23.,42.2916666803226,39.8371685740842));
#10275=CARTESIAN_POINT('Ctrl Pts',(12.3256628518317,42.0833333469893,46.));
#10276=CARTESIAN_POINT('Ctrl Pts',(8.45006291411674E-15,41.8750000136559,
46.));
#10277=CARTESIAN_POINT('Ctrl Pts',(-12.3256628518316,41.6666666803226,46.));
#10278=CARTESIAN_POINT('Ctrl Pts',(-23.,41.4583333469893,39.8371685740842));
#10279=CARTESIAN_POINT('Ctrl Pts',(-33.6743371481683,41.2500000136559,33.6743371481684));
#10280=CARTESIAN_POINT('Ctrl Pts',(-39.8371685740842,41.0416666803226,23.));
#10281=CARTESIAN_POINT('Ctrl Pts',(-46.,40.8333333469893,12.3256628518317));
#10282=CARTESIAN_POINT('Ctrl Pts',(-46.,40.6250000136559,0.));
#10283=CARTESIAN_POINT('Ctrl Pts',(-46.,40.4166666803226,-12.3256628518316));
#10284=CARTESIAN_POINT('Ctrl Pts',(-39.8371685740842,40.2083333469893,-23.));
#10285=CARTESIAN_POINT('Ctrl Pts',(-33.6743371481684,40.0000000136559,-33.6743371481684));
#10286=CARTESIAN_POINT('Ctrl Pts',(-23.,39.7916666803226,-39.8371685740842));
#10287=CARTESIAN_POINT('Ctrl Pts',(-12.3256628518317,39.5833333469893,-46.));
#10288=CARTESIAN_POINT('Ctrl Pts',(-2.81668763803891E-15,39.3750000136559,
-46.));
#10289=CARTESIAN_POINT('Ctrl Pts',(12.3256628518316,39.1666666803226,-46.));
#10290=CARTESIAN_POINT('Ctrl Pts',(23.,38.9583333469893,-39.8371685740842));
#10291=CARTESIAN_POINT('Ctrl Pts',(33.6743371481683,38.7500000136559,-33.6743371481684));
#10292=CARTESIAN_POINT('Ctrl Pts',(39.8371685740842,38.5416666803226,-23.));
#10293=CARTESIAN_POINT('Ctrl Pts',(46.,38.3333333469893,-12.3256628518317));
#10294=CARTESIAN_POINT('Ctrl Pts',(46.,38.1250000136559,-5.63337527607782E-15));
#10295=CARTESIAN_POINT('Ctrl Pts',(46.,37.9166666803226,12.3256628518316));
#10296=CARTESIAN_POINT('Ctrl Pts',(39.8371685740842,37.7083333469893,23.));
#10297=CARTESIAN_POINT('Ctrl Pts',(33.6743371481684,37.5000000136559,33.6743371481683));
#10298=CARTESIAN_POINT('Ctrl Pts',(23.,37.2916666803226,39.8371685740842));
#10299=CARTESIAN_POINT('Ctrl Pts',(12.3256628518317,37.0833333469893,46.));
#10300=CARTESIAN_POINT('Ctrl Pts',(8.45006291411674E-15,36.8750000136559,
46.));
#10301=CARTESIAN_POINT('Ctrl Pts',(-12.3256628518316,36.6666666803226,46.));
#10302=CARTESIAN_POINT('Ctrl Pts',(-23.,36.4583333469893,39.8371685740842));
#10303=CARTESIAN_POINT('Ctrl Pts',(-33.6743371481683,36.2500000136559,33.6743371481684));
#10304=CARTESIAN_POINT('Ctrl Pts',(-39.8371685740842,36.0416666803226,23.));
#10305=CARTESIAN_POINT('Ctrl Pts',(-46.,35.8333333469893,12.3256628518317));
#10306=CARTESIAN_POINT('Ctrl Pts',(-46.,35.6250000136559,0.));
#10307=CARTESIAN_POINT('Ctrl Pts',(-46.,35.4166666803226,-12.3256628518316));
#10308=CARTESIAN_POINT('Ctrl Pts',(-39.8371685740842,35.2083333469893,-23.));
#10309=CARTESIAN_POINT('Ctrl Pts',(-33.6743371481684,35.0000000136559,-33.6743371481684));
#10310=CARTESIAN_POINT('Ctrl Pts',(-23.,34.7916666803226,-39.8371685740842));
#10311=CARTESIAN_POINT('Ctrl Pts',(-12.3256628518317,34.5833333469893,-46.));
#10312=CARTESIAN_POINT('Ctrl Pts',(-2.81668763803891E-15,34.3750000136559,
-46.));
#10313=CARTESIAN_POINT('Ctrl Pts',(12.3256628518316,34.1666666803226,-46.));
#10314=CARTESIAN_POINT('Ctrl Pts',(23.,33.9583333469893,-39.8371685740842));
#10315=CARTESIAN_POINT('Ctrl Pts',(33.6743371481683,33.7500000136559,-33.6743371481684));
#10316=CARTESIAN_POINT('Ctrl Pts',(39.8371685740842,33.5416666803226,-23.));
#10317=CARTESIAN_POINT('Ctrl Pts',(46.,33.3333333469893,-12.3256628518317));
#10318=CARTESIAN_POINT('Ctrl Pts',(46.,33.1250000136559,-5.63337527607782E-15));
#10319=CARTESIAN_POINT('Ctrl Pts',(46.,32.9166666803226,12.3256628518316));
#10320=CARTESIAN_POINT('Ctrl Pts',(39.8371685740842,32.7083333469893,23.));
#10321=CARTESIAN_POINT('Ctrl Pts',(33.6743371481684,32.5000000136559,33.6743371481683));
#10322=CARTESIAN_POINT('Ctrl Pts',(23.,32.2916666803226,39.8371685740842));
#10323=CARTESIAN_POINT('Ctrl Pts',(12.3256628518317,32.0833333469893,46.));
#10324=CARTESIAN_POINT('Ctrl Pts',(8.45006291411674E-15,31.8750000136559,
46.));
#10325=CARTESIAN_POINT('Ctrl Pts',(-12.3256628518316,31.6666666803226,46.));
#10326=CARTESIAN_POINT('Ctrl Pts',(-23.,31.4583333469893,39.8371685740842));
#10327=CARTESIAN_POINT('Ctrl Pts',(-33.6743371481683,31.2500000136559,33.6743371481684));
#10328=CARTESIAN_POINT('Ctrl Pts',(-39.8371685740842,31.0416666803226,23.));
#10329=CARTESIAN_POINT('Ctrl Pts',(-46.,30.8333333469893,12.3256628518317));
#10330=CARTESIAN_POINT('Ctrl Pts',(-46.,30.6250000136559,0.));
#10331=CARTESIAN_POINT('Ctrl Pts',(-46.,30.4166666803226,-12.3256628518316));
#10332=CARTESIAN_POINT('Ctrl Pts',(-39.8371685740842,30.2083333469893,-23.));
#10333=CARTESIAN_POINT('Ctrl Pts',(-33.6743371481684,30.0000000136559,-33.6743371481684));
#10334=CARTESIAN_POINT('Ctrl Pts',(-23.,29.7916666803226,-39.8371685740842));
#10335=CARTESIAN_POINT('Ctrl Pts',(-12.3256628518317,29.5833333469893,-46.));
#10336=CARTESIAN_POINT('Ctrl Pts',(-2.81668763803891E-15,29.3750000136559,
-46.));
#10337=CARTESIAN_POINT('Ctrl Pts',(12.3256628518316,29.1666666803226,-46.));
#10338=CARTESIAN_POINT('Ctrl Pts',(23.,28.9583333469893,-39.8371685740842));
#10339=CARTESIAN_POINT('Ctrl Pts',(33.6743371481683,28.7500000136559,-33.6743371481684));
#10340=CARTESIAN_POINT('Ctrl Pts',(39.8371685740842,28.5416666803226,-23.));
#10341=CARTESIAN_POINT('Ctrl Pts',(46.,28.3333333469893,-12.3256628518317));
#10342=CARTESIAN_POINT('Ctrl Pts',(46.,28.1250000136559,-5.63337527607782E-15));
#10343=CARTESIAN_POINT('Ctrl Pts',(46.,27.9166666803226,12.3256628518316));
#10344=CARTESIAN_POINT('Ctrl Pts',(39.8371685740842,27.7083333469893,23.));
#10345=CARTESIAN_POINT('Ctrl Pts',(33.6743371481684,27.5000000136559,33.6743371481683));
#10346=CARTESIAN_POINT('Ctrl Pts',(23.,27.2916666803226,39.8371685740842));
#10347=CARTESIAN_POINT('Ctrl Pts',(12.3256628518317,27.0833333469893,46.));
#10348=CARTESIAN_POINT('Ctrl Pts',(8.45006291411674E-15,26.8750000136559,
46.));
#10349=CARTESIAN_POINT('Ctrl Pts',(-12.3256628518316,26.6666666803226,46.));
#10350=CARTESIAN_POINT('Ctrl Pts',(-23.,26.4583333469893,39.8371685740842));
#10351=CARTESIAN_POINT('Ctrl Pts',(-33.6743371481683,26.2500000136559,33.6743371481684));
#10352=CARTESIAN_POINT('Ctrl Pts',(-39.8371685740842,26.0416666803226,23.));
#10353=CARTESIAN_POINT('Ctrl Pts',(-46.,25.8333333469893,12.3256628518317));
#10354=CARTESIAN_POINT('Ctrl Pts',(-46.,25.6250000136559,0.));
#10355=CARTESIAN_POINT('Ctrl Pts',(-48.706329375,57.187500006828,-1.8898197019151E-14));
#10356=CARTESIAN_POINT('Ctrl Pts',(-48.706329375,56.9791666734946,-13.0508216223155));
#10357=CARTESIAN_POINT('Ctrl Pts',(-42.1809185638422,56.7708333401613,-24.3531646875));
#10358=CARTESIAN_POINT('Ctrl Pts',(-35.6555077526845,56.562500006828,-35.6555077526845));
#10359=CARTESIAN_POINT('Ctrl Pts',(-24.3531646875,56.3541666734946,-42.1809185638423));
#10360=CARTESIAN_POINT('Ctrl Pts',(-13.0508216223155,56.1458333401613,-48.706329375));
#10361=CARTESIAN_POINT('Ctrl Pts',(1.59157945007855E-14,55.937500006828,
-48.706329375));
#10362=CARTESIAN_POINT('Ctrl Pts',(13.0508216223155,55.7291666734946,-48.706329375));
#10363=CARTESIAN_POINT('Ctrl Pts',(24.3531646875,55.5208333401613,-42.1809185638422));
#10364=CARTESIAN_POINT('Ctrl Pts',(35.6555077526845,55.312500006828,-35.6555077526845));
#10365=CARTESIAN_POINT('Ctrl Pts',(42.1809185638422,55.1041666734946,-24.3531646875));
#10366=CARTESIAN_POINT('Ctrl Pts',(48.706329375,54.8958333401613,-13.0508216223155));
#10367=CARTESIAN_POINT('Ctrl Pts',(48.706329375,54.687500006828,1.293339198242E-14));
#10368=CARTESIAN_POINT('Ctrl Pts',(48.706329375,54.4791666734946,13.0508216223155));
#10369=CARTESIAN_POINT('Ctrl Pts',(42.1809185638422,54.2708333401613,24.3531646875));
#10370=CARTESIAN_POINT('Ctrl Pts',(35.6555077526845,54.062500006828,35.6555077526845));
#10371=CARTESIAN_POINT('Ctrl Pts',(24.3531646875,53.8541666734946,42.1809185638422));
#10372=CARTESIAN_POINT('Ctrl Pts',(13.0508216223155,53.6458333401613,48.706329375));
#10373=CARTESIAN_POINT('Ctrl Pts',(-9.95098946405443E-15,53.437500006828,
48.706329375));
#10374=CARTESIAN_POINT('Ctrl Pts',(-13.0508216223155,53.2291666734946,48.706329375));
#10375=CARTESIAN_POINT('Ctrl Pts',(-24.3531646875,53.0208333401613,42.1809185638423));
#10376=CARTESIAN_POINT('Ctrl Pts',(-35.6555077526845,52.812500006828,35.6555077526845));
#10377=CARTESIAN_POINT('Ctrl Pts',(-42.1809185638422,52.6041666734946,24.3531646875));
#10378=CARTESIAN_POINT('Ctrl Pts',(-48.706329375,52.3958333401613,13.0508216223155));
#10379=CARTESIAN_POINT('Ctrl Pts',(-48.706329375,52.187500006828,-1.8898197019151E-14));
#10380=CARTESIAN_POINT('Ctrl Pts',(-48.706329375,51.9791666734946,-13.0508216223155));
#10381=CARTESIAN_POINT('Ctrl Pts',(-42.1809185638422,51.7708333401613,-24.3531646875));
#10382=CARTESIAN_POINT('Ctrl Pts',(-35.6555077526845,51.562500006828,-35.6555077526845));
#10383=CARTESIAN_POINT('Ctrl Pts',(-24.3531646875,51.3541666734946,-42.1809185638423));
#10384=CARTESIAN_POINT('Ctrl Pts',(-13.0508216223155,51.1458333401613,-48.706329375));
#10385=CARTESIAN_POINT('Ctrl Pts',(1.59157945007855E-14,50.937500006828,
-48.706329375));
#10386=CARTESIAN_POINT('Ctrl Pts',(13.0508216223155,50.7291666734946,-48.706329375));
#10387=CARTESIAN_POINT('Ctrl Pts',(24.3531646875,50.5208333401613,-42.1809185638422));
#10388=CARTESIAN_POINT('Ctrl Pts',(35.6555077526845,50.312500006828,-35.6555077526845));
#10389=CARTESIAN_POINT('Ctrl Pts',(42.1809185638422,50.1041666734946,-24.3531646875));
#10390=CARTESIAN_POINT('Ctrl Pts',(48.706329375,49.8958333401613,-13.0508216223155));
#10391=CARTESIAN_POINT('Ctrl Pts',(48.706329375,49.687500006828,1.293339198242E-14));
#10392=CARTESIAN_POINT('Ctrl Pts',(48.706329375,49.4791666734946,13.0508216223155));
#10393=CARTESIAN_POINT('Ctrl Pts',(42.1809185638422,49.2708333401613,24.3531646875));
#10394=CARTESIAN_POINT('Ctrl Pts',(35.6555077526845,49.062500006828,35.6555077526845));
#10395=CARTESIAN_POINT('Ctrl Pts',(24.3531646875,48.8541666734946,42.1809185638422));
#10396=CARTESIAN_POINT('Ctrl Pts',(13.0508216223155,48.6458333401613,48.706329375));
#10397=CARTESIAN_POINT('Ctrl Pts',(-9.95098946405443E-15,48.437500006828,
48.706329375));
#10398=CARTESIAN_POINT('Ctrl Pts',(-13.0508216223155,48.2291666734946,48.706329375));
#10399=CARTESIAN_POINT('Ctrl Pts',(-24.3531646875,48.0208333401613,42.1809185638423));
#10400=CARTESIAN_POINT('Ctrl Pts',(-35.6555077526845,47.812500006828,35.6555077526845));
#10401=CARTESIAN_POINT('Ctrl Pts',(-42.1809185638422,47.6041666734946,24.3531646875));
#10402=CARTESIAN_POINT('Ctrl Pts',(-48.706329375,47.3958333401613,13.0508216223155));
#10403=CARTESIAN_POINT('Ctrl Pts',(-48.706329375,47.187500006828,-1.8898197019151E-14));
#10404=CARTESIAN_POINT('Ctrl Pts',(-48.706329375,46.9791666734946,-13.0508216223155));
#10405=CARTESIAN_POINT('Ctrl Pts',(-42.1809185638422,46.7708333401613,-24.3531646875));
#10406=CARTESIAN_POINT('Ctrl Pts',(-35.6555077526845,46.562500006828,-35.6555077526845));
#10407=CARTESIAN_POINT('Ctrl Pts',(-24.3531646875,46.3541666734946,-42.1809185638423));
#10408=CARTESIAN_POINT('Ctrl Pts',(-13.0508216223155,46.1458333401613,-48.706329375));
#10409=CARTESIAN_POINT('Ctrl Pts',(1.59157945007855E-14,45.937500006828,
-48.706329375));
#10410=CARTESIAN_POINT('Ctrl Pts',(13.0508216223155,45.7291666734946,-48.706329375));
#10411=CARTESIAN_POINT('Ctrl Pts',(24.3531646875,45.5208333401613,-42.1809185638422));
#10412=CARTESIAN_POINT('Ctrl Pts',(35.6555077526845,45.312500006828,-35.6555077526845));
#10413=CARTESIAN_POINT('Ctrl Pts',(42.1809185638422,45.1041666734946,-24.3531646875));
#10414=CARTESIAN_POINT('Ctrl Pts',(48.706329375,44.8958333401613,-13.0508216223155));
#10415=CARTESIAN_POINT('Ctrl Pts',(48.706329375,44.687500006828,1.293339198242E-14));
#10416=CARTESIAN_POINT('Ctrl Pts',(48.706329375,44.4791666734946,13.0508216223155));
#10417=CARTESIAN_POINT('Ctrl Pts',(42.1809185638422,44.2708333401613,24.3531646875));
#10418=CARTESIAN_POINT('Ctrl Pts',(35.6555077526845,44.062500006828,35.6555077526845));
#10419=CARTESIAN_POINT('Ctrl Pts',(24.3531646875,43.8541666734946,42.1809185638422));
#10420=CARTESIAN_POINT('Ctrl Pts',(13.0508216223155,43.6458333401613,48.706329375));
#10421=CARTESIAN_POINT('Ctrl Pts',(-9.95098946405443E-15,43.437500006828,
48.706329375));
#10422=CARTESIAN_POINT('Ctrl Pts',(-13.0508216223155,43.2291666734946,48.706329375));
#10423=CARTESIAN_POINT('Ctrl Pts',(-24.3531646875,43.0208333401613,42.1809185638423));
#10424=CARTESIAN_POINT('Ctrl Pts',(-35.6555077526845,42.812500006828,35.6555077526845));
#10425=CARTESIAN_POINT('Ctrl Pts',(-42.1809185638422,42.6041666734946,24.3531646875));
#10426=CARTESIAN_POINT('Ctrl Pts',(-48.706329375,42.3958333401613,13.0508216223155));
#10427=CARTESIAN_POINT('Ctrl Pts',(-48.706329375,42.187500006828,-1.8898197019151E-14));
#10428=CARTESIAN_POINT('Ctrl Pts',(-48.706329375,41.9791666734946,-13.0508216223155));
#10429=CARTESIAN_POINT('Ctrl Pts',(-42.1809185638422,41.7708333401613,-24.3531646875));
#10430=CARTESIAN_POINT('Ctrl Pts',(-35.6555077526845,41.562500006828,-35.6555077526845));
#10431=CARTESIAN_POINT('Ctrl Pts',(-24.3531646875,41.3541666734946,-42.1809185638423));
#10432=CARTESIAN_POINT('Ctrl Pts',(-13.0508216223155,41.1458333401613,-48.706329375));
#10433=CARTESIAN_POINT('Ctrl Pts',(1.59157945007855E-14,40.937500006828,
-48.706329375));
#10434=CARTESIAN_POINT('Ctrl Pts',(13.0508216223155,40.7291666734946,-48.706329375));
#10435=CARTESIAN_POINT('Ctrl Pts',(24.3531646875,40.5208333401613,-42.1809185638422));
#10436=CARTESIAN_POINT('Ctrl Pts',(35.6555077526845,40.312500006828,-35.6555077526845));
#10437=CARTESIAN_POINT('Ctrl Pts',(42.1809185638422,40.1041666734946,-24.3531646875));
#10438=CARTESIAN_POINT('Ctrl Pts',(48.706329375,39.8958333401613,-13.0508216223155));
#10439=CARTESIAN_POINT('Ctrl Pts',(48.706329375,39.687500006828,1.293339198242E-14));
#10440=CARTESIAN_POINT('Ctrl Pts',(48.706329375,39.4791666734946,13.0508216223155));
#10441=CARTESIAN_POINT('Ctrl Pts',(42.1809185638422,39.2708333401613,24.3531646875));
#10442=CARTESIAN_POINT('Ctrl Pts',(35.6555077526845,39.062500006828,35.6555077526845));
#10443=CARTESIAN_POINT('Ctrl Pts',(24.3531646875,38.8541666734946,42.1809185638422));
#10444=CARTESIAN_POINT('Ctrl Pts',(13.0508216223155,38.6458333401613,48.706329375));
#10445=CARTESIAN_POINT('Ctrl Pts',(-9.95098946405443E-15,38.437500006828,
48.706329375));
#10446=CARTESIAN_POINT('Ctrl Pts',(-13.0508216223155,38.2291666734946,48.706329375));
#10447=CARTESIAN_POINT('Ctrl Pts',(-24.3531646875,38.0208333401613,42.1809185638423));
#10448=CARTESIAN_POINT('Ctrl Pts',(-35.6555077526845,37.812500006828,35.6555077526845));
#10449=CARTESIAN_POINT('Ctrl Pts',(-42.1809185638422,37.6041666734946,24.3531646875));
#10450=CARTESIAN_POINT('Ctrl Pts',(-48.706329375,37.3958333401613,13.0508216223155));
#10451=CARTESIAN_POINT('Ctrl Pts',(-48.706329375,37.187500006828,-1.8898197019151E-14));
#10452=CARTESIAN_POINT('Ctrl Pts',(-48.706329375,36.9791666734946,-13.0508216223155));
#10453=CARTESIAN_POINT('Ctrl Pts',(-42.1809185638422,36.7708333401613,-24.3531646875));
#10454=CARTESIAN_POINT('Ctrl Pts',(-35.6555077526845,36.562500006828,-35.6555077526845));
#10455=CARTESIAN_POINT('Ctrl Pts',(-24.3531646875,36.3541666734946,-42.1809185638423));
#10456=CARTESIAN_POINT('Ctrl Pts',(-13.0508216223155,36.1458333401613,-48.706329375));
#10457=CARTESIAN_POINT('Ctrl Pts',(1.59157945007855E-14,35.937500006828,
-48.706329375));
#10458=CARTESIAN_POINT('Ctrl Pts',(13.0508216223155,35.7291666734946,-48.706329375));
#10459=CARTESIAN_POINT('Ctrl Pts',(24.3531646875,35.5208333401613,-42.1809185638422));
#10460=CARTESIAN_POINT('Ctrl Pts',(35.6555077526845,35.312500006828,-35.6555077526845));
#10461=CARTESIAN_POINT('Ctrl Pts',(42.1809185638422,35.1041666734946,-24.3531646875));
#10462=CARTESIAN_POINT('Ctrl Pts',(48.706329375,34.8958333401613,-13.0508216223155));
#10463=CARTESIAN_POINT('Ctrl Pts',(48.706329375,34.687500006828,1.293339198242E-14));
#10464=CARTESIAN_POINT('Ctrl Pts',(48.706329375,34.4791666734946,13.0508216223155));
#10465=CARTESIAN_POINT('Ctrl Pts',(42.1809185638422,34.2708333401613,24.3531646875));
#10466=CARTESIAN_POINT('Ctrl Pts',(35.6555077526845,34.062500006828,35.6555077526845));
#10467=CARTESIAN_POINT('Ctrl Pts',(24.3531646875,33.8541666734946,42.1809185638422));
#10468=CARTESIAN_POINT('Ctrl Pts',(13.0508216223155,33.6458333401613,48.706329375));
#10469=CARTESIAN_POINT('Ctrl Pts',(-9.95098946405443E-15,33.437500006828,
48.706329375));
#10470=CARTESIAN_POINT('Ctrl Pts',(-13.0508216223155,33.2291666734946,48.706329375));
#10471=CARTESIAN_POINT('Ctrl Pts',(-24.3531646875,33.0208333401613,42.1809185638423));
#10472=CARTESIAN_POINT('Ctrl Pts',(-35.6555077526845,32.812500006828,35.6555077526845));
#10473=CARTESIAN_POINT('Ctrl Pts',(-42.1809185638422,32.6041666734946,24.3531646875));
#10474=CARTESIAN_POINT('Ctrl Pts',(-48.706329375,32.3958333401613,13.0508216223155));
#10475=CARTESIAN_POINT('Ctrl Pts',(-48.706329375,32.187500006828,-1.8898197019151E-14));
#10476=CARTESIAN_POINT('Ctrl Pts',(-48.706329375,31.9791666734946,-13.0508216223155));
#10477=CARTESIAN_POINT('Ctrl Pts',(-42.1809185638422,31.7708333401613,-24.3531646875));
#10478=CARTESIAN_POINT('Ctrl Pts',(-35.6555077526845,31.562500006828,-35.6555077526845));
#10479=CARTESIAN_POINT('Ctrl Pts',(-24.3531646875,31.3541666734946,-42.1809185638423));
#10480=CARTESIAN_POINT('Ctrl Pts',(-13.0508216223155,31.1458333401613,-48.706329375));
#10481=CARTESIAN_POINT('Ctrl Pts',(1.59157945007855E-14,30.937500006828,
-48.706329375));
#10482=CARTESIAN_POINT('Ctrl Pts',(13.0508216223155,30.7291666734946,-48.706329375));
#10483=CARTESIAN_POINT('Ctrl Pts',(24.3531646875,30.5208333401613,-42.1809185638422));
#10484=CARTESIAN_POINT('Ctrl Pts',(35.6555077526845,30.312500006828,-35.6555077526845));
#10485=CARTESIAN_POINT('Ctrl Pts',(42.1809185638422,30.1041666734946,-24.3531646875));
#10486=CARTESIAN_POINT('Ctrl Pts',(48.706329375,29.8958333401613,-13.0508216223155));
#10487=CARTESIAN_POINT('Ctrl Pts',(48.706329375,29.687500006828,1.293339198242E-14));
#10488=CARTESIAN_POINT('Ctrl Pts',(48.706329375,29.4791666734946,13.0508216223155));
#10489=CARTESIAN_POINT('Ctrl Pts',(42.1809185638422,29.2708333401613,24.3531646875));
#10490=CARTESIAN_POINT('Ctrl Pts',(35.6555077526845,29.062500006828,35.6555077526845));
#10491=CARTESIAN_POINT('Ctrl Pts',(24.3531646875,28.8541666734946,42.1809185638422));
#10492=CARTESIAN_POINT('Ctrl Pts',(13.0508216223155,28.6458333401613,48.706329375));
#10493=CARTESIAN_POINT('Ctrl Pts',(-9.95098946405443E-15,28.437500006828,
48.706329375));
#10494=CARTESIAN_POINT('Ctrl Pts',(-13.0508216223155,28.2291666734946,48.706329375));
#10495=CARTESIAN_POINT('Ctrl Pts',(-24.3531646875,28.0208333401613,42.1809185638423));
#10496=CARTESIAN_POINT('Ctrl Pts',(-35.6555077526845,27.812500006828,35.6555077526845));
#10497=CARTESIAN_POINT('Ctrl Pts',(-42.1809185638422,27.6041666734946,24.3531646875));
#10498=CARTESIAN_POINT('Ctrl Pts',(-48.706329375,27.3958333401613,13.0508216223155));
#10499=CARTESIAN_POINT('Ctrl Pts',(-48.706329375,27.187500006828,-1.8898197019151E-14));
#10500=CARTESIAN_POINT('',(-45.7957082162897,35.5508791552084,-4.33048599679673));
#10501=CARTESIAN_POINT('',(-3.42983911135813,34.4335524565479,-45.8719544348199));
#10502=CARTESIAN_POINT('Ctrl Pts',(-45.7957082162897,35.5508791552084,-4.33048599679673));
#10503=CARTESIAN_POINT('Ctrl Pts',(-44.8515840435634,35.3778446993657,-14.3147776366027));
#10504=CARTESIAN_POINT('Ctrl Pts',(-39.8371685740842,35.2083333469893,-23.));
#10505=CARTESIAN_POINT('Ctrl Pts',(-33.6743371481684,35.0000000136559,-33.6743371481684));
#10506=CARTESIAN_POINT('Ctrl Pts',(-23.,34.7916666803226,-39.8371685740842));
#10507=CARTESIAN_POINT('Ctrl Pts',(-13.903887812949,34.6141359029078,-45.0888113938571));
#10508=CARTESIAN_POINT('Ctrl Pts',(-3.42983911135813,34.4335524565479,-45.8719544348199));
#10509=CARTESIAN_POINT('',(-48.5134353784344,37.1175463684955,-4.33048599679682));
#10510=CARTESIAN_POINT('Ctrl Pts',(-45.7957082162897,35.5508791552084,-4.33048599679673));
#10511=CARTESIAN_POINT('Ctrl Pts',(-46.027322302781,35.6843839384496,-4.33048599679679));
#10512=CARTESIAN_POINT('Ctrl Pts',(-46.4905476657728,35.9513983799647,-4.33048599679657));
#10513=CARTESIAN_POINT('Ctrl Pts',(-46.9537676533565,36.2184221466352,-4.33048599679682));
#10514=CARTESIAN_POINT('Ctrl Pts',(-47.6280672732221,36.6071316973962,-4.33048599679682));
#10515=CARTESIAN_POINT('Ctrl Pts',(-48.0707534890442,36.8623352807796,-4.33048599679682));
#10516=CARTESIAN_POINT('Ctrl Pts',(-48.5134353784344,37.1175463684955,-4.33048599679682));
#10517=CARTESIAN_POINT('',(-4.2120577778781,36.0055185535964,-48.5238610423965));
#10518=CARTESIAN_POINT('Ctrl Pts',(-48.5134353784344,37.1175463684955,-4.33048599679682));
#10519=CARTESIAN_POINT('Ctrl Pts',(-47.5573898704235,36.9424850907232,-15.0408432190651));
#10520=CARTESIAN_POINT('Ctrl Pts',(-42.1809185638422,36.7708333401613,-24.3531646875));
#10521=CARTESIAN_POINT('Ctrl Pts',(-35.6555077526845,36.562500006828,-35.6555077526845));
#10522=CARTESIAN_POINT('Ctrl Pts',(-24.3531646875,36.3541666734946,-42.1809185638423));
#10523=CARTESIAN_POINT('Ctrl Pts',(-14.9868402884059,36.1815195000819,-47.5885684769766));
#10524=CARTESIAN_POINT('Ctrl Pts',(-4.2120577778781,36.0055185535964,-48.5238610423965));
#10525=CARTESIAN_POINT('Ctrl Pts',(-4.21205777787798,36.0055185535964,-48.5238610423965));
#10526=CARTESIAN_POINT('Ctrl Pts',(-4.14747432921768,35.7400881602412,-48.0687061610727));
#10527=CARTESIAN_POINT('Ctrl Pts',(-4.05341057734826,35.4727756853994,-47.6137074546591));
#10528=CARTESIAN_POINT('Ctrl Pts',(-3.79876998734544,34.948351505957,-46.7286766926143));
#10529=CARTESIAN_POINT('Ctrl Pts',(-3.63547301092605,34.6853692057132,-46.2887605423145));
#10530=CARTESIAN_POINT('Ctrl Pts',(-3.42983911135814,34.4335524565479,-45.87195443482));
#10531=CARTESIAN_POINT('Ctrl Pts',(-46.,55.6250000136559,0.));
#10532=CARTESIAN_POINT('Ctrl Pts',(-46.,55.4166666803226,-12.3256628518316));
#10533=CARTESIAN_POINT('Ctrl Pts',(-39.8371685740842,55.2083333469893,-23.));
#10534=CARTESIAN_POINT('Ctrl Pts',(-33.6743371481684,55.0000000136559,-33.6743371481684));
#10535=CARTESIAN_POINT('Ctrl Pts',(-23.,54.7916666803226,-39.8371685740842));
#10536=CARTESIAN_POINT('Ctrl Pts',(-12.3256628518317,54.5833333469893,-46.));
#10537=CARTESIAN_POINT('Ctrl Pts',(-2.81668763803891E-15,54.3750000136559,
-46.));
#10538=CARTESIAN_POINT('Ctrl Pts',(12.3256628518316,54.1666666803226,-46.));
#10539=CARTESIAN_POINT('Ctrl Pts',(23.,53.9583333469893,-39.8371685740842));
#10540=CARTESIAN_POINT('Ctrl Pts',(33.6743371481683,53.7500000136559,-33.6743371481684));
#10541=CARTESIAN_POINT('Ctrl Pts',(39.8371685740842,53.5416666803226,-23.));
#10542=CARTESIAN_POINT('Ctrl Pts',(46.,53.3333333469893,-12.3256628518317));
#10543=CARTESIAN_POINT('Ctrl Pts',(46.,53.1250000136559,-5.63337527607782E-15));
#10544=CARTESIAN_POINT('Ctrl Pts',(46.,52.9166666803226,12.3256628518316));
#10545=CARTESIAN_POINT('Ctrl Pts',(39.8371685740842,52.7083333469893,23.));
#10546=CARTESIAN_POINT('Ctrl Pts',(33.6743371481684,52.5000000136559,33.6743371481683));
#10547=CARTESIAN_POINT('Ctrl Pts',(23.,52.2916666803226,39.8371685740842));
#10548=CARTESIAN_POINT('Ctrl Pts',(12.3256628518317,52.0833333469893,46.));
#10549=CARTESIAN_POINT('Ctrl Pts',(8.45006291411674E-15,51.8750000136559,
46.));
#10550=CARTESIAN_POINT('Ctrl Pts',(-12.3256628518316,51.6666666803226,46.));
#10551=CARTESIAN_POINT('Ctrl Pts',(-23.,51.4583333469893,39.8371685740842));
#10552=CARTESIAN_POINT('Ctrl Pts',(-33.6743371481683,51.2500000136559,33.6743371481684));
#10553=CARTESIAN_POINT('Ctrl Pts',(-39.8371685740842,51.0416666803226,23.));
#10554=CARTESIAN_POINT('Ctrl Pts',(-46.,50.8333333469893,12.3256628518317));
#10555=CARTESIAN_POINT('Ctrl Pts',(-46.,50.6250000136559,0.));
#10556=CARTESIAN_POINT('Ctrl Pts',(-46.,50.4166666803226,-12.3256628518316));
#10557=CARTESIAN_POINT('Ctrl Pts',(-39.8371685740842,50.2083333469893,-23.));
#10558=CARTESIAN_POINT('Ctrl Pts',(-33.6743371481684,50.0000000136559,-33.6743371481684));
#10559=CARTESIAN_POINT('Ctrl Pts',(-23.,49.7916666803226,-39.8371685740842));
#10560=CARTESIAN_POINT('Ctrl Pts',(-12.3256628518317,49.5833333469893,-46.));
#10561=CARTESIAN_POINT('Ctrl Pts',(-2.81668763803891E-15,49.3750000136559,
-46.));
#10562=CARTESIAN_POINT('Ctrl Pts',(12.3256628518316,49.1666666803226,-46.));
#10563=CARTESIAN_POINT('Ctrl Pts',(23.,48.9583333469893,-39.8371685740842));
#10564=CARTESIAN_POINT('Ctrl Pts',(33.6743371481683,48.7500000136559,-33.6743371481684));
#10565=CARTESIAN_POINT('Ctrl Pts',(39.8371685740842,48.5416666803226,-23.));
#10566=CARTESIAN_POINT('Ctrl Pts',(46.,48.3333333469893,-12.3256628518317));
#10567=CARTESIAN_POINT('Ctrl Pts',(46.,48.1250000136559,-5.63337527607782E-15));
#10568=CARTESIAN_POINT('Ctrl Pts',(46.,47.9166666803226,12.3256628518316));
#10569=CARTESIAN_POINT('Ctrl Pts',(39.8371685740842,47.7083333469893,23.));
#10570=CARTESIAN_POINT('Ctrl Pts',(33.6743371481684,47.5000000136559,33.6743371481683));
#10571=CARTESIAN_POINT('Ctrl Pts',(23.,47.2916666803226,39.8371685740842));
#10572=CARTESIAN_POINT('Ctrl Pts',(12.3256628518317,47.0833333469893,46.));
#10573=CARTESIAN_POINT('Ctrl Pts',(8.45006291411674E-15,46.8750000136559,
46.));
#10574=CARTESIAN_POINT('Ctrl Pts',(-12.3256628518316,46.6666666803226,46.));
#10575=CARTESIAN_POINT('Ctrl Pts',(-23.,46.4583333469893,39.8371685740842));
#10576=CARTESIAN_POINT('Ctrl Pts',(-33.6743371481683,46.2500000136559,33.6743371481684));
#10577=CARTESIAN_POINT('Ctrl Pts',(-39.8371685740842,46.0416666803226,23.));
#10578=CARTESIAN_POINT('Ctrl Pts',(-46.,45.8333333469892,12.3256628518317));
#10579=CARTESIAN_POINT('Ctrl Pts',(-46.,45.6250000136559,0.));
#10580=CARTESIAN_POINT('Ctrl Pts',(-46.,45.4166666803226,-12.3256628518316));
#10581=CARTESIAN_POINT('Ctrl Pts',(-39.8371685740842,45.2083333469893,-23.));
#10582=CARTESIAN_POINT('Ctrl Pts',(-33.6743371481684,45.0000000136559,-33.6743371481684));
#10583=CARTESIAN_POINT('Ctrl Pts',(-23.,44.7916666803226,-39.8371685740842));
#10584=CARTESIAN_POINT('Ctrl Pts',(-12.3256628518317,44.5833333469893,-46.));
#10585=CARTESIAN_POINT('Ctrl Pts',(-2.81668763803891E-15,44.3750000136559,
-46.));
#10586=CARTESIAN_POINT('Ctrl Pts',(12.3256628518316,44.1666666803226,-46.));
#10587=CARTESIAN_POINT('Ctrl Pts',(23.,43.9583333469893,-39.8371685740842));
#10588=CARTESIAN_POINT('Ctrl Pts',(33.6743371481683,43.7500000136559,-33.6743371481684));
#10589=CARTESIAN_POINT('Ctrl Pts',(39.8371685740842,43.5416666803226,-23.));
#10590=CARTESIAN_POINT('Ctrl Pts',(46.,43.3333333469893,-12.3256628518317));
#10591=CARTESIAN_POINT('Ctrl Pts',(46.,43.1250000136559,-5.63337527607782E-15));
#10592=CARTESIAN_POINT('Ctrl Pts',(46.,42.9166666803226,12.3256628518316));
#10593=CARTESIAN_POINT('Ctrl Pts',(39.8371685740842,42.7083333469893,23.));
#10594=CARTESIAN_POINT('Ctrl Pts',(33.6743371481684,42.5000000136559,33.6743371481683));
#10595=CARTESIAN_POINT('Ctrl Pts',(23.,42.2916666803226,39.8371685740842));
#10596=CARTESIAN_POINT('Ctrl Pts',(12.3256628518317,42.0833333469893,46.));
#10597=CARTESIAN_POINT('Ctrl Pts',(8.45006291411674E-15,41.8750000136559,
46.));
#10598=CARTESIAN_POINT('Ctrl Pts',(-12.3256628518316,41.6666666803226,46.));
#10599=CARTESIAN_POINT('Ctrl Pts',(-23.,41.4583333469893,39.8371685740842));
#10600=CARTESIAN_POINT('Ctrl Pts',(-33.6743371481683,41.2500000136559,33.6743371481684));
#10601=CARTESIAN_POINT('Ctrl Pts',(-39.8371685740842,41.0416666803226,23.));
#10602=CARTESIAN_POINT('Ctrl Pts',(-46.,40.8333333469893,12.3256628518317));
#10603=CARTESIAN_POINT('Ctrl Pts',(-46.,40.6250000136559,0.));
#10604=CARTESIAN_POINT('Ctrl Pts',(-46.,40.4166666803226,-12.3256628518316));
#10605=CARTESIAN_POINT('Ctrl Pts',(-39.8371685740842,40.2083333469893,-23.));
#10606=CARTESIAN_POINT('Ctrl Pts',(-33.6743371481684,40.0000000136559,-33.6743371481684));
#10607=CARTESIAN_POINT('Ctrl Pts',(-23.,39.7916666803226,-39.8371685740842));
#10608=CARTESIAN_POINT('Ctrl Pts',(-12.3256628518317,39.5833333469893,-46.));
#10609=CARTESIAN_POINT('Ctrl Pts',(-2.81668763803891E-15,39.3750000136559,
-46.));
#10610=CARTESIAN_POINT('Ctrl Pts',(12.3256628518316,39.1666666803226,-46.));
#10611=CARTESIAN_POINT('Ctrl Pts',(23.,38.9583333469893,-39.8371685740842));
#10612=CARTESIAN_POINT('Ctrl Pts',(33.6743371481683,38.7500000136559,-33.6743371481684));
#10613=CARTESIAN_POINT('Ctrl Pts',(39.8371685740842,38.5416666803226,-23.));
#10614=CARTESIAN_POINT('Ctrl Pts',(46.,38.3333333469893,-12.3256628518317));
#10615=CARTESIAN_POINT('Ctrl Pts',(46.,38.1250000136559,-5.63337527607782E-15));
#10616=CARTESIAN_POINT('Ctrl Pts',(46.,37.9166666803226,12.3256628518316));
#10617=CARTESIAN_POINT('Ctrl Pts',(39.8371685740842,37.7083333469893,23.));
#10618=CARTESIAN_POINT('Ctrl Pts',(33.6743371481684,37.5000000136559,33.6743371481683));
#10619=CARTESIAN_POINT('Ctrl Pts',(23.,37.2916666803226,39.8371685740842));
#10620=CARTESIAN_POINT('Ctrl Pts',(12.3256628518317,37.0833333469893,46.));
#10621=CARTESIAN_POINT('Ctrl Pts',(8.45006291411674E-15,36.8750000136559,
46.));
#10622=CARTESIAN_POINT('Ctrl Pts',(-12.3256628518316,36.6666666803226,46.));
#10623=CARTESIAN_POINT('Ctrl Pts',(-23.,36.4583333469893,39.8371685740842));
#10624=CARTESIAN_POINT('Ctrl Pts',(-33.6743371481683,36.2500000136559,33.6743371481684));
#10625=CARTESIAN_POINT('Ctrl Pts',(-39.8371685740842,36.0416666803226,23.));
#10626=CARTESIAN_POINT('Ctrl Pts',(-46.,35.8333333469893,12.3256628518317));
#10627=CARTESIAN_POINT('Ctrl Pts',(-46.,35.6250000136559,0.));
#10628=CARTESIAN_POINT('Ctrl Pts',(-46.,35.4166666803226,-12.3256628518316));
#10629=CARTESIAN_POINT('Ctrl Pts',(-39.8371685740842,35.2083333469893,-23.));
#10630=CARTESIAN_POINT('Ctrl Pts',(-33.6743371481684,35.0000000136559,-33.6743371481684));
#10631=CARTESIAN_POINT('Ctrl Pts',(-23.,34.7916666803226,-39.8371685740842));
#10632=CARTESIAN_POINT('Ctrl Pts',(-12.3256628518317,34.5833333469893,-46.));
#10633=CARTESIAN_POINT('Ctrl Pts',(-2.81668763803891E-15,34.3750000136559,
-46.));
#10634=CARTESIAN_POINT('Ctrl Pts',(12.3256628518316,34.1666666803226,-46.));
#10635=CARTESIAN_POINT('Ctrl Pts',(23.,33.9583333469893,-39.8371685740842));
#10636=CARTESIAN_POINT('Ctrl Pts',(33.6743371481683,33.7500000136559,-33.6743371481684));
#10637=CARTESIAN_POINT('Ctrl Pts',(39.8371685740842,33.5416666803226,-23.));
#10638=CARTESIAN_POINT('Ctrl Pts',(46.,33.3333333469893,-12.3256628518317));
#10639=CARTESIAN_POINT('Ctrl Pts',(46.,33.1250000136559,-5.63337527607782E-15));
#10640=CARTESIAN_POINT('Ctrl Pts',(46.,32.9166666803226,12.3256628518316));
#10641=CARTESIAN_POINT('Ctrl Pts',(39.8371685740842,32.7083333469893,23.));
#10642=CARTESIAN_POINT('Ctrl Pts',(33.6743371481684,32.5000000136559,33.6743371481683));
#10643=CARTESIAN_POINT('Ctrl Pts',(23.,32.2916666803226,39.8371685740842));
#10644=CARTESIAN_POINT('Ctrl Pts',(12.3256628518317,32.0833333469893,46.));
#10645=CARTESIAN_POINT('Ctrl Pts',(8.45006291411674E-15,31.8750000136559,
46.));
#10646=CARTESIAN_POINT('Ctrl Pts',(-12.3256628518316,31.6666666803226,46.));
#10647=CARTESIAN_POINT('Ctrl Pts',(-23.,31.4583333469893,39.8371685740842));
#10648=CARTESIAN_POINT('Ctrl Pts',(-33.6743371481683,31.2500000136559,33.6743371481684));
#10649=CARTESIAN_POINT('Ctrl Pts',(-39.8371685740842,31.0416666803226,23.));
#10650=CARTESIAN_POINT('Ctrl Pts',(-46.,30.8333333469893,12.3256628518317));
#10651=CARTESIAN_POINT('Ctrl Pts',(-46.,30.6250000136559,0.));
#10652=CARTESIAN_POINT('Ctrl Pts',(-46.,30.4166666803226,-12.3256628518316));
#10653=CARTESIAN_POINT('Ctrl Pts',(-39.8371685740842,30.2083333469893,-23.));
#10654=CARTESIAN_POINT('Ctrl Pts',(-33.6743371481684,30.0000000136559,-33.6743371481684));
#10655=CARTESIAN_POINT('Ctrl Pts',(-23.,29.7916666803226,-39.8371685740842));
#10656=CARTESIAN_POINT('Ctrl Pts',(-12.3256628518317,29.5833333469893,-46.));
#10657=CARTESIAN_POINT('Ctrl Pts',(-2.81668763803891E-15,29.3750000136559,
-46.));
#10658=CARTESIAN_POINT('Ctrl Pts',(12.3256628518316,29.1666666803226,-46.));
#10659=CARTESIAN_POINT('Ctrl Pts',(23.,28.9583333469893,-39.8371685740842));
#10660=CARTESIAN_POINT('Ctrl Pts',(33.6743371481683,28.7500000136559,-33.6743371481684));
#10661=CARTESIAN_POINT('Ctrl Pts',(39.8371685740842,28.5416666803226,-23.));
#10662=CARTESIAN_POINT('Ctrl Pts',(46.,28.3333333469893,-12.3256628518317));
#10663=CARTESIAN_POINT('Ctrl Pts',(46.,28.1250000136559,-5.63337527607782E-15));
#10664=CARTESIAN_POINT('Ctrl Pts',(46.,27.9166666803226,12.3256628518316));
#10665=CARTESIAN_POINT('Ctrl Pts',(39.8371685740842,27.7083333469893,23.));
#10666=CARTESIAN_POINT('Ctrl Pts',(33.6743371481684,27.5000000136559,33.6743371481683));
#10667=CARTESIAN_POINT('Ctrl Pts',(23.,27.2916666803226,39.8371685740842));
#10668=CARTESIAN_POINT('Ctrl Pts',(12.3256628518317,27.0833333469893,46.));
#10669=CARTESIAN_POINT('Ctrl Pts',(8.45006291411674E-15,26.8750000136559,
46.));
#10670=CARTESIAN_POINT('Ctrl Pts',(-12.3256628518316,26.6666666803226,46.));
#10671=CARTESIAN_POINT('Ctrl Pts',(-23.,26.4583333469893,39.8371685740842));
#10672=CARTESIAN_POINT('Ctrl Pts',(-33.6743371481683,26.2500000136559,33.6743371481684));
#10673=CARTESIAN_POINT('Ctrl Pts',(-39.8371685740842,26.0416666803226,23.));
#10674=CARTESIAN_POINT('Ctrl Pts',(-46.,25.8333333469893,12.3256628518317));
#10675=CARTESIAN_POINT('Ctrl Pts',(-46.,25.6250000136559,0.));
#10676=CARTESIAN_POINT('Ctrl Pts',(-48.706329375,57.187500006828,-1.8898197019151E-14));
#10677=CARTESIAN_POINT('Ctrl Pts',(-48.706329375,56.9791666734946,-13.0508216223155));
#10678=CARTESIAN_POINT('Ctrl Pts',(-42.1809185638422,56.7708333401613,-24.3531646875));
#10679=CARTESIAN_POINT('Ctrl Pts',(-35.6555077526845,56.562500006828,-35.6555077526845));
#10680=CARTESIAN_POINT('Ctrl Pts',(-24.3531646875,56.3541666734946,-42.1809185638423));
#10681=CARTESIAN_POINT('Ctrl Pts',(-13.0508216223155,56.1458333401613,-48.706329375));
#10682=CARTESIAN_POINT('Ctrl Pts',(1.59157945007855E-14,55.937500006828,
-48.706329375));
#10683=CARTESIAN_POINT('Ctrl Pts',(13.0508216223155,55.7291666734946,-48.706329375));
#10684=CARTESIAN_POINT('Ctrl Pts',(24.3531646875,55.5208333401613,-42.1809185638422));
#10685=CARTESIAN_POINT('Ctrl Pts',(35.6555077526845,55.312500006828,-35.6555077526845));
#10686=CARTESIAN_POINT('Ctrl Pts',(42.1809185638422,55.1041666734946,-24.3531646875));
#10687=CARTESIAN_POINT('Ctrl Pts',(48.706329375,54.8958333401613,-13.0508216223155));
#10688=CARTESIAN_POINT('Ctrl Pts',(48.706329375,54.687500006828,1.293339198242E-14));
#10689=CARTESIAN_POINT('Ctrl Pts',(48.706329375,54.4791666734946,13.0508216223155));
#10690=CARTESIAN_POINT('Ctrl Pts',(42.1809185638422,54.2708333401613,24.3531646875));
#10691=CARTESIAN_POINT('Ctrl Pts',(35.6555077526845,54.062500006828,35.6555077526845));
#10692=CARTESIAN_POINT('Ctrl Pts',(24.3531646875,53.8541666734946,42.1809185638422));
#10693=CARTESIAN_POINT('Ctrl Pts',(13.0508216223155,53.6458333401613,48.706329375));
#10694=CARTESIAN_POINT('Ctrl Pts',(-9.95098946405443E-15,53.437500006828,
48.706329375));
#10695=CARTESIAN_POINT('Ctrl Pts',(-13.0508216223155,53.2291666734946,48.706329375));
#10696=CARTESIAN_POINT('Ctrl Pts',(-24.3531646875,53.0208333401613,42.1809185638423));
#10697=CARTESIAN_POINT('Ctrl Pts',(-35.6555077526845,52.812500006828,35.6555077526845));
#10698=CARTESIAN_POINT('Ctrl Pts',(-42.1809185638422,52.6041666734946,24.3531646875));
#10699=CARTESIAN_POINT('Ctrl Pts',(-48.706329375,52.3958333401613,13.0508216223155));
#10700=CARTESIAN_POINT('Ctrl Pts',(-48.706329375,52.187500006828,-1.8898197019151E-14));
#10701=CARTESIAN_POINT('Ctrl Pts',(-48.706329375,51.9791666734946,-13.0508216223155));
#10702=CARTESIAN_POINT('Ctrl Pts',(-42.1809185638422,51.7708333401613,-24.3531646875));
#10703=CARTESIAN_POINT('Ctrl Pts',(-35.6555077526845,51.562500006828,-35.6555077526845));
#10704=CARTESIAN_POINT('Ctrl Pts',(-24.3531646875,51.3541666734946,-42.1809185638423));
#10705=CARTESIAN_POINT('Ctrl Pts',(-13.0508216223155,51.1458333401613,-48.706329375));
#10706=CARTESIAN_POINT('Ctrl Pts',(1.59157945007855E-14,50.937500006828,
-48.706329375));
#10707=CARTESIAN_POINT('Ctrl Pts',(13.0508216223155,50.7291666734946,-48.706329375));
#10708=CARTESIAN_POINT('Ctrl Pts',(24.3531646875,50.5208333401613,-42.1809185638422));
#10709=CARTESIAN_POINT('Ctrl Pts',(35.6555077526845,50.312500006828,-35.6555077526845));
#10710=CARTESIAN_POINT('Ctrl Pts',(42.1809185638422,50.1041666734946,-24.3531646875));
#10711=CARTESIAN_POINT('Ctrl Pts',(48.706329375,49.8958333401613,-13.0508216223155));
#10712=CARTESIAN_POINT('Ctrl Pts',(48.706329375,49.687500006828,1.293339198242E-14));
#10713=CARTESIAN_POINT('Ctrl Pts',(48.706329375,49.4791666734946,13.0508216223155));
#10714=CARTESIAN_POINT('Ctrl Pts',(42.1809185638422,49.2708333401613,24.3531646875));
#10715=CARTESIAN_POINT('Ctrl Pts',(35.6555077526845,49.062500006828,35.6555077526845));
#10716=CARTESIAN_POINT('Ctrl Pts',(24.3531646875,48.8541666734946,42.1809185638422));
#10717=CARTESIAN_POINT('Ctrl Pts',(13.0508216223155,48.6458333401613,48.706329375));
#10718=CARTESIAN_POINT('Ctrl Pts',(-9.95098946405443E-15,48.437500006828,
48.706329375));
#10719=CARTESIAN_POINT('Ctrl Pts',(-13.0508216223155,48.2291666734946,48.706329375));
#10720=CARTESIAN_POINT('Ctrl Pts',(-24.3531646875,48.0208333401613,42.1809185638423));
#10721=CARTESIAN_POINT('Ctrl Pts',(-35.6555077526845,47.812500006828,35.6555077526845));
#10722=CARTESIAN_POINT('Ctrl Pts',(-42.1809185638422,47.6041666734946,24.3531646875));
#10723=CARTESIAN_POINT('Ctrl Pts',(-48.706329375,47.3958333401613,13.0508216223155));
#10724=CARTESIAN_POINT('Ctrl Pts',(-48.706329375,47.187500006828,-1.8898197019151E-14));
#10725=CARTESIAN_POINT('Ctrl Pts',(-48.706329375,46.9791666734946,-13.0508216223155));
#10726=CARTESIAN_POINT('Ctrl Pts',(-42.1809185638422,46.7708333401613,-24.3531646875));
#10727=CARTESIAN_POINT('Ctrl Pts',(-35.6555077526845,46.562500006828,-35.6555077526845));
#10728=CARTESIAN_POINT('Ctrl Pts',(-24.3531646875,46.3541666734946,-42.1809185638423));
#10729=CARTESIAN_POINT('Ctrl Pts',(-13.0508216223155,46.1458333401613,-48.706329375));
#10730=CARTESIAN_POINT('Ctrl Pts',(1.59157945007855E-14,45.937500006828,
-48.706329375));
#10731=CARTESIAN_POINT('Ctrl Pts',(13.0508216223155,45.7291666734946,-48.706329375));
#10732=CARTESIAN_POINT('Ctrl Pts',(24.3531646875,45.5208333401613,-42.1809185638422));
#10733=CARTESIAN_POINT('Ctrl Pts',(35.6555077526845,45.312500006828,-35.6555077526845));
#10734=CARTESIAN_POINT('Ctrl Pts',(42.1809185638422,45.1041666734946,-24.3531646875));
#10735=CARTESIAN_POINT('Ctrl Pts',(48.706329375,44.8958333401613,-13.0508216223155));
#10736=CARTESIAN_POINT('Ctrl Pts',(48.706329375,44.687500006828,1.293339198242E-14));
#10737=CARTESIAN_POINT('Ctrl Pts',(48.706329375,44.4791666734946,13.0508216223155));
#10738=CARTESIAN_POINT('Ctrl Pts',(42.1809185638422,44.2708333401613,24.3531646875));
#10739=CARTESIAN_POINT('Ctrl Pts',(35.6555077526845,44.062500006828,35.6555077526845));
#10740=CARTESIAN_POINT('Ctrl Pts',(24.3531646875,43.8541666734946,42.1809185638422));
#10741=CARTESIAN_POINT('Ctrl Pts',(13.0508216223155,43.6458333401613,48.706329375));
#10742=CARTESIAN_POINT('Ctrl Pts',(-9.95098946405443E-15,43.437500006828,
48.706329375));
#10743=CARTESIAN_POINT('Ctrl Pts',(-13.0508216223155,43.2291666734946,48.706329375));
#10744=CARTESIAN_POINT('Ctrl Pts',(-24.3531646875,43.0208333401613,42.1809185638423));
#10745=CARTESIAN_POINT('Ctrl Pts',(-35.6555077526845,42.812500006828,35.6555077526845));
#10746=CARTESIAN_POINT('Ctrl Pts',(-42.1809185638422,42.6041666734946,24.3531646875));
#10747=CARTESIAN_POINT('Ctrl Pts',(-48.706329375,42.3958333401613,13.0508216223155));
#10748=CARTESIAN_POINT('Ctrl Pts',(-48.706329375,42.187500006828,-1.8898197019151E-14));
#10749=CARTESIAN_POINT('Ctrl Pts',(-48.706329375,41.9791666734946,-13.0508216223155));
#10750=CARTESIAN_POINT('Ctrl Pts',(-42.1809185638422,41.7708333401613,-24.3531646875));
#10751=CARTESIAN_POINT('Ctrl Pts',(-35.6555077526845,41.562500006828,-35.6555077526845));
#10752=CARTESIAN_POINT('Ctrl Pts',(-24.3531646875,41.3541666734946,-42.1809185638423));
#10753=CARTESIAN_POINT('Ctrl Pts',(-13.0508216223155,41.1458333401613,-48.706329375));
#10754=CARTESIAN_POINT('Ctrl Pts',(1.59157945007855E-14,40.937500006828,
-48.706329375));
#10755=CARTESIAN_POINT('Ctrl Pts',(13.0508216223155,40.7291666734946,-48.706329375));
#10756=CARTESIAN_POINT('Ctrl Pts',(24.3531646875,40.5208333401613,-42.1809185638422));
#10757=CARTESIAN_POINT('Ctrl Pts',(35.6555077526845,40.312500006828,-35.6555077526845));
#10758=CARTESIAN_POINT('Ctrl Pts',(42.1809185638422,40.1041666734946,-24.3531646875));
#10759=CARTESIAN_POINT('Ctrl Pts',(48.706329375,39.8958333401613,-13.0508216223155));
#10760=CARTESIAN_POINT('Ctrl Pts',(48.706329375,39.687500006828,1.293339198242E-14));
#10761=CARTESIAN_POINT('Ctrl Pts',(48.706329375,39.4791666734946,13.0508216223155));
#10762=CARTESIAN_POINT('Ctrl Pts',(42.1809185638422,39.2708333401613,24.3531646875));
#10763=CARTESIAN_POINT('Ctrl Pts',(35.6555077526845,39.062500006828,35.6555077526845));
#10764=CARTESIAN_POINT('Ctrl Pts',(24.3531646875,38.8541666734946,42.1809185638422));
#10765=CARTESIAN_POINT('Ctrl Pts',(13.0508216223155,38.6458333401613,48.706329375));
#10766=CARTESIAN_POINT('Ctrl Pts',(-9.95098946405443E-15,38.437500006828,
48.706329375));
#10767=CARTESIAN_POINT('Ctrl Pts',(-13.0508216223155,38.2291666734946,48.706329375));
#10768=CARTESIAN_POINT('Ctrl Pts',(-24.3531646875,38.0208333401613,42.1809185638423));
#10769=CARTESIAN_POINT('Ctrl Pts',(-35.6555077526845,37.812500006828,35.6555077526845));
#10770=CARTESIAN_POINT('Ctrl Pts',(-42.1809185638422,37.6041666734946,24.3531646875));
#10771=CARTESIAN_POINT('Ctrl Pts',(-48.706329375,37.3958333401613,13.0508216223155));
#10772=CARTESIAN_POINT('Ctrl Pts',(-48.706329375,37.187500006828,-1.8898197019151E-14));
#10773=CARTESIAN_POINT('Ctrl Pts',(-48.706329375,36.9791666734946,-13.0508216223155));
#10774=CARTESIAN_POINT('Ctrl Pts',(-42.1809185638422,36.7708333401613,-24.3531646875));
#10775=CARTESIAN_POINT('Ctrl Pts',(-35.6555077526845,36.562500006828,-35.6555077526845));
#10776=CARTESIAN_POINT('Ctrl Pts',(-24.3531646875,36.3541666734946,-42.1809185638423));
#10777=CARTESIAN_POINT('Ctrl Pts',(-13.0508216223155,36.1458333401613,-48.706329375));
#10778=CARTESIAN_POINT('Ctrl Pts',(1.59157945007855E-14,35.937500006828,
-48.706329375));
#10779=CARTESIAN_POINT('Ctrl Pts',(13.0508216223155,35.7291666734946,-48.706329375));
#10780=CARTESIAN_POINT('Ctrl Pts',(24.3531646875,35.5208333401613,-42.1809185638422));
#10781=CARTESIAN_POINT('Ctrl Pts',(35.6555077526845,35.312500006828,-35.6555077526845));
#10782=CARTESIAN_POINT('Ctrl Pts',(42.1809185638422,35.1041666734946,-24.3531646875));
#10783=CARTESIAN_POINT('Ctrl Pts',(48.706329375,34.8958333401613,-13.0508216223155));
#10784=CARTESIAN_POINT('Ctrl Pts',(48.706329375,34.687500006828,1.293339198242E-14));
#10785=CARTESIAN_POINT('Ctrl Pts',(48.706329375,34.4791666734946,13.0508216223155));
#10786=CARTESIAN_POINT('Ctrl Pts',(42.1809185638422,34.2708333401613,24.3531646875));
#10787=CARTESIAN_POINT('Ctrl Pts',(35.6555077526845,34.062500006828,35.6555077526845));
#10788=CARTESIAN_POINT('Ctrl Pts',(24.3531646875,33.8541666734946,42.1809185638422));
#10789=CARTESIAN_POINT('Ctrl Pts',(13.0508216223155,33.6458333401613,48.706329375));
#10790=CARTESIAN_POINT('Ctrl Pts',(-9.95098946405443E-15,33.437500006828,
48.706329375));
#10791=CARTESIAN_POINT('Ctrl Pts',(-13.0508216223155,33.2291666734946,48.706329375));
#10792=CARTESIAN_POINT('Ctrl Pts',(-24.3531646875,33.0208333401613,42.1809185638423));
#10793=CARTESIAN_POINT('Ctrl Pts',(-35.6555077526845,32.812500006828,35.6555077526845));
#10794=CARTESIAN_POINT('Ctrl Pts',(-42.1809185638422,32.6041666734946,24.3531646875));
#10795=CARTESIAN_POINT('Ctrl Pts',(-48.706329375,32.3958333401613,13.0508216223155));
#10796=CARTESIAN_POINT('Ctrl Pts',(-48.706329375,32.187500006828,-1.8898197019151E-14));
#10797=CARTESIAN_POINT('Ctrl Pts',(-48.706329375,31.9791666734946,-13.0508216223155));
#10798=CARTESIAN_POINT('Ctrl Pts',(-42.1809185638422,31.7708333401613,-24.3531646875));
#10799=CARTESIAN_POINT('Ctrl Pts',(-35.6555077526845,31.562500006828,-35.6555077526845));
#10800=CARTESIAN_POINT('Ctrl Pts',(-24.3531646875,31.3541666734946,-42.1809185638423));
#10801=CARTESIAN_POINT('Ctrl Pts',(-13.0508216223155,31.1458333401613,-48.706329375));
#10802=CARTESIAN_POINT('Ctrl Pts',(1.59157945007855E-14,30.937500006828,
-48.706329375));
#10803=CARTESIAN_POINT('Ctrl Pts',(13.0508216223155,30.7291666734946,-48.706329375));
#10804=CARTESIAN_POINT('Ctrl Pts',(24.3531646875,30.5208333401613,-42.1809185638422));
#10805=CARTESIAN_POINT('Ctrl Pts',(35.6555077526845,30.312500006828,-35.6555077526845));
#10806=CARTESIAN_POINT('Ctrl Pts',(42.1809185638422,30.1041666734946,-24.3531646875));
#10807=CARTESIAN_POINT('Ctrl Pts',(48.706329375,29.8958333401613,-13.0508216223155));
#10808=CARTESIAN_POINT('Ctrl Pts',(48.706329375,29.687500006828,1.293339198242E-14));
#10809=CARTESIAN_POINT('Ctrl Pts',(48.706329375,29.4791666734946,13.0508216223155));
#10810=CARTESIAN_POINT('Ctrl Pts',(42.1809185638422,29.2708333401613,24.3531646875));
#10811=CARTESIAN_POINT('Ctrl Pts',(35.6555077526845,29.062500006828,35.6555077526845));
#10812=CARTESIAN_POINT('Ctrl Pts',(24.3531646875,28.8541666734946,42.1809185638422));
#10813=CARTESIAN_POINT('Ctrl Pts',(13.0508216223155,28.6458333401613,48.706329375));
#10814=CARTESIAN_POINT('Ctrl Pts',(-9.95098946405443E-15,28.437500006828,
48.706329375));
#10815=CARTESIAN_POINT('Ctrl Pts',(-13.0508216223155,28.2291666734946,48.706329375));
#10816=CARTESIAN_POINT('Ctrl Pts',(-24.3531646875,28.0208333401613,42.1809185638423));
#10817=CARTESIAN_POINT('Ctrl Pts',(-35.6555077526845,27.812500006828,35.6555077526845));
#10818=CARTESIAN_POINT('Ctrl Pts',(-42.1809185638422,27.6041666734946,24.3531646875));
#10819=CARTESIAN_POINT('Ctrl Pts',(-48.706329375,27.3958333401613,13.0508216223155));
#10820=CARTESIAN_POINT('Ctrl Pts',(-48.706329375,27.187500006828,-1.8898197019151E-14));
#10821=CARTESIAN_POINT('',(-4.32456003949875,38.3676432269777,48.5139639861634));
#10822=CARTESIAN_POINT('',(-48.5725845633798,37.2456516907297,3.60701400320327));
#10823=CARTESIAN_POINT('Ctrl Pts',(-4.32456003949875,38.3676432269777,48.5139639861634));
#10824=CARTESIAN_POINT('Ctrl Pts',(-15.038141415499,38.1925348924095,47.5589497574396));
#10825=CARTESIAN_POINT('Ctrl Pts',(-24.3531646875,38.0208333401613,42.1809185638423));
#10826=CARTESIAN_POINT('Ctrl Pts',(-35.6555077526845,37.812500006828,35.6555077526845));
#10827=CARTESIAN_POINT('Ctrl Pts',(-42.1809185638422,37.6041666734946,24.3531646875));
#10828=CARTESIAN_POINT('Ctrl Pts',(-47.7480251419552,37.4264286116308,14.7106532430575));
#10829=CARTESIAN_POINT('Ctrl Pts',(-48.5725845633798,37.2456516907297,3.60701400320327));
#10830=CARTESIAN_POINT('',(-45.858362923034,35.686608693912,3.60701400320327));
#10831=CARTESIAN_POINT('Ctrl Pts',(-48.5725845633798,37.2456516907297,3.60701400320327));
#10832=CARTESIAN_POINT('Ctrl Pts',(-48.3407853679392,37.1124685639422,3.60701400320327));
#10833=CARTESIAN_POINT('Ctrl Pts',(-48.1089821836664,36.9792923792741,3.60701400320327));
#10834=CARTESIAN_POINT('Ctrl Pts',(-47.6453674864979,36.7129545080418,3.60701400320327));
#10835=CARTESIAN_POINT('Ctrl Pts',(-47.4135559734254,36.5797928212585,3.60701400320327));
#10836=CARTESIAN_POINT('Ctrl Pts',(-47.1817401099609,36.4466387085919,3.60701400320327));
#10837=CARTESIAN_POINT('Ctrl Pts',(-46.7406305897488,36.1932671494809,3.60701400320327));
#10838=CARTESIAN_POINT('Ctrl Pts',(-46.2995053259033,35.9399229970588,3.60701400320328));
#10839=CARTESIAN_POINT('Ctrl Pts',(-45.858362923034,35.686608693912,3.60701400320327));
#10840=CARTESIAN_POINT('',(-4.32199731091469,36.8010262662206,45.796510120799));
#10841=CARTESIAN_POINT('Ctrl Pts',(-4.32199731091469,36.8010262662206,45.796510120799));
#10842=CARTESIAN_POINT('Ctrl Pts',(-14.3109099936784,36.6279201849842,44.8538170282468));
#10843=CARTESIAN_POINT('Ctrl Pts',(-23.,36.4583333469893,39.8371685740842));
#10844=CARTESIAN_POINT('Ctrl Pts',(-33.6743371481683,36.2500000136559,33.6743371481684));
#10845=CARTESIAN_POINT('Ctrl Pts',(-39.8371685740842,36.0416666803226,23.));
#10846=CARTESIAN_POINT('Ctrl Pts',(-45.0420919829705,35.8657152436245,13.9848082063043));
#10847=CARTESIAN_POINT('Ctrl Pts',(-45.858362923034,35.686608693912,3.60701400320327));
#10848=CARTESIAN_POINT('',(-4.32456320853981,36.9438035983166,46.0440414573356));
#10849=CARTESIAN_POINT('Origin',(11.5422763248982,36.5066019508688,46.295943288233));
#10850=CARTESIAN_POINT('Ctrl Pts',(-4.32456003949885,36.9438034227513,46.0440415585359));
#10851=CARTESIAN_POINT('Ctrl Pts',(-4.32456003949885,37.1552503030329,46.4108661087096));
#10852=CARTESIAN_POINT('Ctrl Pts',(-4.32456003949594,37.3667894036306,46.7778368059273));
#10853=CARTESIAN_POINT('Ctrl Pts',(-4.32456003949594,37.8413187510542,47.6010049167753));
#10854=CARTESIAN_POINT('Ctrl Pts',(-4.32456003949875,38.1045569543834,48.057625392756));
#10855=CARTESIAN_POINT('Ctrl Pts',(-4.32456003949875,38.3676432269777,48.5139639861634));
#10856=CARTESIAN_POINT('Origin',(-7.99360577730113E-14,57.8125000068276,
4.34631818602828E-14));
#10857=CARTESIAN_POINT('',(3.61292728433799,57.1292520480092,-48.5721450795008));
#10858=CARTESIAN_POINT('',(48.5134353784344,56.0074536451604,-4.33048599679673));
#10859=CARTESIAN_POINT('Ctrl Pts',(3.61292728433799,57.1292520480093,-48.5721450795008));
#10860=CARTESIAN_POINT('Ctrl Pts',(14.7133549689477,56.9485216017707,-47.7464652997852));
#10861=CARTESIAN_POINT('Ctrl Pts',(24.3531646875,56.7708333401613,-42.1809185638422));
#10862=CARTESIAN_POINT('Ctrl Pts',(35.6555077526845,56.562500006828,-35.6555077526845));
#10863=CARTESIAN_POINT('Ctrl Pts',(42.1809185638422,56.3541666734946,-24.3531646875));
#10864=CARTESIAN_POINT('Ctrl Pts',(47.5573898704235,56.1825149229327,-15.0408432190651));
#10865=CARTESIAN_POINT('Ctrl Pts',(48.5134353784344,56.0074536451604,-4.33048599679673));
#10866=CARTESIAN_POINT('',(48.5134353784344,56.0074536451604,-4.33048599679673));
#10867=CARTESIAN_POINT('',(3.61292728433799,55.8792520480092,-48.5721450795008));
#10868=CARTESIAN_POINT('Origin',(-7.99360577730113E-14,57.8125000068276,
4.34631818602828E-14));
#10869=CARTESIAN_POINT('',(48.5725845633798,55.8793483229262,3.60701400320328));
#10870=CARTESIAN_POINT('',(48.5725845633798,54.6293483229262,3.60701400320328));
#10871=CARTESIAN_POINT('',(3.612927284338,54.7457479656467,48.5721450795008));
#10872=CARTESIAN_POINT('Ctrl Pts',(48.5725845633798,55.8793483229262,3.60701400320328));
#10873=CARTESIAN_POINT('Ctrl Pts',(47.7480251419552,55.6985714020251,14.7106532430575));
#10874=CARTESIAN_POINT('Ctrl Pts',(42.1809185638422,55.5208333401613,24.3531646875));
#10875=CARTESIAN_POINT('Ctrl Pts',(35.6555077526845,55.312500006828,35.6555077526845));
#10876=CARTESIAN_POINT('Ctrl Pts',(24.3531646875,55.1041666734946,42.1809185638422));
#10877=CARTESIAN_POINT('Ctrl Pts',(14.7133549689477,54.9264784118853,47.7464652997852));
#10878=CARTESIAN_POINT('Ctrl Pts',(3.612927284338,54.7457479656467,48.5721450795008));
#10879=CARTESIAN_POINT('',(3.612927284338,54.7457479656467,48.5721450795008));
#10880=CARTESIAN_POINT('Origin',(-7.99360577730113E-14,57.8125000068276,
4.34631818602828E-14));
#10881=CARTESIAN_POINT('',(3.612927284338,52.1292520480092,-48.5721450795008));
#10882=CARTESIAN_POINT('',(48.5134353784344,51.0074536451604,-4.33048599679671));
#10883=CARTESIAN_POINT('Ctrl Pts',(3.612927284338,52.1292520480092,-48.5721450795008));
#10884=CARTESIAN_POINT('Ctrl Pts',(14.7133549689477,51.9485216017707,-47.7464652997852));
#10885=CARTESIAN_POINT('Ctrl Pts',(24.3531646875,51.7708333401613,-42.1809185638422));
#10886=CARTESIAN_POINT('Ctrl Pts',(35.6555077526845,51.562500006828,-35.6555077526845));
#10887=CARTESIAN_POINT('Ctrl Pts',(42.1809185638422,51.3541666734946,-24.3531646875));
#10888=CARTESIAN_POINT('Ctrl Pts',(47.5573898704235,51.1825149229327,-15.0408432190651));
#10889=CARTESIAN_POINT('Ctrl Pts',(48.5134353784344,51.0074536451604,-4.33048599679671));
#10890=CARTESIAN_POINT('',(48.5134353784344,51.0074536451604,-4.33048599679671));
#10891=CARTESIAN_POINT('',(3.612927284338,50.8792520480092,-48.5721450795008));
#10892=CARTESIAN_POINT('Origin',(-7.99360577730113E-14,57.8125000068276,
4.34631818602828E-14));
#10893=CARTESIAN_POINT('',(48.5725845633798,50.8793483229262,3.60701400320328));
#10894=CARTESIAN_POINT('',(48.5725845633798,49.6293483229262,3.60701400320328));
#10895=CARTESIAN_POINT('',(3.61292728433797,49.7457479656467,48.5721450795008));
#10896=CARTESIAN_POINT('Ctrl Pts',(48.5725845633798,50.8793483229262,3.60701400320328));
#10897=CARTESIAN_POINT('Ctrl Pts',(47.7480251419552,50.6985714020251,14.7106532430575));
#10898=CARTESIAN_POINT('Ctrl Pts',(42.1809185638422,50.5208333401613,24.3531646875));
#10899=CARTESIAN_POINT('Ctrl Pts',(35.6555077526845,50.312500006828,35.6555077526845));
#10900=CARTESIAN_POINT('Ctrl Pts',(24.3531646875,50.1041666734946,42.1809185638422));
#10901=CARTESIAN_POINT('Ctrl Pts',(14.7133549689477,49.9264784118853,47.7464652997852));
#10902=CARTESIAN_POINT('Ctrl Pts',(3.61292728433797,49.7457479656467,48.5721450795008));
#10903=CARTESIAN_POINT('',(3.61292728433797,49.7457479656467,48.5721450795008));
#10904=CARTESIAN_POINT('Origin',(-7.99360577730113E-14,57.8125000068276,
4.34631818602828E-14));
#10905=CARTESIAN_POINT('',(3.61292728433799,47.1292520480092,-48.5721450795008));
#10906=CARTESIAN_POINT('',(48.5134353784344,46.0074536451604,-4.33048599679671));
#10907=CARTESIAN_POINT('Ctrl Pts',(3.61292728433799,47.1292520480092,-48.5721450795008));
#10908=CARTESIAN_POINT('Ctrl Pts',(14.7133549689477,46.9485216017706,-47.7464652997852));
#10909=CARTESIAN_POINT('Ctrl Pts',(24.3531646875,46.7708333401613,-42.1809185638422));
#10910=CARTESIAN_POINT('Ctrl Pts',(35.6555077526845,46.562500006828,-35.6555077526845));
#10911=CARTESIAN_POINT('Ctrl Pts',(42.1809185638422,46.3541666734946,-24.3531646875));
#10912=CARTESIAN_POINT('Ctrl Pts',(47.5573898704235,46.1825149229327,-15.0408432190651));
#10913=CARTESIAN_POINT('Ctrl Pts',(48.5134353784344,46.0074536451604,-4.33048599679671));
#10914=CARTESIAN_POINT('',(48.5134353784344,46.0074536451604,-4.33048599679671));
#10915=CARTESIAN_POINT('',(3.61292728433799,45.8792520480092,-48.5721450795008));
#10916=CARTESIAN_POINT('Origin',(-7.99360577730113E-14,57.8125000068276,
4.34631818602828E-14));
#10917=CARTESIAN_POINT('',(48.5725845633798,45.8793483229262,3.60701400320328));
#10918=CARTESIAN_POINT('',(48.5725845633798,44.6293483229262,3.60701400320328));
#10919=CARTESIAN_POINT('',(3.61292728433797,44.7457479656467,48.5721450795008));
#10920=CARTESIAN_POINT('Ctrl Pts',(48.5725845633798,45.8793483229262,3.60701400320328));
#10921=CARTESIAN_POINT('Ctrl Pts',(47.7480251419552,45.6985714020251,14.7106532430575));
#10922=CARTESIAN_POINT('Ctrl Pts',(42.1809185638422,45.5208333401613,24.3531646875));
#10923=CARTESIAN_POINT('Ctrl Pts',(35.6555077526845,45.312500006828,35.6555077526845));
#10924=CARTESIAN_POINT('Ctrl Pts',(24.3531646875,45.1041666734946,42.1809185638422));
#10925=CARTESIAN_POINT('Ctrl Pts',(14.7133549689477,44.9264784118853,47.7464652997852));
#10926=CARTESIAN_POINT('Ctrl Pts',(3.61292728433797,44.7457479656467,48.5721450795008));
#10927=CARTESIAN_POINT('',(3.61292728433797,44.7457479656467,48.5721450795008));
#10928=CARTESIAN_POINT('Origin',(-7.99360577730113E-14,57.8125000068276,
4.34631818602828E-14));
#10929=CARTESIAN_POINT('',(3.61292728433798,42.1292520480093,-48.5721450795008));
#10930=CARTESIAN_POINT('',(48.5134353784344,41.0074536451604,-4.33048599679679));
#10931=CARTESIAN_POINT('Ctrl Pts',(3.61292728433798,42.1292520480093,-48.5721450795008));
#10932=CARTESIAN_POINT('Ctrl Pts',(14.7133549689477,41.9485216017706,-47.7464652997852));
#10933=CARTESIAN_POINT('Ctrl Pts',(24.3531646875,41.7708333401613,-42.1809185638422));
#10934=CARTESIAN_POINT('Ctrl Pts',(35.6555077526845,41.562500006828,-35.6555077526845));
#10935=CARTESIAN_POINT('Ctrl Pts',(42.1809185638422,41.3541666734946,-24.3531646875));
#10936=CARTESIAN_POINT('Ctrl Pts',(47.5573898704235,41.1825149229327,-15.0408432190651));
#10937=CARTESIAN_POINT('Ctrl Pts',(48.5134353784344,41.0074536451604,-4.33048599679679));
#10938=CARTESIAN_POINT('',(48.5134353784344,41.0074536451604,-4.33048599679679));
#10939=CARTESIAN_POINT('',(3.61292728433798,40.8792520480093,-48.5721450795008));
#10940=CARTESIAN_POINT('Origin',(-7.99360577730113E-14,57.8125000068276,
4.34631818602828E-14));
#10941=CARTESIAN_POINT('',(48.5725845633798,40.8793483229262,3.60701400320329));
#10942=CARTESIAN_POINT('',(48.5725845633798,39.6293483229262,3.60701400320329));
#10943=CARTESIAN_POINT('',(3.61292728433799,39.7457479656467,48.5721450795008));
#10944=CARTESIAN_POINT('Ctrl Pts',(48.5725845633798,40.8793483229262,3.60701400320329));
#10945=CARTESIAN_POINT('Ctrl Pts',(47.7480251419552,40.6985714020251,14.7106532430575));
#10946=CARTESIAN_POINT('Ctrl Pts',(42.1809185638422,40.5208333401613,24.3531646875));
#10947=CARTESIAN_POINT('Ctrl Pts',(35.6555077526845,40.312500006828,35.6555077526845));
#10948=CARTESIAN_POINT('Ctrl Pts',(24.3531646875,40.1041666734946,42.1809185638422));
#10949=CARTESIAN_POINT('Ctrl Pts',(14.7133549689477,39.9264784118853,47.7464652997852));
#10950=CARTESIAN_POINT('Ctrl Pts',(3.61292728433799,39.7457479656467,48.5721450795008));
#10951=CARTESIAN_POINT('',(3.61292728433799,39.7457479656467,48.5721450795008));
#10952=CARTESIAN_POINT('Origin',(-7.99360577730113E-14,57.8125000068276,
4.34631818602828E-14));
#10953=CARTESIAN_POINT('',(-48.5134353784345,58.3675463684955,-4.33048599679673));
#10954=CARTESIAN_POINT('',(-48.5134353784345,57.1175463684955,-4.33048599679673));
#10955=CARTESIAN_POINT('',(-4.32456003949879,57.2573567866782,-48.5139639861634));
#10956=CARTESIAN_POINT('Ctrl Pts',(-48.5134353784344,58.3675463684955,-4.33048599679673));
#10957=CARTESIAN_POINT('Ctrl Pts',(-47.5573898704235,58.1924850907233,-15.0408432190651));
#10958=CARTESIAN_POINT('Ctrl Pts',(-42.1809185638422,58.0208333401613,-24.3531646875));
#10959=CARTESIAN_POINT('Ctrl Pts',(-35.6555077526845,57.812500006828,-35.6555077526845));
#10960=CARTESIAN_POINT('Ctrl Pts',(-24.3531646875,57.6041666734946,-42.1809185638422));
#10961=CARTESIAN_POINT('Ctrl Pts',(-15.038141415499,57.4324651212465,-47.5589497574396));
#10962=CARTESIAN_POINT('Ctrl Pts',(-4.32456003949879,57.2573567866782,-48.5139639861634));
#10963=CARTESIAN_POINT('',(-4.32456003949879,57.2573567866783,-48.5139639861634));
#10964=CARTESIAN_POINT('Origin',(-7.99360577730113E-14,57.8125000068276,
4.34631818602828E-14));
#10965=CARTESIAN_POINT('',(-48.5134353784344,53.3675463684955,-4.33048599679673));
#10966=CARTESIAN_POINT('',(-48.5134353784345,52.1175463684955,-4.33048599679673));
#10967=CARTESIAN_POINT('',(-4.32456003949876,52.2573567866782,-48.5139639861634));
#10968=CARTESIAN_POINT('Ctrl Pts',(-48.5134353784344,53.3675463684955,-4.33048599679673));
#10969=CARTESIAN_POINT('Ctrl Pts',(-47.5573898704235,53.1924850907232,-15.0408432190651));
#10970=CARTESIAN_POINT('Ctrl Pts',(-42.1809185638422,53.0208333401613,-24.3531646875));
#10971=CARTESIAN_POINT('Ctrl Pts',(-35.6555077526845,52.812500006828,-35.6555077526845));
#10972=CARTESIAN_POINT('Ctrl Pts',(-24.3531646875,52.6041666734946,-42.1809185638422));
#10973=CARTESIAN_POINT('Ctrl Pts',(-15.038141415499,52.4324651212465,-47.5589497574396));
#10974=CARTESIAN_POINT('Ctrl Pts',(-4.32456003949876,52.2573567866783,-48.5139639861634));
#10975=CARTESIAN_POINT('',(-4.32456003949876,52.2573567866782,-48.5139639861634));
#10976=CARTESIAN_POINT('Origin',(-7.99360577730113E-14,57.8125000068276,
4.34631818602828E-14));
#10977=CARTESIAN_POINT('',(-4.32456003949878,54.6176432269777,48.5139639861634));
#10978=CARTESIAN_POINT('',(-48.5725845633798,53.4956516907298,3.60701400320327));
#10979=CARTESIAN_POINT('Ctrl Pts',(-4.32456003949878,54.6176432269777,48.5139639861634));
#10980=CARTESIAN_POINT('Ctrl Pts',(-15.038141415499,54.4425348924095,47.5589497574396));
#10981=CARTESIAN_POINT('Ctrl Pts',(-24.3531646875,54.2708333401613,42.1809185638423));
#10982=CARTESIAN_POINT('Ctrl Pts',(-35.6555077526845,54.062500006828,35.6555077526845));
#10983=CARTESIAN_POINT('Ctrl Pts',(-42.1809185638422,53.8541666734946,24.3531646875));
#10984=CARTESIAN_POINT('Ctrl Pts',(-47.7480251419551,53.6764286116308,14.7106532430575));
#10985=CARTESIAN_POINT('Ctrl Pts',(-48.5725845633798,53.4956516907298,3.60701400320327));
#10986=CARTESIAN_POINT('',(-48.5725845633798,53.4956516907298,3.60701400320327));
#10987=CARTESIAN_POINT('',(-4.32456003949878,53.3676432269777,48.5139639861634));
#10988=CARTESIAN_POINT('Origin',(-7.99360577730113E-14,57.8125000068276,
4.34631818602828E-14));
#10989=CARTESIAN_POINT('',(-48.5134353784344,48.3675463684955,-4.33048599679673));
#10990=CARTESIAN_POINT('',(-48.5134353784345,47.1175463684955,-4.33048599679673));
#10991=CARTESIAN_POINT('',(-4.32456003949881,47.2573567866782,-48.5139639861634));
#10992=CARTESIAN_POINT('Ctrl Pts',(-48.5134353784344,48.3675463684955,-4.33048599679673));
#10993=CARTESIAN_POINT('Ctrl Pts',(-47.5573898704235,48.1924850907233,-15.0408432190651));
#10994=CARTESIAN_POINT('Ctrl Pts',(-42.1809185638422,48.0208333401613,-24.3531646875));
#10995=CARTESIAN_POINT('Ctrl Pts',(-35.6555077526845,47.812500006828,-35.6555077526845));
#10996=CARTESIAN_POINT('Ctrl Pts',(-24.3531646875,47.6041666734946,-42.1809185638422));
#10997=CARTESIAN_POINT('Ctrl Pts',(-15.0381414154991,47.4324651212465,-47.5589497574396));
#10998=CARTESIAN_POINT('Ctrl Pts',(-4.32456003949881,47.2573567866782,-48.5139639861634));
#10999=CARTESIAN_POINT('',(-4.32456003949881,47.2573567866783,-48.5139639861634));
#11000=CARTESIAN_POINT('Origin',(-7.99360577730113E-14,57.8125000068276,
4.34631818602828E-14));
#11001=CARTESIAN_POINT('',(-4.32456003949883,49.6176432269777,48.5139639861634));
#11002=CARTESIAN_POINT('',(-48.5725845633798,48.4956516907297,3.60701400320326));
#11003=CARTESIAN_POINT('Ctrl Pts',(-4.32456003949883,49.6176432269777,48.5139639861634));
#11004=CARTESIAN_POINT('Ctrl Pts',(-15.0381414154991,49.4425348924095,47.5589497574396));
#11005=CARTESIAN_POINT('Ctrl Pts',(-24.3531646875,49.2708333401613,42.1809185638423));
#11006=CARTESIAN_POINT('Ctrl Pts',(-35.6555077526845,49.062500006828,35.6555077526845));
#11007=CARTESIAN_POINT('Ctrl Pts',(-42.1809185638422,48.8541666734946,24.3531646875));
#11008=CARTESIAN_POINT('Ctrl Pts',(-47.7480251419552,48.6764286116309,14.7106532430575));
#11009=CARTESIAN_POINT('Ctrl Pts',(-48.5725845633798,48.4956516907297,3.60701400320326));
#11010=CARTESIAN_POINT('',(-48.5725845633798,48.4956516907297,3.60701400320326));
#11011=CARTESIAN_POINT('',(-4.32456003949883,48.3676432269777,48.5139639861634));
#11012=CARTESIAN_POINT('Origin',(-7.99360577730113E-14,57.8125000068276,
4.34631818602828E-14));
#11013=CARTESIAN_POINT('',(-48.5134353784345,43.3675463684955,-4.33048599679665));
#11014=CARTESIAN_POINT('',(-48.5134353784345,42.1175463684956,-4.33048599679665));
#11015=CARTESIAN_POINT('',(-4.32456003949873,42.2573567866782,-48.5139639861634));
#11016=CARTESIAN_POINT('Ctrl Pts',(-48.5134353784345,43.3675463684955,-4.33048599679665));
#11017=CARTESIAN_POINT('Ctrl Pts',(-47.5573898704235,43.1924850907233,-15.040843219065));
#11018=CARTESIAN_POINT('Ctrl Pts',(-42.1809185638422,43.0208333401613,-24.3531646875));
#11019=CARTESIAN_POINT('Ctrl Pts',(-35.6555077526845,42.812500006828,-35.6555077526845));
#11020=CARTESIAN_POINT('Ctrl Pts',(-24.3531646875,42.6041666734946,-42.1809185638422));
#11021=CARTESIAN_POINT('Ctrl Pts',(-15.038141415499,42.4324651212465,-47.5589497574396));
#11022=CARTESIAN_POINT('Ctrl Pts',(-4.32456003949873,42.2573567866782,-48.5139639861634));
#11023=CARTESIAN_POINT('',(-4.32456003949873,42.2573567866783,-48.5139639861634));
#11024=CARTESIAN_POINT('Origin',(-7.99360577730113E-14,57.8125000068276,
4.34631818602828E-14));
#11025=CARTESIAN_POINT('',(-4.32456003949883,44.6176432269777,48.5139639861634));
#11026=CARTESIAN_POINT('',(-48.5725845633798,43.4956516907297,3.60701400320326));
#11027=CARTESIAN_POINT('Ctrl Pts',(-4.32456003949883,44.6176432269777,48.5139639861634));
#11028=CARTESIAN_POINT('Ctrl Pts',(-15.0381414154991,44.4425348924095,47.5589497574396));
#11029=CARTESIAN_POINT('Ctrl Pts',(-24.3531646875,44.2708333401613,42.1809185638423));
#11030=CARTESIAN_POINT('Ctrl Pts',(-35.6555077526845,44.062500006828,35.6555077526845));
#11031=CARTESIAN_POINT('Ctrl Pts',(-42.1809185638422,43.8541666734946,24.3531646875));
#11032=CARTESIAN_POINT('Ctrl Pts',(-47.7480251419552,43.6764286116309,14.7106532430575));
#11033=CARTESIAN_POINT('Ctrl Pts',(-48.5725845633798,43.4956516907297,3.60701400320326));
#11034=CARTESIAN_POINT('',(-48.5725845633798,43.4956516907297,3.60701400320326));
#11035=CARTESIAN_POINT('',(-4.32456003949883,43.3676432269777,48.5139639861634));
#11036=CARTESIAN_POINT('Origin',(-7.99360577730113E-14,57.8125000068276,
4.34631818602828E-14));
#11037=CARTESIAN_POINT('',(-48.5134353784344,38.3675463684955,-4.33048599679682));
#11038=CARTESIAN_POINT('',(-48.5134353784344,37.1175463684955,-4.33048599679682));
#11039=CARTESIAN_POINT('',(-4.32456003949869,37.2573567866782,-48.5139639861634));
#11040=CARTESIAN_POINT('Ctrl Pts',(-48.5134353784344,38.3675463684955,-4.33048599679682));
#11041=CARTESIAN_POINT('Ctrl Pts',(-47.5573898704235,38.1924850907232,-15.0408432190651));
#11042=CARTESIAN_POINT('Ctrl Pts',(-42.1809185638422,38.0208333401613,-24.3531646875));
#11043=CARTESIAN_POINT('Ctrl Pts',(-35.6555077526845,37.812500006828,-35.6555077526845));
#11044=CARTESIAN_POINT('Ctrl Pts',(-24.3531646875,37.6041666734946,-42.1809185638422));
#11045=CARTESIAN_POINT('Ctrl Pts',(-15.038141415499,37.4324651212465,-47.5589497574396));
#11046=CARTESIAN_POINT('Ctrl Pts',(-4.32456003949869,37.2573567866782,-48.5139639861634));
#11047=CARTESIAN_POINT('',(-4.32456320853981,36.9438035983105,-48.513963421183));
#11048=CARTESIAN_POINT('',(-4.32456003949878,37.2573567866782,-48.5139639861634));
#11049=CARTESIAN_POINT('Ctrl Pts',(-4.32456637758084,36.9438035983105,-48.5139634211829));
#11050=CARTESIAN_POINT('Ctrl Pts',(-4.32456637758084,36.6377267119794,-48.5139634211829));
#11051=CARTESIAN_POINT('Ctrl Pts',(-4.2883015397967,36.3188714657862,-48.5172427906022));
#11052=CARTESIAN_POINT('Ctrl Pts',(-4.21205777787802,36.0055185535965,-48.5238610423963));
#11053=CARTESIAN_POINT('Origin',(-7.99360577730113E-14,57.8125000068276,
4.34631818602828E-14));
#11054=CARTESIAN_POINT('',(-4.32456003949875,39.6176432269777,48.5139639861634));
#11055=CARTESIAN_POINT('',(-48.5725845633798,38.4956516907297,3.60701400320327));
#11056=CARTESIAN_POINT('Ctrl Pts',(-4.32456003949875,39.6176432269777,48.5139639861634));
#11057=CARTESIAN_POINT('Ctrl Pts',(-15.038141415499,39.4425348924095,47.5589497574396));
#11058=CARTESIAN_POINT('Ctrl Pts',(-24.3531646875,39.2708333401613,42.1809185638423));
#11059=CARTESIAN_POINT('Ctrl Pts',(-35.6555077526845,39.062500006828,35.6555077526845));
#11060=CARTESIAN_POINT('Ctrl Pts',(-42.1809185638422,38.8541666734946,24.3531646875));
#11061=CARTESIAN_POINT('Ctrl Pts',(-47.7480251419552,38.6764286116308,14.7106532430575));
#11062=CARTESIAN_POINT('Ctrl Pts',(-48.5725845633798,38.4956516907297,3.60701400320327));
#11063=CARTESIAN_POINT('',(-48.5725845633798,38.4956516907298,3.60701400320327));
#11064=CARTESIAN_POINT('',(-4.32456003949875,38.3676432269777,48.5139639861634));
#11065=CARTESIAN_POINT('Origin',(-7.99360577730113E-14,57.8125000068276,
4.34631818602828E-14));
#11066=CARTESIAN_POINT('',(3.61292728433801,37.1292520480092,-48.5721450795008));
#11067=CARTESIAN_POINT('',(48.5134353784344,36.0074536451604,-4.33048599679682));
#11068=CARTESIAN_POINT('Ctrl Pts',(3.61292728433801,37.1292520480092,-48.5721450795008));
#11069=CARTESIAN_POINT('Ctrl Pts',(14.7133549689477,36.9485216017706,-47.7464652997852));
#11070=CARTESIAN_POINT('Ctrl Pts',(24.3531646875,36.7708333401613,-42.1809185638422));
#11071=CARTESIAN_POINT('Ctrl Pts',(35.6555077526845,36.562500006828,-35.6555077526845));
#11072=CARTESIAN_POINT('Ctrl Pts',(42.1809185638422,36.3541666734946,-24.3531646875));
#11073=CARTESIAN_POINT('Ctrl Pts',(47.5573898704234,36.1825149229327,-15.0408432190651));
#11074=CARTESIAN_POINT('Ctrl Pts',(48.5134353784344,36.0074536451604,-4.33048599679682));
#11075=CARTESIAN_POINT('',(48.5134353784344,34.7574536451604,-4.33048599679682));
#11076=CARTESIAN_POINT('',(48.5134353784344,36.0074536451604,-4.33048599679682));
#11077=CARTESIAN_POINT('',(3.46814984980029,35.8816082987783,-48.5826971030358));
#11078=CARTESIAN_POINT('Ctrl Pts',(3.46814984980029,35.8816082987783,-48.5826971030357));
#11079=CARTESIAN_POINT('Ctrl Pts',(14.6471927118254,35.6997411545207,-47.7846640967449));
#11080=CARTESIAN_POINT('Ctrl Pts',(24.3531646875,35.5208333401613,-42.1809185638422));
#11081=CARTESIAN_POINT('Ctrl Pts',(35.6555077526845,35.312500006828,-35.6555077526845));
#11082=CARTESIAN_POINT('Ctrl Pts',(42.1809185638422,35.1041666734946,-24.3531646875));
#11083=CARTESIAN_POINT('Ctrl Pts',(47.5573898704235,34.9325149229327,-15.0408432190651));
#11084=CARTESIAN_POINT('Ctrl Pts',(48.5134353784344,34.7574536451604,-4.33048599679682));
#11085=CARTESIAN_POINT('',(3.61293045337858,36.9438035983107,-48.5721446080567));
#11086=CARTESIAN_POINT('Ctrl Pts',(3.46814984980031,35.8816082987783,-48.5826971030356));
#11087=CARTESIAN_POINT('Ctrl Pts',(3.56615768657923,36.2344423378917,-48.5757006642894));
#11088=CARTESIAN_POINT('Ctrl Pts',(3.61293362241916,36.5973099952525,-48.5721446080566));
#11089=CARTESIAN_POINT('Ctrl Pts',(3.61293362241916,36.9438035983105,-48.5721446080566));
#11090=CARTESIAN_POINT('',(3.61292728433799,36.9438035983105,-48.5721446080568));
#11091=CARTESIAN_POINT('Origin',(-7.99360577730113E-14,57.8125000068276,
4.34631818602828E-14));
#11092=CARTESIAN_POINT('',(48.5725845633798,34.6293483229262,3.60701400320329));
#11093=CARTESIAN_POINT('',(1.54954344745643,33.4623411901214,48.6816745427931));
#11094=CARTESIAN_POINT('Ctrl Pts',(48.5725845633798,34.6293483229262,3.60701400320329));
#11095=CARTESIAN_POINT('Ctrl Pts',(47.7480251419552,34.4485714020251,14.7106532430575));
#11096=CARTESIAN_POINT('Ctrl Pts',(42.1809185638422,34.2708333401613,24.3531646875));
#11097=CARTESIAN_POINT('Ctrl Pts',(35.6555077526845,34.062500006828,35.6555077526845));
#11098=CARTESIAN_POINT('Ctrl Pts',(24.3531646875,33.8541666734946,42.1809185638422));
#11099=CARTESIAN_POINT('Ctrl Pts',(13.7670955736885,33.6590362432238,48.2927884163613));
#11100=CARTESIAN_POINT('Ctrl Pts',(1.54954344745643,33.4623411901214,48.6816745427932));
#11101=CARTESIAN_POINT('',(48.5725845633798,35.8793483229262,3.60701400320329));
#11102=CARTESIAN_POINT('',(48.5725845633798,34.6293483229262,3.60701400320329));
#11103=CARTESIAN_POINT('',(2.94136876951422,34.7348340040708,48.6174338169726));
#11104=CARTESIAN_POINT('Ctrl Pts',(48.5725845633798,35.8793483229262,3.60701400320329));
#11105=CARTESIAN_POINT('Ctrl Pts',(47.7480251419552,35.6985714020251,14.7106532430575));
#11106=CARTESIAN_POINT('Ctrl Pts',(42.1809185638422,35.5208333401613,24.3531646875));
#11107=CARTESIAN_POINT('Ctrl Pts',(35.6555077526845,35.312500006828,35.6555077526845));
#11108=CARTESIAN_POINT('Ctrl Pts',(24.3531646875,35.1041666734946,42.1809185638422));
#11109=CARTESIAN_POINT('Ctrl Pts',(14.4061866175215,34.9208164525749,47.9238090301676));
#11110=CARTESIAN_POINT('Ctrl Pts',(2.94136876951422,34.7348340040708,48.6174338169726));
#11111=CARTESIAN_POINT('Ctrl Pts',(2.94136876951423,34.7348340040708,48.6174338169726));
#11112=CARTESIAN_POINT('Ctrl Pts',(2.79472533668362,34.5159488958697,48.6263057869578));
#11113=CARTESIAN_POINT('Ctrl Pts',(2.62805668979196,34.3149976738954,48.6357018449976));
#11114=CARTESIAN_POINT('Ctrl Pts',(2.19334294752016,33.880330228219,48.6575995652533));
#11115=CARTESIAN_POINT('Ctrl Pts',(1.88701847015379,33.6470369515028,48.6709326729825));
#11116=CARTESIAN_POINT('Ctrl Pts',(1.54954344745642,33.4623411901214,48.6816745427931));
#11117=CARTESIAN_POINT('Ctrl Pts',(-48.706329375,58.437500006828,-1.8898197019151E-14));
#11118=CARTESIAN_POINT('Ctrl Pts',(-48.706329375,58.2291666734946,-13.0508216223155));
#11119=CARTESIAN_POINT('Ctrl Pts',(-42.1809185638422,58.0208333401613,-24.3531646875));
#11120=CARTESIAN_POINT('Ctrl Pts',(-35.6555077526845,57.812500006828,-35.6555077526845));
#11121=CARTESIAN_POINT('Ctrl Pts',(-24.3531646875,57.6041666734946,-42.1809185638422));
#11122=CARTESIAN_POINT('Ctrl Pts',(-13.0508216223155,57.3958333401613,-48.706329375));
#11123=CARTESIAN_POINT('Ctrl Pts',(1.59157945007855E-14,57.187500006828,
-48.706329375));
#11124=CARTESIAN_POINT('Ctrl Pts',(13.0508216223155,56.9791666734946,-48.706329375));
#11125=CARTESIAN_POINT('Ctrl Pts',(24.3531646875,56.7708333401613,-42.1809185638422));
#11126=CARTESIAN_POINT('Ctrl Pts',(35.6555077526845,56.562500006828,-35.6555077526845));
#11127=CARTESIAN_POINT('Ctrl Pts',(42.1809185638422,56.3541666734946,-24.3531646875));
#11128=CARTESIAN_POINT('Ctrl Pts',(48.706329375,56.1458333401613,-13.0508216223155));
#11129=CARTESIAN_POINT('Ctrl Pts',(48.706329375,55.937500006828,1.293339198242E-14));
#11130=CARTESIAN_POINT('Ctrl Pts',(48.706329375,55.7291666734946,13.0508216223155));
#11131=CARTESIAN_POINT('Ctrl Pts',(42.1809185638422,55.5208333401613,24.3531646875));
#11132=CARTESIAN_POINT('Ctrl Pts',(35.6555077526845,55.312500006828,35.6555077526845));
#11133=CARTESIAN_POINT('Ctrl Pts',(24.3531646875,55.1041666734946,42.1809185638422));
#11134=CARTESIAN_POINT('Ctrl Pts',(13.0508216223155,54.8958333401613,48.706329375));
#11135=CARTESIAN_POINT('Ctrl Pts',(-9.95098946405443E-15,54.687500006828,
48.706329375));
#11136=CARTESIAN_POINT('Ctrl Pts',(-13.0508216223155,54.4791666734946,48.706329375));
#11137=CARTESIAN_POINT('Ctrl Pts',(-24.3531646875,54.2708333401613,42.1809185638423));
#11138=CARTESIAN_POINT('Ctrl Pts',(-35.6555077526845,54.062500006828,35.6555077526845));
#11139=CARTESIAN_POINT('Ctrl Pts',(-42.1809185638422,53.8541666734946,24.3531646875));
#11140=CARTESIAN_POINT('Ctrl Pts',(-48.706329375,53.6458333401613,13.0508216223155));
#11141=CARTESIAN_POINT('Ctrl Pts',(-48.706329375,53.437500006828,-1.8898197019151E-14));
#11142=CARTESIAN_POINT('Ctrl Pts',(-48.706329375,53.2291666734946,-13.0508216223155));
#11143=CARTESIAN_POINT('Ctrl Pts',(-42.1809185638422,53.0208333401613,-24.3531646875));
#11144=CARTESIAN_POINT('Ctrl Pts',(-35.6555077526845,52.812500006828,-35.6555077526845));
#11145=CARTESIAN_POINT('Ctrl Pts',(-24.3531646875,52.6041666734946,-42.1809185638422));
#11146=CARTESIAN_POINT('Ctrl Pts',(-13.0508216223155,52.3958333401613,-48.706329375));
#11147=CARTESIAN_POINT('Ctrl Pts',(1.59157945007855E-14,52.187500006828,
-48.706329375));
#11148=CARTESIAN_POINT('Ctrl Pts',(13.0508216223155,51.9791666734946,-48.706329375));
#11149=CARTESIAN_POINT('Ctrl Pts',(24.3531646875,51.7708333401613,-42.1809185638422));
#11150=CARTESIAN_POINT('Ctrl Pts',(35.6555077526845,51.562500006828,-35.6555077526845));
#11151=CARTESIAN_POINT('Ctrl Pts',(42.1809185638422,51.3541666734946,-24.3531646875));
#11152=CARTESIAN_POINT('Ctrl Pts',(48.706329375,51.1458333401613,-13.0508216223155));
#11153=CARTESIAN_POINT('Ctrl Pts',(48.706329375,50.937500006828,1.293339198242E-14));
#11154=CARTESIAN_POINT('Ctrl Pts',(48.706329375,50.7291666734946,13.0508216223155));
#11155=CARTESIAN_POINT('Ctrl Pts',(42.1809185638422,50.5208333401613,24.3531646875));
#11156=CARTESIAN_POINT('Ctrl Pts',(35.6555077526845,50.312500006828,35.6555077526845));
#11157=CARTESIAN_POINT('Ctrl Pts',(24.3531646875,50.1041666734946,42.1809185638422));
#11158=CARTESIAN_POINT('Ctrl Pts',(13.0508216223155,49.8958333401613,48.706329375));
#11159=CARTESIAN_POINT('Ctrl Pts',(-9.95098946405443E-15,49.687500006828,
48.706329375));
#11160=CARTESIAN_POINT('Ctrl Pts',(-13.0508216223155,49.4791666734946,48.706329375));
#11161=CARTESIAN_POINT('Ctrl Pts',(-24.3531646875,49.2708333401613,42.1809185638423));
#11162=CARTESIAN_POINT('Ctrl Pts',(-35.6555077526845,49.062500006828,35.6555077526845));
#11163=CARTESIAN_POINT('Ctrl Pts',(-42.1809185638422,48.8541666734946,24.3531646875));
#11164=CARTESIAN_POINT('Ctrl Pts',(-48.706329375,48.6458333401613,13.0508216223155));
#11165=CARTESIAN_POINT('Ctrl Pts',(-48.706329375,48.437500006828,-1.8898197019151E-14));
#11166=CARTESIAN_POINT('Ctrl Pts',(-48.706329375,48.2291666734946,-13.0508216223155));
#11167=CARTESIAN_POINT('Ctrl Pts',(-42.1809185638422,48.0208333401613,-24.3531646875));
#11168=CARTESIAN_POINT('Ctrl Pts',(-35.6555077526845,47.812500006828,-35.6555077526845));
#11169=CARTESIAN_POINT('Ctrl Pts',(-24.3531646875,47.6041666734946,-42.1809185638422));
#11170=CARTESIAN_POINT('Ctrl Pts',(-13.0508216223155,47.3958333401613,-48.706329375));
#11171=CARTESIAN_POINT('Ctrl Pts',(1.59157945007855E-14,47.187500006828,
-48.706329375));
#11172=CARTESIAN_POINT('Ctrl Pts',(13.0508216223155,46.9791666734946,-48.706329375));
#11173=CARTESIAN_POINT('Ctrl Pts',(24.3531646875,46.7708333401613,-42.1809185638422));
#11174=CARTESIAN_POINT('Ctrl Pts',(35.6555077526845,46.562500006828,-35.6555077526845));
#11175=CARTESIAN_POINT('Ctrl Pts',(42.1809185638422,46.3541666734946,-24.3531646875));
#11176=CARTESIAN_POINT('Ctrl Pts',(48.706329375,46.1458333401613,-13.0508216223155));
#11177=CARTESIAN_POINT('Ctrl Pts',(48.706329375,45.937500006828,1.293339198242E-14));
#11178=CARTESIAN_POINT('Ctrl Pts',(48.706329375,45.7291666734946,13.0508216223155));
#11179=CARTESIAN_POINT('Ctrl Pts',(42.1809185638422,45.5208333401613,24.3531646875));
#11180=CARTESIAN_POINT('Ctrl Pts',(35.6555077526845,45.312500006828,35.6555077526845));
#11181=CARTESIAN_POINT('Ctrl Pts',(24.3531646875,45.1041666734946,42.1809185638422));
#11182=CARTESIAN_POINT('Ctrl Pts',(13.0508216223155,44.8958333401613,48.706329375));
#11183=CARTESIAN_POINT('Ctrl Pts',(-9.95098946405443E-15,44.687500006828,
48.706329375));
#11184=CARTESIAN_POINT('Ctrl Pts',(-13.0508216223155,44.4791666734946,48.706329375));
#11185=CARTESIAN_POINT('Ctrl Pts',(-24.3531646875,44.2708333401613,42.1809185638423));
#11186=CARTESIAN_POINT('Ctrl Pts',(-35.6555077526845,44.062500006828,35.6555077526845));
#11187=CARTESIAN_POINT('Ctrl Pts',(-42.1809185638422,43.8541666734946,24.3531646875));
#11188=CARTESIAN_POINT('Ctrl Pts',(-48.706329375,43.6458333401613,13.0508216223155));
#11189=CARTESIAN_POINT('Ctrl Pts',(-48.706329375,43.437500006828,-1.8898197019151E-14));
#11190=CARTESIAN_POINT('Ctrl Pts',(-48.706329375,43.2291666734946,-13.0508216223155));
#11191=CARTESIAN_POINT('Ctrl Pts',(-42.1809185638422,43.0208333401613,-24.3531646875));
#11192=CARTESIAN_POINT('Ctrl Pts',(-35.6555077526845,42.812500006828,-35.6555077526845));
#11193=CARTESIAN_POINT('Ctrl Pts',(-24.3531646875,42.6041666734946,-42.1809185638422));
#11194=CARTESIAN_POINT('Ctrl Pts',(-13.0508216223155,42.3958333401613,-48.706329375));
#11195=CARTESIAN_POINT('Ctrl Pts',(1.59157945007855E-14,42.187500006828,
-48.706329375));
#11196=CARTESIAN_POINT('Ctrl Pts',(13.0508216223155,41.9791666734946,-48.706329375));
#11197=CARTESIAN_POINT('Ctrl Pts',(24.3531646875,41.7708333401613,-42.1809185638422));
#11198=CARTESIAN_POINT('Ctrl Pts',(35.6555077526845,41.562500006828,-35.6555077526845));
#11199=CARTESIAN_POINT('Ctrl Pts',(42.1809185638422,41.3541666734946,-24.3531646875));
#11200=CARTESIAN_POINT('Ctrl Pts',(48.706329375,41.1458333401613,-13.0508216223155));
#11201=CARTESIAN_POINT('Ctrl Pts',(48.706329375,40.937500006828,1.293339198242E-14));
#11202=CARTESIAN_POINT('Ctrl Pts',(48.706329375,40.7291666734946,13.0508216223155));
#11203=CARTESIAN_POINT('Ctrl Pts',(42.1809185638422,40.5208333401613,24.3531646875));
#11204=CARTESIAN_POINT('Ctrl Pts',(35.6555077526845,40.312500006828,35.6555077526845));
#11205=CARTESIAN_POINT('Ctrl Pts',(24.3531646875,40.1041666734946,42.1809185638422));
#11206=CARTESIAN_POINT('Ctrl Pts',(13.0508216223155,39.8958333401613,48.706329375));
#11207=CARTESIAN_POINT('Ctrl Pts',(-9.95098946405443E-15,39.687500006828,
48.706329375));
#11208=CARTESIAN_POINT('Ctrl Pts',(-13.0508216223155,39.4791666734946,48.706329375));
#11209=CARTESIAN_POINT('Ctrl Pts',(-24.3531646875,39.2708333401613,42.1809185638423));
#11210=CARTESIAN_POINT('Ctrl Pts',(-35.6555077526845,39.062500006828,35.6555077526845));
#11211=CARTESIAN_POINT('Ctrl Pts',(-42.1809185638422,38.8541666734946,24.3531646875));
#11212=CARTESIAN_POINT('Ctrl Pts',(-48.706329375,38.6458333401613,13.0508216223155));
#11213=CARTESIAN_POINT('Ctrl Pts',(-48.706329375,38.437500006828,-1.8898197019151E-14));
#11214=CARTESIAN_POINT('Ctrl Pts',(-48.706329375,38.2291666734946,-13.0508216223155));
#11215=CARTESIAN_POINT('Ctrl Pts',(-42.1809185638422,38.0208333401613,-24.3531646875));
#11216=CARTESIAN_POINT('Ctrl Pts',(-35.6555077526845,37.812500006828,-35.6555077526845));
#11217=CARTESIAN_POINT('Ctrl Pts',(-24.3531646875,37.6041666734946,-42.1809185638422));
#11218=CARTESIAN_POINT('Ctrl Pts',(-13.0508216223155,37.3958333401613,-48.706329375));
#11219=CARTESIAN_POINT('Ctrl Pts',(1.59157945007855E-14,37.187500006828,
-48.706329375));
#11220=CARTESIAN_POINT('Ctrl Pts',(13.0508216223155,36.9791666734946,-48.706329375));
#11221=CARTESIAN_POINT('Ctrl Pts',(24.3531646875,36.7708333401613,-42.1809185638422));
#11222=CARTESIAN_POINT('Ctrl Pts',(35.6555077526845,36.562500006828,-35.6555077526845));
#11223=CARTESIAN_POINT('Ctrl Pts',(42.1809185638422,36.3541666734946,-24.3531646875));
#11224=CARTESIAN_POINT('Ctrl Pts',(48.706329375,36.1458333401613,-13.0508216223155));
#11225=CARTESIAN_POINT('Ctrl Pts',(48.706329375,35.937500006828,1.293339198242E-14));
#11226=CARTESIAN_POINT('Ctrl Pts',(48.706329375,35.7291666734946,13.0508216223155));
#11227=CARTESIAN_POINT('Ctrl Pts',(42.1809185638422,35.5208333401613,24.3531646875));
#11228=CARTESIAN_POINT('Ctrl Pts',(35.6555077526845,35.312500006828,35.6555077526845));
#11229=CARTESIAN_POINT('Ctrl Pts',(24.3531646875,35.1041666734946,42.1809185638422));
#11230=CARTESIAN_POINT('Ctrl Pts',(13.0508216223155,34.8958333401613,48.706329375));
#11231=CARTESIAN_POINT('Ctrl Pts',(-9.95098946405443E-15,34.687500006828,
48.706329375));
#11232=CARTESIAN_POINT('Ctrl Pts',(-13.0508216223155,34.4791666734946,48.706329375));
#11233=CARTESIAN_POINT('Ctrl Pts',(-24.3531646875,34.2708333401613,42.1809185638423));
#11234=CARTESIAN_POINT('Ctrl Pts',(-35.6555077526845,34.062500006828,35.6555077526845));
#11235=CARTESIAN_POINT('Ctrl Pts',(-42.1809185638422,33.8541666734946,24.3531646875));
#11236=CARTESIAN_POINT('Ctrl Pts',(-48.706329375,33.6458333401613,13.0508216223155));
#11237=CARTESIAN_POINT('Ctrl Pts',(-48.706329375,33.437500006828,-1.8898197019151E-14));
#11238=CARTESIAN_POINT('Ctrl Pts',(-48.706329375,33.2291666734946,-13.0508216223155));
#11239=CARTESIAN_POINT('Ctrl Pts',(-42.1809185638422,33.0208333401613,-24.3531646875));
#11240=CARTESIAN_POINT('Ctrl Pts',(-35.6555077526845,32.812500006828,-35.6555077526845));
#11241=CARTESIAN_POINT('Ctrl Pts',(-24.3531646875,32.6041666734946,-42.1809185638422));
#11242=CARTESIAN_POINT('Ctrl Pts',(-13.0508216223155,32.3958333401613,-48.706329375));
#11243=CARTESIAN_POINT('Ctrl Pts',(1.59157945007855E-14,32.187500006828,
-48.706329375));
#11244=CARTESIAN_POINT('Ctrl Pts',(13.0508216223155,31.9791666734946,-48.706329375));
#11245=CARTESIAN_POINT('Ctrl Pts',(24.3531646875,31.7708333401613,-42.1809185638422));
#11246=CARTESIAN_POINT('Ctrl Pts',(35.6555077526845,31.562500006828,-35.6555077526845));
#11247=CARTESIAN_POINT('Ctrl Pts',(42.1809185638422,31.3541666734946,-24.3531646875));
#11248=CARTESIAN_POINT('Ctrl Pts',(48.706329375,31.1458333401613,-13.0508216223155));
#11249=CARTESIAN_POINT('Ctrl Pts',(48.706329375,30.937500006828,1.293339198242E-14));
#11250=CARTESIAN_POINT('Ctrl Pts',(48.706329375,30.7291666734946,13.0508216223155));
#11251=CARTESIAN_POINT('Ctrl Pts',(42.1809185638422,30.5208333401613,24.3531646875));
#11252=CARTESIAN_POINT('Ctrl Pts',(35.6555077526845,30.312500006828,35.6555077526845));
#11253=CARTESIAN_POINT('Ctrl Pts',(24.3531646875,30.1041666734946,42.1809185638422));
#11254=CARTESIAN_POINT('Ctrl Pts',(13.0508216223155,29.8958333401613,48.706329375));
#11255=CARTESIAN_POINT('Ctrl Pts',(-9.95098946405443E-15,29.687500006828,
48.706329375));
#11256=CARTESIAN_POINT('Ctrl Pts',(-13.0508216223155,29.4791666734946,48.706329375));
#11257=CARTESIAN_POINT('Ctrl Pts',(-24.3531646875,29.2708333401613,42.1809185638423));
#11258=CARTESIAN_POINT('Ctrl Pts',(-35.6555077526845,29.062500006828,35.6555077526845));
#11259=CARTESIAN_POINT('Ctrl Pts',(-42.1809185638422,28.8541666734946,24.3531646875));
#11260=CARTESIAN_POINT('Ctrl Pts',(-48.706329375,28.6458333401613,13.0508216223155));
#11261=CARTESIAN_POINT('Ctrl Pts',(-48.706329375,28.437500006828,-1.8898197019151E-14));
#11262=CARTESIAN_POINT('Ctrl Pts',(-46.,60.,0.));
#11263=CARTESIAN_POINT('Ctrl Pts',(-46.,59.7916666666667,-12.3256628518316));
#11264=CARTESIAN_POINT('Ctrl Pts',(-39.8371685740842,59.5833333333333,-23.));
#11265=CARTESIAN_POINT('Ctrl Pts',(-33.6743371481684,59.375,-33.6743371481684));
#11266=CARTESIAN_POINT('Ctrl Pts',(-23.,59.1666666666667,-39.8371685740842));
#11267=CARTESIAN_POINT('Ctrl Pts',(-12.3256628518317,58.9583333333333,-46.));
#11268=CARTESIAN_POINT('Ctrl Pts',(-2.81668763803891E-15,58.75,-46.));
#11269=CARTESIAN_POINT('Ctrl Pts',(12.3256628518316,58.5416666666667,-46.));
#11270=CARTESIAN_POINT('Ctrl Pts',(23.,58.3333333333333,-39.8371685740842));
#11271=CARTESIAN_POINT('Ctrl Pts',(33.6743371481683,58.125,-33.6743371481684));
#11272=CARTESIAN_POINT('Ctrl Pts',(39.8371685740842,57.9166666666667,-23.));
#11273=CARTESIAN_POINT('Ctrl Pts',(46.,57.7083333333333,-12.3256628518317));
#11274=CARTESIAN_POINT('Ctrl Pts',(46.,57.5,-5.63337527607782E-15));
#11275=CARTESIAN_POINT('Ctrl Pts',(46.,57.2916666666667,12.3256628518316));
#11276=CARTESIAN_POINT('Ctrl Pts',(39.8371685740842,57.0833333333333,23.));
#11277=CARTESIAN_POINT('Ctrl Pts',(33.6743371481684,56.875,33.6743371481683));
#11278=CARTESIAN_POINT('Ctrl Pts',(23.,56.6666666666667,39.8371685740842));
#11279=CARTESIAN_POINT('Ctrl Pts',(12.3256628518317,56.4583333333333,46.));
#11280=CARTESIAN_POINT('Ctrl Pts',(8.45006291411674E-15,56.25,46.));
#11281=CARTESIAN_POINT('Ctrl Pts',(-12.3256628518316,56.0416666666667,46.));
#11282=CARTESIAN_POINT('Ctrl Pts',(-23.,55.8333333333333,39.8371685740842));
#11283=CARTESIAN_POINT('Ctrl Pts',(-33.6743371481683,55.625,33.6743371481684));
#11284=CARTESIAN_POINT('Ctrl Pts',(-39.8371685740842,55.4166666666667,23.));
#11285=CARTESIAN_POINT('Ctrl Pts',(-46.,55.2083333333333,12.3256628518317));
#11286=CARTESIAN_POINT('Ctrl Pts',(-46.,55.,0.));
#11287=CARTESIAN_POINT('Ctrl Pts',(-46.,54.7916666666667,-12.3256628518316));
#11288=CARTESIAN_POINT('Ctrl Pts',(-39.8371685740842,54.5833333333333,-23.));
#11289=CARTESIAN_POINT('Ctrl Pts',(-33.6743371481684,54.375,-33.6743371481684));
#11290=CARTESIAN_POINT('Ctrl Pts',(-23.,54.1666666666667,-39.8371685740842));
#11291=CARTESIAN_POINT('Ctrl Pts',(-12.3256628518317,53.9583333333333,-46.));
#11292=CARTESIAN_POINT('Ctrl Pts',(-2.81668763803891E-15,53.75,-46.));
#11293=CARTESIAN_POINT('Ctrl Pts',(12.3256628518316,53.5416666666667,-46.));
#11294=CARTESIAN_POINT('Ctrl Pts',(23.,53.3333333333333,-39.8371685740842));
#11295=CARTESIAN_POINT('Ctrl Pts',(33.6743371481683,53.125,-33.6743371481684));
#11296=CARTESIAN_POINT('Ctrl Pts',(39.8371685740842,52.9166666666667,-23.));
#11297=CARTESIAN_POINT('Ctrl Pts',(46.,52.7083333333333,-12.3256628518317));
#11298=CARTESIAN_POINT('Ctrl Pts',(46.,52.5,-5.63337527607782E-15));
#11299=CARTESIAN_POINT('Ctrl Pts',(46.,52.2916666666667,12.3256628518316));
#11300=CARTESIAN_POINT('Ctrl Pts',(39.8371685740842,52.0833333333333,23.));
#11301=CARTESIAN_POINT('Ctrl Pts',(33.6743371481684,51.875,33.6743371481683));
#11302=CARTESIAN_POINT('Ctrl Pts',(23.,51.6666666666667,39.8371685740842));
#11303=CARTESIAN_POINT('Ctrl Pts',(12.3256628518317,51.4583333333333,46.));
#11304=CARTESIAN_POINT('Ctrl Pts',(8.45006291411674E-15,51.25,46.));
#11305=CARTESIAN_POINT('Ctrl Pts',(-12.3256628518316,51.0416666666667,46.));
#11306=CARTESIAN_POINT('Ctrl Pts',(-23.,50.8333333333333,39.8371685740842));
#11307=CARTESIAN_POINT('Ctrl Pts',(-33.6743371481683,50.625,33.6743371481684));
#11308=CARTESIAN_POINT('Ctrl Pts',(-39.8371685740842,50.4166666666667,23.));
#11309=CARTESIAN_POINT('Ctrl Pts',(-46.,50.2083333333333,12.3256628518317));
#11310=CARTESIAN_POINT('Ctrl Pts',(-46.,50.,0.));
#11311=CARTESIAN_POINT('Ctrl Pts',(-46.,49.7916666666667,-12.3256628518316));
#11312=CARTESIAN_POINT('Ctrl Pts',(-39.8371685740842,49.5833333333333,-23.));
#11313=CARTESIAN_POINT('Ctrl Pts',(-33.6743371481684,49.375,-33.6743371481684));
#11314=CARTESIAN_POINT('Ctrl Pts',(-23.,49.1666666666667,-39.8371685740842));
#11315=CARTESIAN_POINT('Ctrl Pts',(-12.3256628518317,48.9583333333333,-46.));
#11316=CARTESIAN_POINT('Ctrl Pts',(-2.81668763803891E-15,48.75,-46.));
#11317=CARTESIAN_POINT('Ctrl Pts',(12.3256628518316,48.5416666666667,-46.));
#11318=CARTESIAN_POINT('Ctrl Pts',(23.,48.3333333333333,-39.8371685740842));
#11319=CARTESIAN_POINT('Ctrl Pts',(33.6743371481683,48.125,-33.6743371481684));
#11320=CARTESIAN_POINT('Ctrl Pts',(39.8371685740842,47.9166666666667,-23.));
#11321=CARTESIAN_POINT('Ctrl Pts',(46.,47.7083333333333,-12.3256628518317));
#11322=CARTESIAN_POINT('Ctrl Pts',(46.,47.5,-5.63337527607782E-15));
#11323=CARTESIAN_POINT('Ctrl Pts',(46.,47.2916666666667,12.3256628518316));
#11324=CARTESIAN_POINT('Ctrl Pts',(39.8371685740842,47.0833333333333,23.));
#11325=CARTESIAN_POINT('Ctrl Pts',(33.6743371481684,46.875,33.6743371481683));
#11326=CARTESIAN_POINT('Ctrl Pts',(23.,46.6666666666667,39.8371685740842));
#11327=CARTESIAN_POINT('Ctrl Pts',(12.3256628518317,46.4583333333333,46.));
#11328=CARTESIAN_POINT('Ctrl Pts',(8.45006291411674E-15,46.25,46.));
#11329=CARTESIAN_POINT('Ctrl Pts',(-12.3256628518316,46.0416666666667,46.));
#11330=CARTESIAN_POINT('Ctrl Pts',(-23.,45.8333333333333,39.8371685740842));
#11331=CARTESIAN_POINT('Ctrl Pts',(-33.6743371481683,45.625,33.6743371481684));
#11332=CARTESIAN_POINT('Ctrl Pts',(-39.8371685740842,45.4166666666667,23.));
#11333=CARTESIAN_POINT('Ctrl Pts',(-46.,45.2083333333333,12.3256628518317));
#11334=CARTESIAN_POINT('Ctrl Pts',(-46.,45.,0.));
#11335=CARTESIAN_POINT('Ctrl Pts',(-46.,44.7916666666667,-12.3256628518316));
#11336=CARTESIAN_POINT('Ctrl Pts',(-39.8371685740842,44.5833333333333,-23.));
#11337=CARTESIAN_POINT('Ctrl Pts',(-33.6743371481684,44.375,-33.6743371481684));
#11338=CARTESIAN_POINT('Ctrl Pts',(-23.,44.1666666666667,-39.8371685740842));
#11339=CARTESIAN_POINT('Ctrl Pts',(-12.3256628518317,43.9583333333333,-46.));
#11340=CARTESIAN_POINT('Ctrl Pts',(-2.81668763803891E-15,43.75,-46.));
#11341=CARTESIAN_POINT('Ctrl Pts',(12.3256628518316,43.5416666666667,-46.));
#11342=CARTESIAN_POINT('Ctrl Pts',(23.,43.3333333333333,-39.8371685740842));
#11343=CARTESIAN_POINT('Ctrl Pts',(33.6743371481683,43.125,-33.6743371481684));
#11344=CARTESIAN_POINT('Ctrl Pts',(39.8371685740842,42.9166666666667,-23.));
#11345=CARTESIAN_POINT('Ctrl Pts',(46.,42.7083333333333,-12.3256628518317));
#11346=CARTESIAN_POINT('Ctrl Pts',(46.,42.5,-5.63337527607782E-15));
#11347=CARTESIAN_POINT('Ctrl Pts',(46.,42.2916666666667,12.3256628518316));
#11348=CARTESIAN_POINT('Ctrl Pts',(39.8371685740842,42.0833333333333,23.));
#11349=CARTESIAN_POINT('Ctrl Pts',(33.6743371481684,41.875,33.6743371481683));
#11350=CARTESIAN_POINT('Ctrl Pts',(23.,41.6666666666667,39.8371685740842));
#11351=CARTESIAN_POINT('Ctrl Pts',(12.3256628518317,41.4583333333333,46.));
#11352=CARTESIAN_POINT('Ctrl Pts',(8.45006291411674E-15,41.25,46.));
#11353=CARTESIAN_POINT('Ctrl Pts',(-12.3256628518316,41.0416666666667,46.));
#11354=CARTESIAN_POINT('Ctrl Pts',(-23.,40.8333333333333,39.8371685740842));
#11355=CARTESIAN_POINT('Ctrl Pts',(-33.6743371481683,40.625,33.6743371481684));
#11356=CARTESIAN_POINT('Ctrl Pts',(-39.8371685740842,40.4166666666667,23.));
#11357=CARTESIAN_POINT('Ctrl Pts',(-46.,40.2083333333333,12.3256628518317));
#11358=CARTESIAN_POINT('Ctrl Pts',(-46.,40.,0.));
#11359=CARTESIAN_POINT('Ctrl Pts',(-46.,39.7916666666667,-12.3256628518316));
#11360=CARTESIAN_POINT('Ctrl Pts',(-39.8371685740842,39.5833333333333,-23.));
#11361=CARTESIAN_POINT('Ctrl Pts',(-33.6743371481684,39.375,-33.6743371481684));
#11362=CARTESIAN_POINT('Ctrl Pts',(-23.,39.1666666666667,-39.8371685740842));
#11363=CARTESIAN_POINT('Ctrl Pts',(-12.3256628518317,38.9583333333333,-46.));
#11364=CARTESIAN_POINT('Ctrl Pts',(-2.81668763803891E-15,38.75,-46.));
#11365=CARTESIAN_POINT('Ctrl Pts',(12.3256628518316,38.5416666666667,-46.));
#11366=CARTESIAN_POINT('Ctrl Pts',(23.,38.3333333333333,-39.8371685740842));
#11367=CARTESIAN_POINT('Ctrl Pts',(33.6743371481683,38.125,-33.6743371481684));
#11368=CARTESIAN_POINT('Ctrl Pts',(39.8371685740842,37.9166666666667,-23.));
#11369=CARTESIAN_POINT('Ctrl Pts',(46.,37.7083333333333,-12.3256628518317));
#11370=CARTESIAN_POINT('Ctrl Pts',(46.,37.5,-5.63337527607782E-15));
#11371=CARTESIAN_POINT('Ctrl Pts',(46.,37.2916666666667,12.3256628518316));
#11372=CARTESIAN_POINT('Ctrl Pts',(39.8371685740842,37.0833333333333,23.));
#11373=CARTESIAN_POINT('Ctrl Pts',(33.6743371481684,36.875,33.6743371481683));
#11374=CARTESIAN_POINT('Ctrl Pts',(23.,36.6666666666667,39.8371685740842));
#11375=CARTESIAN_POINT('Ctrl Pts',(12.3256628518317,36.4583333333333,46.));
#11376=CARTESIAN_POINT('Ctrl Pts',(8.45006291411674E-15,36.25,46.));
#11377=CARTESIAN_POINT('Ctrl Pts',(-12.3256628518316,36.0416666666667,46.));
#11378=CARTESIAN_POINT('Ctrl Pts',(-23.,35.8333333333333,39.8371685740842));
#11379=CARTESIAN_POINT('Ctrl Pts',(-33.6743371481683,35.625,33.6743371481684));
#11380=CARTESIAN_POINT('Ctrl Pts',(-39.8371685740842,35.4166666666667,23.));
#11381=CARTESIAN_POINT('Ctrl Pts',(-46.,35.2083333333333,12.3256628518317));
#11382=CARTESIAN_POINT('Ctrl Pts',(-46.,35.,0.));
#11383=CARTESIAN_POINT('Ctrl Pts',(-46.,34.7916666666667,-12.3256628518316));
#11384=CARTESIAN_POINT('Ctrl Pts',(-39.8371685740842,34.5833333333333,-23.));
#11385=CARTESIAN_POINT('Ctrl Pts',(-33.6743371481684,34.375,-33.6743371481684));
#11386=CARTESIAN_POINT('Ctrl Pts',(-23.,34.1666666666667,-39.8371685740842));
#11387=CARTESIAN_POINT('Ctrl Pts',(-12.3256628518317,33.9583333333333,-46.));
#11388=CARTESIAN_POINT('Ctrl Pts',(-2.81668763803891E-15,33.75,-46.));
#11389=CARTESIAN_POINT('Ctrl Pts',(12.3256628518316,33.5416666666667,-46.));
#11390=CARTESIAN_POINT('Ctrl Pts',(23.,33.3333333333333,-39.8371685740842));
#11391=CARTESIAN_POINT('Ctrl Pts',(33.6743371481683,33.125,-33.6743371481684));
#11392=CARTESIAN_POINT('Ctrl Pts',(39.8371685740842,32.9166666666667,-23.));
#11393=CARTESIAN_POINT('Ctrl Pts',(46.,32.7083333333333,-12.3256628518317));
#11394=CARTESIAN_POINT('Ctrl Pts',(46.,32.5,-5.63337527607782E-15));
#11395=CARTESIAN_POINT('Ctrl Pts',(46.,32.2916666666667,12.3256628518316));
#11396=CARTESIAN_POINT('Ctrl Pts',(39.8371685740842,32.0833333333333,23.));
#11397=CARTESIAN_POINT('Ctrl Pts',(33.6743371481684,31.875,33.6743371481683));
#11398=CARTESIAN_POINT('Ctrl Pts',(23.,31.6666666666667,39.8371685740842));
#11399=CARTESIAN_POINT('Ctrl Pts',(12.3256628518317,31.4583333333333,46.));
#11400=CARTESIAN_POINT('Ctrl Pts',(8.45006291411674E-15,31.25,46.));
#11401=CARTESIAN_POINT('Ctrl Pts',(-12.3256628518316,31.0416666666667,46.));
#11402=CARTESIAN_POINT('Ctrl Pts',(-23.,30.8333333333333,39.8371685740842));
#11403=CARTESIAN_POINT('Ctrl Pts',(-33.6743371481683,30.625,33.6743371481684));
#11404=CARTESIAN_POINT('Ctrl Pts',(-39.8371685740842,30.4166666666667,23.));
#11405=CARTESIAN_POINT('Ctrl Pts',(-46.,30.2083333333333,12.3256628518317));
#11406=CARTESIAN_POINT('Ctrl Pts',(-46.,30.,0.));
#11407=CARTESIAN_POINT('',(15.5677347613557,57.,-46.0186009836189));
#11408=CARTESIAN_POINT('',(46.79170203032,56.9999999999858,-4.33048599679673));
#11409=CARTESIAN_POINT('Ctrl Pts',(15.5677347613557,57.,-46.0186009836189));
#11410=CARTESIAN_POINT('Ctrl Pts',(17.7310349698886,57.,-45.2170526223414));
#11411=CARTESIAN_POINT('Ctrl Pts',(19.834567405171,57.0000000000088,-44.2626483761178));
#11412=CARTESIAN_POINT('Ctrl Pts',(23.9079865381294,57.0000000000088,-42.0529745645465));
#11413=CARTESIAN_POINT('Ctrl Pts',(25.8779679347109,57.,-40.7943833295357));
#11414=CARTESIAN_POINT('Ctrl Pts',(31.3891578561493,57.,-36.6723214087039));
#11415=CARTESIAN_POINT('Ctrl Pts',(34.6227678874526,57.,-33.4466510749012));
#11416=CARTESIAN_POINT('Ctrl Pts',(40.1411508117922,57.,-26.1061863972564));
#11417=CARTESIAN_POINT('Ctrl Pts',(42.3917117517447,57.,-21.991753538455));
#11418=CARTESIAN_POINT('Ctrl Pts',(45.5641231823138,57.,-13.3433502223045));
#11419=CARTESIAN_POINT('Ctrl Pts',(46.5051362525069,57.,-8.86952477496529));
#11420=CARTESIAN_POINT('Ctrl Pts',(46.7917020302955,57.,-4.33048599679518));
#11421=CARTESIAN_POINT('Ctrl Pts',(46.79170203032,56.9999999999858,-4.33048599679673));
#11422=CARTESIAN_POINT('Ctrl Pts',(46.9229272270402,56.92435531248,-4.33048599679673));
#11423=CARTESIAN_POINT('Ctrl Pts',(47.0541520004637,56.8487098906525,-4.33048599679673));
#11424=CARTESIAN_POINT('Ctrl Pts',(47.6280672732221,56.5178683162597,-4.33048599679673));
#11425=CARTESIAN_POINT('Ctrl Pts',(48.0707534890442,56.2626647328764,-4.33048599679674));
#11426=CARTESIAN_POINT('Ctrl Pts',(48.5134353784344,56.0074536451604,-4.33048599679673));
#11427=CARTESIAN_POINT('',(3.612927284338,57.2017412484791,-48.4459777332189));
#11428=CARTESIAN_POINT('',(3.61292728433799,57.1292520480092,-48.5721450795008));
#11429=CARTESIAN_POINT('Origin',(-0.00341856678684749,57.0518082227792,
0.0127587930744433));
#11430=CARTESIAN_POINT('Ctrl Pts',(-48.706329375,58.437500006828,-1.8898197019151E-14));
#11431=CARTESIAN_POINT('Ctrl Pts',(-48.706329375,58.2291666734946,-13.0508216223155));
#11432=CARTESIAN_POINT('Ctrl Pts',(-42.1809185638422,58.0208333401613,-24.3531646875));
#11433=CARTESIAN_POINT('Ctrl Pts',(-35.6555077526845,57.812500006828,-35.6555077526845));
#11434=CARTESIAN_POINT('Ctrl Pts',(-24.3531646875,57.6041666734946,-42.1809185638422));
#11435=CARTESIAN_POINT('Ctrl Pts',(-13.0508216223155,57.3958333401613,-48.706329375));
#11436=CARTESIAN_POINT('Ctrl Pts',(1.59157945007855E-14,57.187500006828,
-48.706329375));
#11437=CARTESIAN_POINT('Ctrl Pts',(13.0508216223155,56.9791666734946,-48.706329375));
#11438=CARTESIAN_POINT('Ctrl Pts',(24.3531646875,56.7708333401613,-42.1809185638422));
#11439=CARTESIAN_POINT('Ctrl Pts',(35.6555077526845,56.562500006828,-35.6555077526845));
#11440=CARTESIAN_POINT('Ctrl Pts',(42.1809185638422,56.3541666734946,-24.3531646875));
#11441=CARTESIAN_POINT('Ctrl Pts',(48.706329375,56.1458333401613,-13.0508216223155));
#11442=CARTESIAN_POINT('Ctrl Pts',(48.706329375,55.937500006828,1.293339198242E-14));
#11443=CARTESIAN_POINT('Ctrl Pts',(48.706329375,55.7291666734946,13.0508216223155));
#11444=CARTESIAN_POINT('Ctrl Pts',(42.1809185638422,55.5208333401613,24.3531646875));
#11445=CARTESIAN_POINT('Ctrl Pts',(35.6555077526845,55.312500006828,35.6555077526845));
#11446=CARTESIAN_POINT('Ctrl Pts',(24.3531646875,55.1041666734946,42.1809185638422));
#11447=CARTESIAN_POINT('Ctrl Pts',(13.0508216223155,54.8958333401613,48.706329375));
#11448=CARTESIAN_POINT('Ctrl Pts',(-9.95098946405443E-15,54.687500006828,
48.706329375));
#11449=CARTESIAN_POINT('Ctrl Pts',(-13.0508216223155,54.4791666734946,48.706329375));
#11450=CARTESIAN_POINT('Ctrl Pts',(-24.3531646875,54.2708333401613,42.1809185638423));
#11451=CARTESIAN_POINT('Ctrl Pts',(-35.6555077526845,54.062500006828,35.6555077526845));
#11452=CARTESIAN_POINT('Ctrl Pts',(-42.1809185638422,53.8541666734946,24.3531646875));
#11453=CARTESIAN_POINT('Ctrl Pts',(-48.706329375,53.6458333401613,13.0508216223155));
#11454=CARTESIAN_POINT('Ctrl Pts',(-48.706329375,53.437500006828,-1.8898197019151E-14));
#11455=CARTESIAN_POINT('Ctrl Pts',(-48.706329375,53.2291666734946,-13.0508216223155));
#11456=CARTESIAN_POINT('Ctrl Pts',(-42.1809185638422,53.0208333401613,-24.3531646875));
#11457=CARTESIAN_POINT('Ctrl Pts',(-35.6555077526845,52.812500006828,-35.6555077526845));
#11458=CARTESIAN_POINT('Ctrl Pts',(-24.3531646875,52.6041666734946,-42.1809185638422));
#11459=CARTESIAN_POINT('Ctrl Pts',(-13.0508216223155,52.3958333401613,-48.706329375));
#11460=CARTESIAN_POINT('Ctrl Pts',(1.59157945007855E-14,52.187500006828,
-48.706329375));
#11461=CARTESIAN_POINT('Ctrl Pts',(13.0508216223155,51.9791666734946,-48.706329375));
#11462=CARTESIAN_POINT('Ctrl Pts',(24.3531646875,51.7708333401613,-42.1809185638422));
#11463=CARTESIAN_POINT('Ctrl Pts',(35.6555077526845,51.562500006828,-35.6555077526845));
#11464=CARTESIAN_POINT('Ctrl Pts',(42.1809185638422,51.3541666734946,-24.3531646875));
#11465=CARTESIAN_POINT('Ctrl Pts',(48.706329375,51.1458333401613,-13.0508216223155));
#11466=CARTESIAN_POINT('Ctrl Pts',(48.706329375,50.937500006828,1.293339198242E-14));
#11467=CARTESIAN_POINT('Ctrl Pts',(48.706329375,50.7291666734946,13.0508216223155));
#11468=CARTESIAN_POINT('Ctrl Pts',(42.1809185638422,50.5208333401613,24.3531646875));
#11469=CARTESIAN_POINT('Ctrl Pts',(35.6555077526845,50.312500006828,35.6555077526845));
#11470=CARTESIAN_POINT('Ctrl Pts',(24.3531646875,50.1041666734946,42.1809185638422));
#11471=CARTESIAN_POINT('Ctrl Pts',(13.0508216223155,49.8958333401613,48.706329375));
#11472=CARTESIAN_POINT('Ctrl Pts',(-9.95098946405443E-15,49.687500006828,
48.706329375));
#11473=CARTESIAN_POINT('Ctrl Pts',(-13.0508216223155,49.4791666734946,48.706329375));
#11474=CARTESIAN_POINT('Ctrl Pts',(-24.3531646875,49.2708333401613,42.1809185638423));
#11475=CARTESIAN_POINT('Ctrl Pts',(-35.6555077526845,49.062500006828,35.6555077526845));
#11476=CARTESIAN_POINT('Ctrl Pts',(-42.1809185638422,48.8541666734946,24.3531646875));
#11477=CARTESIAN_POINT('Ctrl Pts',(-48.706329375,48.6458333401613,13.0508216223155));
#11478=CARTESIAN_POINT('Ctrl Pts',(-48.706329375,48.437500006828,-1.8898197019151E-14));
#11479=CARTESIAN_POINT('Ctrl Pts',(-48.706329375,48.2291666734946,-13.0508216223155));
#11480=CARTESIAN_POINT('Ctrl Pts',(-42.1809185638422,48.0208333401613,-24.3531646875));
#11481=CARTESIAN_POINT('Ctrl Pts',(-35.6555077526845,47.812500006828,-35.6555077526845));
#11482=CARTESIAN_POINT('Ctrl Pts',(-24.3531646875,47.6041666734946,-42.1809185638422));
#11483=CARTESIAN_POINT('Ctrl Pts',(-13.0508216223155,47.3958333401613,-48.706329375));
#11484=CARTESIAN_POINT('Ctrl Pts',(1.59157945007855E-14,47.187500006828,
-48.706329375));
#11485=CARTESIAN_POINT('Ctrl Pts',(13.0508216223155,46.9791666734946,-48.706329375));
#11486=CARTESIAN_POINT('Ctrl Pts',(24.3531646875,46.7708333401613,-42.1809185638422));
#11487=CARTESIAN_POINT('Ctrl Pts',(35.6555077526845,46.562500006828,-35.6555077526845));
#11488=CARTESIAN_POINT('Ctrl Pts',(42.1809185638422,46.3541666734946,-24.3531646875));
#11489=CARTESIAN_POINT('Ctrl Pts',(48.706329375,46.1458333401613,-13.0508216223155));
#11490=CARTESIAN_POINT('Ctrl Pts',(48.706329375,45.937500006828,1.293339198242E-14));
#11491=CARTESIAN_POINT('Ctrl Pts',(48.706329375,45.7291666734946,13.0508216223155));
#11492=CARTESIAN_POINT('Ctrl Pts',(42.1809185638422,45.5208333401613,24.3531646875));
#11493=CARTESIAN_POINT('Ctrl Pts',(35.6555077526845,45.312500006828,35.6555077526845));
#11494=CARTESIAN_POINT('Ctrl Pts',(24.3531646875,45.1041666734946,42.1809185638422));
#11495=CARTESIAN_POINT('Ctrl Pts',(13.0508216223155,44.8958333401613,48.706329375));
#11496=CARTESIAN_POINT('Ctrl Pts',(-9.95098946405443E-15,44.687500006828,
48.706329375));
#11497=CARTESIAN_POINT('Ctrl Pts',(-13.0508216223155,44.4791666734946,48.706329375));
#11498=CARTESIAN_POINT('Ctrl Pts',(-24.3531646875,44.2708333401613,42.1809185638423));
#11499=CARTESIAN_POINT('Ctrl Pts',(-35.6555077526845,44.062500006828,35.6555077526845));
#11500=CARTESIAN_POINT('Ctrl Pts',(-42.1809185638422,43.8541666734946,24.3531646875));
#11501=CARTESIAN_POINT('Ctrl Pts',(-48.706329375,43.6458333401613,13.0508216223155));
#11502=CARTESIAN_POINT('Ctrl Pts',(-48.706329375,43.437500006828,-1.8898197019151E-14));
#11503=CARTESIAN_POINT('Ctrl Pts',(-48.706329375,43.2291666734946,-13.0508216223155));
#11504=CARTESIAN_POINT('Ctrl Pts',(-42.1809185638422,43.0208333401613,-24.3531646875));
#11505=CARTESIAN_POINT('Ctrl Pts',(-35.6555077526845,42.812500006828,-35.6555077526845));
#11506=CARTESIAN_POINT('Ctrl Pts',(-24.3531646875,42.6041666734946,-42.1809185638422));
#11507=CARTESIAN_POINT('Ctrl Pts',(-13.0508216223155,42.3958333401613,-48.706329375));
#11508=CARTESIAN_POINT('Ctrl Pts',(1.59157945007855E-14,42.187500006828,
-48.706329375));
#11509=CARTESIAN_POINT('Ctrl Pts',(13.0508216223155,41.9791666734946,-48.706329375));
#11510=CARTESIAN_POINT('Ctrl Pts',(24.3531646875,41.7708333401613,-42.1809185638422));
#11511=CARTESIAN_POINT('Ctrl Pts',(35.6555077526845,41.562500006828,-35.6555077526845));
#11512=CARTESIAN_POINT('Ctrl Pts',(42.1809185638422,41.3541666734946,-24.3531646875));
#11513=CARTESIAN_POINT('Ctrl Pts',(48.706329375,41.1458333401613,-13.0508216223155));
#11514=CARTESIAN_POINT('Ctrl Pts',(48.706329375,40.937500006828,1.293339198242E-14));
#11515=CARTESIAN_POINT('Ctrl Pts',(48.706329375,40.7291666734946,13.0508216223155));
#11516=CARTESIAN_POINT('Ctrl Pts',(42.1809185638422,40.5208333401613,24.3531646875));
#11517=CARTESIAN_POINT('Ctrl Pts',(35.6555077526845,40.312500006828,35.6555077526845));
#11518=CARTESIAN_POINT('Ctrl Pts',(24.3531646875,40.1041666734946,42.1809185638422));
#11519=CARTESIAN_POINT('Ctrl Pts',(13.0508216223155,39.8958333401613,48.706329375));
#11520=CARTESIAN_POINT('Ctrl Pts',(-9.95098946405443E-15,39.687500006828,
48.706329375));
#11521=CARTESIAN_POINT('Ctrl Pts',(-13.0508216223155,39.4791666734946,48.706329375));
#11522=CARTESIAN_POINT('Ctrl Pts',(-24.3531646875,39.2708333401613,42.1809185638423));
#11523=CARTESIAN_POINT('Ctrl Pts',(-35.6555077526845,39.062500006828,35.6555077526845));
#11524=CARTESIAN_POINT('Ctrl Pts',(-42.1809185638422,38.8541666734946,24.3531646875));
#11525=CARTESIAN_POINT('Ctrl Pts',(-48.706329375,38.6458333401613,13.0508216223155));
#11526=CARTESIAN_POINT('Ctrl Pts',(-48.706329375,38.437500006828,-1.8898197019151E-14));
#11527=CARTESIAN_POINT('Ctrl Pts',(-48.706329375,38.2291666734946,-13.0508216223155));
#11528=CARTESIAN_POINT('Ctrl Pts',(-42.1809185638422,38.0208333401613,-24.3531646875));
#11529=CARTESIAN_POINT('Ctrl Pts',(-35.6555077526845,37.812500006828,-35.6555077526845));
#11530=CARTESIAN_POINT('Ctrl Pts',(-24.3531646875,37.6041666734946,-42.1809185638422));
#11531=CARTESIAN_POINT('Ctrl Pts',(-13.0508216223155,37.3958333401613,-48.706329375));
#11532=CARTESIAN_POINT('Ctrl Pts',(1.59157945007855E-14,37.187500006828,
-48.706329375));
#11533=CARTESIAN_POINT('Ctrl Pts',(13.0508216223155,36.9791666734946,-48.706329375));
#11534=CARTESIAN_POINT('Ctrl Pts',(24.3531646875,36.7708333401613,-42.1809185638422));
#11535=CARTESIAN_POINT('Ctrl Pts',(35.6555077526845,36.562500006828,-35.6555077526845));
#11536=CARTESIAN_POINT('Ctrl Pts',(42.1809185638422,36.3541666734946,-24.3531646875));
#11537=CARTESIAN_POINT('Ctrl Pts',(48.706329375,36.1458333401613,-13.0508216223155));
#11538=CARTESIAN_POINT('Ctrl Pts',(48.706329375,35.937500006828,1.293339198242E-14));
#11539=CARTESIAN_POINT('Ctrl Pts',(48.706329375,35.7291666734946,13.0508216223155));
#11540=CARTESIAN_POINT('Ctrl Pts',(42.1809185638422,35.5208333401613,24.3531646875));
#11541=CARTESIAN_POINT('Ctrl Pts',(35.6555077526845,35.312500006828,35.6555077526845));
#11542=CARTESIAN_POINT('Ctrl Pts',(24.3531646875,35.1041666734946,42.1809185638422));
#11543=CARTESIAN_POINT('Ctrl Pts',(13.0508216223155,34.8958333401613,48.706329375));
#11544=CARTESIAN_POINT('Ctrl Pts',(-9.95098946405443E-15,34.687500006828,
48.706329375));
#11545=CARTESIAN_POINT('Ctrl Pts',(-13.0508216223155,34.4791666734946,48.706329375));
#11546=CARTESIAN_POINT('Ctrl Pts',(-24.3531646875,34.2708333401613,42.1809185638423));
#11547=CARTESIAN_POINT('Ctrl Pts',(-35.6555077526845,34.062500006828,35.6555077526845));
#11548=CARTESIAN_POINT('Ctrl Pts',(-42.1809185638422,33.8541666734946,24.3531646875));
#11549=CARTESIAN_POINT('Ctrl Pts',(-48.706329375,33.6458333401613,13.0508216223155));
#11550=CARTESIAN_POINT('Ctrl Pts',(-48.706329375,33.437500006828,-1.8898197019151E-14));
#11551=CARTESIAN_POINT('Ctrl Pts',(-48.706329375,33.2291666734946,-13.0508216223155));
#11552=CARTESIAN_POINT('Ctrl Pts',(-42.1809185638422,33.0208333401613,-24.3531646875));
#11553=CARTESIAN_POINT('Ctrl Pts',(-35.6555077526845,32.812500006828,-35.6555077526845));
#11554=CARTESIAN_POINT('Ctrl Pts',(-24.3531646875,32.6041666734946,-42.1809185638422));
#11555=CARTESIAN_POINT('Ctrl Pts',(-13.0508216223155,32.3958333401613,-48.706329375));
#11556=CARTESIAN_POINT('Ctrl Pts',(1.59157945007855E-14,32.187500006828,
-48.706329375));
#11557=CARTESIAN_POINT('Ctrl Pts',(13.0508216223155,31.9791666734946,-48.706329375));
#11558=CARTESIAN_POINT('Ctrl Pts',(24.3531646875,31.7708333401613,-42.1809185638422));
#11559=CARTESIAN_POINT('Ctrl Pts',(35.6555077526845,31.562500006828,-35.6555077526845));
#11560=CARTESIAN_POINT('Ctrl Pts',(42.1809185638422,31.3541666734946,-24.3531646875));
#11561=CARTESIAN_POINT('Ctrl Pts',(48.706329375,31.1458333401613,-13.0508216223155));
#11562=CARTESIAN_POINT('Ctrl Pts',(48.706329375,30.937500006828,1.293339198242E-14));
#11563=CARTESIAN_POINT('Ctrl Pts',(48.706329375,30.7291666734946,13.0508216223155));
#11564=CARTESIAN_POINT('Ctrl Pts',(42.1809185638422,30.5208333401613,24.3531646875));
#11565=CARTESIAN_POINT('Ctrl Pts',(35.6555077526845,30.312500006828,35.6555077526845));
#11566=CARTESIAN_POINT('Ctrl Pts',(24.3531646875,30.1041666734946,42.1809185638422));
#11567=CARTESIAN_POINT('Ctrl Pts',(13.0508216223155,29.8958333401613,48.706329375));
#11568=CARTESIAN_POINT('Ctrl Pts',(-9.95098946405443E-15,29.687500006828,
48.706329375));
#11569=CARTESIAN_POINT('Ctrl Pts',(-13.0508216223155,29.4791666734946,48.706329375));
#11570=CARTESIAN_POINT('Ctrl Pts',(-24.3531646875,29.2708333401613,42.1809185638423));
#11571=CARTESIAN_POINT('Ctrl Pts',(-35.6555077526845,29.062500006828,35.6555077526845));
#11572=CARTESIAN_POINT('Ctrl Pts',(-42.1809185638422,28.8541666734946,24.3531646875));
#11573=CARTESIAN_POINT('Ctrl Pts',(-48.706329375,28.6458333401613,13.0508216223155));
#11574=CARTESIAN_POINT('Ctrl Pts',(-48.706329375,28.437500006828,-1.8898197019151E-14));
#11575=CARTESIAN_POINT('Ctrl Pts',(-46.,60.,0.));
#11576=CARTESIAN_POINT('Ctrl Pts',(-46.,59.7916666666667,-12.3256628518316));
#11577=CARTESIAN_POINT('Ctrl Pts',(-39.8371685740842,59.5833333333333,-23.));
#11578=CARTESIAN_POINT('Ctrl Pts',(-33.6743371481684,59.375,-33.6743371481684));
#11579=CARTESIAN_POINT('Ctrl Pts',(-23.,59.1666666666667,-39.8371685740842));
#11580=CARTESIAN_POINT('Ctrl Pts',(-12.3256628518317,58.9583333333333,-46.));
#11581=CARTESIAN_POINT('Ctrl Pts',(-2.81668763803891E-15,58.75,-46.));
#11582=CARTESIAN_POINT('Ctrl Pts',(12.3256628518316,58.5416666666667,-46.));
#11583=CARTESIAN_POINT('Ctrl Pts',(23.,58.3333333333333,-39.8371685740842));
#11584=CARTESIAN_POINT('Ctrl Pts',(33.6743371481683,58.125,-33.6743371481684));
#11585=CARTESIAN_POINT('Ctrl Pts',(39.8371685740842,57.9166666666667,-23.));
#11586=CARTESIAN_POINT('Ctrl Pts',(46.,57.7083333333333,-12.3256628518317));
#11587=CARTESIAN_POINT('Ctrl Pts',(46.,57.5,-5.63337527607782E-15));
#11588=CARTESIAN_POINT('Ctrl Pts',(46.,57.2916666666667,12.3256628518316));
#11589=CARTESIAN_POINT('Ctrl Pts',(39.8371685740842,57.0833333333333,23.));
#11590=CARTESIAN_POINT('Ctrl Pts',(33.6743371481684,56.875,33.6743371481683));
#11591=CARTESIAN_POINT('Ctrl Pts',(23.,56.6666666666667,39.8371685740842));
#11592=CARTESIAN_POINT('Ctrl Pts',(12.3256628518317,56.4583333333333,46.));
#11593=CARTESIAN_POINT('Ctrl Pts',(8.45006291411674E-15,56.25,46.));
#11594=CARTESIAN_POINT('Ctrl Pts',(-12.3256628518316,56.0416666666667,46.));
#11595=CARTESIAN_POINT('Ctrl Pts',(-23.,55.8333333333333,39.8371685740842));
#11596=CARTESIAN_POINT('Ctrl Pts',(-33.6743371481683,55.625,33.6743371481684));
#11597=CARTESIAN_POINT('Ctrl Pts',(-39.8371685740842,55.4166666666667,23.));
#11598=CARTESIAN_POINT('Ctrl Pts',(-46.,55.2083333333333,12.3256628518317));
#11599=CARTESIAN_POINT('Ctrl Pts',(-46.,55.,0.));
#11600=CARTESIAN_POINT('Ctrl Pts',(-46.,54.7916666666667,-12.3256628518316));
#11601=CARTESIAN_POINT('Ctrl Pts',(-39.8371685740842,54.5833333333333,-23.));
#11602=CARTESIAN_POINT('Ctrl Pts',(-33.6743371481684,54.375,-33.6743371481684));
#11603=CARTESIAN_POINT('Ctrl Pts',(-23.,54.1666666666667,-39.8371685740842));
#11604=CARTESIAN_POINT('Ctrl Pts',(-12.3256628518317,53.9583333333333,-46.));
#11605=CARTESIAN_POINT('Ctrl Pts',(-2.81668763803891E-15,53.75,-46.));
#11606=CARTESIAN_POINT('Ctrl Pts',(12.3256628518316,53.5416666666667,-46.));
#11607=CARTESIAN_POINT('Ctrl Pts',(23.,53.3333333333333,-39.8371685740842));
#11608=CARTESIAN_POINT('Ctrl Pts',(33.6743371481683,53.125,-33.6743371481684));
#11609=CARTESIAN_POINT('Ctrl Pts',(39.8371685740842,52.9166666666667,-23.));
#11610=CARTESIAN_POINT('Ctrl Pts',(46.,52.7083333333333,-12.3256628518317));
#11611=CARTESIAN_POINT('Ctrl Pts',(46.,52.5,-5.63337527607782E-15));
#11612=CARTESIAN_POINT('Ctrl Pts',(46.,52.2916666666667,12.3256628518316));
#11613=CARTESIAN_POINT('Ctrl Pts',(39.8371685740842,52.0833333333333,23.));
#11614=CARTESIAN_POINT('Ctrl Pts',(33.6743371481684,51.875,33.6743371481683));
#11615=CARTESIAN_POINT('Ctrl Pts',(23.,51.6666666666667,39.8371685740842));
#11616=CARTESIAN_POINT('Ctrl Pts',(12.3256628518317,51.4583333333333,46.));
#11617=CARTESIAN_POINT('Ctrl Pts',(8.45006291411674E-15,51.25,46.));
#11618=CARTESIAN_POINT('Ctrl Pts',(-12.3256628518316,51.0416666666667,46.));
#11619=CARTESIAN_POINT('Ctrl Pts',(-23.,50.8333333333333,39.8371685740842));
#11620=CARTESIAN_POINT('Ctrl Pts',(-33.6743371481683,50.625,33.6743371481684));
#11621=CARTESIAN_POINT('Ctrl Pts',(-39.8371685740842,50.4166666666667,23.));
#11622=CARTESIAN_POINT('Ctrl Pts',(-46.,50.2083333333333,12.3256628518317));
#11623=CARTESIAN_POINT('Ctrl Pts',(-46.,50.,0.));
#11624=CARTESIAN_POINT('Ctrl Pts',(-46.,49.7916666666667,-12.3256628518316));
#11625=CARTESIAN_POINT('Ctrl Pts',(-39.8371685740842,49.5833333333333,-23.));
#11626=CARTESIAN_POINT('Ctrl Pts',(-33.6743371481684,49.375,-33.6743371481684));
#11627=CARTESIAN_POINT('Ctrl Pts',(-23.,49.1666666666667,-39.8371685740842));
#11628=CARTESIAN_POINT('Ctrl Pts',(-12.3256628518317,48.9583333333333,-46.));
#11629=CARTESIAN_POINT('Ctrl Pts',(-2.81668763803891E-15,48.75,-46.));
#11630=CARTESIAN_POINT('Ctrl Pts',(12.3256628518316,48.5416666666667,-46.));
#11631=CARTESIAN_POINT('Ctrl Pts',(23.,48.3333333333333,-39.8371685740842));
#11632=CARTESIAN_POINT('Ctrl Pts',(33.6743371481683,48.125,-33.6743371481684));
#11633=CARTESIAN_POINT('Ctrl Pts',(39.8371685740842,47.9166666666667,-23.));
#11634=CARTESIAN_POINT('Ctrl Pts',(46.,47.7083333333333,-12.3256628518317));
#11635=CARTESIAN_POINT('Ctrl Pts',(46.,47.5,-5.63337527607782E-15));
#11636=CARTESIAN_POINT('Ctrl Pts',(46.,47.2916666666667,12.3256628518316));
#11637=CARTESIAN_POINT('Ctrl Pts',(39.8371685740842,47.0833333333333,23.));
#11638=CARTESIAN_POINT('Ctrl Pts',(33.6743371481684,46.875,33.6743371481683));
#11639=CARTESIAN_POINT('Ctrl Pts',(23.,46.6666666666667,39.8371685740842));
#11640=CARTESIAN_POINT('Ctrl Pts',(12.3256628518317,46.4583333333333,46.));
#11641=CARTESIAN_POINT('Ctrl Pts',(8.45006291411674E-15,46.25,46.));
#11642=CARTESIAN_POINT('Ctrl Pts',(-12.3256628518316,46.0416666666667,46.));
#11643=CARTESIAN_POINT('Ctrl Pts',(-23.,45.8333333333333,39.8371685740842));
#11644=CARTESIAN_POINT('Ctrl Pts',(-33.6743371481683,45.625,33.6743371481684));
#11645=CARTESIAN_POINT('Ctrl Pts',(-39.8371685740842,45.4166666666667,23.));
#11646=CARTESIAN_POINT('Ctrl Pts',(-46.,45.2083333333333,12.3256628518317));
#11647=CARTESIAN_POINT('Ctrl Pts',(-46.,45.,0.));
#11648=CARTESIAN_POINT('Ctrl Pts',(-46.,44.7916666666667,-12.3256628518316));
#11649=CARTESIAN_POINT('Ctrl Pts',(-39.8371685740842,44.5833333333333,-23.));
#11650=CARTESIAN_POINT('Ctrl Pts',(-33.6743371481684,44.375,-33.6743371481684));
#11651=CARTESIAN_POINT('Ctrl Pts',(-23.,44.1666666666667,-39.8371685740842));
#11652=CARTESIAN_POINT('Ctrl Pts',(-12.3256628518317,43.9583333333333,-46.));
#11653=CARTESIAN_POINT('Ctrl Pts',(-2.81668763803891E-15,43.75,-46.));
#11654=CARTESIAN_POINT('Ctrl Pts',(12.3256628518316,43.5416666666667,-46.));
#11655=CARTESIAN_POINT('Ctrl Pts',(23.,43.3333333333333,-39.8371685740842));
#11656=CARTESIAN_POINT('Ctrl Pts',(33.6743371481683,43.125,-33.6743371481684));
#11657=CARTESIAN_POINT('Ctrl Pts',(39.8371685740842,42.9166666666667,-23.));
#11658=CARTESIAN_POINT('Ctrl Pts',(46.,42.7083333333333,-12.3256628518317));
#11659=CARTESIAN_POINT('Ctrl Pts',(46.,42.5,-5.63337527607782E-15));
#11660=CARTESIAN_POINT('Ctrl Pts',(46.,42.2916666666667,12.3256628518316));
#11661=CARTESIAN_POINT('Ctrl Pts',(39.8371685740842,42.0833333333333,23.));
#11662=CARTESIAN_POINT('Ctrl Pts',(33.6743371481684,41.875,33.6743371481683));
#11663=CARTESIAN_POINT('Ctrl Pts',(23.,41.6666666666667,39.8371685740842));
#11664=CARTESIAN_POINT('Ctrl Pts',(12.3256628518317,41.4583333333333,46.));
#11665=CARTESIAN_POINT('Ctrl Pts',(8.45006291411674E-15,41.25,46.));
#11666=CARTESIAN_POINT('Ctrl Pts',(-12.3256628518316,41.0416666666667,46.));
#11667=CARTESIAN_POINT('Ctrl Pts',(-23.,40.8333333333333,39.8371685740842));
#11668=CARTESIAN_POINT('Ctrl Pts',(-33.6743371481683,40.625,33.6743371481684));
#11669=CARTESIAN_POINT('Ctrl Pts',(-39.8371685740842,40.4166666666667,23.));
#11670=CARTESIAN_POINT('Ctrl Pts',(-46.,40.2083333333333,12.3256628518317));
#11671=CARTESIAN_POINT('Ctrl Pts',(-46.,40.,0.));
#11672=CARTESIAN_POINT('Ctrl Pts',(-46.,39.7916666666667,-12.3256628518316));
#11673=CARTESIAN_POINT('Ctrl Pts',(-39.8371685740842,39.5833333333333,-23.));
#11674=CARTESIAN_POINT('Ctrl Pts',(-33.6743371481684,39.375,-33.6743371481684));
#11675=CARTESIAN_POINT('Ctrl Pts',(-23.,39.1666666666667,-39.8371685740842));
#11676=CARTESIAN_POINT('Ctrl Pts',(-12.3256628518317,38.9583333333333,-46.));
#11677=CARTESIAN_POINT('Ctrl Pts',(-2.81668763803891E-15,38.75,-46.));
#11678=CARTESIAN_POINT('Ctrl Pts',(12.3256628518316,38.5416666666667,-46.));
#11679=CARTESIAN_POINT('Ctrl Pts',(23.,38.3333333333333,-39.8371685740842));
#11680=CARTESIAN_POINT('Ctrl Pts',(33.6743371481683,38.125,-33.6743371481684));
#11681=CARTESIAN_POINT('Ctrl Pts',(39.8371685740842,37.9166666666667,-23.));
#11682=CARTESIAN_POINT('Ctrl Pts',(46.,37.7083333333333,-12.3256628518317));
#11683=CARTESIAN_POINT('Ctrl Pts',(46.,37.5,-5.63337527607782E-15));
#11684=CARTESIAN_POINT('Ctrl Pts',(46.,37.2916666666667,12.3256628518316));
#11685=CARTESIAN_POINT('Ctrl Pts',(39.8371685740842,37.0833333333333,23.));
#11686=CARTESIAN_POINT('Ctrl Pts',(33.6743371481684,36.875,33.6743371481683));
#11687=CARTESIAN_POINT('Ctrl Pts',(23.,36.6666666666667,39.8371685740842));
#11688=CARTESIAN_POINT('Ctrl Pts',(12.3256628518317,36.4583333333333,46.));
#11689=CARTESIAN_POINT('Ctrl Pts',(8.45006291411674E-15,36.25,46.));
#11690=CARTESIAN_POINT('Ctrl Pts',(-12.3256628518316,36.0416666666667,46.));
#11691=CARTESIAN_POINT('Ctrl Pts',(-23.,35.8333333333333,39.8371685740842));
#11692=CARTESIAN_POINT('Ctrl Pts',(-33.6743371481683,35.625,33.6743371481684));
#11693=CARTESIAN_POINT('Ctrl Pts',(-39.8371685740842,35.4166666666667,23.));
#11694=CARTESIAN_POINT('Ctrl Pts',(-46.,35.2083333333333,12.3256628518317));
#11695=CARTESIAN_POINT('Ctrl Pts',(-46.,35.,0.));
#11696=CARTESIAN_POINT('Ctrl Pts',(-46.,34.7916666666667,-12.3256628518316));
#11697=CARTESIAN_POINT('Ctrl Pts',(-39.8371685740842,34.5833333333333,-23.));
#11698=CARTESIAN_POINT('Ctrl Pts',(-33.6743371481684,34.375,-33.6743371481684));
#11699=CARTESIAN_POINT('Ctrl Pts',(-23.,34.1666666666667,-39.8371685740842));
#11700=CARTESIAN_POINT('Ctrl Pts',(-12.3256628518317,33.9583333333333,-46.));
#11701=CARTESIAN_POINT('Ctrl Pts',(-2.81668763803891E-15,33.75,-46.));
#11702=CARTESIAN_POINT('Ctrl Pts',(12.3256628518316,33.5416666666667,-46.));
#11703=CARTESIAN_POINT('Ctrl Pts',(23.,33.3333333333333,-39.8371685740842));
#11704=CARTESIAN_POINT('Ctrl Pts',(33.6743371481683,33.125,-33.6743371481684));
#11705=CARTESIAN_POINT('Ctrl Pts',(39.8371685740842,32.9166666666667,-23.));
#11706=CARTESIAN_POINT('Ctrl Pts',(46.,32.7083333333333,-12.3256628518317));
#11707=CARTESIAN_POINT('Ctrl Pts',(46.,32.5,-5.63337527607782E-15));
#11708=CARTESIAN_POINT('Ctrl Pts',(46.,32.2916666666667,12.3256628518316));
#11709=CARTESIAN_POINT('Ctrl Pts',(39.8371685740842,32.0833333333333,23.));
#11710=CARTESIAN_POINT('Ctrl Pts',(33.6743371481684,31.875,33.6743371481683));
#11711=CARTESIAN_POINT('Ctrl Pts',(23.,31.6666666666667,39.8371685740842));
#11712=CARTESIAN_POINT('Ctrl Pts',(12.3256628518317,31.4583333333333,46.));
#11713=CARTESIAN_POINT('Ctrl Pts',(8.45006291411674E-15,31.25,46.));
#11714=CARTESIAN_POINT('Ctrl Pts',(-12.3256628518316,31.0416666666667,46.));
#11715=CARTESIAN_POINT('Ctrl Pts',(-23.,30.8333333333333,39.8371685740842));
#11716=CARTESIAN_POINT('Ctrl Pts',(-33.6743371481683,30.625,33.6743371481684));
#11717=CARTESIAN_POINT('Ctrl Pts',(-39.8371685740842,30.4166666666667,23.));
#11718=CARTESIAN_POINT('Ctrl Pts',(-46.,30.2083333333333,12.3256628518317));
#11719=CARTESIAN_POINT('Ctrl Pts',(-46.,30.,0.));
#11720=CARTESIAN_POINT('',(46.6217457715553,57.,3.60701400320327));
#11721=CARTESIAN_POINT('Ctrl Pts',(48.5725845633798,55.8793483229262,3.60701400320328));
#11722=CARTESIAN_POINT('Ctrl Pts',(48.3407853679392,56.0125314497137,3.60701400320328));
#11723=CARTESIAN_POINT('Ctrl Pts',(48.1089821836664,56.1457076343818,3.60701400320327));
#11724=CARTESIAN_POINT('Ctrl Pts',(47.6453674864979,56.4120455056142,3.60701400320327));
#11725=CARTESIAN_POINT('Ctrl Pts',(47.4135559734254,56.5452071923974,3.60701400320327));
#11726=CARTESIAN_POINT('Ctrl Pts',(47.1817401099609,56.6783613050641,3.60701400320327));
#11727=CARTESIAN_POINT('Ctrl Pts',(46.995078185609,56.7855791741705,3.60701400320327));
#11728=CARTESIAN_POINT('Ctrl Pts',(46.8084134402483,56.8927921321767,3.60701400320327));
#11729=CARTESIAN_POINT('Ctrl Pts',(46.6217457715553,57.,3.60701400320327));
#11730=CARTESIAN_POINT('',(37.183468849883,57.,27.0811677054329));
#11731=CARTESIAN_POINT('Ctrl Pts',(46.6217457715554,57.,3.60701400320327));
#11732=CARTESIAN_POINT('Ctrl Pts',(46.1677264415782,57.,7.85340573112802));
#11733=CARTESIAN_POINT('Ctrl Pts',(45.1307231920318,57.,12.0169900453439));
#11734=CARTESIAN_POINT('Ctrl Pts',(41.9496451502407,57.,19.9424594354284));
#11735=CARTESIAN_POINT('Ctrl Pts',(39.8111418078332,57.,23.691305179069));
#11736=CARTESIAN_POINT('Ctrl Pts',(37.183468849883,57.,27.0811677054329));
#11737=CARTESIAN_POINT('',(3.61292728433799,56.311710737147,45.8578974271399));
#11738=CARTESIAN_POINT('Ctrl Pts',(37.183468849883,57.,27.0811677054329));
#11739=CARTESIAN_POINT('Ctrl Pts',(31.4435637667069,56.8314615162496,34.9622747604562));
#11740=CARTESIAN_POINT('Ctrl Pts',(23.,56.6666666666667,39.8371685740842));
#11741=CARTESIAN_POINT('Ctrl Pts',(13.9875081498766,56.4907679253478,45.0405331698223));
#11742=CARTESIAN_POINT('Ctrl Pts',(3.61292728433799,56.311710737147,45.8578974271399));
#11743=CARTESIAN_POINT('Ctrl Pts',(3.61292728433799,56.311710737147,45.8578974271399));
#11744=CARTESIAN_POINT('Ctrl Pts',(3.612927284338,56.178117727701,46.089460636719));
#11745=CARTESIAN_POINT('Ctrl Pts',(3.61292728433797,55.9109294856547,46.5525857733052));
#11746=CARTESIAN_POINT('Ctrl Pts',(3.61292728433799,55.6437369897944,47.0157084557285));
#11747=CARTESIAN_POINT('Ctrl Pts',(3.61292728433799,55.2553460757965,47.6888965792834));
#11748=CARTESIAN_POINT('Ctrl Pts',(3.612927284338,55.0005487265709,48.1305218136162));
#11749=CARTESIAN_POINT('Ctrl Pts',(3.612927284338,54.7457479656467,48.5721450795008));
#11750=CARTESIAN_POINT('Ctrl Pts',(-48.706329375,58.437500006828,-1.8898197019151E-14));
#11751=CARTESIAN_POINT('Ctrl Pts',(-48.706329375,58.2291666734946,-13.0508216223155));
#11752=CARTESIAN_POINT('Ctrl Pts',(-42.1809185638422,58.0208333401613,-24.3531646875));
#11753=CARTESIAN_POINT('Ctrl Pts',(-35.6555077526845,57.812500006828,-35.6555077526845));
#11754=CARTESIAN_POINT('Ctrl Pts',(-24.3531646875,57.6041666734946,-42.1809185638422));
#11755=CARTESIAN_POINT('Ctrl Pts',(-13.0508216223155,57.3958333401613,-48.706329375));
#11756=CARTESIAN_POINT('Ctrl Pts',(1.59157945007855E-14,57.187500006828,
-48.706329375));
#11757=CARTESIAN_POINT('Ctrl Pts',(13.0508216223155,56.9791666734946,-48.706329375));
#11758=CARTESIAN_POINT('Ctrl Pts',(24.3531646875,56.7708333401613,-42.1809185638422));
#11759=CARTESIAN_POINT('Ctrl Pts',(35.6555077526845,56.562500006828,-35.6555077526845));
#11760=CARTESIAN_POINT('Ctrl Pts',(42.1809185638422,56.3541666734946,-24.3531646875));
#11761=CARTESIAN_POINT('Ctrl Pts',(48.706329375,56.1458333401613,-13.0508216223155));
#11762=CARTESIAN_POINT('Ctrl Pts',(48.706329375,55.937500006828,1.293339198242E-14));
#11763=CARTESIAN_POINT('Ctrl Pts',(48.706329375,55.7291666734946,13.0508216223155));
#11764=CARTESIAN_POINT('Ctrl Pts',(42.1809185638422,55.5208333401613,24.3531646875));
#11765=CARTESIAN_POINT('Ctrl Pts',(35.6555077526845,55.312500006828,35.6555077526845));
#11766=CARTESIAN_POINT('Ctrl Pts',(24.3531646875,55.1041666734946,42.1809185638422));
#11767=CARTESIAN_POINT('Ctrl Pts',(13.0508216223155,54.8958333401613,48.706329375));
#11768=CARTESIAN_POINT('Ctrl Pts',(-9.95098946405443E-15,54.687500006828,
48.706329375));
#11769=CARTESIAN_POINT('Ctrl Pts',(-13.0508216223155,54.4791666734946,48.706329375));
#11770=CARTESIAN_POINT('Ctrl Pts',(-24.3531646875,54.2708333401613,42.1809185638423));
#11771=CARTESIAN_POINT('Ctrl Pts',(-35.6555077526845,54.062500006828,35.6555077526845));
#11772=CARTESIAN_POINT('Ctrl Pts',(-42.1809185638422,53.8541666734946,24.3531646875));
#11773=CARTESIAN_POINT('Ctrl Pts',(-48.706329375,53.6458333401613,13.0508216223155));
#11774=CARTESIAN_POINT('Ctrl Pts',(-48.706329375,53.437500006828,-1.8898197019151E-14));
#11775=CARTESIAN_POINT('Ctrl Pts',(-48.706329375,53.2291666734946,-13.0508216223155));
#11776=CARTESIAN_POINT('Ctrl Pts',(-42.1809185638422,53.0208333401613,-24.3531646875));
#11777=CARTESIAN_POINT('Ctrl Pts',(-35.6555077526845,52.812500006828,-35.6555077526845));
#11778=CARTESIAN_POINT('Ctrl Pts',(-24.3531646875,52.6041666734946,-42.1809185638422));
#11779=CARTESIAN_POINT('Ctrl Pts',(-13.0508216223155,52.3958333401613,-48.706329375));
#11780=CARTESIAN_POINT('Ctrl Pts',(1.59157945007855E-14,52.187500006828,
-48.706329375));
#11781=CARTESIAN_POINT('Ctrl Pts',(13.0508216223155,51.9791666734946,-48.706329375));
#11782=CARTESIAN_POINT('Ctrl Pts',(24.3531646875,51.7708333401613,-42.1809185638422));
#11783=CARTESIAN_POINT('Ctrl Pts',(35.6555077526845,51.562500006828,-35.6555077526845));
#11784=CARTESIAN_POINT('Ctrl Pts',(42.1809185638422,51.3541666734946,-24.3531646875));
#11785=CARTESIAN_POINT('Ctrl Pts',(48.706329375,51.1458333401613,-13.0508216223155));
#11786=CARTESIAN_POINT('Ctrl Pts',(48.706329375,50.937500006828,1.293339198242E-14));
#11787=CARTESIAN_POINT('Ctrl Pts',(48.706329375,50.7291666734946,13.0508216223155));
#11788=CARTESIAN_POINT('Ctrl Pts',(42.1809185638422,50.5208333401613,24.3531646875));
#11789=CARTESIAN_POINT('Ctrl Pts',(35.6555077526845,50.312500006828,35.6555077526845));
#11790=CARTESIAN_POINT('Ctrl Pts',(24.3531646875,50.1041666734946,42.1809185638422));
#11791=CARTESIAN_POINT('Ctrl Pts',(13.0508216223155,49.8958333401613,48.706329375));
#11792=CARTESIAN_POINT('Ctrl Pts',(-9.95098946405443E-15,49.687500006828,
48.706329375));
#11793=CARTESIAN_POINT('Ctrl Pts',(-13.0508216223155,49.4791666734946,48.706329375));
#11794=CARTESIAN_POINT('Ctrl Pts',(-24.3531646875,49.2708333401613,42.1809185638423));
#11795=CARTESIAN_POINT('Ctrl Pts',(-35.6555077526845,49.062500006828,35.6555077526845));
#11796=CARTESIAN_POINT('Ctrl Pts',(-42.1809185638422,48.8541666734946,24.3531646875));
#11797=CARTESIAN_POINT('Ctrl Pts',(-48.706329375,48.6458333401613,13.0508216223155));
#11798=CARTESIAN_POINT('Ctrl Pts',(-48.706329375,48.437500006828,-1.8898197019151E-14));
#11799=CARTESIAN_POINT('Ctrl Pts',(-48.706329375,48.2291666734946,-13.0508216223155));
#11800=CARTESIAN_POINT('Ctrl Pts',(-42.1809185638422,48.0208333401613,-24.3531646875));
#11801=CARTESIAN_POINT('Ctrl Pts',(-35.6555077526845,47.812500006828,-35.6555077526845));
#11802=CARTESIAN_POINT('Ctrl Pts',(-24.3531646875,47.6041666734946,-42.1809185638422));
#11803=CARTESIAN_POINT('Ctrl Pts',(-13.0508216223155,47.3958333401613,-48.706329375));
#11804=CARTESIAN_POINT('Ctrl Pts',(1.59157945007855E-14,47.187500006828,
-48.706329375));
#11805=CARTESIAN_POINT('Ctrl Pts',(13.0508216223155,46.9791666734946,-48.706329375));
#11806=CARTESIAN_POINT('Ctrl Pts',(24.3531646875,46.7708333401613,-42.1809185638422));
#11807=CARTESIAN_POINT('Ctrl Pts',(35.6555077526845,46.562500006828,-35.6555077526845));
#11808=CARTESIAN_POINT('Ctrl Pts',(42.1809185638422,46.3541666734946,-24.3531646875));
#11809=CARTESIAN_POINT('Ctrl Pts',(48.706329375,46.1458333401613,-13.0508216223155));
#11810=CARTESIAN_POINT('Ctrl Pts',(48.706329375,45.937500006828,1.293339198242E-14));
#11811=CARTESIAN_POINT('Ctrl Pts',(48.706329375,45.7291666734946,13.0508216223155));
#11812=CARTESIAN_POINT('Ctrl Pts',(42.1809185638422,45.5208333401613,24.3531646875));
#11813=CARTESIAN_POINT('Ctrl Pts',(35.6555077526845,45.312500006828,35.6555077526845));
#11814=CARTESIAN_POINT('Ctrl Pts',(24.3531646875,45.1041666734946,42.1809185638422));
#11815=CARTESIAN_POINT('Ctrl Pts',(13.0508216223155,44.8958333401613,48.706329375));
#11816=CARTESIAN_POINT('Ctrl Pts',(-9.95098946405443E-15,44.687500006828,
48.706329375));
#11817=CARTESIAN_POINT('Ctrl Pts',(-13.0508216223155,44.4791666734946,48.706329375));
#11818=CARTESIAN_POINT('Ctrl Pts',(-24.3531646875,44.2708333401613,42.1809185638423));
#11819=CARTESIAN_POINT('Ctrl Pts',(-35.6555077526845,44.062500006828,35.6555077526845));
#11820=CARTESIAN_POINT('Ctrl Pts',(-42.1809185638422,43.8541666734946,24.3531646875));
#11821=CARTESIAN_POINT('Ctrl Pts',(-48.706329375,43.6458333401613,13.0508216223155));
#11822=CARTESIAN_POINT('Ctrl Pts',(-48.706329375,43.437500006828,-1.8898197019151E-14));
#11823=CARTESIAN_POINT('Ctrl Pts',(-48.706329375,43.2291666734946,-13.0508216223155));
#11824=CARTESIAN_POINT('Ctrl Pts',(-42.1809185638422,43.0208333401613,-24.3531646875));
#11825=CARTESIAN_POINT('Ctrl Pts',(-35.6555077526845,42.812500006828,-35.6555077526845));
#11826=CARTESIAN_POINT('Ctrl Pts',(-24.3531646875,42.6041666734946,-42.1809185638422));
#11827=CARTESIAN_POINT('Ctrl Pts',(-13.0508216223155,42.3958333401613,-48.706329375));
#11828=CARTESIAN_POINT('Ctrl Pts',(1.59157945007855E-14,42.187500006828,
-48.706329375));
#11829=CARTESIAN_POINT('Ctrl Pts',(13.0508216223155,41.9791666734946,-48.706329375));
#11830=CARTESIAN_POINT('Ctrl Pts',(24.3531646875,41.7708333401613,-42.1809185638422));
#11831=CARTESIAN_POINT('Ctrl Pts',(35.6555077526845,41.562500006828,-35.6555077526845));
#11832=CARTESIAN_POINT('Ctrl Pts',(42.1809185638422,41.3541666734946,-24.3531646875));
#11833=CARTESIAN_POINT('Ctrl Pts',(48.706329375,41.1458333401613,-13.0508216223155));
#11834=CARTESIAN_POINT('Ctrl Pts',(48.706329375,40.937500006828,1.293339198242E-14));
#11835=CARTESIAN_POINT('Ctrl Pts',(48.706329375,40.7291666734946,13.0508216223155));
#11836=CARTESIAN_POINT('Ctrl Pts',(42.1809185638422,40.5208333401613,24.3531646875));
#11837=CARTESIAN_POINT('Ctrl Pts',(35.6555077526845,40.312500006828,35.6555077526845));
#11838=CARTESIAN_POINT('Ctrl Pts',(24.3531646875,40.1041666734946,42.1809185638422));
#11839=CARTESIAN_POINT('Ctrl Pts',(13.0508216223155,39.8958333401613,48.706329375));
#11840=CARTESIAN_POINT('Ctrl Pts',(-9.95098946405443E-15,39.687500006828,
48.706329375));
#11841=CARTESIAN_POINT('Ctrl Pts',(-13.0508216223155,39.4791666734946,48.706329375));
#11842=CARTESIAN_POINT('Ctrl Pts',(-24.3531646875,39.2708333401613,42.1809185638423));
#11843=CARTESIAN_POINT('Ctrl Pts',(-35.6555077526845,39.062500006828,35.6555077526845));
#11844=CARTESIAN_POINT('Ctrl Pts',(-42.1809185638422,38.8541666734946,24.3531646875));
#11845=CARTESIAN_POINT('Ctrl Pts',(-48.706329375,38.6458333401613,13.0508216223155));
#11846=CARTESIAN_POINT('Ctrl Pts',(-48.706329375,38.437500006828,-1.8898197019151E-14));
#11847=CARTESIAN_POINT('Ctrl Pts',(-48.706329375,38.2291666734946,-13.0508216223155));
#11848=CARTESIAN_POINT('Ctrl Pts',(-42.1809185638422,38.0208333401613,-24.3531646875));
#11849=CARTESIAN_POINT('Ctrl Pts',(-35.6555077526845,37.812500006828,-35.6555077526845));
#11850=CARTESIAN_POINT('Ctrl Pts',(-24.3531646875,37.6041666734946,-42.1809185638422));
#11851=CARTESIAN_POINT('Ctrl Pts',(-13.0508216223155,37.3958333401613,-48.706329375));
#11852=CARTESIAN_POINT('Ctrl Pts',(1.59157945007855E-14,37.187500006828,
-48.706329375));
#11853=CARTESIAN_POINT('Ctrl Pts',(13.0508216223155,36.9791666734946,-48.706329375));
#11854=CARTESIAN_POINT('Ctrl Pts',(24.3531646875,36.7708333401613,-42.1809185638422));
#11855=CARTESIAN_POINT('Ctrl Pts',(35.6555077526845,36.562500006828,-35.6555077526845));
#11856=CARTESIAN_POINT('Ctrl Pts',(42.1809185638422,36.3541666734946,-24.3531646875));
#11857=CARTESIAN_POINT('Ctrl Pts',(48.706329375,36.1458333401613,-13.0508216223155));
#11858=CARTESIAN_POINT('Ctrl Pts',(48.706329375,35.937500006828,1.293339198242E-14));
#11859=CARTESIAN_POINT('Ctrl Pts',(48.706329375,35.7291666734946,13.0508216223155));
#11860=CARTESIAN_POINT('Ctrl Pts',(42.1809185638422,35.5208333401613,24.3531646875));
#11861=CARTESIAN_POINT('Ctrl Pts',(35.6555077526845,35.312500006828,35.6555077526845));
#11862=CARTESIAN_POINT('Ctrl Pts',(24.3531646875,35.1041666734946,42.1809185638422));
#11863=CARTESIAN_POINT('Ctrl Pts',(13.0508216223155,34.8958333401613,48.706329375));
#11864=CARTESIAN_POINT('Ctrl Pts',(-9.95098946405443E-15,34.687500006828,
48.706329375));
#11865=CARTESIAN_POINT('Ctrl Pts',(-13.0508216223155,34.4791666734946,48.706329375));
#11866=CARTESIAN_POINT('Ctrl Pts',(-24.3531646875,34.2708333401613,42.1809185638423));
#11867=CARTESIAN_POINT('Ctrl Pts',(-35.6555077526845,34.062500006828,35.6555077526845));
#11868=CARTESIAN_POINT('Ctrl Pts',(-42.1809185638422,33.8541666734946,24.3531646875));
#11869=CARTESIAN_POINT('Ctrl Pts',(-48.706329375,33.6458333401613,13.0508216223155));
#11870=CARTESIAN_POINT('Ctrl Pts',(-48.706329375,33.437500006828,-1.8898197019151E-14));
#11871=CARTESIAN_POINT('Ctrl Pts',(-48.706329375,33.2291666734946,-13.0508216223155));
#11872=CARTESIAN_POINT('Ctrl Pts',(-42.1809185638422,33.0208333401613,-24.3531646875));
#11873=CARTESIAN_POINT('Ctrl Pts',(-35.6555077526845,32.812500006828,-35.6555077526845));
#11874=CARTESIAN_POINT('Ctrl Pts',(-24.3531646875,32.6041666734946,-42.1809185638422));
#11875=CARTESIAN_POINT('Ctrl Pts',(-13.0508216223155,32.3958333401613,-48.706329375));
#11876=CARTESIAN_POINT('Ctrl Pts',(1.59157945007855E-14,32.187500006828,
-48.706329375));
#11877=CARTESIAN_POINT('Ctrl Pts',(13.0508216223155,31.9791666734946,-48.706329375));
#11878=CARTESIAN_POINT('Ctrl Pts',(24.3531646875,31.7708333401613,-42.1809185638422));
#11879=CARTESIAN_POINT('Ctrl Pts',(35.6555077526845,31.562500006828,-35.6555077526845));
#11880=CARTESIAN_POINT('Ctrl Pts',(42.1809185638422,31.3541666734946,-24.3531646875));
#11881=CARTESIAN_POINT('Ctrl Pts',(48.706329375,31.1458333401613,-13.0508216223155));
#11882=CARTESIAN_POINT('Ctrl Pts',(48.706329375,30.937500006828,1.293339198242E-14));
#11883=CARTESIAN_POINT('Ctrl Pts',(48.706329375,30.7291666734946,13.0508216223155));
#11884=CARTESIAN_POINT('Ctrl Pts',(42.1809185638422,30.5208333401613,24.3531646875));
#11885=CARTESIAN_POINT('Ctrl Pts',(35.6555077526845,30.312500006828,35.6555077526845));
#11886=CARTESIAN_POINT('Ctrl Pts',(24.3531646875,30.1041666734946,42.1809185638422));
#11887=CARTESIAN_POINT('Ctrl Pts',(13.0508216223155,29.8958333401613,48.706329375));
#11888=CARTESIAN_POINT('Ctrl Pts',(-9.95098946405443E-15,29.687500006828,
48.706329375));
#11889=CARTESIAN_POINT('Ctrl Pts',(-13.0508216223155,29.4791666734946,48.706329375));
#11890=CARTESIAN_POINT('Ctrl Pts',(-24.3531646875,29.2708333401613,42.1809185638423));
#11891=CARTESIAN_POINT('Ctrl Pts',(-35.6555077526845,29.062500006828,35.6555077526845));
#11892=CARTESIAN_POINT('Ctrl Pts',(-42.1809185638422,28.8541666734946,24.3531646875));
#11893=CARTESIAN_POINT('Ctrl Pts',(-48.706329375,28.6458333401613,13.0508216223155));
#11894=CARTESIAN_POINT('Ctrl Pts',(-48.706329375,28.437500006828,-1.8898197019151E-14));
#11895=CARTESIAN_POINT('Ctrl Pts',(-46.,60.,0.));
#11896=CARTESIAN_POINT('Ctrl Pts',(-46.,59.7916666666667,-12.3256628518316));
#11897=CARTESIAN_POINT('Ctrl Pts',(-39.8371685740842,59.5833333333333,-23.));
#11898=CARTESIAN_POINT('Ctrl Pts',(-33.6743371481684,59.375,-33.6743371481684));
#11899=CARTESIAN_POINT('Ctrl Pts',(-23.,59.1666666666667,-39.8371685740842));
#11900=CARTESIAN_POINT('Ctrl Pts',(-12.3256628518317,58.9583333333333,-46.));
#11901=CARTESIAN_POINT('Ctrl Pts',(-2.81668763803891E-15,58.75,-46.));
#11902=CARTESIAN_POINT('Ctrl Pts',(12.3256628518316,58.5416666666667,-46.));
#11903=CARTESIAN_POINT('Ctrl Pts',(23.,58.3333333333333,-39.8371685740842));
#11904=CARTESIAN_POINT('Ctrl Pts',(33.6743371481683,58.125,-33.6743371481684));
#11905=CARTESIAN_POINT('Ctrl Pts',(39.8371685740842,57.9166666666667,-23.));
#11906=CARTESIAN_POINT('Ctrl Pts',(46.,57.7083333333333,-12.3256628518317));
#11907=CARTESIAN_POINT('Ctrl Pts',(46.,57.5,-5.63337527607782E-15));
#11908=CARTESIAN_POINT('Ctrl Pts',(46.,57.2916666666667,12.3256628518316));
#11909=CARTESIAN_POINT('Ctrl Pts',(39.8371685740842,57.0833333333333,23.));
#11910=CARTESIAN_POINT('Ctrl Pts',(33.6743371481684,56.875,33.6743371481683));
#11911=CARTESIAN_POINT('Ctrl Pts',(23.,56.6666666666667,39.8371685740842));
#11912=CARTESIAN_POINT('Ctrl Pts',(12.3256628518317,56.4583333333333,46.));
#11913=CARTESIAN_POINT('Ctrl Pts',(8.45006291411674E-15,56.25,46.));
#11914=CARTESIAN_POINT('Ctrl Pts',(-12.3256628518316,56.0416666666667,46.));
#11915=CARTESIAN_POINT('Ctrl Pts',(-23.,55.8333333333333,39.8371685740842));
#11916=CARTESIAN_POINT('Ctrl Pts',(-33.6743371481683,55.625,33.6743371481684));
#11917=CARTESIAN_POINT('Ctrl Pts',(-39.8371685740842,55.4166666666667,23.));
#11918=CARTESIAN_POINT('Ctrl Pts',(-46.,55.2083333333333,12.3256628518317));
#11919=CARTESIAN_POINT('Ctrl Pts',(-46.,55.,0.));
#11920=CARTESIAN_POINT('Ctrl Pts',(-46.,54.7916666666667,-12.3256628518316));
#11921=CARTESIAN_POINT('Ctrl Pts',(-39.8371685740842,54.5833333333333,-23.));
#11922=CARTESIAN_POINT('Ctrl Pts',(-33.6743371481684,54.375,-33.6743371481684));
#11923=CARTESIAN_POINT('Ctrl Pts',(-23.,54.1666666666667,-39.8371685740842));
#11924=CARTESIAN_POINT('Ctrl Pts',(-12.3256628518317,53.9583333333333,-46.));
#11925=CARTESIAN_POINT('Ctrl Pts',(-2.81668763803891E-15,53.75,-46.));
#11926=CARTESIAN_POINT('Ctrl Pts',(12.3256628518316,53.5416666666667,-46.));
#11927=CARTESIAN_POINT('Ctrl Pts',(23.,53.3333333333333,-39.8371685740842));
#11928=CARTESIAN_POINT('Ctrl Pts',(33.6743371481683,53.125,-33.6743371481684));
#11929=CARTESIAN_POINT('Ctrl Pts',(39.8371685740842,52.9166666666667,-23.));
#11930=CARTESIAN_POINT('Ctrl Pts',(46.,52.7083333333333,-12.3256628518317));
#11931=CARTESIAN_POINT('Ctrl Pts',(46.,52.5,-5.63337527607782E-15));
#11932=CARTESIAN_POINT('Ctrl Pts',(46.,52.2916666666667,12.3256628518316));
#11933=CARTESIAN_POINT('Ctrl Pts',(39.8371685740842,52.0833333333333,23.));
#11934=CARTESIAN_POINT('Ctrl Pts',(33.6743371481684,51.875,33.6743371481683));
#11935=CARTESIAN_POINT('Ctrl Pts',(23.,51.6666666666667,39.8371685740842));
#11936=CARTESIAN_POINT('Ctrl Pts',(12.3256628518317,51.4583333333333,46.));
#11937=CARTESIAN_POINT('Ctrl Pts',(8.45006291411674E-15,51.25,46.));
#11938=CARTESIAN_POINT('Ctrl Pts',(-12.3256628518316,51.0416666666667,46.));
#11939=CARTESIAN_POINT('Ctrl Pts',(-23.,50.8333333333333,39.8371685740842));
#11940=CARTESIAN_POINT('Ctrl Pts',(-33.6743371481683,50.625,33.6743371481684));
#11941=CARTESIAN_POINT('Ctrl Pts',(-39.8371685740842,50.4166666666667,23.));
#11942=CARTESIAN_POINT('Ctrl Pts',(-46.,50.2083333333333,12.3256628518317));
#11943=CARTESIAN_POINT('Ctrl Pts',(-46.,50.,0.));
#11944=CARTESIAN_POINT('Ctrl Pts',(-46.,49.7916666666667,-12.3256628518316));
#11945=CARTESIAN_POINT('Ctrl Pts',(-39.8371685740842,49.5833333333333,-23.));
#11946=CARTESIAN_POINT('Ctrl Pts',(-33.6743371481684,49.375,-33.6743371481684));
#11947=CARTESIAN_POINT('Ctrl Pts',(-23.,49.1666666666667,-39.8371685740842));
#11948=CARTESIAN_POINT('Ctrl Pts',(-12.3256628518317,48.9583333333333,-46.));
#11949=CARTESIAN_POINT('Ctrl Pts',(-2.81668763803891E-15,48.75,-46.));
#11950=CARTESIAN_POINT('Ctrl Pts',(12.3256628518316,48.5416666666667,-46.));
#11951=CARTESIAN_POINT('Ctrl Pts',(23.,48.3333333333333,-39.8371685740842));
#11952=CARTESIAN_POINT('Ctrl Pts',(33.6743371481683,48.125,-33.6743371481684));
#11953=CARTESIAN_POINT('Ctrl Pts',(39.8371685740842,47.9166666666667,-23.));
#11954=CARTESIAN_POINT('Ctrl Pts',(46.,47.7083333333333,-12.3256628518317));
#11955=CARTESIAN_POINT('Ctrl Pts',(46.,47.5,-5.63337527607782E-15));
#11956=CARTESIAN_POINT('Ctrl Pts',(46.,47.2916666666667,12.3256628518316));
#11957=CARTESIAN_POINT('Ctrl Pts',(39.8371685740842,47.0833333333333,23.));
#11958=CARTESIAN_POINT('Ctrl Pts',(33.6743371481684,46.875,33.6743371481683));
#11959=CARTESIAN_POINT('Ctrl Pts',(23.,46.6666666666667,39.8371685740842));
#11960=CARTESIAN_POINT('Ctrl Pts',(12.3256628518317,46.4583333333333,46.));
#11961=CARTESIAN_POINT('Ctrl Pts',(8.45006291411674E-15,46.25,46.));
#11962=CARTESIAN_POINT('Ctrl Pts',(-12.3256628518316,46.0416666666667,46.));
#11963=CARTESIAN_POINT('Ctrl Pts',(-23.,45.8333333333333,39.8371685740842));
#11964=CARTESIAN_POINT('Ctrl Pts',(-33.6743371481683,45.625,33.6743371481684));
#11965=CARTESIAN_POINT('Ctrl Pts',(-39.8371685740842,45.4166666666667,23.));
#11966=CARTESIAN_POINT('Ctrl Pts',(-46.,45.2083333333333,12.3256628518317));
#11967=CARTESIAN_POINT('Ctrl Pts',(-46.,45.,0.));
#11968=CARTESIAN_POINT('Ctrl Pts',(-46.,44.7916666666667,-12.3256628518316));
#11969=CARTESIAN_POINT('Ctrl Pts',(-39.8371685740842,44.5833333333333,-23.));
#11970=CARTESIAN_POINT('Ctrl Pts',(-33.6743371481684,44.375,-33.6743371481684));
#11971=CARTESIAN_POINT('Ctrl Pts',(-23.,44.1666666666667,-39.8371685740842));
#11972=CARTESIAN_POINT('Ctrl Pts',(-12.3256628518317,43.9583333333333,-46.));
#11973=CARTESIAN_POINT('Ctrl Pts',(-2.81668763803891E-15,43.75,-46.));
#11974=CARTESIAN_POINT('Ctrl Pts',(12.3256628518316,43.5416666666667,-46.));
#11975=CARTESIAN_POINT('Ctrl Pts',(23.,43.3333333333333,-39.8371685740842));
#11976=CARTESIAN_POINT('Ctrl Pts',(33.6743371481683,43.125,-33.6743371481684));
#11977=CARTESIAN_POINT('Ctrl Pts',(39.8371685740842,42.9166666666667,-23.));
#11978=CARTESIAN_POINT('Ctrl Pts',(46.,42.7083333333333,-12.3256628518317));
#11979=CARTESIAN_POINT('Ctrl Pts',(46.,42.5,-5.63337527607782E-15));
#11980=CARTESIAN_POINT('Ctrl Pts',(46.,42.2916666666667,12.3256628518316));
#11981=CARTESIAN_POINT('Ctrl Pts',(39.8371685740842,42.0833333333333,23.));
#11982=CARTESIAN_POINT('Ctrl Pts',(33.6743371481684,41.875,33.6743371481683));
#11983=CARTESIAN_POINT('Ctrl Pts',(23.,41.6666666666667,39.8371685740842));
#11984=CARTESIAN_POINT('Ctrl Pts',(12.3256628518317,41.4583333333333,46.));
#11985=CARTESIAN_POINT('Ctrl Pts',(8.45006291411674E-15,41.25,46.));
#11986=CARTESIAN_POINT('Ctrl Pts',(-12.3256628518316,41.0416666666667,46.));
#11987=CARTESIAN_POINT('Ctrl Pts',(-23.,40.8333333333333,39.8371685740842));
#11988=CARTESIAN_POINT('Ctrl Pts',(-33.6743371481683,40.625,33.6743371481684));
#11989=CARTESIAN_POINT('Ctrl Pts',(-39.8371685740842,40.4166666666667,23.));
#11990=CARTESIAN_POINT('Ctrl Pts',(-46.,40.2083333333333,12.3256628518317));
#11991=CARTESIAN_POINT('Ctrl Pts',(-46.,40.,0.));
#11992=CARTESIAN_POINT('Ctrl Pts',(-46.,39.7916666666667,-12.3256628518316));
#11993=CARTESIAN_POINT('Ctrl Pts',(-39.8371685740842,39.5833333333333,-23.));
#11994=CARTESIAN_POINT('Ctrl Pts',(-33.6743371481684,39.375,-33.6743371481684));
#11995=CARTESIAN_POINT('Ctrl Pts',(-23.,39.1666666666667,-39.8371685740842));
#11996=CARTESIAN_POINT('Ctrl Pts',(-12.3256628518317,38.9583333333333,-46.));
#11997=CARTESIAN_POINT('Ctrl Pts',(-2.81668763803891E-15,38.75,-46.));
#11998=CARTESIAN_POINT('Ctrl Pts',(12.3256628518316,38.5416666666667,-46.));
#11999=CARTESIAN_POINT('Ctrl Pts',(23.,38.3333333333333,-39.8371685740842));
#12000=CARTESIAN_POINT('Ctrl Pts',(33.6743371481683,38.125,-33.6743371481684));
#12001=CARTESIAN_POINT('Ctrl Pts',(39.8371685740842,37.9166666666667,-23.));
#12002=CARTESIAN_POINT('Ctrl Pts',(46.,37.7083333333333,-12.3256628518317));
#12003=CARTESIAN_POINT('Ctrl Pts',(46.,37.5,-5.63337527607782E-15));
#12004=CARTESIAN_POINT('Ctrl Pts',(46.,37.2916666666667,12.3256628518316));
#12005=CARTESIAN_POINT('Ctrl Pts',(39.8371685740842,37.0833333333333,23.));
#12006=CARTESIAN_POINT('Ctrl Pts',(33.6743371481684,36.875,33.6743371481683));
#12007=CARTESIAN_POINT('Ctrl Pts',(23.,36.6666666666667,39.8371685740842));
#12008=CARTESIAN_POINT('Ctrl Pts',(12.3256628518317,36.4583333333333,46.));
#12009=CARTESIAN_POINT('Ctrl Pts',(8.45006291411674E-15,36.25,46.));
#12010=CARTESIAN_POINT('Ctrl Pts',(-12.3256628518316,36.0416666666667,46.));
#12011=CARTESIAN_POINT('Ctrl Pts',(-23.,35.8333333333333,39.8371685740842));
#12012=CARTESIAN_POINT('Ctrl Pts',(-33.6743371481683,35.625,33.6743371481684));
#12013=CARTESIAN_POINT('Ctrl Pts',(-39.8371685740842,35.4166666666667,23.));
#12014=CARTESIAN_POINT('Ctrl Pts',(-46.,35.2083333333333,12.3256628518317));
#12015=CARTESIAN_POINT('Ctrl Pts',(-46.,35.,0.));
#12016=CARTESIAN_POINT('Ctrl Pts',(-46.,34.7916666666667,-12.3256628518316));
#12017=CARTESIAN_POINT('Ctrl Pts',(-39.8371685740842,34.5833333333333,-23.));
#12018=CARTESIAN_POINT('Ctrl Pts',(-33.6743371481684,34.375,-33.6743371481684));
#12019=CARTESIAN_POINT('Ctrl Pts',(-23.,34.1666666666667,-39.8371685740842));
#12020=CARTESIAN_POINT('Ctrl Pts',(-12.3256628518317,33.9583333333333,-46.));
#12021=CARTESIAN_POINT('Ctrl Pts',(-2.81668763803891E-15,33.75,-46.));
#12022=CARTESIAN_POINT('Ctrl Pts',(12.3256628518316,33.5416666666667,-46.));
#12023=CARTESIAN_POINT('Ctrl Pts',(23.,33.3333333333333,-39.8371685740842));
#12024=CARTESIAN_POINT('Ctrl Pts',(33.6743371481683,33.125,-33.6743371481684));
#12025=CARTESIAN_POINT('Ctrl Pts',(39.8371685740842,32.9166666666667,-23.));
#12026=CARTESIAN_POINT('Ctrl Pts',(46.,32.7083333333333,-12.3256628518317));
#12027=CARTESIAN_POINT('Ctrl Pts',(46.,32.5,-5.63337527607782E-15));
#12028=CARTESIAN_POINT('Ctrl Pts',(46.,32.2916666666667,12.3256628518316));
#12029=CARTESIAN_POINT('Ctrl Pts',(39.8371685740842,32.0833333333333,23.));
#12030=CARTESIAN_POINT('Ctrl Pts',(33.6743371481684,31.875,33.6743371481683));
#12031=CARTESIAN_POINT('Ctrl Pts',(23.,31.6666666666667,39.8371685740842));
#12032=CARTESIAN_POINT('Ctrl Pts',(12.3256628518317,31.4583333333333,46.));
#12033=CARTESIAN_POINT('Ctrl Pts',(8.45006291411674E-15,31.25,46.));
#12034=CARTESIAN_POINT('Ctrl Pts',(-12.3256628518316,31.0416666666667,46.));
#12035=CARTESIAN_POINT('Ctrl Pts',(-23.,30.8333333333333,39.8371685740842));
#12036=CARTESIAN_POINT('Ctrl Pts',(-33.6743371481683,30.625,33.6743371481684));
#12037=CARTESIAN_POINT('Ctrl Pts',(-39.8371685740842,30.4166666666667,23.));
#12038=CARTESIAN_POINT('Ctrl Pts',(-46.,30.2083333333333,12.3256628518317));
#12039=CARTESIAN_POINT('Ctrl Pts',(-46.,30.,0.));
#12040=CARTESIAN_POINT('Ctrl Pts',(45.7957082162897,52.5741208584476,-4.33048599679672));
#12041=CARTESIAN_POINT('Ctrl Pts',(46.027322302781,52.4406160752063,-4.33048599679672));
#12042=CARTESIAN_POINT('Ctrl Pts',(46.4905476657728,52.1736016336912,-4.33048599679677));
#12043=CARTESIAN_POINT('Ctrl Pts',(46.9537676533565,51.9065778670208,-4.33048599679672));
#12044=CARTESIAN_POINT('Ctrl Pts',(47.6280672732221,51.5178683162597,-4.33048599679672));
#12045=CARTESIAN_POINT('Ctrl Pts',(48.0707534890442,51.2626647328764,-4.33048599679671));
#12046=CARTESIAN_POINT('Ctrl Pts',(48.5134353784344,51.0074536451604,-4.33048599679671));
#12047=CARTESIAN_POINT('Ctrl Pts',(3.612927284338,52.1292520480092,-48.5721450795008));
#12048=CARTESIAN_POINT('Ctrl Pts',(3.612927284338,52.2624339185675,-48.3403451622817));
#12049=CARTESIAN_POINT('Ctrl Pts',(3.61292728433801,52.395608829009,-48.1085412459393));
#12050=CARTESIAN_POINT('Ctrl Pts',(3.61292728433801,52.6619441142016,-47.6449250631479));
#12051=CARTESIAN_POINT('Ctrl Pts',(3.612927284338,52.7951044891727,-47.4131127965212));
#12052=CARTESIAN_POINT('Ctrl Pts',(3.612927284338,52.9282572703913,-47.1812961682826));
#12053=CARTESIAN_POINT('Ctrl Pts',(3.612927284338,53.1816295626638,-46.7401795055578));
#12054=CARTESIAN_POINT('Ctrl Pts',(3.61292728433801,53.4349743764897,-46.2990470581854));
#12055=CARTESIAN_POINT('Ctrl Pts',(3.61292728433801,53.688289262853,-45.8578974271399));
#12056=CARTESIAN_POINT('Ctrl Pts',(-48.706329375,58.437500006828,-1.8898197019151E-14));
#12057=CARTESIAN_POINT('Ctrl Pts',(-48.706329375,58.2291666734946,-13.0508216223155));
#12058=CARTESIAN_POINT('Ctrl Pts',(-42.1809185638422,58.0208333401613,-24.3531646875));
#12059=CARTESIAN_POINT('Ctrl Pts',(-35.6555077526845,57.812500006828,-35.6555077526845));
#12060=CARTESIAN_POINT('Ctrl Pts',(-24.3531646875,57.6041666734946,-42.1809185638422));
#12061=CARTESIAN_POINT('Ctrl Pts',(-13.0508216223155,57.3958333401613,-48.706329375));
#12062=CARTESIAN_POINT('Ctrl Pts',(1.59157945007855E-14,57.187500006828,
-48.706329375));
#12063=CARTESIAN_POINT('Ctrl Pts',(13.0508216223155,56.9791666734946,-48.706329375));
#12064=CARTESIAN_POINT('Ctrl Pts',(24.3531646875,56.7708333401613,-42.1809185638422));
#12065=CARTESIAN_POINT('Ctrl Pts',(35.6555077526845,56.562500006828,-35.6555077526845));
#12066=CARTESIAN_POINT('Ctrl Pts',(42.1809185638422,56.3541666734946,-24.3531646875));
#12067=CARTESIAN_POINT('Ctrl Pts',(48.706329375,56.1458333401613,-13.0508216223155));
#12068=CARTESIAN_POINT('Ctrl Pts',(48.706329375,55.937500006828,1.293339198242E-14));
#12069=CARTESIAN_POINT('Ctrl Pts',(48.706329375,55.7291666734946,13.0508216223155));
#12070=CARTESIAN_POINT('Ctrl Pts',(42.1809185638422,55.5208333401613,24.3531646875));
#12071=CARTESIAN_POINT('Ctrl Pts',(35.6555077526845,55.312500006828,35.6555077526845));
#12072=CARTESIAN_POINT('Ctrl Pts',(24.3531646875,55.1041666734946,42.1809185638422));
#12073=CARTESIAN_POINT('Ctrl Pts',(13.0508216223155,54.8958333401613,48.706329375));
#12074=CARTESIAN_POINT('Ctrl Pts',(-9.95098946405443E-15,54.687500006828,
48.706329375));
#12075=CARTESIAN_POINT('Ctrl Pts',(-13.0508216223155,54.4791666734946,48.706329375));
#12076=CARTESIAN_POINT('Ctrl Pts',(-24.3531646875,54.2708333401613,42.1809185638423));
#12077=CARTESIAN_POINT('Ctrl Pts',(-35.6555077526845,54.062500006828,35.6555077526845));
#12078=CARTESIAN_POINT('Ctrl Pts',(-42.1809185638422,53.8541666734946,24.3531646875));
#12079=CARTESIAN_POINT('Ctrl Pts',(-48.706329375,53.6458333401613,13.0508216223155));
#12080=CARTESIAN_POINT('Ctrl Pts',(-48.706329375,53.437500006828,-1.8898197019151E-14));
#12081=CARTESIAN_POINT('Ctrl Pts',(-48.706329375,53.2291666734946,-13.0508216223155));
#12082=CARTESIAN_POINT('Ctrl Pts',(-42.1809185638422,53.0208333401613,-24.3531646875));
#12083=CARTESIAN_POINT('Ctrl Pts',(-35.6555077526845,52.812500006828,-35.6555077526845));
#12084=CARTESIAN_POINT('Ctrl Pts',(-24.3531646875,52.6041666734946,-42.1809185638422));
#12085=CARTESIAN_POINT('Ctrl Pts',(-13.0508216223155,52.3958333401613,-48.706329375));
#12086=CARTESIAN_POINT('Ctrl Pts',(1.59157945007855E-14,52.187500006828,
-48.706329375));
#12087=CARTESIAN_POINT('Ctrl Pts',(13.0508216223155,51.9791666734946,-48.706329375));
#12088=CARTESIAN_POINT('Ctrl Pts',(24.3531646875,51.7708333401613,-42.1809185638422));
#12089=CARTESIAN_POINT('Ctrl Pts',(35.6555077526845,51.562500006828,-35.6555077526845));
#12090=CARTESIAN_POINT('Ctrl Pts',(42.1809185638422,51.3541666734946,-24.3531646875));
#12091=CARTESIAN_POINT('Ctrl Pts',(48.706329375,51.1458333401613,-13.0508216223155));
#12092=CARTESIAN_POINT('Ctrl Pts',(48.706329375,50.937500006828,1.293339198242E-14));
#12093=CARTESIAN_POINT('Ctrl Pts',(48.706329375,50.7291666734946,13.0508216223155));
#12094=CARTESIAN_POINT('Ctrl Pts',(42.1809185638422,50.5208333401613,24.3531646875));
#12095=CARTESIAN_POINT('Ctrl Pts',(35.6555077526845,50.312500006828,35.6555077526845));
#12096=CARTESIAN_POINT('Ctrl Pts',(24.3531646875,50.1041666734946,42.1809185638422));
#12097=CARTESIAN_POINT('Ctrl Pts',(13.0508216223155,49.8958333401613,48.706329375));
#12098=CARTESIAN_POINT('Ctrl Pts',(-9.95098946405443E-15,49.687500006828,
48.706329375));
#12099=CARTESIAN_POINT('Ctrl Pts',(-13.0508216223155,49.4791666734946,48.706329375));
#12100=CARTESIAN_POINT('Ctrl Pts',(-24.3531646875,49.2708333401613,42.1809185638423));
#12101=CARTESIAN_POINT('Ctrl Pts',(-35.6555077526845,49.062500006828,35.6555077526845));
#12102=CARTESIAN_POINT('Ctrl Pts',(-42.1809185638422,48.8541666734946,24.3531646875));
#12103=CARTESIAN_POINT('Ctrl Pts',(-48.706329375,48.6458333401613,13.0508216223155));
#12104=CARTESIAN_POINT('Ctrl Pts',(-48.706329375,48.437500006828,-1.8898197019151E-14));
#12105=CARTESIAN_POINT('Ctrl Pts',(-48.706329375,48.2291666734946,-13.0508216223155));
#12106=CARTESIAN_POINT('Ctrl Pts',(-42.1809185638422,48.0208333401613,-24.3531646875));
#12107=CARTESIAN_POINT('Ctrl Pts',(-35.6555077526845,47.812500006828,-35.6555077526845));
#12108=CARTESIAN_POINT('Ctrl Pts',(-24.3531646875,47.6041666734946,-42.1809185638422));
#12109=CARTESIAN_POINT('Ctrl Pts',(-13.0508216223155,47.3958333401613,-48.706329375));
#12110=CARTESIAN_POINT('Ctrl Pts',(1.59157945007855E-14,47.187500006828,
-48.706329375));
#12111=CARTESIAN_POINT('Ctrl Pts',(13.0508216223155,46.9791666734946,-48.706329375));
#12112=CARTESIAN_POINT('Ctrl Pts',(24.3531646875,46.7708333401613,-42.1809185638422));
#12113=CARTESIAN_POINT('Ctrl Pts',(35.6555077526845,46.562500006828,-35.6555077526845));
#12114=CARTESIAN_POINT('Ctrl Pts',(42.1809185638422,46.3541666734946,-24.3531646875));
#12115=CARTESIAN_POINT('Ctrl Pts',(48.706329375,46.1458333401613,-13.0508216223155));
#12116=CARTESIAN_POINT('Ctrl Pts',(48.706329375,45.937500006828,1.293339198242E-14));
#12117=CARTESIAN_POINT('Ctrl Pts',(48.706329375,45.7291666734946,13.0508216223155));
#12118=CARTESIAN_POINT('Ctrl Pts',(42.1809185638422,45.5208333401613,24.3531646875));
#12119=CARTESIAN_POINT('Ctrl Pts',(35.6555077526845,45.312500006828,35.6555077526845));
#12120=CARTESIAN_POINT('Ctrl Pts',(24.3531646875,45.1041666734946,42.1809185638422));
#12121=CARTESIAN_POINT('Ctrl Pts',(13.0508216223155,44.8958333401613,48.706329375));
#12122=CARTESIAN_POINT('Ctrl Pts',(-9.95098946405443E-15,44.687500006828,
48.706329375));
#12123=CARTESIAN_POINT('Ctrl Pts',(-13.0508216223155,44.4791666734946,48.706329375));
#12124=CARTESIAN_POINT('Ctrl Pts',(-24.3531646875,44.2708333401613,42.1809185638423));
#12125=CARTESIAN_POINT('Ctrl Pts',(-35.6555077526845,44.062500006828,35.6555077526845));
#12126=CARTESIAN_POINT('Ctrl Pts',(-42.1809185638422,43.8541666734946,24.3531646875));
#12127=CARTESIAN_POINT('Ctrl Pts',(-48.706329375,43.6458333401613,13.0508216223155));
#12128=CARTESIAN_POINT('Ctrl Pts',(-48.706329375,43.437500006828,-1.8898197019151E-14));
#12129=CARTESIAN_POINT('Ctrl Pts',(-48.706329375,43.2291666734946,-13.0508216223155));
#12130=CARTESIAN_POINT('Ctrl Pts',(-42.1809185638422,43.0208333401613,-24.3531646875));
#12131=CARTESIAN_POINT('Ctrl Pts',(-35.6555077526845,42.812500006828,-35.6555077526845));
#12132=CARTESIAN_POINT('Ctrl Pts',(-24.3531646875,42.6041666734946,-42.1809185638422));
#12133=CARTESIAN_POINT('Ctrl Pts',(-13.0508216223155,42.3958333401613,-48.706329375));
#12134=CARTESIAN_POINT('Ctrl Pts',(1.59157945007855E-14,42.187500006828,
-48.706329375));
#12135=CARTESIAN_POINT('Ctrl Pts',(13.0508216223155,41.9791666734946,-48.706329375));
#12136=CARTESIAN_POINT('Ctrl Pts',(24.3531646875,41.7708333401613,-42.1809185638422));
#12137=CARTESIAN_POINT('Ctrl Pts',(35.6555077526845,41.562500006828,-35.6555077526845));
#12138=CARTESIAN_POINT('Ctrl Pts',(42.1809185638422,41.3541666734946,-24.3531646875));
#12139=CARTESIAN_POINT('Ctrl Pts',(48.706329375,41.1458333401613,-13.0508216223155));
#12140=CARTESIAN_POINT('Ctrl Pts',(48.706329375,40.937500006828,1.293339198242E-14));
#12141=CARTESIAN_POINT('Ctrl Pts',(48.706329375,40.7291666734946,13.0508216223155));
#12142=CARTESIAN_POINT('Ctrl Pts',(42.1809185638422,40.5208333401613,24.3531646875));
#12143=CARTESIAN_POINT('Ctrl Pts',(35.6555077526845,40.312500006828,35.6555077526845));
#12144=CARTESIAN_POINT('Ctrl Pts',(24.3531646875,40.1041666734946,42.1809185638422));
#12145=CARTESIAN_POINT('Ctrl Pts',(13.0508216223155,39.8958333401613,48.706329375));
#12146=CARTESIAN_POINT('Ctrl Pts',(-9.95098946405443E-15,39.687500006828,
48.706329375));
#12147=CARTESIAN_POINT('Ctrl Pts',(-13.0508216223155,39.4791666734946,48.706329375));
#12148=CARTESIAN_POINT('Ctrl Pts',(-24.3531646875,39.2708333401613,42.1809185638423));
#12149=CARTESIAN_POINT('Ctrl Pts',(-35.6555077526845,39.062500006828,35.6555077526845));
#12150=CARTESIAN_POINT('Ctrl Pts',(-42.1809185638422,38.8541666734946,24.3531646875));
#12151=CARTESIAN_POINT('Ctrl Pts',(-48.706329375,38.6458333401613,13.0508216223155));
#12152=CARTESIAN_POINT('Ctrl Pts',(-48.706329375,38.437500006828,-1.8898197019151E-14));
#12153=CARTESIAN_POINT('Ctrl Pts',(-48.706329375,38.2291666734946,-13.0508216223155));
#12154=CARTESIAN_POINT('Ctrl Pts',(-42.1809185638422,38.0208333401613,-24.3531646875));
#12155=CARTESIAN_POINT('Ctrl Pts',(-35.6555077526845,37.812500006828,-35.6555077526845));
#12156=CARTESIAN_POINT('Ctrl Pts',(-24.3531646875,37.6041666734946,-42.1809185638422));
#12157=CARTESIAN_POINT('Ctrl Pts',(-13.0508216223155,37.3958333401613,-48.706329375));
#12158=CARTESIAN_POINT('Ctrl Pts',(1.59157945007855E-14,37.187500006828,
-48.706329375));
#12159=CARTESIAN_POINT('Ctrl Pts',(13.0508216223155,36.9791666734946,-48.706329375));
#12160=CARTESIAN_POINT('Ctrl Pts',(24.3531646875,36.7708333401613,-42.1809185638422));
#12161=CARTESIAN_POINT('Ctrl Pts',(35.6555077526845,36.562500006828,-35.6555077526845));
#12162=CARTESIAN_POINT('Ctrl Pts',(42.1809185638422,36.3541666734946,-24.3531646875));
#12163=CARTESIAN_POINT('Ctrl Pts',(48.706329375,36.1458333401613,-13.0508216223155));
#12164=CARTESIAN_POINT('Ctrl Pts',(48.706329375,35.937500006828,1.293339198242E-14));
#12165=CARTESIAN_POINT('Ctrl Pts',(48.706329375,35.7291666734946,13.0508216223155));
#12166=CARTESIAN_POINT('Ctrl Pts',(42.1809185638422,35.5208333401613,24.3531646875));
#12167=CARTESIAN_POINT('Ctrl Pts',(35.6555077526845,35.312500006828,35.6555077526845));
#12168=CARTESIAN_POINT('Ctrl Pts',(24.3531646875,35.1041666734946,42.1809185638422));
#12169=CARTESIAN_POINT('Ctrl Pts',(13.0508216223155,34.8958333401613,48.706329375));
#12170=CARTESIAN_POINT('Ctrl Pts',(-9.95098946405443E-15,34.687500006828,
48.706329375));
#12171=CARTESIAN_POINT('Ctrl Pts',(-13.0508216223155,34.4791666734946,48.706329375));
#12172=CARTESIAN_POINT('Ctrl Pts',(-24.3531646875,34.2708333401613,42.1809185638423));
#12173=CARTESIAN_POINT('Ctrl Pts',(-35.6555077526845,34.062500006828,35.6555077526845));
#12174=CARTESIAN_POINT('Ctrl Pts',(-42.1809185638422,33.8541666734946,24.3531646875));
#12175=CARTESIAN_POINT('Ctrl Pts',(-48.706329375,33.6458333401613,13.0508216223155));
#12176=CARTESIAN_POINT('Ctrl Pts',(-48.706329375,33.437500006828,-1.8898197019151E-14));
#12177=CARTESIAN_POINT('Ctrl Pts',(-48.706329375,33.2291666734946,-13.0508216223155));
#12178=CARTESIAN_POINT('Ctrl Pts',(-42.1809185638422,33.0208333401613,-24.3531646875));
#12179=CARTESIAN_POINT('Ctrl Pts',(-35.6555077526845,32.812500006828,-35.6555077526845));
#12180=CARTESIAN_POINT('Ctrl Pts',(-24.3531646875,32.6041666734946,-42.1809185638422));
#12181=CARTESIAN_POINT('Ctrl Pts',(-13.0508216223155,32.3958333401613,-48.706329375));
#12182=CARTESIAN_POINT('Ctrl Pts',(1.59157945007855E-14,32.187500006828,
-48.706329375));
#12183=CARTESIAN_POINT('Ctrl Pts',(13.0508216223155,31.9791666734946,-48.706329375));
#12184=CARTESIAN_POINT('Ctrl Pts',(24.3531646875,31.7708333401613,-42.1809185638422));
#12185=CARTESIAN_POINT('Ctrl Pts',(35.6555077526845,31.562500006828,-35.6555077526845));
#12186=CARTESIAN_POINT('Ctrl Pts',(42.1809185638422,31.3541666734946,-24.3531646875));
#12187=CARTESIAN_POINT('Ctrl Pts',(48.706329375,31.1458333401613,-13.0508216223155));
#12188=CARTESIAN_POINT('Ctrl Pts',(48.706329375,30.937500006828,1.293339198242E-14));
#12189=CARTESIAN_POINT('Ctrl Pts',(48.706329375,30.7291666734946,13.0508216223155));
#12190=CARTESIAN_POINT('Ctrl Pts',(42.1809185638422,30.5208333401613,24.3531646875));
#12191=CARTESIAN_POINT('Ctrl Pts',(35.6555077526845,30.312500006828,35.6555077526845));
#12192=CARTESIAN_POINT('Ctrl Pts',(24.3531646875,30.1041666734946,42.1809185638422));
#12193=CARTESIAN_POINT('Ctrl Pts',(13.0508216223155,29.8958333401613,48.706329375));
#12194=CARTESIAN_POINT('Ctrl Pts',(-9.95098946405443E-15,29.687500006828,
48.706329375));
#12195=CARTESIAN_POINT('Ctrl Pts',(-13.0508216223155,29.4791666734946,48.706329375));
#12196=CARTESIAN_POINT('Ctrl Pts',(-24.3531646875,29.2708333401613,42.1809185638423));
#12197=CARTESIAN_POINT('Ctrl Pts',(-35.6555077526845,29.062500006828,35.6555077526845));
#12198=CARTESIAN_POINT('Ctrl Pts',(-42.1809185638422,28.8541666734946,24.3531646875));
#12199=CARTESIAN_POINT('Ctrl Pts',(-48.706329375,28.6458333401613,13.0508216223155));
#12200=CARTESIAN_POINT('Ctrl Pts',(-48.706329375,28.437500006828,-1.8898197019151E-14));
#12201=CARTESIAN_POINT('Ctrl Pts',(-46.,60.,0.));
#12202=CARTESIAN_POINT('Ctrl Pts',(-46.,59.7916666666667,-12.3256628518316));
#12203=CARTESIAN_POINT('Ctrl Pts',(-39.8371685740842,59.5833333333333,-23.));
#12204=CARTESIAN_POINT('Ctrl Pts',(-33.6743371481684,59.375,-33.6743371481684));
#12205=CARTESIAN_POINT('Ctrl Pts',(-23.,59.1666666666667,-39.8371685740842));
#12206=CARTESIAN_POINT('Ctrl Pts',(-12.3256628518317,58.9583333333333,-46.));
#12207=CARTESIAN_POINT('Ctrl Pts',(-2.81668763803891E-15,58.75,-46.));
#12208=CARTESIAN_POINT('Ctrl Pts',(12.3256628518316,58.5416666666667,-46.));
#12209=CARTESIAN_POINT('Ctrl Pts',(23.,58.3333333333333,-39.8371685740842));
#12210=CARTESIAN_POINT('Ctrl Pts',(33.6743371481683,58.125,-33.6743371481684));
#12211=CARTESIAN_POINT('Ctrl Pts',(39.8371685740842,57.9166666666667,-23.));
#12212=CARTESIAN_POINT('Ctrl Pts',(46.,57.7083333333333,-12.3256628518317));
#12213=CARTESIAN_POINT('Ctrl Pts',(46.,57.5,-5.63337527607782E-15));
#12214=CARTESIAN_POINT('Ctrl Pts',(46.,57.2916666666667,12.3256628518316));
#12215=CARTESIAN_POINT('Ctrl Pts',(39.8371685740842,57.0833333333333,23.));
#12216=CARTESIAN_POINT('Ctrl Pts',(33.6743371481684,56.875,33.6743371481683));
#12217=CARTESIAN_POINT('Ctrl Pts',(23.,56.6666666666667,39.8371685740842));
#12218=CARTESIAN_POINT('Ctrl Pts',(12.3256628518317,56.4583333333333,46.));
#12219=CARTESIAN_POINT('Ctrl Pts',(8.45006291411674E-15,56.25,46.));
#12220=CARTESIAN_POINT('Ctrl Pts',(-12.3256628518316,56.0416666666667,46.));
#12221=CARTESIAN_POINT('Ctrl Pts',(-23.,55.8333333333333,39.8371685740842));
#12222=CARTESIAN_POINT('Ctrl Pts',(-33.6743371481683,55.625,33.6743371481684));
#12223=CARTESIAN_POINT('Ctrl Pts',(-39.8371685740842,55.4166666666667,23.));
#12224=CARTESIAN_POINT('Ctrl Pts',(-46.,55.2083333333333,12.3256628518317));
#12225=CARTESIAN_POINT('Ctrl Pts',(-46.,55.,0.));
#12226=CARTESIAN_POINT('Ctrl Pts',(-46.,54.7916666666667,-12.3256628518316));
#12227=CARTESIAN_POINT('Ctrl Pts',(-39.8371685740842,54.5833333333333,-23.));
#12228=CARTESIAN_POINT('Ctrl Pts',(-33.6743371481684,54.375,-33.6743371481684));
#12229=CARTESIAN_POINT('Ctrl Pts',(-23.,54.1666666666667,-39.8371685740842));
#12230=CARTESIAN_POINT('Ctrl Pts',(-12.3256628518317,53.9583333333333,-46.));
#12231=CARTESIAN_POINT('Ctrl Pts',(-2.81668763803891E-15,53.75,-46.));
#12232=CARTESIAN_POINT('Ctrl Pts',(12.3256628518316,53.5416666666667,-46.));
#12233=CARTESIAN_POINT('Ctrl Pts',(23.,53.3333333333333,-39.8371685740842));
#12234=CARTESIAN_POINT('Ctrl Pts',(33.6743371481683,53.125,-33.6743371481684));
#12235=CARTESIAN_POINT('Ctrl Pts',(39.8371685740842,52.9166666666667,-23.));
#12236=CARTESIAN_POINT('Ctrl Pts',(46.,52.7083333333333,-12.3256628518317));
#12237=CARTESIAN_POINT('Ctrl Pts',(46.,52.5,-5.63337527607782E-15));
#12238=CARTESIAN_POINT('Ctrl Pts',(46.,52.2916666666667,12.3256628518316));
#12239=CARTESIAN_POINT('Ctrl Pts',(39.8371685740842,52.0833333333333,23.));
#12240=CARTESIAN_POINT('Ctrl Pts',(33.6743371481684,51.875,33.6743371481683));
#12241=CARTESIAN_POINT('Ctrl Pts',(23.,51.6666666666667,39.8371685740842));
#12242=CARTESIAN_POINT('Ctrl Pts',(12.3256628518317,51.4583333333333,46.));
#12243=CARTESIAN_POINT('Ctrl Pts',(8.45006291411674E-15,51.25,46.));
#12244=CARTESIAN_POINT('Ctrl Pts',(-12.3256628518316,51.0416666666667,46.));
#12245=CARTESIAN_POINT('Ctrl Pts',(-23.,50.8333333333333,39.8371685740842));
#12246=CARTESIAN_POINT('Ctrl Pts',(-33.6743371481683,50.625,33.6743371481684));
#12247=CARTESIAN_POINT('Ctrl Pts',(-39.8371685740842,50.4166666666667,23.));
#12248=CARTESIAN_POINT('Ctrl Pts',(-46.,50.2083333333333,12.3256628518317));
#12249=CARTESIAN_POINT('Ctrl Pts',(-46.,50.,0.));
#12250=CARTESIAN_POINT('Ctrl Pts',(-46.,49.7916666666667,-12.3256628518316));
#12251=CARTESIAN_POINT('Ctrl Pts',(-39.8371685740842,49.5833333333333,-23.));
#12252=CARTESIAN_POINT('Ctrl Pts',(-33.6743371481684,49.375,-33.6743371481684));
#12253=CARTESIAN_POINT('Ctrl Pts',(-23.,49.1666666666667,-39.8371685740842));
#12254=CARTESIAN_POINT('Ctrl Pts',(-12.3256628518317,48.9583333333333,-46.));
#12255=CARTESIAN_POINT('Ctrl Pts',(-2.81668763803891E-15,48.75,-46.));
#12256=CARTESIAN_POINT('Ctrl Pts',(12.3256628518316,48.5416666666667,-46.));
#12257=CARTESIAN_POINT('Ctrl Pts',(23.,48.3333333333333,-39.8371685740842));
#12258=CARTESIAN_POINT('Ctrl Pts',(33.6743371481683,48.125,-33.6743371481684));
#12259=CARTESIAN_POINT('Ctrl Pts',(39.8371685740842,47.9166666666667,-23.));
#12260=CARTESIAN_POINT('Ctrl Pts',(46.,47.7083333333333,-12.3256628518317));
#12261=CARTESIAN_POINT('Ctrl Pts',(46.,47.5,-5.63337527607782E-15));
#12262=CARTESIAN_POINT('Ctrl Pts',(46.,47.2916666666667,12.3256628518316));
#12263=CARTESIAN_POINT('Ctrl Pts',(39.8371685740842,47.0833333333333,23.));
#12264=CARTESIAN_POINT('Ctrl Pts',(33.6743371481684,46.875,33.6743371481683));
#12265=CARTESIAN_POINT('Ctrl Pts',(23.,46.6666666666667,39.8371685740842));
#12266=CARTESIAN_POINT('Ctrl Pts',(12.3256628518317,46.4583333333333,46.));
#12267=CARTESIAN_POINT('Ctrl Pts',(8.45006291411674E-15,46.25,46.));
#12268=CARTESIAN_POINT('Ctrl Pts',(-12.3256628518316,46.0416666666667,46.));
#12269=CARTESIAN_POINT('Ctrl Pts',(-23.,45.8333333333333,39.8371685740842));
#12270=CARTESIAN_POINT('Ctrl Pts',(-33.6743371481683,45.625,33.6743371481684));
#12271=CARTESIAN_POINT('Ctrl Pts',(-39.8371685740842,45.4166666666667,23.));
#12272=CARTESIAN_POINT('Ctrl Pts',(-46.,45.2083333333333,12.3256628518317));
#12273=CARTESIAN_POINT('Ctrl Pts',(-46.,45.,0.));
#12274=CARTESIAN_POINT('Ctrl Pts',(-46.,44.7916666666667,-12.3256628518316));
#12275=CARTESIAN_POINT('Ctrl Pts',(-39.8371685740842,44.5833333333333,-23.));
#12276=CARTESIAN_POINT('Ctrl Pts',(-33.6743371481684,44.375,-33.6743371481684));
#12277=CARTESIAN_POINT('Ctrl Pts',(-23.,44.1666666666667,-39.8371685740842));
#12278=CARTESIAN_POINT('Ctrl Pts',(-12.3256628518317,43.9583333333333,-46.));
#12279=CARTESIAN_POINT('Ctrl Pts',(-2.81668763803891E-15,43.75,-46.));
#12280=CARTESIAN_POINT('Ctrl Pts',(12.3256628518316,43.5416666666667,-46.));
#12281=CARTESIAN_POINT('Ctrl Pts',(23.,43.3333333333333,-39.8371685740842));
#12282=CARTESIAN_POINT('Ctrl Pts',(33.6743371481683,43.125,-33.6743371481684));
#12283=CARTESIAN_POINT('Ctrl Pts',(39.8371685740842,42.9166666666667,-23.));
#12284=CARTESIAN_POINT('Ctrl Pts',(46.,42.7083333333333,-12.3256628518317));
#12285=CARTESIAN_POINT('Ctrl Pts',(46.,42.5,-5.63337527607782E-15));
#12286=CARTESIAN_POINT('Ctrl Pts',(46.,42.2916666666667,12.3256628518316));
#12287=CARTESIAN_POINT('Ctrl Pts',(39.8371685740842,42.0833333333333,23.));
#12288=CARTESIAN_POINT('Ctrl Pts',(33.6743371481684,41.875,33.6743371481683));
#12289=CARTESIAN_POINT('Ctrl Pts',(23.,41.6666666666667,39.8371685740842));
#12290=CARTESIAN_POINT('Ctrl Pts',(12.3256628518317,41.4583333333333,46.));
#12291=CARTESIAN_POINT('Ctrl Pts',(8.45006291411674E-15,41.25,46.));
#12292=CARTESIAN_POINT('Ctrl Pts',(-12.3256628518316,41.0416666666667,46.));
#12293=CARTESIAN_POINT('Ctrl Pts',(-23.,40.8333333333333,39.8371685740842));
#12294=CARTESIAN_POINT('Ctrl Pts',(-33.6743371481683,40.625,33.6743371481684));
#12295=CARTESIAN_POINT('Ctrl Pts',(-39.8371685740842,40.4166666666667,23.));
#12296=CARTESIAN_POINT('Ctrl Pts',(-46.,40.2083333333333,12.3256628518317));
#12297=CARTESIAN_POINT('Ctrl Pts',(-46.,40.,0.));
#12298=CARTESIAN_POINT('Ctrl Pts',(-46.,39.7916666666667,-12.3256628518316));
#12299=CARTESIAN_POINT('Ctrl Pts',(-39.8371685740842,39.5833333333333,-23.));
#12300=CARTESIAN_POINT('Ctrl Pts',(-33.6743371481684,39.375,-33.6743371481684));
#12301=CARTESIAN_POINT('Ctrl Pts',(-23.,39.1666666666667,-39.8371685740842));
#12302=CARTESIAN_POINT('Ctrl Pts',(-12.3256628518317,38.9583333333333,-46.));
#12303=CARTESIAN_POINT('Ctrl Pts',(-2.81668763803891E-15,38.75,-46.));
#12304=CARTESIAN_POINT('Ctrl Pts',(12.3256628518316,38.5416666666667,-46.));
#12305=CARTESIAN_POINT('Ctrl Pts',(23.,38.3333333333333,-39.8371685740842));
#12306=CARTESIAN_POINT('Ctrl Pts',(33.6743371481683,38.125,-33.6743371481684));
#12307=CARTESIAN_POINT('Ctrl Pts',(39.8371685740842,37.9166666666667,-23.));
#12308=CARTESIAN_POINT('Ctrl Pts',(46.,37.7083333333333,-12.3256628518317));
#12309=CARTESIAN_POINT('Ctrl Pts',(46.,37.5,-5.63337527607782E-15));
#12310=CARTESIAN_POINT('Ctrl Pts',(46.,37.2916666666667,12.3256628518316));
#12311=CARTESIAN_POINT('Ctrl Pts',(39.8371685740842,37.0833333333333,23.));
#12312=CARTESIAN_POINT('Ctrl Pts',(33.6743371481684,36.875,33.6743371481683));
#12313=CARTESIAN_POINT('Ctrl Pts',(23.,36.6666666666667,39.8371685740842));
#12314=CARTESIAN_POINT('Ctrl Pts',(12.3256628518317,36.4583333333333,46.));
#12315=CARTESIAN_POINT('Ctrl Pts',(8.45006291411674E-15,36.25,46.));
#12316=CARTESIAN_POINT('Ctrl Pts',(-12.3256628518316,36.0416666666667,46.));
#12317=CARTESIAN_POINT('Ctrl Pts',(-23.,35.8333333333333,39.8371685740842));
#12318=CARTESIAN_POINT('Ctrl Pts',(-33.6743371481683,35.625,33.6743371481684));
#12319=CARTESIAN_POINT('Ctrl Pts',(-39.8371685740842,35.4166666666667,23.));
#12320=CARTESIAN_POINT('Ctrl Pts',(-46.,35.2083333333333,12.3256628518317));
#12321=CARTESIAN_POINT('Ctrl Pts',(-46.,35.,0.));
#12322=CARTESIAN_POINT('Ctrl Pts',(-46.,34.7916666666667,-12.3256628518316));
#12323=CARTESIAN_POINT('Ctrl Pts',(-39.8371685740842,34.5833333333333,-23.));
#12324=CARTESIAN_POINT('Ctrl Pts',(-33.6743371481684,34.375,-33.6743371481684));
#12325=CARTESIAN_POINT('Ctrl Pts',(-23.,34.1666666666667,-39.8371685740842));
#12326=CARTESIAN_POINT('Ctrl Pts',(-12.3256628518317,33.9583333333333,-46.));
#12327=CARTESIAN_POINT('Ctrl Pts',(-2.81668763803891E-15,33.75,-46.));
#12328=CARTESIAN_POINT('Ctrl Pts',(12.3256628518316,33.5416666666667,-46.));
#12329=CARTESIAN_POINT('Ctrl Pts',(23.,33.3333333333333,-39.8371685740842));
#12330=CARTESIAN_POINT('Ctrl Pts',(33.6743371481683,33.125,-33.6743371481684));
#12331=CARTESIAN_POINT('Ctrl Pts',(39.8371685740842,32.9166666666667,-23.));
#12332=CARTESIAN_POINT('Ctrl Pts',(46.,32.7083333333333,-12.3256628518317));
#12333=CARTESIAN_POINT('Ctrl Pts',(46.,32.5,-5.63337527607782E-15));
#12334=CARTESIAN_POINT('Ctrl Pts',(46.,32.2916666666667,12.3256628518316));
#12335=CARTESIAN_POINT('Ctrl Pts',(39.8371685740842,32.0833333333333,23.));
#12336=CARTESIAN_POINT('Ctrl Pts',(33.6743371481684,31.875,33.6743371481683));
#12337=CARTESIAN_POINT('Ctrl Pts',(23.,31.6666666666667,39.8371685740842));
#12338=CARTESIAN_POINT('Ctrl Pts',(12.3256628518317,31.4583333333333,46.));
#12339=CARTESIAN_POINT('Ctrl Pts',(8.45006291411674E-15,31.25,46.));
#12340=CARTESIAN_POINT('Ctrl Pts',(-12.3256628518316,31.0416666666667,46.));
#12341=CARTESIAN_POINT('Ctrl Pts',(-23.,30.8333333333333,39.8371685740842));
#12342=CARTESIAN_POINT('Ctrl Pts',(-33.6743371481683,30.625,33.6743371481684));
#12343=CARTESIAN_POINT('Ctrl Pts',(-39.8371685740842,30.4166666666667,23.));
#12344=CARTESIAN_POINT('Ctrl Pts',(-46.,30.2083333333333,12.3256628518317));
#12345=CARTESIAN_POINT('Ctrl Pts',(-46.,30.,0.));
#12346=CARTESIAN_POINT('Ctrl Pts',(48.5725845633798,50.8793483229262,3.60701400320328));
#12347=CARTESIAN_POINT('Ctrl Pts',(48.3407853679392,51.0125314497137,3.60701400320328));
#12348=CARTESIAN_POINT('Ctrl Pts',(48.1089821836664,51.1457076343818,3.60701400320327));
#12349=CARTESIAN_POINT('Ctrl Pts',(47.6453674864979,51.4120455056142,3.60701400320327));
#12350=CARTESIAN_POINT('Ctrl Pts',(47.4135559734254,51.5452071923974,3.60701400320325));
#12351=CARTESIAN_POINT('Ctrl Pts',(47.1817401099609,51.6783613050641,3.60701400320325));
#12352=CARTESIAN_POINT('Ctrl Pts',(46.7406305897488,51.9317328641751,3.60701400320325));
#12353=CARTESIAN_POINT('Ctrl Pts',(46.2995053259033,52.1850770165971,3.60701400320324));
#12354=CARTESIAN_POINT('Ctrl Pts',(45.858362923034,52.438391319744,3.60701400320324));
#12355=CARTESIAN_POINT('Ctrl Pts',(3.61292728433799,51.311710737147,45.8578974271399));
#12356=CARTESIAN_POINT('Ctrl Pts',(3.61292728433798,51.178117727701,46.089460636719));
#12357=CARTESIAN_POINT('Ctrl Pts',(3.61292728433804,50.9109294856547,46.5525857733052));
#12358=CARTESIAN_POINT('Ctrl Pts',(3.61292728433797,50.6437369897944,47.0157084557285));
#12359=CARTESIAN_POINT('Ctrl Pts',(3.61292728433797,50.2553460757965,47.6888965792834));
#12360=CARTESIAN_POINT('Ctrl Pts',(3.61292728433797,50.0005487265709,48.1305218136162));
#12361=CARTESIAN_POINT('Ctrl Pts',(3.61292728433797,49.7457479656467,48.5721450795008));
#12362=CARTESIAN_POINT('Ctrl Pts',(-48.706329375,58.437500006828,-1.8898197019151E-14));
#12363=CARTESIAN_POINT('Ctrl Pts',(-48.706329375,58.2291666734946,-13.0508216223155));
#12364=CARTESIAN_POINT('Ctrl Pts',(-42.1809185638422,58.0208333401613,-24.3531646875));
#12365=CARTESIAN_POINT('Ctrl Pts',(-35.6555077526845,57.812500006828,-35.6555077526845));
#12366=CARTESIAN_POINT('Ctrl Pts',(-24.3531646875,57.6041666734946,-42.1809185638422));
#12367=CARTESIAN_POINT('Ctrl Pts',(-13.0508216223155,57.3958333401613,-48.706329375));
#12368=CARTESIAN_POINT('Ctrl Pts',(1.59157945007855E-14,57.187500006828,
-48.706329375));
#12369=CARTESIAN_POINT('Ctrl Pts',(13.0508216223155,56.9791666734946,-48.706329375));
#12370=CARTESIAN_POINT('Ctrl Pts',(24.3531646875,56.7708333401613,-42.1809185638422));
#12371=CARTESIAN_POINT('Ctrl Pts',(35.6555077526845,56.562500006828,-35.6555077526845));
#12372=CARTESIAN_POINT('Ctrl Pts',(42.1809185638422,56.3541666734946,-24.3531646875));
#12373=CARTESIAN_POINT('Ctrl Pts',(48.706329375,56.1458333401613,-13.0508216223155));
#12374=CARTESIAN_POINT('Ctrl Pts',(48.706329375,55.937500006828,1.293339198242E-14));
#12375=CARTESIAN_POINT('Ctrl Pts',(48.706329375,55.7291666734946,13.0508216223155));
#12376=CARTESIAN_POINT('Ctrl Pts',(42.1809185638422,55.5208333401613,24.3531646875));
#12377=CARTESIAN_POINT('Ctrl Pts',(35.6555077526845,55.312500006828,35.6555077526845));
#12378=CARTESIAN_POINT('Ctrl Pts',(24.3531646875,55.1041666734946,42.1809185638422));
#12379=CARTESIAN_POINT('Ctrl Pts',(13.0508216223155,54.8958333401613,48.706329375));
#12380=CARTESIAN_POINT('Ctrl Pts',(-9.95098946405443E-15,54.687500006828,
48.706329375));
#12381=CARTESIAN_POINT('Ctrl Pts',(-13.0508216223155,54.4791666734946,48.706329375));
#12382=CARTESIAN_POINT('Ctrl Pts',(-24.3531646875,54.2708333401613,42.1809185638423));
#12383=CARTESIAN_POINT('Ctrl Pts',(-35.6555077526845,54.062500006828,35.6555077526845));
#12384=CARTESIAN_POINT('Ctrl Pts',(-42.1809185638422,53.8541666734946,24.3531646875));
#12385=CARTESIAN_POINT('Ctrl Pts',(-48.706329375,53.6458333401613,13.0508216223155));
#12386=CARTESIAN_POINT('Ctrl Pts',(-48.706329375,53.437500006828,-1.8898197019151E-14));
#12387=CARTESIAN_POINT('Ctrl Pts',(-48.706329375,53.2291666734946,-13.0508216223155));
#12388=CARTESIAN_POINT('Ctrl Pts',(-42.1809185638422,53.0208333401613,-24.3531646875));
#12389=CARTESIAN_POINT('Ctrl Pts',(-35.6555077526845,52.812500006828,-35.6555077526845));
#12390=CARTESIAN_POINT('Ctrl Pts',(-24.3531646875,52.6041666734946,-42.1809185638422));
#12391=CARTESIAN_POINT('Ctrl Pts',(-13.0508216223155,52.3958333401613,-48.706329375));
#12392=CARTESIAN_POINT('Ctrl Pts',(1.59157945007855E-14,52.187500006828,
-48.706329375));
#12393=CARTESIAN_POINT('Ctrl Pts',(13.0508216223155,51.9791666734946,-48.706329375));
#12394=CARTESIAN_POINT('Ctrl Pts',(24.3531646875,51.7708333401613,-42.1809185638422));
#12395=CARTESIAN_POINT('Ctrl Pts',(35.6555077526845,51.562500006828,-35.6555077526845));
#12396=CARTESIAN_POINT('Ctrl Pts',(42.1809185638422,51.3541666734946,-24.3531646875));
#12397=CARTESIAN_POINT('Ctrl Pts',(48.706329375,51.1458333401613,-13.0508216223155));
#12398=CARTESIAN_POINT('Ctrl Pts',(48.706329375,50.937500006828,1.293339198242E-14));
#12399=CARTESIAN_POINT('Ctrl Pts',(48.706329375,50.7291666734946,13.0508216223155));
#12400=CARTESIAN_POINT('Ctrl Pts',(42.1809185638422,50.5208333401613,24.3531646875));
#12401=CARTESIAN_POINT('Ctrl Pts',(35.6555077526845,50.312500006828,35.6555077526845));
#12402=CARTESIAN_POINT('Ctrl Pts',(24.3531646875,50.1041666734946,42.1809185638422));
#12403=CARTESIAN_POINT('Ctrl Pts',(13.0508216223155,49.8958333401613,48.706329375));
#12404=CARTESIAN_POINT('Ctrl Pts',(-9.95098946405443E-15,49.687500006828,
48.706329375));
#12405=CARTESIAN_POINT('Ctrl Pts',(-13.0508216223155,49.4791666734946,48.706329375));
#12406=CARTESIAN_POINT('Ctrl Pts',(-24.3531646875,49.2708333401613,42.1809185638423));
#12407=CARTESIAN_POINT('Ctrl Pts',(-35.6555077526845,49.062500006828,35.6555077526845));
#12408=CARTESIAN_POINT('Ctrl Pts',(-42.1809185638422,48.8541666734946,24.3531646875));
#12409=CARTESIAN_POINT('Ctrl Pts',(-48.706329375,48.6458333401613,13.0508216223155));
#12410=CARTESIAN_POINT('Ctrl Pts',(-48.706329375,48.437500006828,-1.8898197019151E-14));
#12411=CARTESIAN_POINT('Ctrl Pts',(-48.706329375,48.2291666734946,-13.0508216223155));
#12412=CARTESIAN_POINT('Ctrl Pts',(-42.1809185638422,48.0208333401613,-24.3531646875));
#12413=CARTESIAN_POINT('Ctrl Pts',(-35.6555077526845,47.812500006828,-35.6555077526845));
#12414=CARTESIAN_POINT('Ctrl Pts',(-24.3531646875,47.6041666734946,-42.1809185638422));
#12415=CARTESIAN_POINT('Ctrl Pts',(-13.0508216223155,47.3958333401613,-48.706329375));
#12416=CARTESIAN_POINT('Ctrl Pts',(1.59157945007855E-14,47.187500006828,
-48.706329375));
#12417=CARTESIAN_POINT('Ctrl Pts',(13.0508216223155,46.9791666734946,-48.706329375));
#12418=CARTESIAN_POINT('Ctrl Pts',(24.3531646875,46.7708333401613,-42.1809185638422));
#12419=CARTESIAN_POINT('Ctrl Pts',(35.6555077526845,46.562500006828,-35.6555077526845));
#12420=CARTESIAN_POINT('Ctrl Pts',(42.1809185638422,46.3541666734946,-24.3531646875));
#12421=CARTESIAN_POINT('Ctrl Pts',(48.706329375,46.1458333401613,-13.0508216223155));
#12422=CARTESIAN_POINT('Ctrl Pts',(48.706329375,45.937500006828,1.293339198242E-14));
#12423=CARTESIAN_POINT('Ctrl Pts',(48.706329375,45.7291666734946,13.0508216223155));
#12424=CARTESIAN_POINT('Ctrl Pts',(42.1809185638422,45.5208333401613,24.3531646875));
#12425=CARTESIAN_POINT('Ctrl Pts',(35.6555077526845,45.312500006828,35.6555077526845));
#12426=CARTESIAN_POINT('Ctrl Pts',(24.3531646875,45.1041666734946,42.1809185638422));
#12427=CARTESIAN_POINT('Ctrl Pts',(13.0508216223155,44.8958333401613,48.706329375));
#12428=CARTESIAN_POINT('Ctrl Pts',(-9.95098946405443E-15,44.687500006828,
48.706329375));
#12429=CARTESIAN_POINT('Ctrl Pts',(-13.0508216223155,44.4791666734946,48.706329375));
#12430=CARTESIAN_POINT('Ctrl Pts',(-24.3531646875,44.2708333401613,42.1809185638423));
#12431=CARTESIAN_POINT('Ctrl Pts',(-35.6555077526845,44.062500006828,35.6555077526845));
#12432=CARTESIAN_POINT('Ctrl Pts',(-42.1809185638422,43.8541666734946,24.3531646875));
#12433=CARTESIAN_POINT('Ctrl Pts',(-48.706329375,43.6458333401613,13.0508216223155));
#12434=CARTESIAN_POINT('Ctrl Pts',(-48.706329375,43.437500006828,-1.8898197019151E-14));
#12435=CARTESIAN_POINT('Ctrl Pts',(-48.706329375,43.2291666734946,-13.0508216223155));
#12436=CARTESIAN_POINT('Ctrl Pts',(-42.1809185638422,43.0208333401613,-24.3531646875));
#12437=CARTESIAN_POINT('Ctrl Pts',(-35.6555077526845,42.812500006828,-35.6555077526845));
#12438=CARTESIAN_POINT('Ctrl Pts',(-24.3531646875,42.6041666734946,-42.1809185638422));
#12439=CARTESIAN_POINT('Ctrl Pts',(-13.0508216223155,42.3958333401613,-48.706329375));
#12440=CARTESIAN_POINT('Ctrl Pts',(1.59157945007855E-14,42.187500006828,
-48.706329375));
#12441=CARTESIAN_POINT('Ctrl Pts',(13.0508216223155,41.9791666734946,-48.706329375));
#12442=CARTESIAN_POINT('Ctrl Pts',(24.3531646875,41.7708333401613,-42.1809185638422));
#12443=CARTESIAN_POINT('Ctrl Pts',(35.6555077526845,41.562500006828,-35.6555077526845));
#12444=CARTESIAN_POINT('Ctrl Pts',(42.1809185638422,41.3541666734946,-24.3531646875));
#12445=CARTESIAN_POINT('Ctrl Pts',(48.706329375,41.1458333401613,-13.0508216223155));
#12446=CARTESIAN_POINT('Ctrl Pts',(48.706329375,40.937500006828,1.293339198242E-14));
#12447=CARTESIAN_POINT('Ctrl Pts',(48.706329375,40.7291666734946,13.0508216223155));
#12448=CARTESIAN_POINT('Ctrl Pts',(42.1809185638422,40.5208333401613,24.3531646875));
#12449=CARTESIAN_POINT('Ctrl Pts',(35.6555077526845,40.312500006828,35.6555077526845));
#12450=CARTESIAN_POINT('Ctrl Pts',(24.3531646875,40.1041666734946,42.1809185638422));
#12451=CARTESIAN_POINT('Ctrl Pts',(13.0508216223155,39.8958333401613,48.706329375));
#12452=CARTESIAN_POINT('Ctrl Pts',(-9.95098946405443E-15,39.687500006828,
48.706329375));
#12453=CARTESIAN_POINT('Ctrl Pts',(-13.0508216223155,39.4791666734946,48.706329375));
#12454=CARTESIAN_POINT('Ctrl Pts',(-24.3531646875,39.2708333401613,42.1809185638423));
#12455=CARTESIAN_POINT('Ctrl Pts',(-35.6555077526845,39.062500006828,35.6555077526845));
#12456=CARTESIAN_POINT('Ctrl Pts',(-42.1809185638422,38.8541666734946,24.3531646875));
#12457=CARTESIAN_POINT('Ctrl Pts',(-48.706329375,38.6458333401613,13.0508216223155));
#12458=CARTESIAN_POINT('Ctrl Pts',(-48.706329375,38.437500006828,-1.8898197019151E-14));
#12459=CARTESIAN_POINT('Ctrl Pts',(-48.706329375,38.2291666734946,-13.0508216223155));
#12460=CARTESIAN_POINT('Ctrl Pts',(-42.1809185638422,38.0208333401613,-24.3531646875));
#12461=CARTESIAN_POINT('Ctrl Pts',(-35.6555077526845,37.812500006828,-35.6555077526845));
#12462=CARTESIAN_POINT('Ctrl Pts',(-24.3531646875,37.6041666734946,-42.1809185638422));
#12463=CARTESIAN_POINT('Ctrl Pts',(-13.0508216223155,37.3958333401613,-48.706329375));
#12464=CARTESIAN_POINT('Ctrl Pts',(1.59157945007855E-14,37.187500006828,
-48.706329375));
#12465=CARTESIAN_POINT('Ctrl Pts',(13.0508216223155,36.9791666734946,-48.706329375));
#12466=CARTESIAN_POINT('Ctrl Pts',(24.3531646875,36.7708333401613,-42.1809185638422));
#12467=CARTESIAN_POINT('Ctrl Pts',(35.6555077526845,36.562500006828,-35.6555077526845));
#12468=CARTESIAN_POINT('Ctrl Pts',(42.1809185638422,36.3541666734946,-24.3531646875));
#12469=CARTESIAN_POINT('Ctrl Pts',(48.706329375,36.1458333401613,-13.0508216223155));
#12470=CARTESIAN_POINT('Ctrl Pts',(48.706329375,35.937500006828,1.293339198242E-14));
#12471=CARTESIAN_POINT('Ctrl Pts',(48.706329375,35.7291666734946,13.0508216223155));
#12472=CARTESIAN_POINT('Ctrl Pts',(42.1809185638422,35.5208333401613,24.3531646875));
#12473=CARTESIAN_POINT('Ctrl Pts',(35.6555077526845,35.312500006828,35.6555077526845));
#12474=CARTESIAN_POINT('Ctrl Pts',(24.3531646875,35.1041666734946,42.1809185638422));
#12475=CARTESIAN_POINT('Ctrl Pts',(13.0508216223155,34.8958333401613,48.706329375));
#12476=CARTESIAN_POINT('Ctrl Pts',(-9.95098946405443E-15,34.687500006828,
48.706329375));
#12477=CARTESIAN_POINT('Ctrl Pts',(-13.0508216223155,34.4791666734946,48.706329375));
#12478=CARTESIAN_POINT('Ctrl Pts',(-24.3531646875,34.2708333401613,42.1809185638423));
#12479=CARTESIAN_POINT('Ctrl Pts',(-35.6555077526845,34.062500006828,35.6555077526845));
#12480=CARTESIAN_POINT('Ctrl Pts',(-42.1809185638422,33.8541666734946,24.3531646875));
#12481=CARTESIAN_POINT('Ctrl Pts',(-48.706329375,33.6458333401613,13.0508216223155));
#12482=CARTESIAN_POINT('Ctrl Pts',(-48.706329375,33.437500006828,-1.8898197019151E-14));
#12483=CARTESIAN_POINT('Ctrl Pts',(-48.706329375,33.2291666734946,-13.0508216223155));
#12484=CARTESIAN_POINT('Ctrl Pts',(-42.1809185638422,33.0208333401613,-24.3531646875));
#12485=CARTESIAN_POINT('Ctrl Pts',(-35.6555077526845,32.812500006828,-35.6555077526845));
#12486=CARTESIAN_POINT('Ctrl Pts',(-24.3531646875,32.6041666734946,-42.1809185638422));
#12487=CARTESIAN_POINT('Ctrl Pts',(-13.0508216223155,32.3958333401613,-48.706329375));
#12488=CARTESIAN_POINT('Ctrl Pts',(1.59157945007855E-14,32.187500006828,
-48.706329375));
#12489=CARTESIAN_POINT('Ctrl Pts',(13.0508216223155,31.9791666734946,-48.706329375));
#12490=CARTESIAN_POINT('Ctrl Pts',(24.3531646875,31.7708333401613,-42.1809185638422));
#12491=CARTESIAN_POINT('Ctrl Pts',(35.6555077526845,31.562500006828,-35.6555077526845));
#12492=CARTESIAN_POINT('Ctrl Pts',(42.1809185638422,31.3541666734946,-24.3531646875));
#12493=CARTESIAN_POINT('Ctrl Pts',(48.706329375,31.1458333401613,-13.0508216223155));
#12494=CARTESIAN_POINT('Ctrl Pts',(48.706329375,30.937500006828,1.293339198242E-14));
#12495=CARTESIAN_POINT('Ctrl Pts',(48.706329375,30.7291666734946,13.0508216223155));
#12496=CARTESIAN_POINT('Ctrl Pts',(42.1809185638422,30.5208333401613,24.3531646875));
#12497=CARTESIAN_POINT('Ctrl Pts',(35.6555077526845,30.312500006828,35.6555077526845));
#12498=CARTESIAN_POINT('Ctrl Pts',(24.3531646875,30.1041666734946,42.1809185638422));
#12499=CARTESIAN_POINT('Ctrl Pts',(13.0508216223155,29.8958333401613,48.706329375));
#12500=CARTESIAN_POINT('Ctrl Pts',(-9.95098946405443E-15,29.687500006828,
48.706329375));
#12501=CARTESIAN_POINT('Ctrl Pts',(-13.0508216223155,29.4791666734946,48.706329375));
#12502=CARTESIAN_POINT('Ctrl Pts',(-24.3531646875,29.2708333401613,42.1809185638423));
#12503=CARTESIAN_POINT('Ctrl Pts',(-35.6555077526845,29.062500006828,35.6555077526845));
#12504=CARTESIAN_POINT('Ctrl Pts',(-42.1809185638422,28.8541666734946,24.3531646875));
#12505=CARTESIAN_POINT('Ctrl Pts',(-48.706329375,28.6458333401613,13.0508216223155));
#12506=CARTESIAN_POINT('Ctrl Pts',(-48.706329375,28.437500006828,-1.8898197019151E-14));
#12507=CARTESIAN_POINT('Ctrl Pts',(-46.,60.,0.));
#12508=CARTESIAN_POINT('Ctrl Pts',(-46.,59.7916666666667,-12.3256628518316));
#12509=CARTESIAN_POINT('Ctrl Pts',(-39.8371685740842,59.5833333333333,-23.));
#12510=CARTESIAN_POINT('Ctrl Pts',(-33.6743371481684,59.375,-33.6743371481684));
#12511=CARTESIAN_POINT('Ctrl Pts',(-23.,59.1666666666667,-39.8371685740842));
#12512=CARTESIAN_POINT('Ctrl Pts',(-12.3256628518317,58.9583333333333,-46.));
#12513=CARTESIAN_POINT('Ctrl Pts',(-2.81668763803891E-15,58.75,-46.));
#12514=CARTESIAN_POINT('Ctrl Pts',(12.3256628518316,58.5416666666667,-46.));
#12515=CARTESIAN_POINT('Ctrl Pts',(23.,58.3333333333333,-39.8371685740842));
#12516=CARTESIAN_POINT('Ctrl Pts',(33.6743371481683,58.125,-33.6743371481684));
#12517=CARTESIAN_POINT('Ctrl Pts',(39.8371685740842,57.9166666666667,-23.));
#12518=CARTESIAN_POINT('Ctrl Pts',(46.,57.7083333333333,-12.3256628518317));
#12519=CARTESIAN_POINT('Ctrl Pts',(46.,57.5,-5.63337527607782E-15));
#12520=CARTESIAN_POINT('Ctrl Pts',(46.,57.2916666666667,12.3256628518316));
#12521=CARTESIAN_POINT('Ctrl Pts',(39.8371685740842,57.0833333333333,23.));
#12522=CARTESIAN_POINT('Ctrl Pts',(33.6743371481684,56.875,33.6743371481683));
#12523=CARTESIAN_POINT('Ctrl Pts',(23.,56.6666666666667,39.8371685740842));
#12524=CARTESIAN_POINT('Ctrl Pts',(12.3256628518317,56.4583333333333,46.));
#12525=CARTESIAN_POINT('Ctrl Pts',(8.45006291411674E-15,56.25,46.));
#12526=CARTESIAN_POINT('Ctrl Pts',(-12.3256628518316,56.0416666666667,46.));
#12527=CARTESIAN_POINT('Ctrl Pts',(-23.,55.8333333333333,39.8371685740842));
#12528=CARTESIAN_POINT('Ctrl Pts',(-33.6743371481683,55.625,33.6743371481684));
#12529=CARTESIAN_POINT('Ctrl Pts',(-39.8371685740842,55.4166666666667,23.));
#12530=CARTESIAN_POINT('Ctrl Pts',(-46.,55.2083333333333,12.3256628518317));
#12531=CARTESIAN_POINT('Ctrl Pts',(-46.,55.,0.));
#12532=CARTESIAN_POINT('Ctrl Pts',(-46.,54.7916666666667,-12.3256628518316));
#12533=CARTESIAN_POINT('Ctrl Pts',(-39.8371685740842,54.5833333333333,-23.));
#12534=CARTESIAN_POINT('Ctrl Pts',(-33.6743371481684,54.375,-33.6743371481684));
#12535=CARTESIAN_POINT('Ctrl Pts',(-23.,54.1666666666667,-39.8371685740842));
#12536=CARTESIAN_POINT('Ctrl Pts',(-12.3256628518317,53.9583333333333,-46.));
#12537=CARTESIAN_POINT('Ctrl Pts',(-2.81668763803891E-15,53.75,-46.));
#12538=CARTESIAN_POINT('Ctrl Pts',(12.3256628518316,53.5416666666667,-46.));
#12539=CARTESIAN_POINT('Ctrl Pts',(23.,53.3333333333333,-39.8371685740842));
#12540=CARTESIAN_POINT('Ctrl Pts',(33.6743371481683,53.125,-33.6743371481684));
#12541=CARTESIAN_POINT('Ctrl Pts',(39.8371685740842,52.9166666666667,-23.));
#12542=CARTESIAN_POINT('Ctrl Pts',(46.,52.7083333333333,-12.3256628518317));
#12543=CARTESIAN_POINT('Ctrl Pts',(46.,52.5,-5.63337527607782E-15));
#12544=CARTESIAN_POINT('Ctrl Pts',(46.,52.2916666666667,12.3256628518316));
#12545=CARTESIAN_POINT('Ctrl Pts',(39.8371685740842,52.0833333333333,23.));
#12546=CARTESIAN_POINT('Ctrl Pts',(33.6743371481684,51.875,33.6743371481683));
#12547=CARTESIAN_POINT('Ctrl Pts',(23.,51.6666666666667,39.8371685740842));
#12548=CARTESIAN_POINT('Ctrl Pts',(12.3256628518317,51.4583333333333,46.));
#12549=CARTESIAN_POINT('Ctrl Pts',(8.45006291411674E-15,51.25,46.));
#12550=CARTESIAN_POINT('Ctrl Pts',(-12.3256628518316,51.0416666666667,46.));
#12551=CARTESIAN_POINT('Ctrl Pts',(-23.,50.8333333333333,39.8371685740842));
#12552=CARTESIAN_POINT('Ctrl Pts',(-33.6743371481683,50.625,33.6743371481684));
#12553=CARTESIAN_POINT('Ctrl Pts',(-39.8371685740842,50.4166666666667,23.));
#12554=CARTESIAN_POINT('Ctrl Pts',(-46.,50.2083333333333,12.3256628518317));
#12555=CARTESIAN_POINT('Ctrl Pts',(-46.,50.,0.));
#12556=CARTESIAN_POINT('Ctrl Pts',(-46.,49.7916666666667,-12.3256628518316));
#12557=CARTESIAN_POINT('Ctrl Pts',(-39.8371685740842,49.5833333333333,-23.));
#12558=CARTESIAN_POINT('Ctrl Pts',(-33.6743371481684,49.375,-33.6743371481684));
#12559=CARTESIAN_POINT('Ctrl Pts',(-23.,49.1666666666667,-39.8371685740842));
#12560=CARTESIAN_POINT('Ctrl Pts',(-12.3256628518317,48.9583333333333,-46.));
#12561=CARTESIAN_POINT('Ctrl Pts',(-2.81668763803891E-15,48.75,-46.));
#12562=CARTESIAN_POINT('Ctrl Pts',(12.3256628518316,48.5416666666667,-46.));
#12563=CARTESIAN_POINT('Ctrl Pts',(23.,48.3333333333333,-39.8371685740842));
#12564=CARTESIAN_POINT('Ctrl Pts',(33.6743371481683,48.125,-33.6743371481684));
#12565=CARTESIAN_POINT('Ctrl Pts',(39.8371685740842,47.9166666666667,-23.));
#12566=CARTESIAN_POINT('Ctrl Pts',(46.,47.7083333333333,-12.3256628518317));
#12567=CARTESIAN_POINT('Ctrl Pts',(46.,47.5,-5.63337527607782E-15));
#12568=CARTESIAN_POINT('Ctrl Pts',(46.,47.2916666666667,12.3256628518316));
#12569=CARTESIAN_POINT('Ctrl Pts',(39.8371685740842,47.0833333333333,23.));
#12570=CARTESIAN_POINT('Ctrl Pts',(33.6743371481684,46.875,33.6743371481683));
#12571=CARTESIAN_POINT('Ctrl Pts',(23.,46.6666666666667,39.8371685740842));
#12572=CARTESIAN_POINT('Ctrl Pts',(12.3256628518317,46.4583333333333,46.));
#12573=CARTESIAN_POINT('Ctrl Pts',(8.45006291411674E-15,46.25,46.));
#12574=CARTESIAN_POINT('Ctrl Pts',(-12.3256628518316,46.0416666666667,46.));
#12575=CARTESIAN_POINT('Ctrl Pts',(-23.,45.8333333333333,39.8371685740842));
#12576=CARTESIAN_POINT('Ctrl Pts',(-33.6743371481683,45.625,33.6743371481684));
#12577=CARTESIAN_POINT('Ctrl Pts',(-39.8371685740842,45.4166666666667,23.));
#12578=CARTESIAN_POINT('Ctrl Pts',(-46.,45.2083333333333,12.3256628518317));
#12579=CARTESIAN_POINT('Ctrl Pts',(-46.,45.,0.));
#12580=CARTESIAN_POINT('Ctrl Pts',(-46.,44.7916666666667,-12.3256628518316));
#12581=CARTESIAN_POINT('Ctrl Pts',(-39.8371685740842,44.5833333333333,-23.));
#12582=CARTESIAN_POINT('Ctrl Pts',(-33.6743371481684,44.375,-33.6743371481684));
#12583=CARTESIAN_POINT('Ctrl Pts',(-23.,44.1666666666667,-39.8371685740842));
#12584=CARTESIAN_POINT('Ctrl Pts',(-12.3256628518317,43.9583333333333,-46.));
#12585=CARTESIAN_POINT('Ctrl Pts',(-2.81668763803891E-15,43.75,-46.));
#12586=CARTESIAN_POINT('Ctrl Pts',(12.3256628518316,43.5416666666667,-46.));
#12587=CARTESIAN_POINT('Ctrl Pts',(23.,43.3333333333333,-39.8371685740842));
#12588=CARTESIAN_POINT('Ctrl Pts',(33.6743371481683,43.125,-33.6743371481684));
#12589=CARTESIAN_POINT('Ctrl Pts',(39.8371685740842,42.9166666666667,-23.));
#12590=CARTESIAN_POINT('Ctrl Pts',(46.,42.7083333333333,-12.3256628518317));
#12591=CARTESIAN_POINT('Ctrl Pts',(46.,42.5,-5.63337527607782E-15));
#12592=CARTESIAN_POINT('Ctrl Pts',(46.,42.2916666666667,12.3256628518316));
#12593=CARTESIAN_POINT('Ctrl Pts',(39.8371685740842,42.0833333333333,23.));
#12594=CARTESIAN_POINT('Ctrl Pts',(33.6743371481684,41.875,33.6743371481683));
#12595=CARTESIAN_POINT('Ctrl Pts',(23.,41.6666666666667,39.8371685740842));
#12596=CARTESIAN_POINT('Ctrl Pts',(12.3256628518317,41.4583333333333,46.));
#12597=CARTESIAN_POINT('Ctrl Pts',(8.45006291411674E-15,41.25,46.));
#12598=CARTESIAN_POINT('Ctrl Pts',(-12.3256628518316,41.0416666666667,46.));
#12599=CARTESIAN_POINT('Ctrl Pts',(-23.,40.8333333333333,39.8371685740842));
#12600=CARTESIAN_POINT('Ctrl Pts',(-33.6743371481683,40.625,33.6743371481684));
#12601=CARTESIAN_POINT('Ctrl Pts',(-39.8371685740842,40.4166666666667,23.));
#12602=CARTESIAN_POINT('Ctrl Pts',(-46.,40.2083333333333,12.3256628518317));
#12603=CARTESIAN_POINT('Ctrl Pts',(-46.,40.,0.));
#12604=CARTESIAN_POINT('Ctrl Pts',(-46.,39.7916666666667,-12.3256628518316));
#12605=CARTESIAN_POINT('Ctrl Pts',(-39.8371685740842,39.5833333333333,-23.));
#12606=CARTESIAN_POINT('Ctrl Pts',(-33.6743371481684,39.375,-33.6743371481684));
#12607=CARTESIAN_POINT('Ctrl Pts',(-23.,39.1666666666667,-39.8371685740842));
#12608=CARTESIAN_POINT('Ctrl Pts',(-12.3256628518317,38.9583333333333,-46.));
#12609=CARTESIAN_POINT('Ctrl Pts',(-2.81668763803891E-15,38.75,-46.));
#12610=CARTESIAN_POINT('Ctrl Pts',(12.3256628518316,38.5416666666667,-46.));
#12611=CARTESIAN_POINT('Ctrl Pts',(23.,38.3333333333333,-39.8371685740842));
#12612=CARTESIAN_POINT('Ctrl Pts',(33.6743371481683,38.125,-33.6743371481684));
#12613=CARTESIAN_POINT('Ctrl Pts',(39.8371685740842,37.9166666666667,-23.));
#12614=CARTESIAN_POINT('Ctrl Pts',(46.,37.7083333333333,-12.3256628518317));
#12615=CARTESIAN_POINT('Ctrl Pts',(46.,37.5,-5.63337527607782E-15));
#12616=CARTESIAN_POINT('Ctrl Pts',(46.,37.2916666666667,12.3256628518316));
#12617=CARTESIAN_POINT('Ctrl Pts',(39.8371685740842,37.0833333333333,23.));
#12618=CARTESIAN_POINT('Ctrl Pts',(33.6743371481684,36.875,33.6743371481683));
#12619=CARTESIAN_POINT('Ctrl Pts',(23.,36.6666666666667,39.8371685740842));
#12620=CARTESIAN_POINT('Ctrl Pts',(12.3256628518317,36.4583333333333,46.));
#12621=CARTESIAN_POINT('Ctrl Pts',(8.45006291411674E-15,36.25,46.));
#12622=CARTESIAN_POINT('Ctrl Pts',(-12.3256628518316,36.0416666666667,46.));
#12623=CARTESIAN_POINT('Ctrl Pts',(-23.,35.8333333333333,39.8371685740842));
#12624=CARTESIAN_POINT('Ctrl Pts',(-33.6743371481683,35.625,33.6743371481684));
#12625=CARTESIAN_POINT('Ctrl Pts',(-39.8371685740842,35.4166666666667,23.));
#12626=CARTESIAN_POINT('Ctrl Pts',(-46.,35.2083333333333,12.3256628518317));
#12627=CARTESIAN_POINT('Ctrl Pts',(-46.,35.,0.));
#12628=CARTESIAN_POINT('Ctrl Pts',(-46.,34.7916666666667,-12.3256628518316));
#12629=CARTESIAN_POINT('Ctrl Pts',(-39.8371685740842,34.5833333333333,-23.));
#12630=CARTESIAN_POINT('Ctrl Pts',(-33.6743371481684,34.375,-33.6743371481684));
#12631=CARTESIAN_POINT('Ctrl Pts',(-23.,34.1666666666667,-39.8371685740842));
#12632=CARTESIAN_POINT('Ctrl Pts',(-12.3256628518317,33.9583333333333,-46.));
#12633=CARTESIAN_POINT('Ctrl Pts',(-2.81668763803891E-15,33.75,-46.));
#12634=CARTESIAN_POINT('Ctrl Pts',(12.3256628518316,33.5416666666667,-46.));
#12635=CARTESIAN_POINT('Ctrl Pts',(23.,33.3333333333333,-39.8371685740842));
#12636=CARTESIAN_POINT('Ctrl Pts',(33.6743371481683,33.125,-33.6743371481684));
#12637=CARTESIAN_POINT('Ctrl Pts',(39.8371685740842,32.9166666666667,-23.));
#12638=CARTESIAN_POINT('Ctrl Pts',(46.,32.7083333333333,-12.3256628518317));
#12639=CARTESIAN_POINT('Ctrl Pts',(46.,32.5,-5.63337527607782E-15));
#12640=CARTESIAN_POINT('Ctrl Pts',(46.,32.2916666666667,12.3256628518316));
#12641=CARTESIAN_POINT('Ctrl Pts',(39.8371685740842,32.0833333333333,23.));
#12642=CARTESIAN_POINT('Ctrl Pts',(33.6743371481684,31.875,33.6743371481683));
#12643=CARTESIAN_POINT('Ctrl Pts',(23.,31.6666666666667,39.8371685740842));
#12644=CARTESIAN_POINT('Ctrl Pts',(12.3256628518317,31.4583333333333,46.));
#12645=CARTESIAN_POINT('Ctrl Pts',(8.45006291411674E-15,31.25,46.));
#12646=CARTESIAN_POINT('Ctrl Pts',(-12.3256628518316,31.0416666666667,46.));
#12647=CARTESIAN_POINT('Ctrl Pts',(-23.,30.8333333333333,39.8371685740842));
#12648=CARTESIAN_POINT('Ctrl Pts',(-33.6743371481683,30.625,33.6743371481684));
#12649=CARTESIAN_POINT('Ctrl Pts',(-39.8371685740842,30.4166666666667,23.));
#12650=CARTESIAN_POINT('Ctrl Pts',(-46.,30.2083333333333,12.3256628518317));
#12651=CARTESIAN_POINT('Ctrl Pts',(-46.,30.,0.));
#12652=CARTESIAN_POINT('Ctrl Pts',(45.7957082162897,47.5741208584476,-4.33048599679672));
#12653=CARTESIAN_POINT('Ctrl Pts',(46.027322302781,47.4406160752063,-4.33048599679672));
#12654=CARTESIAN_POINT('Ctrl Pts',(46.4905476657728,47.1736016336912,-4.33048599679667));
#12655=CARTESIAN_POINT('Ctrl Pts',(46.9537676533565,46.9065778670208,-4.33048599679672));
#12656=CARTESIAN_POINT('Ctrl Pts',(47.6280672732221,46.5178683162597,-4.33048599679672));
#12657=CARTESIAN_POINT('Ctrl Pts',(48.0707534890442,46.2626647328764,-4.33048599679671));
#12658=CARTESIAN_POINT('Ctrl Pts',(48.5134353784344,46.0074536451604,-4.33048599679671));
#12659=CARTESIAN_POINT('Ctrl Pts',(3.61292728433799,47.1292520480092,-48.5721450795008));
#12660=CARTESIAN_POINT('Ctrl Pts',(3.61292728433799,47.2624339185675,-48.3403451622817));
#12661=CARTESIAN_POINT('Ctrl Pts',(3.612927284338,47.395608829009,-48.1085412459393));
#12662=CARTESIAN_POINT('Ctrl Pts',(3.612927284338,47.6619441142016,-47.6449250631479));
#12663=CARTESIAN_POINT('Ctrl Pts',(3.61292728433804,47.7951044891727,-47.4131127965212));
#12664=CARTESIAN_POINT('Ctrl Pts',(3.61292728433804,47.9282572703914,-47.1812961682826));
#12665=CARTESIAN_POINT('Ctrl Pts',(3.61292728433804,48.1816295626638,-46.7401795055578));
#12666=CARTESIAN_POINT('Ctrl Pts',(3.61292728433796,48.4349743764897,-46.2990470581854));
#12667=CARTESIAN_POINT('Ctrl Pts',(3.61292728433796,48.688289262853,-45.8578974271399));
#12668=CARTESIAN_POINT('Ctrl Pts',(-48.706329375,58.437500006828,-1.8898197019151E-14));
#12669=CARTESIAN_POINT('Ctrl Pts',(-48.706329375,58.2291666734946,-13.0508216223155));
#12670=CARTESIAN_POINT('Ctrl Pts',(-42.1809185638422,58.0208333401613,-24.3531646875));
#12671=CARTESIAN_POINT('Ctrl Pts',(-35.6555077526845,57.812500006828,-35.6555077526845));
#12672=CARTESIAN_POINT('Ctrl Pts',(-24.3531646875,57.6041666734946,-42.1809185638422));
#12673=CARTESIAN_POINT('Ctrl Pts',(-13.0508216223155,57.3958333401613,-48.706329375));
#12674=CARTESIAN_POINT('Ctrl Pts',(1.59157945007855E-14,57.187500006828,
-48.706329375));
#12675=CARTESIAN_POINT('Ctrl Pts',(13.0508216223155,56.9791666734946,-48.706329375));
#12676=CARTESIAN_POINT('Ctrl Pts',(24.3531646875,56.7708333401613,-42.1809185638422));
#12677=CARTESIAN_POINT('Ctrl Pts',(35.6555077526845,56.562500006828,-35.6555077526845));
#12678=CARTESIAN_POINT('Ctrl Pts',(42.1809185638422,56.3541666734946,-24.3531646875));
#12679=CARTESIAN_POINT('Ctrl Pts',(48.706329375,56.1458333401613,-13.0508216223155));
#12680=CARTESIAN_POINT('Ctrl Pts',(48.706329375,55.937500006828,1.293339198242E-14));
#12681=CARTESIAN_POINT('Ctrl Pts',(48.706329375,55.7291666734946,13.0508216223155));
#12682=CARTESIAN_POINT('Ctrl Pts',(42.1809185638422,55.5208333401613,24.3531646875));
#12683=CARTESIAN_POINT('Ctrl Pts',(35.6555077526845,55.312500006828,35.6555077526845));
#12684=CARTESIAN_POINT('Ctrl Pts',(24.3531646875,55.1041666734946,42.1809185638422));
#12685=CARTESIAN_POINT('Ctrl Pts',(13.0508216223155,54.8958333401613,48.706329375));
#12686=CARTESIAN_POINT('Ctrl Pts',(-9.95098946405443E-15,54.687500006828,
48.706329375));
#12687=CARTESIAN_POINT('Ctrl Pts',(-13.0508216223155,54.4791666734946,48.706329375));
#12688=CARTESIAN_POINT('Ctrl Pts',(-24.3531646875,54.2708333401613,42.1809185638423));
#12689=CARTESIAN_POINT('Ctrl Pts',(-35.6555077526845,54.062500006828,35.6555077526845));
#12690=CARTESIAN_POINT('Ctrl Pts',(-42.1809185638422,53.8541666734946,24.3531646875));
#12691=CARTESIAN_POINT('Ctrl Pts',(-48.706329375,53.6458333401613,13.0508216223155));
#12692=CARTESIAN_POINT('Ctrl Pts',(-48.706329375,53.437500006828,-1.8898197019151E-14));
#12693=CARTESIAN_POINT('Ctrl Pts',(-48.706329375,53.2291666734946,-13.0508216223155));
#12694=CARTESIAN_POINT('Ctrl Pts',(-42.1809185638422,53.0208333401613,-24.3531646875));
#12695=CARTESIAN_POINT('Ctrl Pts',(-35.6555077526845,52.812500006828,-35.6555077526845));
#12696=CARTESIAN_POINT('Ctrl Pts',(-24.3531646875,52.6041666734946,-42.1809185638422));
#12697=CARTESIAN_POINT('Ctrl Pts',(-13.0508216223155,52.3958333401613,-48.706329375));
#12698=CARTESIAN_POINT('Ctrl Pts',(1.59157945007855E-14,52.187500006828,
-48.706329375));
#12699=CARTESIAN_POINT('Ctrl Pts',(13.0508216223155,51.9791666734946,-48.706329375));
#12700=CARTESIAN_POINT('Ctrl Pts',(24.3531646875,51.7708333401613,-42.1809185638422));
#12701=CARTESIAN_POINT('Ctrl Pts',(35.6555077526845,51.562500006828,-35.6555077526845));
#12702=CARTESIAN_POINT('Ctrl Pts',(42.1809185638422,51.3541666734946,-24.3531646875));
#12703=CARTESIAN_POINT('Ctrl Pts',(48.706329375,51.1458333401613,-13.0508216223155));
#12704=CARTESIAN_POINT('Ctrl Pts',(48.706329375,50.937500006828,1.293339198242E-14));
#12705=CARTESIAN_POINT('Ctrl Pts',(48.706329375,50.7291666734946,13.0508216223155));
#12706=CARTESIAN_POINT('Ctrl Pts',(42.1809185638422,50.5208333401613,24.3531646875));
#12707=CARTESIAN_POINT('Ctrl Pts',(35.6555077526845,50.312500006828,35.6555077526845));
#12708=CARTESIAN_POINT('Ctrl Pts',(24.3531646875,50.1041666734946,42.1809185638422));
#12709=CARTESIAN_POINT('Ctrl Pts',(13.0508216223155,49.8958333401613,48.706329375));
#12710=CARTESIAN_POINT('Ctrl Pts',(-9.95098946405443E-15,49.687500006828,
48.706329375));
#12711=CARTESIAN_POINT('Ctrl Pts',(-13.0508216223155,49.4791666734946,48.706329375));
#12712=CARTESIAN_POINT('Ctrl Pts',(-24.3531646875,49.2708333401613,42.1809185638423));
#12713=CARTESIAN_POINT('Ctrl Pts',(-35.6555077526845,49.062500006828,35.6555077526845));
#12714=CARTESIAN_POINT('Ctrl Pts',(-42.1809185638422,48.8541666734946,24.3531646875));
#12715=CARTESIAN_POINT('Ctrl Pts',(-48.706329375,48.6458333401613,13.0508216223155));
#12716=CARTESIAN_POINT('Ctrl Pts',(-48.706329375,48.437500006828,-1.8898197019151E-14));
#12717=CARTESIAN_POINT('Ctrl Pts',(-48.706329375,48.2291666734946,-13.0508216223155));
#12718=CARTESIAN_POINT('Ctrl Pts',(-42.1809185638422,48.0208333401613,-24.3531646875));
#12719=CARTESIAN_POINT('Ctrl Pts',(-35.6555077526845,47.812500006828,-35.6555077526845));
#12720=CARTESIAN_POINT('Ctrl Pts',(-24.3531646875,47.6041666734946,-42.1809185638422));
#12721=CARTESIAN_POINT('Ctrl Pts',(-13.0508216223155,47.3958333401613,-48.706329375));
#12722=CARTESIAN_POINT('Ctrl Pts',(1.59157945007855E-14,47.187500006828,
-48.706329375));
#12723=CARTESIAN_POINT('Ctrl Pts',(13.0508216223155,46.9791666734946,-48.706329375));
#12724=CARTESIAN_POINT('Ctrl Pts',(24.3531646875,46.7708333401613,-42.1809185638422));
#12725=CARTESIAN_POINT('Ctrl Pts',(35.6555077526845,46.562500006828,-35.6555077526845));
#12726=CARTESIAN_POINT('Ctrl Pts',(42.1809185638422,46.3541666734946,-24.3531646875));
#12727=CARTESIAN_POINT('Ctrl Pts',(48.706329375,46.1458333401613,-13.0508216223155));
#12728=CARTESIAN_POINT('Ctrl Pts',(48.706329375,45.937500006828,1.293339198242E-14));
#12729=CARTESIAN_POINT('Ctrl Pts',(48.706329375,45.7291666734946,13.0508216223155));
#12730=CARTESIAN_POINT('Ctrl Pts',(42.1809185638422,45.5208333401613,24.3531646875));
#12731=CARTESIAN_POINT('Ctrl Pts',(35.6555077526845,45.312500006828,35.6555077526845));
#12732=CARTESIAN_POINT('Ctrl Pts',(24.3531646875,45.1041666734946,42.1809185638422));
#12733=CARTESIAN_POINT('Ctrl Pts',(13.0508216223155,44.8958333401613,48.706329375));
#12734=CARTESIAN_POINT('Ctrl Pts',(-9.95098946405443E-15,44.687500006828,
48.706329375));
#12735=CARTESIAN_POINT('Ctrl Pts',(-13.0508216223155,44.4791666734946,48.706329375));
#12736=CARTESIAN_POINT('Ctrl Pts',(-24.3531646875,44.2708333401613,42.1809185638423));
#12737=CARTESIAN_POINT('Ctrl Pts',(-35.6555077526845,44.062500006828,35.6555077526845));
#12738=CARTESIAN_POINT('Ctrl Pts',(-42.1809185638422,43.8541666734946,24.3531646875));
#12739=CARTESIAN_POINT('Ctrl Pts',(-48.706329375,43.6458333401613,13.0508216223155));
#12740=CARTESIAN_POINT('Ctrl Pts',(-48.706329375,43.437500006828,-1.8898197019151E-14));
#12741=CARTESIAN_POINT('Ctrl Pts',(-48.706329375,43.2291666734946,-13.0508216223155));
#12742=CARTESIAN_POINT('Ctrl Pts',(-42.1809185638422,43.0208333401613,-24.3531646875));
#12743=CARTESIAN_POINT('Ctrl Pts',(-35.6555077526845,42.812500006828,-35.6555077526845));
#12744=CARTESIAN_POINT('Ctrl Pts',(-24.3531646875,42.6041666734946,-42.1809185638422));
#12745=CARTESIAN_POINT('Ctrl Pts',(-13.0508216223155,42.3958333401613,-48.706329375));
#12746=CARTESIAN_POINT('Ctrl Pts',(1.59157945007855E-14,42.187500006828,
-48.706329375));
#12747=CARTESIAN_POINT('Ctrl Pts',(13.0508216223155,41.9791666734946,-48.706329375));
#12748=CARTESIAN_POINT('Ctrl Pts',(24.3531646875,41.7708333401613,-42.1809185638422));
#12749=CARTESIAN_POINT('Ctrl Pts',(35.6555077526845,41.562500006828,-35.6555077526845));
#12750=CARTESIAN_POINT('Ctrl Pts',(42.1809185638422,41.3541666734946,-24.3531646875));
#12751=CARTESIAN_POINT('Ctrl Pts',(48.706329375,41.1458333401613,-13.0508216223155));
#12752=CARTESIAN_POINT('Ctrl Pts',(48.706329375,40.937500006828,1.293339198242E-14));
#12753=CARTESIAN_POINT('Ctrl Pts',(48.706329375,40.7291666734946,13.0508216223155));
#12754=CARTESIAN_POINT('Ctrl Pts',(42.1809185638422,40.5208333401613,24.3531646875));
#12755=CARTESIAN_POINT('Ctrl Pts',(35.6555077526845,40.312500006828,35.6555077526845));
#12756=CARTESIAN_POINT('Ctrl Pts',(24.3531646875,40.1041666734946,42.1809185638422));
#12757=CARTESIAN_POINT('Ctrl Pts',(13.0508216223155,39.8958333401613,48.706329375));
#12758=CARTESIAN_POINT('Ctrl Pts',(-9.95098946405443E-15,39.687500006828,
48.706329375));
#12759=CARTESIAN_POINT('Ctrl Pts',(-13.0508216223155,39.4791666734946,48.706329375));
#12760=CARTESIAN_POINT('Ctrl Pts',(-24.3531646875,39.2708333401613,42.1809185638423));
#12761=CARTESIAN_POINT('Ctrl Pts',(-35.6555077526845,39.062500006828,35.6555077526845));
#12762=CARTESIAN_POINT('Ctrl Pts',(-42.1809185638422,38.8541666734946,24.3531646875));
#12763=CARTESIAN_POINT('Ctrl Pts',(-48.706329375,38.6458333401613,13.0508216223155));
#12764=CARTESIAN_POINT('Ctrl Pts',(-48.706329375,38.437500006828,-1.8898197019151E-14));
#12765=CARTESIAN_POINT('Ctrl Pts',(-48.706329375,38.2291666734946,-13.0508216223155));
#12766=CARTESIAN_POINT('Ctrl Pts',(-42.1809185638422,38.0208333401613,-24.3531646875));
#12767=CARTESIAN_POINT('Ctrl Pts',(-35.6555077526845,37.812500006828,-35.6555077526845));
#12768=CARTESIAN_POINT('Ctrl Pts',(-24.3531646875,37.6041666734946,-42.1809185638422));
#12769=CARTESIAN_POINT('Ctrl Pts',(-13.0508216223155,37.3958333401613,-48.706329375));
#12770=CARTESIAN_POINT('Ctrl Pts',(1.59157945007855E-14,37.187500006828,
-48.706329375));
#12771=CARTESIAN_POINT('Ctrl Pts',(13.0508216223155,36.9791666734946,-48.706329375));
#12772=CARTESIAN_POINT('Ctrl Pts',(24.3531646875,36.7708333401613,-42.1809185638422));
#12773=CARTESIAN_POINT('Ctrl Pts',(35.6555077526845,36.562500006828,-35.6555077526845));
#12774=CARTESIAN_POINT('Ctrl Pts',(42.1809185638422,36.3541666734946,-24.3531646875));
#12775=CARTESIAN_POINT('Ctrl Pts',(48.706329375,36.1458333401613,-13.0508216223155));
#12776=CARTESIAN_POINT('Ctrl Pts',(48.706329375,35.937500006828,1.293339198242E-14));
#12777=CARTESIAN_POINT('Ctrl Pts',(48.706329375,35.7291666734946,13.0508216223155));
#12778=CARTESIAN_POINT('Ctrl Pts',(42.1809185638422,35.5208333401613,24.3531646875));
#12779=CARTESIAN_POINT('Ctrl Pts',(35.6555077526845,35.312500006828,35.6555077526845));
#12780=CARTESIAN_POINT('Ctrl Pts',(24.3531646875,35.1041666734946,42.1809185638422));
#12781=CARTESIAN_POINT('Ctrl Pts',(13.0508216223155,34.8958333401613,48.706329375));
#12782=CARTESIAN_POINT('Ctrl Pts',(-9.95098946405443E-15,34.687500006828,
48.706329375));
#12783=CARTESIAN_POINT('Ctrl Pts',(-13.0508216223155,34.4791666734946,48.706329375));
#12784=CARTESIAN_POINT('Ctrl Pts',(-24.3531646875,34.2708333401613,42.1809185638423));
#12785=CARTESIAN_POINT('Ctrl Pts',(-35.6555077526845,34.062500006828,35.6555077526845));
#12786=CARTESIAN_POINT('Ctrl Pts',(-42.1809185638422,33.8541666734946,24.3531646875));
#12787=CARTESIAN_POINT('Ctrl Pts',(-48.706329375,33.6458333401613,13.0508216223155));
#12788=CARTESIAN_POINT('Ctrl Pts',(-48.706329375,33.437500006828,-1.8898197019151E-14));
#12789=CARTESIAN_POINT('Ctrl Pts',(-48.706329375,33.2291666734946,-13.0508216223155));
#12790=CARTESIAN_POINT('Ctrl Pts',(-42.1809185638422,33.0208333401613,-24.3531646875));
#12791=CARTESIAN_POINT('Ctrl Pts',(-35.6555077526845,32.812500006828,-35.6555077526845));
#12792=CARTESIAN_POINT('Ctrl Pts',(-24.3531646875,32.6041666734946,-42.1809185638422));
#12793=CARTESIAN_POINT('Ctrl Pts',(-13.0508216223155,32.3958333401613,-48.706329375));
#12794=CARTESIAN_POINT('Ctrl Pts',(1.59157945007855E-14,32.187500006828,
-48.706329375));
#12795=CARTESIAN_POINT('Ctrl Pts',(13.0508216223155,31.9791666734946,-48.706329375));
#12796=CARTESIAN_POINT('Ctrl Pts',(24.3531646875,31.7708333401613,-42.1809185638422));
#12797=CARTESIAN_POINT('Ctrl Pts',(35.6555077526845,31.562500006828,-35.6555077526845));
#12798=CARTESIAN_POINT('Ctrl Pts',(42.1809185638422,31.3541666734946,-24.3531646875));
#12799=CARTESIAN_POINT('Ctrl Pts',(48.706329375,31.1458333401613,-13.0508216223155));
#12800=CARTESIAN_POINT('Ctrl Pts',(48.706329375,30.937500006828,1.293339198242E-14));
#12801=CARTESIAN_POINT('Ctrl Pts',(48.706329375,30.7291666734946,13.0508216223155));
#12802=CARTESIAN_POINT('Ctrl Pts',(42.1809185638422,30.5208333401613,24.3531646875));
#12803=CARTESIAN_POINT('Ctrl Pts',(35.6555077526845,30.312500006828,35.6555077526845));
#12804=CARTESIAN_POINT('Ctrl Pts',(24.3531646875,30.1041666734946,42.1809185638422));
#12805=CARTESIAN_POINT('Ctrl Pts',(13.0508216223155,29.8958333401613,48.706329375));
#12806=CARTESIAN_POINT('Ctrl Pts',(-9.95098946405443E-15,29.687500006828,
48.706329375));
#12807=CARTESIAN_POINT('Ctrl Pts',(-13.0508216223155,29.4791666734946,48.706329375));
#12808=CARTESIAN_POINT('Ctrl Pts',(-24.3531646875,29.2708333401613,42.1809185638423));
#12809=CARTESIAN_POINT('Ctrl Pts',(-35.6555077526845,29.062500006828,35.6555077526845));
#12810=CARTESIAN_POINT('Ctrl Pts',(-42.1809185638422,28.8541666734946,24.3531646875));
#12811=CARTESIAN_POINT('Ctrl Pts',(-48.706329375,28.6458333401613,13.0508216223155));
#12812=CARTESIAN_POINT('Ctrl Pts',(-48.706329375,28.437500006828,-1.8898197019151E-14));
#12813=CARTESIAN_POINT('Ctrl Pts',(-46.,60.,0.));
#12814=CARTESIAN_POINT('Ctrl Pts',(-46.,59.7916666666667,-12.3256628518316));
#12815=CARTESIAN_POINT('Ctrl Pts',(-39.8371685740842,59.5833333333333,-23.));
#12816=CARTESIAN_POINT('Ctrl Pts',(-33.6743371481684,59.375,-33.6743371481684));
#12817=CARTESIAN_POINT('Ctrl Pts',(-23.,59.1666666666667,-39.8371685740842));
#12818=CARTESIAN_POINT('Ctrl Pts',(-12.3256628518317,58.9583333333333,-46.));
#12819=CARTESIAN_POINT('Ctrl Pts',(-2.81668763803891E-15,58.75,-46.));
#12820=CARTESIAN_POINT('Ctrl Pts',(12.3256628518316,58.5416666666667,-46.));
#12821=CARTESIAN_POINT('Ctrl Pts',(23.,58.3333333333333,-39.8371685740842));
#12822=CARTESIAN_POINT('Ctrl Pts',(33.6743371481683,58.125,-33.6743371481684));
#12823=CARTESIAN_POINT('Ctrl Pts',(39.8371685740842,57.9166666666667,-23.));
#12824=CARTESIAN_POINT('Ctrl Pts',(46.,57.7083333333333,-12.3256628518317));
#12825=CARTESIAN_POINT('Ctrl Pts',(46.,57.5,-5.63337527607782E-15));
#12826=CARTESIAN_POINT('Ctrl Pts',(46.,57.2916666666667,12.3256628518316));
#12827=CARTESIAN_POINT('Ctrl Pts',(39.8371685740842,57.0833333333333,23.));
#12828=CARTESIAN_POINT('Ctrl Pts',(33.6743371481684,56.875,33.6743371481683));
#12829=CARTESIAN_POINT('Ctrl Pts',(23.,56.6666666666667,39.8371685740842));
#12830=CARTESIAN_POINT('Ctrl Pts',(12.3256628518317,56.4583333333333,46.));
#12831=CARTESIAN_POINT('Ctrl Pts',(8.45006291411674E-15,56.25,46.));
#12832=CARTESIAN_POINT('Ctrl Pts',(-12.3256628518316,56.0416666666667,46.));
#12833=CARTESIAN_POINT('Ctrl Pts',(-23.,55.8333333333333,39.8371685740842));
#12834=CARTESIAN_POINT('Ctrl Pts',(-33.6743371481683,55.625,33.6743371481684));
#12835=CARTESIAN_POINT('Ctrl Pts',(-39.8371685740842,55.4166666666667,23.));
#12836=CARTESIAN_POINT('Ctrl Pts',(-46.,55.2083333333333,12.3256628518317));
#12837=CARTESIAN_POINT('Ctrl Pts',(-46.,55.,0.));
#12838=CARTESIAN_POINT('Ctrl Pts',(-46.,54.7916666666667,-12.3256628518316));
#12839=CARTESIAN_POINT('Ctrl Pts',(-39.8371685740842,54.5833333333333,-23.));
#12840=CARTESIAN_POINT('Ctrl Pts',(-33.6743371481684,54.375,-33.6743371481684));
#12841=CARTESIAN_POINT('Ctrl Pts',(-23.,54.1666666666667,-39.8371685740842));
#12842=CARTESIAN_POINT('Ctrl Pts',(-12.3256628518317,53.9583333333333,-46.));
#12843=CARTESIAN_POINT('Ctrl Pts',(-2.81668763803891E-15,53.75,-46.));
#12844=CARTESIAN_POINT('Ctrl Pts',(12.3256628518316,53.5416666666667,-46.));
#12845=CARTESIAN_POINT('Ctrl Pts',(23.,53.3333333333333,-39.8371685740842));
#12846=CARTESIAN_POINT('Ctrl Pts',(33.6743371481683,53.125,-33.6743371481684));
#12847=CARTESIAN_POINT('Ctrl Pts',(39.8371685740842,52.9166666666667,-23.));
#12848=CARTESIAN_POINT('Ctrl Pts',(46.,52.7083333333333,-12.3256628518317));
#12849=CARTESIAN_POINT('Ctrl Pts',(46.,52.5,-5.63337527607782E-15));
#12850=CARTESIAN_POINT('Ctrl Pts',(46.,52.2916666666667,12.3256628518316));
#12851=CARTESIAN_POINT('Ctrl Pts',(39.8371685740842,52.0833333333333,23.));
#12852=CARTESIAN_POINT('Ctrl Pts',(33.6743371481684,51.875,33.6743371481683));
#12853=CARTESIAN_POINT('Ctrl Pts',(23.,51.6666666666667,39.8371685740842));
#12854=CARTESIAN_POINT('Ctrl Pts',(12.3256628518317,51.4583333333333,46.));
#12855=CARTESIAN_POINT('Ctrl Pts',(8.45006291411674E-15,51.25,46.));
#12856=CARTESIAN_POINT('Ctrl Pts',(-12.3256628518316,51.0416666666667,46.));
#12857=CARTESIAN_POINT('Ctrl Pts',(-23.,50.8333333333333,39.8371685740842));
#12858=CARTESIAN_POINT('Ctrl Pts',(-33.6743371481683,50.625,33.6743371481684));
#12859=CARTESIAN_POINT('Ctrl Pts',(-39.8371685740842,50.4166666666667,23.));
#12860=CARTESIAN_POINT('Ctrl Pts',(-46.,50.2083333333333,12.3256628518317));
#12861=CARTESIAN_POINT('Ctrl Pts',(-46.,50.,0.));
#12862=CARTESIAN_POINT('Ctrl Pts',(-46.,49.7916666666667,-12.3256628518316));
#12863=CARTESIAN_POINT('Ctrl Pts',(-39.8371685740842,49.5833333333333,-23.));
#12864=CARTESIAN_POINT('Ctrl Pts',(-33.6743371481684,49.375,-33.6743371481684));
#12865=CARTESIAN_POINT('Ctrl Pts',(-23.,49.1666666666667,-39.8371685740842));
#12866=CARTESIAN_POINT('Ctrl Pts',(-12.3256628518317,48.9583333333333,-46.));
#12867=CARTESIAN_POINT('Ctrl Pts',(-2.81668763803891E-15,48.75,-46.));
#12868=CARTESIAN_POINT('Ctrl Pts',(12.3256628518316,48.5416666666667,-46.));
#12869=CARTESIAN_POINT('Ctrl Pts',(23.,48.3333333333333,-39.8371685740842));
#12870=CARTESIAN_POINT('Ctrl Pts',(33.6743371481683,48.125,-33.6743371481684));
#12871=CARTESIAN_POINT('Ctrl Pts',(39.8371685740842,47.9166666666667,-23.));
#12872=CARTESIAN_POINT('Ctrl Pts',(46.,47.7083333333333,-12.3256628518317));
#12873=CARTESIAN_POINT('Ctrl Pts',(46.,47.5,-5.63337527607782E-15));
#12874=CARTESIAN_POINT('Ctrl Pts',(46.,47.2916666666667,12.3256628518316));
#12875=CARTESIAN_POINT('Ctrl Pts',(39.8371685740842,47.0833333333333,23.));
#12876=CARTESIAN_POINT('Ctrl Pts',(33.6743371481684,46.875,33.6743371481683));
#12877=CARTESIAN_POINT('Ctrl Pts',(23.,46.6666666666667,39.8371685740842));
#12878=CARTESIAN_POINT('Ctrl Pts',(12.3256628518317,46.4583333333333,46.));
#12879=CARTESIAN_POINT('Ctrl Pts',(8.45006291411674E-15,46.25,46.));
#12880=CARTESIAN_POINT('Ctrl Pts',(-12.3256628518316,46.0416666666667,46.));
#12881=CARTESIAN_POINT('Ctrl Pts',(-23.,45.8333333333333,39.8371685740842));
#12882=CARTESIAN_POINT('Ctrl Pts',(-33.6743371481683,45.625,33.6743371481684));
#12883=CARTESIAN_POINT('Ctrl Pts',(-39.8371685740842,45.4166666666667,23.));
#12884=CARTESIAN_POINT('Ctrl Pts',(-46.,45.2083333333333,12.3256628518317));
#12885=CARTESIAN_POINT('Ctrl Pts',(-46.,45.,0.));
#12886=CARTESIAN_POINT('Ctrl Pts',(-46.,44.7916666666667,-12.3256628518316));
#12887=CARTESIAN_POINT('Ctrl Pts',(-39.8371685740842,44.5833333333333,-23.));
#12888=CARTESIAN_POINT('Ctrl Pts',(-33.6743371481684,44.375,-33.6743371481684));
#12889=CARTESIAN_POINT('Ctrl Pts',(-23.,44.1666666666667,-39.8371685740842));
#12890=CARTESIAN_POINT('Ctrl Pts',(-12.3256628518317,43.9583333333333,-46.));
#12891=CARTESIAN_POINT('Ctrl Pts',(-2.81668763803891E-15,43.75,-46.));
#12892=CARTESIAN_POINT('Ctrl Pts',(12.3256628518316,43.5416666666667,-46.));
#12893=CARTESIAN_POINT('Ctrl Pts',(23.,43.3333333333333,-39.8371685740842));
#12894=CARTESIAN_POINT('Ctrl Pts',(33.6743371481683,43.125,-33.6743371481684));
#12895=CARTESIAN_POINT('Ctrl Pts',(39.8371685740842,42.9166666666667,-23.));
#12896=CARTESIAN_POINT('Ctrl Pts',(46.,42.7083333333333,-12.3256628518317));
#12897=CARTESIAN_POINT('Ctrl Pts',(46.,42.5,-5.63337527607782E-15));
#12898=CARTESIAN_POINT('Ctrl Pts',(46.,42.2916666666667,12.3256628518316));
#12899=CARTESIAN_POINT('Ctrl Pts',(39.8371685740842,42.0833333333333,23.));
#12900=CARTESIAN_POINT('Ctrl Pts',(33.6743371481684,41.875,33.6743371481683));
#12901=CARTESIAN_POINT('Ctrl Pts',(23.,41.6666666666667,39.8371685740842));
#12902=CARTESIAN_POINT('Ctrl Pts',(12.3256628518317,41.4583333333333,46.));
#12903=CARTESIAN_POINT('Ctrl Pts',(8.45006291411674E-15,41.25,46.));
#12904=CARTESIAN_POINT('Ctrl Pts',(-12.3256628518316,41.0416666666667,46.));
#12905=CARTESIAN_POINT('Ctrl Pts',(-23.,40.8333333333333,39.8371685740842));
#12906=CARTESIAN_POINT('Ctrl Pts',(-33.6743371481683,40.625,33.6743371481684));
#12907=CARTESIAN_POINT('Ctrl Pts',(-39.8371685740842,40.4166666666667,23.));
#12908=CARTESIAN_POINT('Ctrl Pts',(-46.,40.2083333333333,12.3256628518317));
#12909=CARTESIAN_POINT('Ctrl Pts',(-46.,40.,0.));
#12910=CARTESIAN_POINT('Ctrl Pts',(-46.,39.7916666666667,-12.3256628518316));
#12911=CARTESIAN_POINT('Ctrl Pts',(-39.8371685740842,39.5833333333333,-23.));
#12912=CARTESIAN_POINT('Ctrl Pts',(-33.6743371481684,39.375,-33.6743371481684));
#12913=CARTESIAN_POINT('Ctrl Pts',(-23.,39.1666666666667,-39.8371685740842));
#12914=CARTESIAN_POINT('Ctrl Pts',(-12.3256628518317,38.9583333333333,-46.));
#12915=CARTESIAN_POINT('Ctrl Pts',(-2.81668763803891E-15,38.75,-46.));
#12916=CARTESIAN_POINT('Ctrl Pts',(12.3256628518316,38.5416666666667,-46.));
#12917=CARTESIAN_POINT('Ctrl Pts',(23.,38.3333333333333,-39.8371685740842));
#12918=CARTESIAN_POINT('Ctrl Pts',(33.6743371481683,38.125,-33.6743371481684));
#12919=CARTESIAN_POINT('Ctrl Pts',(39.8371685740842,37.9166666666667,-23.));
#12920=CARTESIAN_POINT('Ctrl Pts',(46.,37.7083333333333,-12.3256628518317));
#12921=CARTESIAN_POINT('Ctrl Pts',(46.,37.5,-5.63337527607782E-15));
#12922=CARTESIAN_POINT('Ctrl Pts',(46.,37.2916666666667,12.3256628518316));
#12923=CARTESIAN_POINT('Ctrl Pts',(39.8371685740842,37.0833333333333,23.));
#12924=CARTESIAN_POINT('Ctrl Pts',(33.6743371481684,36.875,33.6743371481683));
#12925=CARTESIAN_POINT('Ctrl Pts',(23.,36.6666666666667,39.8371685740842));
#12926=CARTESIAN_POINT('Ctrl Pts',(12.3256628518317,36.4583333333333,46.));
#12927=CARTESIAN_POINT('Ctrl Pts',(8.45006291411674E-15,36.25,46.));
#12928=CARTESIAN_POINT('Ctrl Pts',(-12.3256628518316,36.0416666666667,46.));
#12929=CARTESIAN_POINT('Ctrl Pts',(-23.,35.8333333333333,39.8371685740842));
#12930=CARTESIAN_POINT('Ctrl Pts',(-33.6743371481683,35.625,33.6743371481684));
#12931=CARTESIAN_POINT('Ctrl Pts',(-39.8371685740842,35.4166666666667,23.));
#12932=CARTESIAN_POINT('Ctrl Pts',(-46.,35.2083333333333,12.3256628518317));
#12933=CARTESIAN_POINT('Ctrl Pts',(-46.,35.,0.));
#12934=CARTESIAN_POINT('Ctrl Pts',(-46.,34.7916666666667,-12.3256628518316));
#12935=CARTESIAN_POINT('Ctrl Pts',(-39.8371685740842,34.5833333333333,-23.));
#12936=CARTESIAN_POINT('Ctrl Pts',(-33.6743371481684,34.375,-33.6743371481684));
#12937=CARTESIAN_POINT('Ctrl Pts',(-23.,34.1666666666667,-39.8371685740842));
#12938=CARTESIAN_POINT('Ctrl Pts',(-12.3256628518317,33.9583333333333,-46.));
#12939=CARTESIAN_POINT('Ctrl Pts',(-2.81668763803891E-15,33.75,-46.));
#12940=CARTESIAN_POINT('Ctrl Pts',(12.3256628518316,33.5416666666667,-46.));
#12941=CARTESIAN_POINT('Ctrl Pts',(23.,33.3333333333333,-39.8371685740842));
#12942=CARTESIAN_POINT('Ctrl Pts',(33.6743371481683,33.125,-33.6743371481684));
#12943=CARTESIAN_POINT('Ctrl Pts',(39.8371685740842,32.9166666666667,-23.));
#12944=CARTESIAN_POINT('Ctrl Pts',(46.,32.7083333333333,-12.3256628518317));
#12945=CARTESIAN_POINT('Ctrl Pts',(46.,32.5,-5.63337527607782E-15));
#12946=CARTESIAN_POINT('Ctrl Pts',(46.,32.2916666666667,12.3256628518316));
#12947=CARTESIAN_POINT('Ctrl Pts',(39.8371685740842,32.0833333333333,23.));
#12948=CARTESIAN_POINT('Ctrl Pts',(33.6743371481684,31.875,33.6743371481683));
#12949=CARTESIAN_POINT('Ctrl Pts',(23.,31.6666666666667,39.8371685740842));
#12950=CARTESIAN_POINT('Ctrl Pts',(12.3256628518317,31.4583333333333,46.));
#12951=CARTESIAN_POINT('Ctrl Pts',(8.45006291411674E-15,31.25,46.));
#12952=CARTESIAN_POINT('Ctrl Pts',(-12.3256628518316,31.0416666666667,46.));
#12953=CARTESIAN_POINT('Ctrl Pts',(-23.,30.8333333333333,39.8371685740842));
#12954=CARTESIAN_POINT('Ctrl Pts',(-33.6743371481683,30.625,33.6743371481684));
#12955=CARTESIAN_POINT('Ctrl Pts',(-39.8371685740842,30.4166666666667,23.));
#12956=CARTESIAN_POINT('Ctrl Pts',(-46.,30.2083333333333,12.3256628518317));
#12957=CARTESIAN_POINT('Ctrl Pts',(-46.,30.,0.));
#12958=CARTESIAN_POINT('Ctrl Pts',(48.5725845633798,45.8793483229262,3.60701400320328));
#12959=CARTESIAN_POINT('Ctrl Pts',(48.3407853679392,46.0125314497137,3.60701400320328));
#12960=CARTESIAN_POINT('Ctrl Pts',(48.1089821836664,46.1457076343819,3.60701400320327));
#12961=CARTESIAN_POINT('Ctrl Pts',(47.6453674864979,46.4120455056142,3.60701400320327));
#12962=CARTESIAN_POINT('Ctrl Pts',(47.4135559734254,46.5452071923974,3.60701400320325));
#12963=CARTESIAN_POINT('Ctrl Pts',(47.1817401099609,46.6783613050641,3.60701400320325));
#12964=CARTESIAN_POINT('Ctrl Pts',(46.7406305897488,46.9317328641751,3.60701400320325));
#12965=CARTESIAN_POINT('Ctrl Pts',(46.2995053259033,47.1850770165971,3.60701400320324));
#12966=CARTESIAN_POINT('Ctrl Pts',(45.858362923034,47.438391319744,3.60701400320324));
#12967=CARTESIAN_POINT('Ctrl Pts',(3.61292728433799,46.311710737147,45.8578974271399));
#12968=CARTESIAN_POINT('Ctrl Pts',(3.61292728433798,46.178117727701,46.089460636719));
#12969=CARTESIAN_POINT('Ctrl Pts',(3.61292728433804,45.9109294856547,46.5525857733052));
#12970=CARTESIAN_POINT('Ctrl Pts',(3.61292728433797,45.6437369897944,47.0157084557285));
#12971=CARTESIAN_POINT('Ctrl Pts',(3.61292728433797,45.2553460757965,47.6888965792834));
#12972=CARTESIAN_POINT('Ctrl Pts',(3.61292728433797,45.0005487265709,48.1305218136162));
#12973=CARTESIAN_POINT('Ctrl Pts',(3.61292728433797,44.7457479656467,48.5721450795008));
#12974=CARTESIAN_POINT('Ctrl Pts',(-48.706329375,58.437500006828,-1.8898197019151E-14));
#12975=CARTESIAN_POINT('Ctrl Pts',(-48.706329375,58.2291666734946,-13.0508216223155));
#12976=CARTESIAN_POINT('Ctrl Pts',(-42.1809185638422,58.0208333401613,-24.3531646875));
#12977=CARTESIAN_POINT('Ctrl Pts',(-35.6555077526845,57.812500006828,-35.6555077526845));
#12978=CARTESIAN_POINT('Ctrl Pts',(-24.3531646875,57.6041666734946,-42.1809185638422));
#12979=CARTESIAN_POINT('Ctrl Pts',(-13.0508216223155,57.3958333401613,-48.706329375));
#12980=CARTESIAN_POINT('Ctrl Pts',(1.59157945007855E-14,57.187500006828,
-48.706329375));
#12981=CARTESIAN_POINT('Ctrl Pts',(13.0508216223155,56.9791666734946,-48.706329375));
#12982=CARTESIAN_POINT('Ctrl Pts',(24.3531646875,56.7708333401613,-42.1809185638422));
#12983=CARTESIAN_POINT('Ctrl Pts',(35.6555077526845,56.562500006828,-35.6555077526845));
#12984=CARTESIAN_POINT('Ctrl Pts',(42.1809185638422,56.3541666734946,-24.3531646875));
#12985=CARTESIAN_POINT('Ctrl Pts',(48.706329375,56.1458333401613,-13.0508216223155));
#12986=CARTESIAN_POINT('Ctrl Pts',(48.706329375,55.937500006828,1.293339198242E-14));
#12987=CARTESIAN_POINT('Ctrl Pts',(48.706329375,55.7291666734946,13.0508216223155));
#12988=CARTESIAN_POINT('Ctrl Pts',(42.1809185638422,55.5208333401613,24.3531646875));
#12989=CARTESIAN_POINT('Ctrl Pts',(35.6555077526845,55.312500006828,35.6555077526845));
#12990=CARTESIAN_POINT('Ctrl Pts',(24.3531646875,55.1041666734946,42.1809185638422));
#12991=CARTESIAN_POINT('Ctrl Pts',(13.0508216223155,54.8958333401613,48.706329375));
#12992=CARTESIAN_POINT('Ctrl Pts',(-9.95098946405443E-15,54.687500006828,
48.706329375));
#12993=CARTESIAN_POINT('Ctrl Pts',(-13.0508216223155,54.4791666734946,48.706329375));
#12994=CARTESIAN_POINT('Ctrl Pts',(-24.3531646875,54.2708333401613,42.1809185638423));
#12995=CARTESIAN_POINT('Ctrl Pts',(-35.6555077526845,54.062500006828,35.6555077526845));
#12996=CARTESIAN_POINT('Ctrl Pts',(-42.1809185638422,53.8541666734946,24.3531646875));
#12997=CARTESIAN_POINT('Ctrl Pts',(-48.706329375,53.6458333401613,13.0508216223155));
#12998=CARTESIAN_POINT('Ctrl Pts',(-48.706329375,53.437500006828,-1.8898197019151E-14));
#12999=CARTESIAN_POINT('Ctrl Pts',(-48.706329375,53.2291666734946,-13.0508216223155));
#13000=CARTESIAN_POINT('Ctrl Pts',(-42.1809185638422,53.0208333401613,-24.3531646875));
#13001=CARTESIAN_POINT('Ctrl Pts',(-35.6555077526845,52.812500006828,-35.6555077526845));
#13002=CARTESIAN_POINT('Ctrl Pts',(-24.3531646875,52.6041666734946,-42.1809185638422));
#13003=CARTESIAN_POINT('Ctrl Pts',(-13.0508216223155,52.3958333401613,-48.706329375));
#13004=CARTESIAN_POINT('Ctrl Pts',(1.59157945007855E-14,52.187500006828,
-48.706329375));
#13005=CARTESIAN_POINT('Ctrl Pts',(13.0508216223155,51.9791666734946,-48.706329375));
#13006=CARTESIAN_POINT('Ctrl Pts',(24.3531646875,51.7708333401613,-42.1809185638422));
#13007=CARTESIAN_POINT('Ctrl Pts',(35.6555077526845,51.562500006828,-35.6555077526845));
#13008=CARTESIAN_POINT('Ctrl Pts',(42.1809185638422,51.3541666734946,-24.3531646875));
#13009=CARTESIAN_POINT('Ctrl Pts',(48.706329375,51.1458333401613,-13.0508216223155));
#13010=CARTESIAN_POINT('Ctrl Pts',(48.706329375,50.937500006828,1.293339198242E-14));
#13011=CARTESIAN_POINT('Ctrl Pts',(48.706329375,50.7291666734946,13.0508216223155));
#13012=CARTESIAN_POINT('Ctrl Pts',(42.1809185638422,50.5208333401613,24.3531646875));
#13013=CARTESIAN_POINT('Ctrl Pts',(35.6555077526845,50.312500006828,35.6555077526845));
#13014=CARTESIAN_POINT('Ctrl Pts',(24.3531646875,50.1041666734946,42.1809185638422));
#13015=CARTESIAN_POINT('Ctrl Pts',(13.0508216223155,49.8958333401613,48.706329375));
#13016=CARTESIAN_POINT('Ctrl Pts',(-9.95098946405443E-15,49.687500006828,
48.706329375));
#13017=CARTESIAN_POINT('Ctrl Pts',(-13.0508216223155,49.4791666734946,48.706329375));
#13018=CARTESIAN_POINT('Ctrl Pts',(-24.3531646875,49.2708333401613,42.1809185638423));
#13019=CARTESIAN_POINT('Ctrl Pts',(-35.6555077526845,49.062500006828,35.6555077526845));
#13020=CARTESIAN_POINT('Ctrl Pts',(-42.1809185638422,48.8541666734946,24.3531646875));
#13021=CARTESIAN_POINT('Ctrl Pts',(-48.706329375,48.6458333401613,13.0508216223155));
#13022=CARTESIAN_POINT('Ctrl Pts',(-48.706329375,48.437500006828,-1.8898197019151E-14));
#13023=CARTESIAN_POINT('Ctrl Pts',(-48.706329375,48.2291666734946,-13.0508216223155));
#13024=CARTESIAN_POINT('Ctrl Pts',(-42.1809185638422,48.0208333401613,-24.3531646875));
#13025=CARTESIAN_POINT('Ctrl Pts',(-35.6555077526845,47.812500006828,-35.6555077526845));
#13026=CARTESIAN_POINT('Ctrl Pts',(-24.3531646875,47.6041666734946,-42.1809185638422));
#13027=CARTESIAN_POINT('Ctrl Pts',(-13.0508216223155,47.3958333401613,-48.706329375));
#13028=CARTESIAN_POINT('Ctrl Pts',(1.59157945007855E-14,47.187500006828,
-48.706329375));
#13029=CARTESIAN_POINT('Ctrl Pts',(13.0508216223155,46.9791666734946,-48.706329375));
#13030=CARTESIAN_POINT('Ctrl Pts',(24.3531646875,46.7708333401613,-42.1809185638422));
#13031=CARTESIAN_POINT('Ctrl Pts',(35.6555077526845,46.562500006828,-35.6555077526845));
#13032=CARTESIAN_POINT('Ctrl Pts',(42.1809185638422,46.3541666734946,-24.3531646875));
#13033=CARTESIAN_POINT('Ctrl Pts',(48.706329375,46.1458333401613,-13.0508216223155));
#13034=CARTESIAN_POINT('Ctrl Pts',(48.706329375,45.937500006828,1.293339198242E-14));
#13035=CARTESIAN_POINT('Ctrl Pts',(48.706329375,45.7291666734946,13.0508216223155));
#13036=CARTESIAN_POINT('Ctrl Pts',(42.1809185638422,45.5208333401613,24.3531646875));
#13037=CARTESIAN_POINT('Ctrl Pts',(35.6555077526845,45.312500006828,35.6555077526845));
#13038=CARTESIAN_POINT('Ctrl Pts',(24.3531646875,45.1041666734946,42.1809185638422));
#13039=CARTESIAN_POINT('Ctrl Pts',(13.0508216223155,44.8958333401613,48.706329375));
#13040=CARTESIAN_POINT('Ctrl Pts',(-9.95098946405443E-15,44.687500006828,
48.706329375));
#13041=CARTESIAN_POINT('Ctrl Pts',(-13.0508216223155,44.4791666734946,48.706329375));
#13042=CARTESIAN_POINT('Ctrl Pts',(-24.3531646875,44.2708333401613,42.1809185638423));
#13043=CARTESIAN_POINT('Ctrl Pts',(-35.6555077526845,44.062500006828,35.6555077526845));
#13044=CARTESIAN_POINT('Ctrl Pts',(-42.1809185638422,43.8541666734946,24.3531646875));
#13045=CARTESIAN_POINT('Ctrl Pts',(-48.706329375,43.6458333401613,13.0508216223155));
#13046=CARTESIAN_POINT('Ctrl Pts',(-48.706329375,43.437500006828,-1.8898197019151E-14));
#13047=CARTESIAN_POINT('Ctrl Pts',(-48.706329375,43.2291666734946,-13.0508216223155));
#13048=CARTESIAN_POINT('Ctrl Pts',(-42.1809185638422,43.0208333401613,-24.3531646875));
#13049=CARTESIAN_POINT('Ctrl Pts',(-35.6555077526845,42.812500006828,-35.6555077526845));
#13050=CARTESIAN_POINT('Ctrl Pts',(-24.3531646875,42.6041666734946,-42.1809185638422));
#13051=CARTESIAN_POINT('Ctrl Pts',(-13.0508216223155,42.3958333401613,-48.706329375));
#13052=CARTESIAN_POINT('Ctrl Pts',(1.59157945007855E-14,42.187500006828,
-48.706329375));
#13053=CARTESIAN_POINT('Ctrl Pts',(13.0508216223155,41.9791666734946,-48.706329375));
#13054=CARTESIAN_POINT('Ctrl Pts',(24.3531646875,41.7708333401613,-42.1809185638422));
#13055=CARTESIAN_POINT('Ctrl Pts',(35.6555077526845,41.562500006828,-35.6555077526845));
#13056=CARTESIAN_POINT('Ctrl Pts',(42.1809185638422,41.3541666734946,-24.3531646875));
#13057=CARTESIAN_POINT('Ctrl Pts',(48.706329375,41.1458333401613,-13.0508216223155));
#13058=CARTESIAN_POINT('Ctrl Pts',(48.706329375,40.937500006828,1.293339198242E-14));
#13059=CARTESIAN_POINT('Ctrl Pts',(48.706329375,40.7291666734946,13.0508216223155));
#13060=CARTESIAN_POINT('Ctrl Pts',(42.1809185638422,40.5208333401613,24.3531646875));
#13061=CARTESIAN_POINT('Ctrl Pts',(35.6555077526845,40.312500006828,35.6555077526845));
#13062=CARTESIAN_POINT('Ctrl Pts',(24.3531646875,40.1041666734946,42.1809185638422));
#13063=CARTESIAN_POINT('Ctrl Pts',(13.0508216223155,39.8958333401613,48.706329375));
#13064=CARTESIAN_POINT('Ctrl Pts',(-9.95098946405443E-15,39.687500006828,
48.706329375));
#13065=CARTESIAN_POINT('Ctrl Pts',(-13.0508216223155,39.4791666734946,48.706329375));
#13066=CARTESIAN_POINT('Ctrl Pts',(-24.3531646875,39.2708333401613,42.1809185638423));
#13067=CARTESIAN_POINT('Ctrl Pts',(-35.6555077526845,39.062500006828,35.6555077526845));
#13068=CARTESIAN_POINT('Ctrl Pts',(-42.1809185638422,38.8541666734946,24.3531646875));
#13069=CARTESIAN_POINT('Ctrl Pts',(-48.706329375,38.6458333401613,13.0508216223155));
#13070=CARTESIAN_POINT('Ctrl Pts',(-48.706329375,38.437500006828,-1.8898197019151E-14));
#13071=CARTESIAN_POINT('Ctrl Pts',(-48.706329375,38.2291666734946,-13.0508216223155));
#13072=CARTESIAN_POINT('Ctrl Pts',(-42.1809185638422,38.0208333401613,-24.3531646875));
#13073=CARTESIAN_POINT('Ctrl Pts',(-35.6555077526845,37.812500006828,-35.6555077526845));
#13074=CARTESIAN_POINT('Ctrl Pts',(-24.3531646875,37.6041666734946,-42.1809185638422));
#13075=CARTESIAN_POINT('Ctrl Pts',(-13.0508216223155,37.3958333401613,-48.706329375));
#13076=CARTESIAN_POINT('Ctrl Pts',(1.59157945007855E-14,37.187500006828,
-48.706329375));
#13077=CARTESIAN_POINT('Ctrl Pts',(13.0508216223155,36.9791666734946,-48.706329375));
#13078=CARTESIAN_POINT('Ctrl Pts',(24.3531646875,36.7708333401613,-42.1809185638422));
#13079=CARTESIAN_POINT('Ctrl Pts',(35.6555077526845,36.562500006828,-35.6555077526845));
#13080=CARTESIAN_POINT('Ctrl Pts',(42.1809185638422,36.3541666734946,-24.3531646875));
#13081=CARTESIAN_POINT('Ctrl Pts',(48.706329375,36.1458333401613,-13.0508216223155));
#13082=CARTESIAN_POINT('Ctrl Pts',(48.706329375,35.937500006828,1.293339198242E-14));
#13083=CARTESIAN_POINT('Ctrl Pts',(48.706329375,35.7291666734946,13.0508216223155));
#13084=CARTESIAN_POINT('Ctrl Pts',(42.1809185638422,35.5208333401613,24.3531646875));
#13085=CARTESIAN_POINT('Ctrl Pts',(35.6555077526845,35.312500006828,35.6555077526845));
#13086=CARTESIAN_POINT('Ctrl Pts',(24.3531646875,35.1041666734946,42.1809185638422));
#13087=CARTESIAN_POINT('Ctrl Pts',(13.0508216223155,34.8958333401613,48.706329375));
#13088=CARTESIAN_POINT('Ctrl Pts',(-9.95098946405443E-15,34.687500006828,
48.706329375));
#13089=CARTESIAN_POINT('Ctrl Pts',(-13.0508216223155,34.4791666734946,48.706329375));
#13090=CARTESIAN_POINT('Ctrl Pts',(-24.3531646875,34.2708333401613,42.1809185638423));
#13091=CARTESIAN_POINT('Ctrl Pts',(-35.6555077526845,34.062500006828,35.6555077526845));
#13092=CARTESIAN_POINT('Ctrl Pts',(-42.1809185638422,33.8541666734946,24.3531646875));
#13093=CARTESIAN_POINT('Ctrl Pts',(-48.706329375,33.6458333401613,13.0508216223155));
#13094=CARTESIAN_POINT('Ctrl Pts',(-48.706329375,33.437500006828,-1.8898197019151E-14));
#13095=CARTESIAN_POINT('Ctrl Pts',(-48.706329375,33.2291666734946,-13.0508216223155));
#13096=CARTESIAN_POINT('Ctrl Pts',(-42.1809185638422,33.0208333401613,-24.3531646875));
#13097=CARTESIAN_POINT('Ctrl Pts',(-35.6555077526845,32.812500006828,-35.6555077526845));
#13098=CARTESIAN_POINT('Ctrl Pts',(-24.3531646875,32.6041666734946,-42.1809185638422));
#13099=CARTESIAN_POINT('Ctrl Pts',(-13.0508216223155,32.3958333401613,-48.706329375));
#13100=CARTESIAN_POINT('Ctrl Pts',(1.59157945007855E-14,32.187500006828,
-48.706329375));
#13101=CARTESIAN_POINT('Ctrl Pts',(13.0508216223155,31.9791666734946,-48.706329375));
#13102=CARTESIAN_POINT('Ctrl Pts',(24.3531646875,31.7708333401613,-42.1809185638422));
#13103=CARTESIAN_POINT('Ctrl Pts',(35.6555077526845,31.562500006828,-35.6555077526845));
#13104=CARTESIAN_POINT('Ctrl Pts',(42.1809185638422,31.3541666734946,-24.3531646875));
#13105=CARTESIAN_POINT('Ctrl Pts',(48.706329375,31.1458333401613,-13.0508216223155));
#13106=CARTESIAN_POINT('Ctrl Pts',(48.706329375,30.937500006828,1.293339198242E-14));
#13107=CARTESIAN_POINT('Ctrl Pts',(48.706329375,30.7291666734946,13.0508216223155));
#13108=CARTESIAN_POINT('Ctrl Pts',(42.1809185638422,30.5208333401613,24.3531646875));
#13109=CARTESIAN_POINT('Ctrl Pts',(35.6555077526845,30.312500006828,35.6555077526845));
#13110=CARTESIAN_POINT('Ctrl Pts',(24.3531646875,30.1041666734946,42.1809185638422));
#13111=CARTESIAN_POINT('Ctrl Pts',(13.0508216223155,29.8958333401613,48.706329375));
#13112=CARTESIAN_POINT('Ctrl Pts',(-9.95098946405443E-15,29.687500006828,
48.706329375));
#13113=CARTESIAN_POINT('Ctrl Pts',(-13.0508216223155,29.4791666734946,48.706329375));
#13114=CARTESIAN_POINT('Ctrl Pts',(-24.3531646875,29.2708333401613,42.1809185638423));
#13115=CARTESIAN_POINT('Ctrl Pts',(-35.6555077526845,29.062500006828,35.6555077526845));
#13116=CARTESIAN_POINT('Ctrl Pts',(-42.1809185638422,28.8541666734946,24.3531646875));
#13117=CARTESIAN_POINT('Ctrl Pts',(-48.706329375,28.6458333401613,13.0508216223155));
#13118=CARTESIAN_POINT('Ctrl Pts',(-48.706329375,28.437500006828,-1.8898197019151E-14));
#13119=CARTESIAN_POINT('Ctrl Pts',(-46.,60.,0.));
#13120=CARTESIAN_POINT('Ctrl Pts',(-46.,59.7916666666667,-12.3256628518316));
#13121=CARTESIAN_POINT('Ctrl Pts',(-39.8371685740842,59.5833333333333,-23.));
#13122=CARTESIAN_POINT('Ctrl Pts',(-33.6743371481684,59.375,-33.6743371481684));
#13123=CARTESIAN_POINT('Ctrl Pts',(-23.,59.1666666666667,-39.8371685740842));
#13124=CARTESIAN_POINT('Ctrl Pts',(-12.3256628518317,58.9583333333333,-46.));
#13125=CARTESIAN_POINT('Ctrl Pts',(-2.81668763803891E-15,58.75,-46.));
#13126=CARTESIAN_POINT('Ctrl Pts',(12.3256628518316,58.5416666666667,-46.));
#13127=CARTESIAN_POINT('Ctrl Pts',(23.,58.3333333333333,-39.8371685740842));
#13128=CARTESIAN_POINT('Ctrl Pts',(33.6743371481683,58.125,-33.6743371481684));
#13129=CARTESIAN_POINT('Ctrl Pts',(39.8371685740842,57.9166666666667,-23.));
#13130=CARTESIAN_POINT('Ctrl Pts',(46.,57.7083333333333,-12.3256628518317));
#13131=CARTESIAN_POINT('Ctrl Pts',(46.,57.5,-5.63337527607782E-15));
#13132=CARTESIAN_POINT('Ctrl Pts',(46.,57.2916666666667,12.3256628518316));
#13133=CARTESIAN_POINT('Ctrl Pts',(39.8371685740842,57.0833333333333,23.));
#13134=CARTESIAN_POINT('Ctrl Pts',(33.6743371481684,56.875,33.6743371481683));
#13135=CARTESIAN_POINT('Ctrl Pts',(23.,56.6666666666667,39.8371685740842));
#13136=CARTESIAN_POINT('Ctrl Pts',(12.3256628518317,56.4583333333333,46.));
#13137=CARTESIAN_POINT('Ctrl Pts',(8.45006291411674E-15,56.25,46.));
#13138=CARTESIAN_POINT('Ctrl Pts',(-12.3256628518316,56.0416666666667,46.));
#13139=CARTESIAN_POINT('Ctrl Pts',(-23.,55.8333333333333,39.8371685740842));
#13140=CARTESIAN_POINT('Ctrl Pts',(-33.6743371481683,55.625,33.6743371481684));
#13141=CARTESIAN_POINT('Ctrl Pts',(-39.8371685740842,55.4166666666667,23.));
#13142=CARTESIAN_POINT('Ctrl Pts',(-46.,55.2083333333333,12.3256628518317));
#13143=CARTESIAN_POINT('Ctrl Pts',(-46.,55.,0.));
#13144=CARTESIAN_POINT('Ctrl Pts',(-46.,54.7916666666667,-12.3256628518316));
#13145=CARTESIAN_POINT('Ctrl Pts',(-39.8371685740842,54.5833333333333,-23.));
#13146=CARTESIAN_POINT('Ctrl Pts',(-33.6743371481684,54.375,-33.6743371481684));
#13147=CARTESIAN_POINT('Ctrl Pts',(-23.,54.1666666666667,-39.8371685740842));
#13148=CARTESIAN_POINT('Ctrl Pts',(-12.3256628518317,53.9583333333333,-46.));
#13149=CARTESIAN_POINT('Ctrl Pts',(-2.81668763803891E-15,53.75,-46.));
#13150=CARTESIAN_POINT('Ctrl Pts',(12.3256628518316,53.5416666666667,-46.));
#13151=CARTESIAN_POINT('Ctrl Pts',(23.,53.3333333333333,-39.8371685740842));
#13152=CARTESIAN_POINT('Ctrl Pts',(33.6743371481683,53.125,-33.6743371481684));
#13153=CARTESIAN_POINT('Ctrl Pts',(39.8371685740842,52.9166666666667,-23.));
#13154=CARTESIAN_POINT('Ctrl Pts',(46.,52.7083333333333,-12.3256628518317));
#13155=CARTESIAN_POINT('Ctrl Pts',(46.,52.5,-5.63337527607782E-15));
#13156=CARTESIAN_POINT('Ctrl Pts',(46.,52.2916666666667,12.3256628518316));
#13157=CARTESIAN_POINT('Ctrl Pts',(39.8371685740842,52.0833333333333,23.));
#13158=CARTESIAN_POINT('Ctrl Pts',(33.6743371481684,51.875,33.6743371481683));
#13159=CARTESIAN_POINT('Ctrl Pts',(23.,51.6666666666667,39.8371685740842));
#13160=CARTESIAN_POINT('Ctrl Pts',(12.3256628518317,51.4583333333333,46.));
#13161=CARTESIAN_POINT('Ctrl Pts',(8.45006291411674E-15,51.25,46.));
#13162=CARTESIAN_POINT('Ctrl Pts',(-12.3256628518316,51.0416666666667,46.));
#13163=CARTESIAN_POINT('Ctrl Pts',(-23.,50.8333333333333,39.8371685740842));
#13164=CARTESIAN_POINT('Ctrl Pts',(-33.6743371481683,50.625,33.6743371481684));
#13165=CARTESIAN_POINT('Ctrl Pts',(-39.8371685740842,50.4166666666667,23.));
#13166=CARTESIAN_POINT('Ctrl Pts',(-46.,50.2083333333333,12.3256628518317));
#13167=CARTESIAN_POINT('Ctrl Pts',(-46.,50.,0.));
#13168=CARTESIAN_POINT('Ctrl Pts',(-46.,49.7916666666667,-12.3256628518316));
#13169=CARTESIAN_POINT('Ctrl Pts',(-39.8371685740842,49.5833333333333,-23.));
#13170=CARTESIAN_POINT('Ctrl Pts',(-33.6743371481684,49.375,-33.6743371481684));
#13171=CARTESIAN_POINT('Ctrl Pts',(-23.,49.1666666666667,-39.8371685740842));
#13172=CARTESIAN_POINT('Ctrl Pts',(-12.3256628518317,48.9583333333333,-46.));
#13173=CARTESIAN_POINT('Ctrl Pts',(-2.81668763803891E-15,48.75,-46.));
#13174=CARTESIAN_POINT('Ctrl Pts',(12.3256628518316,48.5416666666667,-46.));
#13175=CARTESIAN_POINT('Ctrl Pts',(23.,48.3333333333333,-39.8371685740842));
#13176=CARTESIAN_POINT('Ctrl Pts',(33.6743371481683,48.125,-33.6743371481684));
#13177=CARTESIAN_POINT('Ctrl Pts',(39.8371685740842,47.9166666666667,-23.));
#13178=CARTESIAN_POINT('Ctrl Pts',(46.,47.7083333333333,-12.3256628518317));
#13179=CARTESIAN_POINT('Ctrl Pts',(46.,47.5,-5.63337527607782E-15));
#13180=CARTESIAN_POINT('Ctrl Pts',(46.,47.2916666666667,12.3256628518316));
#13181=CARTESIAN_POINT('Ctrl Pts',(39.8371685740842,47.0833333333333,23.));
#13182=CARTESIAN_POINT('Ctrl Pts',(33.6743371481684,46.875,33.6743371481683));
#13183=CARTESIAN_POINT('Ctrl Pts',(23.,46.6666666666667,39.8371685740842));
#13184=CARTESIAN_POINT('Ctrl Pts',(12.3256628518317,46.4583333333333,46.));
#13185=CARTESIAN_POINT('Ctrl Pts',(8.45006291411674E-15,46.25,46.));
#13186=CARTESIAN_POINT('Ctrl Pts',(-12.3256628518316,46.0416666666667,46.));
#13187=CARTESIAN_POINT('Ctrl Pts',(-23.,45.8333333333333,39.8371685740842));
#13188=CARTESIAN_POINT('Ctrl Pts',(-33.6743371481683,45.625,33.6743371481684));
#13189=CARTESIAN_POINT('Ctrl Pts',(-39.8371685740842,45.4166666666667,23.));
#13190=CARTESIAN_POINT('Ctrl Pts',(-46.,45.2083333333333,12.3256628518317));
#13191=CARTESIAN_POINT('Ctrl Pts',(-46.,45.,0.));
#13192=CARTESIAN_POINT('Ctrl Pts',(-46.,44.7916666666667,-12.3256628518316));
#13193=CARTESIAN_POINT('Ctrl Pts',(-39.8371685740842,44.5833333333333,-23.));
#13194=CARTESIAN_POINT('Ctrl Pts',(-33.6743371481684,44.375,-33.6743371481684));
#13195=CARTESIAN_POINT('Ctrl Pts',(-23.,44.1666666666667,-39.8371685740842));
#13196=CARTESIAN_POINT('Ctrl Pts',(-12.3256628518317,43.9583333333333,-46.));
#13197=CARTESIAN_POINT('Ctrl Pts',(-2.81668763803891E-15,43.75,-46.));
#13198=CARTESIAN_POINT('Ctrl Pts',(12.3256628518316,43.5416666666667,-46.));
#13199=CARTESIAN_POINT('Ctrl Pts',(23.,43.3333333333333,-39.8371685740842));
#13200=CARTESIAN_POINT('Ctrl Pts',(33.6743371481683,43.125,-33.6743371481684));
#13201=CARTESIAN_POINT('Ctrl Pts',(39.8371685740842,42.9166666666667,-23.));
#13202=CARTESIAN_POINT('Ctrl Pts',(46.,42.7083333333333,-12.3256628518317));
#13203=CARTESIAN_POINT('Ctrl Pts',(46.,42.5,-5.63337527607782E-15));
#13204=CARTESIAN_POINT('Ctrl Pts',(46.,42.2916666666667,12.3256628518316));
#13205=CARTESIAN_POINT('Ctrl Pts',(39.8371685740842,42.0833333333333,23.));
#13206=CARTESIAN_POINT('Ctrl Pts',(33.6743371481684,41.875,33.6743371481683));
#13207=CARTESIAN_POINT('Ctrl Pts',(23.,41.6666666666667,39.8371685740842));
#13208=CARTESIAN_POINT('Ctrl Pts',(12.3256628518317,41.4583333333333,46.));
#13209=CARTESIAN_POINT('Ctrl Pts',(8.45006291411674E-15,41.25,46.));
#13210=CARTESIAN_POINT('Ctrl Pts',(-12.3256628518316,41.0416666666667,46.));
#13211=CARTESIAN_POINT('Ctrl Pts',(-23.,40.8333333333333,39.8371685740842));
#13212=CARTESIAN_POINT('Ctrl Pts',(-33.6743371481683,40.625,33.6743371481684));
#13213=CARTESIAN_POINT('Ctrl Pts',(-39.8371685740842,40.4166666666667,23.));
#13214=CARTESIAN_POINT('Ctrl Pts',(-46.,40.2083333333333,12.3256628518317));
#13215=CARTESIAN_POINT('Ctrl Pts',(-46.,40.,0.));
#13216=CARTESIAN_POINT('Ctrl Pts',(-46.,39.7916666666667,-12.3256628518316));
#13217=CARTESIAN_POINT('Ctrl Pts',(-39.8371685740842,39.5833333333333,-23.));
#13218=CARTESIAN_POINT('Ctrl Pts',(-33.6743371481684,39.375,-33.6743371481684));
#13219=CARTESIAN_POINT('Ctrl Pts',(-23.,39.1666666666667,-39.8371685740842));
#13220=CARTESIAN_POINT('Ctrl Pts',(-12.3256628518317,38.9583333333333,-46.));
#13221=CARTESIAN_POINT('Ctrl Pts',(-2.81668763803891E-15,38.75,-46.));
#13222=CARTESIAN_POINT('Ctrl Pts',(12.3256628518316,38.5416666666667,-46.));
#13223=CARTESIAN_POINT('Ctrl Pts',(23.,38.3333333333333,-39.8371685740842));
#13224=CARTESIAN_POINT('Ctrl Pts',(33.6743371481683,38.125,-33.6743371481684));
#13225=CARTESIAN_POINT('Ctrl Pts',(39.8371685740842,37.9166666666667,-23.));
#13226=CARTESIAN_POINT('Ctrl Pts',(46.,37.7083333333333,-12.3256628518317));
#13227=CARTESIAN_POINT('Ctrl Pts',(46.,37.5,-5.63337527607782E-15));
#13228=CARTESIAN_POINT('Ctrl Pts',(46.,37.2916666666667,12.3256628518316));
#13229=CARTESIAN_POINT('Ctrl Pts',(39.8371685740842,37.0833333333333,23.));
#13230=CARTESIAN_POINT('Ctrl Pts',(33.6743371481684,36.875,33.6743371481683));
#13231=CARTESIAN_POINT('Ctrl Pts',(23.,36.6666666666667,39.8371685740842));
#13232=CARTESIAN_POINT('Ctrl Pts',(12.3256628518317,36.4583333333333,46.));
#13233=CARTESIAN_POINT('Ctrl Pts',(8.45006291411674E-15,36.25,46.));
#13234=CARTESIAN_POINT('Ctrl Pts',(-12.3256628518316,36.0416666666667,46.));
#13235=CARTESIAN_POINT('Ctrl Pts',(-23.,35.8333333333333,39.8371685740842));
#13236=CARTESIAN_POINT('Ctrl Pts',(-33.6743371481683,35.625,33.6743371481684));
#13237=CARTESIAN_POINT('Ctrl Pts',(-39.8371685740842,35.4166666666667,23.));
#13238=CARTESIAN_POINT('Ctrl Pts',(-46.,35.2083333333333,12.3256628518317));
#13239=CARTESIAN_POINT('Ctrl Pts',(-46.,35.,0.));
#13240=CARTESIAN_POINT('Ctrl Pts',(-46.,34.7916666666667,-12.3256628518316));
#13241=CARTESIAN_POINT('Ctrl Pts',(-39.8371685740842,34.5833333333333,-23.));
#13242=CARTESIAN_POINT('Ctrl Pts',(-33.6743371481684,34.375,-33.6743371481684));
#13243=CARTESIAN_POINT('Ctrl Pts',(-23.,34.1666666666667,-39.8371685740842));
#13244=CARTESIAN_POINT('Ctrl Pts',(-12.3256628518317,33.9583333333333,-46.));
#13245=CARTESIAN_POINT('Ctrl Pts',(-2.81668763803891E-15,33.75,-46.));
#13246=CARTESIAN_POINT('Ctrl Pts',(12.3256628518316,33.5416666666667,-46.));
#13247=CARTESIAN_POINT('Ctrl Pts',(23.,33.3333333333333,-39.8371685740842));
#13248=CARTESIAN_POINT('Ctrl Pts',(33.6743371481683,33.125,-33.6743371481684));
#13249=CARTESIAN_POINT('Ctrl Pts',(39.8371685740842,32.9166666666667,-23.));
#13250=CARTESIAN_POINT('Ctrl Pts',(46.,32.7083333333333,-12.3256628518317));
#13251=CARTESIAN_POINT('Ctrl Pts',(46.,32.5,-5.63337527607782E-15));
#13252=CARTESIAN_POINT('Ctrl Pts',(46.,32.2916666666667,12.3256628518316));
#13253=CARTESIAN_POINT('Ctrl Pts',(39.8371685740842,32.0833333333333,23.));
#13254=CARTESIAN_POINT('Ctrl Pts',(33.6743371481684,31.875,33.6743371481683));
#13255=CARTESIAN_POINT('Ctrl Pts',(23.,31.6666666666667,39.8371685740842));
#13256=CARTESIAN_POINT('Ctrl Pts',(12.3256628518317,31.4583333333333,46.));
#13257=CARTESIAN_POINT('Ctrl Pts',(8.45006291411674E-15,31.25,46.));
#13258=CARTESIAN_POINT('Ctrl Pts',(-12.3256628518316,31.0416666666667,46.));
#13259=CARTESIAN_POINT('Ctrl Pts',(-23.,30.8333333333333,39.8371685740842));
#13260=CARTESIAN_POINT('Ctrl Pts',(-33.6743371481683,30.625,33.6743371481684));
#13261=CARTESIAN_POINT('Ctrl Pts',(-39.8371685740842,30.4166666666667,23.));
#13262=CARTESIAN_POINT('Ctrl Pts',(-46.,30.2083333333333,12.3256628518317));
#13263=CARTESIAN_POINT('Ctrl Pts',(-46.,30.,0.));
#13264=CARTESIAN_POINT('Ctrl Pts',(45.7957082162897,42.5741208584476,-4.3304859967968));
#13265=CARTESIAN_POINT('Ctrl Pts',(46.027322302781,42.4406160752063,-4.3304859967968));
#13266=CARTESIAN_POINT('Ctrl Pts',(46.4905476657727,42.1736016336912,-4.33048599679655));
#13267=CARTESIAN_POINT('Ctrl Pts',(46.9537676533565,41.9065778670208,-4.33048599679681));
#13268=CARTESIAN_POINT('Ctrl Pts',(47.6280672732221,41.5178683162597,-4.33048599679681));
#13269=CARTESIAN_POINT('Ctrl Pts',(48.0707534890442,41.2626647328764,-4.33048599679679));
#13270=CARTESIAN_POINT('Ctrl Pts',(48.5134353784344,41.0074536451604,-4.33048599679679));
#13271=CARTESIAN_POINT('Ctrl Pts',(3.61292728433798,42.1292520480093,-48.5721450795008));
#13272=CARTESIAN_POINT('Ctrl Pts',(3.61292728433798,42.2624339185675,-48.3403451622818));
#13273=CARTESIAN_POINT('Ctrl Pts',(3.61292728433799,42.395608829009,-48.1085412459393));
#13274=CARTESIAN_POINT('Ctrl Pts',(3.61292728433799,42.6619441142016,-47.6449250631479));
#13275=CARTESIAN_POINT('Ctrl Pts',(3.61292728433793,42.7951044891727,-47.4131127965212));
#13276=CARTESIAN_POINT('Ctrl Pts',(3.61292728433793,42.9282572703914,-47.1812961682826));
#13277=CARTESIAN_POINT('Ctrl Pts',(3.61292728433793,43.1816295626638,-46.7401795055578));
#13278=CARTESIAN_POINT('Ctrl Pts',(3.61292728433795,43.4349743764897,-46.2990470581854));
#13279=CARTESIAN_POINT('Ctrl Pts',(3.61292728433795,43.688289262853,-45.8578974271399));
#13280=CARTESIAN_POINT('Ctrl Pts',(-48.706329375,58.437500006828,-1.8898197019151E-14));
#13281=CARTESIAN_POINT('Ctrl Pts',(-48.706329375,58.2291666734946,-13.0508216223155));
#13282=CARTESIAN_POINT('Ctrl Pts',(-42.1809185638422,58.0208333401613,-24.3531646875));
#13283=CARTESIAN_POINT('Ctrl Pts',(-35.6555077526845,57.812500006828,-35.6555077526845));
#13284=CARTESIAN_POINT('Ctrl Pts',(-24.3531646875,57.6041666734946,-42.1809185638422));
#13285=CARTESIAN_POINT('Ctrl Pts',(-13.0508216223155,57.3958333401613,-48.706329375));
#13286=CARTESIAN_POINT('Ctrl Pts',(1.59157945007855E-14,57.187500006828,
-48.706329375));
#13287=CARTESIAN_POINT('Ctrl Pts',(13.0508216223155,56.9791666734946,-48.706329375));
#13288=CARTESIAN_POINT('Ctrl Pts',(24.3531646875,56.7708333401613,-42.1809185638422));
#13289=CARTESIAN_POINT('Ctrl Pts',(35.6555077526845,56.562500006828,-35.6555077526845));
#13290=CARTESIAN_POINT('Ctrl Pts',(42.1809185638422,56.3541666734946,-24.3531646875));
#13291=CARTESIAN_POINT('Ctrl Pts',(48.706329375,56.1458333401613,-13.0508216223155));
#13292=CARTESIAN_POINT('Ctrl Pts',(48.706329375,55.937500006828,1.293339198242E-14));
#13293=CARTESIAN_POINT('Ctrl Pts',(48.706329375,55.7291666734946,13.0508216223155));
#13294=CARTESIAN_POINT('Ctrl Pts',(42.1809185638422,55.5208333401613,24.3531646875));
#13295=CARTESIAN_POINT('Ctrl Pts',(35.6555077526845,55.312500006828,35.6555077526845));
#13296=CARTESIAN_POINT('Ctrl Pts',(24.3531646875,55.1041666734946,42.1809185638422));
#13297=CARTESIAN_POINT('Ctrl Pts',(13.0508216223155,54.8958333401613,48.706329375));
#13298=CARTESIAN_POINT('Ctrl Pts',(-9.95098946405443E-15,54.687500006828,
48.706329375));
#13299=CARTESIAN_POINT('Ctrl Pts',(-13.0508216223155,54.4791666734946,48.706329375));
#13300=CARTESIAN_POINT('Ctrl Pts',(-24.3531646875,54.2708333401613,42.1809185638423));
#13301=CARTESIAN_POINT('Ctrl Pts',(-35.6555077526845,54.062500006828,35.6555077526845));
#13302=CARTESIAN_POINT('Ctrl Pts',(-42.1809185638422,53.8541666734946,24.3531646875));
#13303=CARTESIAN_POINT('Ctrl Pts',(-48.706329375,53.6458333401613,13.0508216223155));
#13304=CARTESIAN_POINT('Ctrl Pts',(-48.706329375,53.437500006828,-1.8898197019151E-14));
#13305=CARTESIAN_POINT('Ctrl Pts',(-48.706329375,53.2291666734946,-13.0508216223155));
#13306=CARTESIAN_POINT('Ctrl Pts',(-42.1809185638422,53.0208333401613,-24.3531646875));
#13307=CARTESIAN_POINT('Ctrl Pts',(-35.6555077526845,52.812500006828,-35.6555077526845));
#13308=CARTESIAN_POINT('Ctrl Pts',(-24.3531646875,52.6041666734946,-42.1809185638422));
#13309=CARTESIAN_POINT('Ctrl Pts',(-13.0508216223155,52.3958333401613,-48.706329375));
#13310=CARTESIAN_POINT('Ctrl Pts',(1.59157945007855E-14,52.187500006828,
-48.706329375));
#13311=CARTESIAN_POINT('Ctrl Pts',(13.0508216223155,51.9791666734946,-48.706329375));
#13312=CARTESIAN_POINT('Ctrl Pts',(24.3531646875,51.7708333401613,-42.1809185638422));
#13313=CARTESIAN_POINT('Ctrl Pts',(35.6555077526845,51.562500006828,-35.6555077526845));
#13314=CARTESIAN_POINT('Ctrl Pts',(42.1809185638422,51.3541666734946,-24.3531646875));
#13315=CARTESIAN_POINT('Ctrl Pts',(48.706329375,51.1458333401613,-13.0508216223155));
#13316=CARTESIAN_POINT('Ctrl Pts',(48.706329375,50.937500006828,1.293339198242E-14));
#13317=CARTESIAN_POINT('Ctrl Pts',(48.706329375,50.7291666734946,13.0508216223155));
#13318=CARTESIAN_POINT('Ctrl Pts',(42.1809185638422,50.5208333401613,24.3531646875));
#13319=CARTESIAN_POINT('Ctrl Pts',(35.6555077526845,50.312500006828,35.6555077526845));
#13320=CARTESIAN_POINT('Ctrl Pts',(24.3531646875,50.1041666734946,42.1809185638422));
#13321=CARTESIAN_POINT('Ctrl Pts',(13.0508216223155,49.8958333401613,48.706329375));
#13322=CARTESIAN_POINT('Ctrl Pts',(-9.95098946405443E-15,49.687500006828,
48.706329375));
#13323=CARTESIAN_POINT('Ctrl Pts',(-13.0508216223155,49.4791666734946,48.706329375));
#13324=CARTESIAN_POINT('Ctrl Pts',(-24.3531646875,49.2708333401613,42.1809185638423));
#13325=CARTESIAN_POINT('Ctrl Pts',(-35.6555077526845,49.062500006828,35.6555077526845));
#13326=CARTESIAN_POINT('Ctrl Pts',(-42.1809185638422,48.8541666734946,24.3531646875));
#13327=CARTESIAN_POINT('Ctrl Pts',(-48.706329375,48.6458333401613,13.0508216223155));
#13328=CARTESIAN_POINT('Ctrl Pts',(-48.706329375,48.437500006828,-1.8898197019151E-14));
#13329=CARTESIAN_POINT('Ctrl Pts',(-48.706329375,48.2291666734946,-13.0508216223155));
#13330=CARTESIAN_POINT('Ctrl Pts',(-42.1809185638422,48.0208333401613,-24.3531646875));
#13331=CARTESIAN_POINT('Ctrl Pts',(-35.6555077526845,47.812500006828,-35.6555077526845));
#13332=CARTESIAN_POINT('Ctrl Pts',(-24.3531646875,47.6041666734946,-42.1809185638422));
#13333=CARTESIAN_POINT('Ctrl Pts',(-13.0508216223155,47.3958333401613,-48.706329375));
#13334=CARTESIAN_POINT('Ctrl Pts',(1.59157945007855E-14,47.187500006828,
-48.706329375));
#13335=CARTESIAN_POINT('Ctrl Pts',(13.0508216223155,46.9791666734946,-48.706329375));
#13336=CARTESIAN_POINT('Ctrl Pts',(24.3531646875,46.7708333401613,-42.1809185638422));
#13337=CARTESIAN_POINT('Ctrl Pts',(35.6555077526845,46.562500006828,-35.6555077526845));
#13338=CARTESIAN_POINT('Ctrl Pts',(42.1809185638422,46.3541666734946,-24.3531646875));
#13339=CARTESIAN_POINT('Ctrl Pts',(48.706329375,46.1458333401613,-13.0508216223155));
#13340=CARTESIAN_POINT('Ctrl Pts',(48.706329375,45.937500006828,1.293339198242E-14));
#13341=CARTESIAN_POINT('Ctrl Pts',(48.706329375,45.7291666734946,13.0508216223155));
#13342=CARTESIAN_POINT('Ctrl Pts',(42.1809185638422,45.5208333401613,24.3531646875));
#13343=CARTESIAN_POINT('Ctrl Pts',(35.6555077526845,45.312500006828,35.6555077526845));
#13344=CARTESIAN_POINT('Ctrl Pts',(24.3531646875,45.1041666734946,42.1809185638422));
#13345=CARTESIAN_POINT('Ctrl Pts',(13.0508216223155,44.8958333401613,48.706329375));
#13346=CARTESIAN_POINT('Ctrl Pts',(-9.95098946405443E-15,44.687500006828,
48.706329375));
#13347=CARTESIAN_POINT('Ctrl Pts',(-13.0508216223155,44.4791666734946,48.706329375));
#13348=CARTESIAN_POINT('Ctrl Pts',(-24.3531646875,44.2708333401613,42.1809185638423));
#13349=CARTESIAN_POINT('Ctrl Pts',(-35.6555077526845,44.062500006828,35.6555077526845));
#13350=CARTESIAN_POINT('Ctrl Pts',(-42.1809185638422,43.8541666734946,24.3531646875));
#13351=CARTESIAN_POINT('Ctrl Pts',(-48.706329375,43.6458333401613,13.0508216223155));
#13352=CARTESIAN_POINT('Ctrl Pts',(-48.706329375,43.437500006828,-1.8898197019151E-14));
#13353=CARTESIAN_POINT('Ctrl Pts',(-48.706329375,43.2291666734946,-13.0508216223155));
#13354=CARTESIAN_POINT('Ctrl Pts',(-42.1809185638422,43.0208333401613,-24.3531646875));
#13355=CARTESIAN_POINT('Ctrl Pts',(-35.6555077526845,42.812500006828,-35.6555077526845));
#13356=CARTESIAN_POINT('Ctrl Pts',(-24.3531646875,42.6041666734946,-42.1809185638422));
#13357=CARTESIAN_POINT('Ctrl Pts',(-13.0508216223155,42.3958333401613,-48.706329375));
#13358=CARTESIAN_POINT('Ctrl Pts',(1.59157945007855E-14,42.187500006828,
-48.706329375));
#13359=CARTESIAN_POINT('Ctrl Pts',(13.0508216223155,41.9791666734946,-48.706329375));
#13360=CARTESIAN_POINT('Ctrl Pts',(24.3531646875,41.7708333401613,-42.1809185638422));
#13361=CARTESIAN_POINT('Ctrl Pts',(35.6555077526845,41.562500006828,-35.6555077526845));
#13362=CARTESIAN_POINT('Ctrl Pts',(42.1809185638422,41.3541666734946,-24.3531646875));
#13363=CARTESIAN_POINT('Ctrl Pts',(48.706329375,41.1458333401613,-13.0508216223155));
#13364=CARTESIAN_POINT('Ctrl Pts',(48.706329375,40.937500006828,1.293339198242E-14));
#13365=CARTESIAN_POINT('Ctrl Pts',(48.706329375,40.7291666734946,13.0508216223155));
#13366=CARTESIAN_POINT('Ctrl Pts',(42.1809185638422,40.5208333401613,24.3531646875));
#13367=CARTESIAN_POINT('Ctrl Pts',(35.6555077526845,40.312500006828,35.6555077526845));
#13368=CARTESIAN_POINT('Ctrl Pts',(24.3531646875,40.1041666734946,42.1809185638422));
#13369=CARTESIAN_POINT('Ctrl Pts',(13.0508216223155,39.8958333401613,48.706329375));
#13370=CARTESIAN_POINT('Ctrl Pts',(-9.95098946405443E-15,39.687500006828,
48.706329375));
#13371=CARTESIAN_POINT('Ctrl Pts',(-13.0508216223155,39.4791666734946,48.706329375));
#13372=CARTESIAN_POINT('Ctrl Pts',(-24.3531646875,39.2708333401613,42.1809185638423));
#13373=CARTESIAN_POINT('Ctrl Pts',(-35.6555077526845,39.062500006828,35.6555077526845));
#13374=CARTESIAN_POINT('Ctrl Pts',(-42.1809185638422,38.8541666734946,24.3531646875));
#13375=CARTESIAN_POINT('Ctrl Pts',(-48.706329375,38.6458333401613,13.0508216223155));
#13376=CARTESIAN_POINT('Ctrl Pts',(-48.706329375,38.437500006828,-1.8898197019151E-14));
#13377=CARTESIAN_POINT('Ctrl Pts',(-48.706329375,38.2291666734946,-13.0508216223155));
#13378=CARTESIAN_POINT('Ctrl Pts',(-42.1809185638422,38.0208333401613,-24.3531646875));
#13379=CARTESIAN_POINT('Ctrl Pts',(-35.6555077526845,37.812500006828,-35.6555077526845));
#13380=CARTESIAN_POINT('Ctrl Pts',(-24.3531646875,37.6041666734946,-42.1809185638422));
#13381=CARTESIAN_POINT('Ctrl Pts',(-13.0508216223155,37.3958333401613,-48.706329375));
#13382=CARTESIAN_POINT('Ctrl Pts',(1.59157945007855E-14,37.187500006828,
-48.706329375));
#13383=CARTESIAN_POINT('Ctrl Pts',(13.0508216223155,36.9791666734946,-48.706329375));
#13384=CARTESIAN_POINT('Ctrl Pts',(24.3531646875,36.7708333401613,-42.1809185638422));
#13385=CARTESIAN_POINT('Ctrl Pts',(35.6555077526845,36.562500006828,-35.6555077526845));
#13386=CARTESIAN_POINT('Ctrl Pts',(42.1809185638422,36.3541666734946,-24.3531646875));
#13387=CARTESIAN_POINT('Ctrl Pts',(48.706329375,36.1458333401613,-13.0508216223155));
#13388=CARTESIAN_POINT('Ctrl Pts',(48.706329375,35.937500006828,1.293339198242E-14));
#13389=CARTESIAN_POINT('Ctrl Pts',(48.706329375,35.7291666734946,13.0508216223155));
#13390=CARTESIAN_POINT('Ctrl Pts',(42.1809185638422,35.5208333401613,24.3531646875));
#13391=CARTESIAN_POINT('Ctrl Pts',(35.6555077526845,35.312500006828,35.6555077526845));
#13392=CARTESIAN_POINT('Ctrl Pts',(24.3531646875,35.1041666734946,42.1809185638422));
#13393=CARTESIAN_POINT('Ctrl Pts',(13.0508216223155,34.8958333401613,48.706329375));
#13394=CARTESIAN_POINT('Ctrl Pts',(-9.95098946405443E-15,34.687500006828,
48.706329375));
#13395=CARTESIAN_POINT('Ctrl Pts',(-13.0508216223155,34.4791666734946,48.706329375));
#13396=CARTESIAN_POINT('Ctrl Pts',(-24.3531646875,34.2708333401613,42.1809185638423));
#13397=CARTESIAN_POINT('Ctrl Pts',(-35.6555077526845,34.062500006828,35.6555077526845));
#13398=CARTESIAN_POINT('Ctrl Pts',(-42.1809185638422,33.8541666734946,24.3531646875));
#13399=CARTESIAN_POINT('Ctrl Pts',(-48.706329375,33.6458333401613,13.0508216223155));
#13400=CARTESIAN_POINT('Ctrl Pts',(-48.706329375,33.437500006828,-1.8898197019151E-14));
#13401=CARTESIAN_POINT('Ctrl Pts',(-48.706329375,33.2291666734946,-13.0508216223155));
#13402=CARTESIAN_POINT('Ctrl Pts',(-42.1809185638422,33.0208333401613,-24.3531646875));
#13403=CARTESIAN_POINT('Ctrl Pts',(-35.6555077526845,32.812500006828,-35.6555077526845));
#13404=CARTESIAN_POINT('Ctrl Pts',(-24.3531646875,32.6041666734946,-42.1809185638422));
#13405=CARTESIAN_POINT('Ctrl Pts',(-13.0508216223155,32.3958333401613,-48.706329375));
#13406=CARTESIAN_POINT('Ctrl Pts',(1.59157945007855E-14,32.187500006828,
-48.706329375));
#13407=CARTESIAN_POINT('Ctrl Pts',(13.0508216223155,31.9791666734946,-48.706329375));
#13408=CARTESIAN_POINT('Ctrl Pts',(24.3531646875,31.7708333401613,-42.1809185638422));
#13409=CARTESIAN_POINT('Ctrl Pts',(35.6555077526845,31.562500006828,-35.6555077526845));
#13410=CARTESIAN_POINT('Ctrl Pts',(42.1809185638422,31.3541666734946,-24.3531646875));
#13411=CARTESIAN_POINT('Ctrl Pts',(48.706329375,31.1458333401613,-13.0508216223155));
#13412=CARTESIAN_POINT('Ctrl Pts',(48.706329375,30.937500006828,1.293339198242E-14));
#13413=CARTESIAN_POINT('Ctrl Pts',(48.706329375,30.7291666734946,13.0508216223155));
#13414=CARTESIAN_POINT('Ctrl Pts',(42.1809185638422,30.5208333401613,24.3531646875));
#13415=CARTESIAN_POINT('Ctrl Pts',(35.6555077526845,30.312500006828,35.6555077526845));
#13416=CARTESIAN_POINT('Ctrl Pts',(24.3531646875,30.1041666734946,42.1809185638422));
#13417=CARTESIAN_POINT('Ctrl Pts',(13.0508216223155,29.8958333401613,48.706329375));
#13418=CARTESIAN_POINT('Ctrl Pts',(-9.95098946405443E-15,29.687500006828,
48.706329375));
#13419=CARTESIAN_POINT('Ctrl Pts',(-13.0508216223155,29.4791666734946,48.706329375));
#13420=CARTESIAN_POINT('Ctrl Pts',(-24.3531646875,29.2708333401613,42.1809185638423));
#13421=CARTESIAN_POINT('Ctrl Pts',(-35.6555077526845,29.062500006828,35.6555077526845));
#13422=CARTESIAN_POINT('Ctrl Pts',(-42.1809185638422,28.8541666734946,24.3531646875));
#13423=CARTESIAN_POINT('Ctrl Pts',(-48.706329375,28.6458333401613,13.0508216223155));
#13424=CARTESIAN_POINT('Ctrl Pts',(-48.706329375,28.437500006828,-1.8898197019151E-14));
#13425=CARTESIAN_POINT('Ctrl Pts',(-46.,60.,0.));
#13426=CARTESIAN_POINT('Ctrl Pts',(-46.,59.7916666666667,-12.3256628518316));
#13427=CARTESIAN_POINT('Ctrl Pts',(-39.8371685740842,59.5833333333333,-23.));
#13428=CARTESIAN_POINT('Ctrl Pts',(-33.6743371481684,59.375,-33.6743371481684));
#13429=CARTESIAN_POINT('Ctrl Pts',(-23.,59.1666666666667,-39.8371685740842));
#13430=CARTESIAN_POINT('Ctrl Pts',(-12.3256628518317,58.9583333333333,-46.));
#13431=CARTESIAN_POINT('Ctrl Pts',(-2.81668763803891E-15,58.75,-46.));
#13432=CARTESIAN_POINT('Ctrl Pts',(12.3256628518316,58.5416666666667,-46.));
#13433=CARTESIAN_POINT('Ctrl Pts',(23.,58.3333333333333,-39.8371685740842));
#13434=CARTESIAN_POINT('Ctrl Pts',(33.6743371481683,58.125,-33.6743371481684));
#13435=CARTESIAN_POINT('Ctrl Pts',(39.8371685740842,57.9166666666667,-23.));
#13436=CARTESIAN_POINT('Ctrl Pts',(46.,57.7083333333333,-12.3256628518317));
#13437=CARTESIAN_POINT('Ctrl Pts',(46.,57.5,-5.63337527607782E-15));
#13438=CARTESIAN_POINT('Ctrl Pts',(46.,57.2916666666667,12.3256628518316));
#13439=CARTESIAN_POINT('Ctrl Pts',(39.8371685740842,57.0833333333333,23.));
#13440=CARTESIAN_POINT('Ctrl Pts',(33.6743371481684,56.875,33.6743371481683));
#13441=CARTESIAN_POINT('Ctrl Pts',(23.,56.6666666666667,39.8371685740842));
#13442=CARTESIAN_POINT('Ctrl Pts',(12.3256628518317,56.4583333333333,46.));
#13443=CARTESIAN_POINT('Ctrl Pts',(8.45006291411674E-15,56.25,46.));
#13444=CARTESIAN_POINT('Ctrl Pts',(-12.3256628518316,56.0416666666667,46.));
#13445=CARTESIAN_POINT('Ctrl Pts',(-23.,55.8333333333333,39.8371685740842));
#13446=CARTESIAN_POINT('Ctrl Pts',(-33.6743371481683,55.625,33.6743371481684));
#13447=CARTESIAN_POINT('Ctrl Pts',(-39.8371685740842,55.4166666666667,23.));
#13448=CARTESIAN_POINT('Ctrl Pts',(-46.,55.2083333333333,12.3256628518317));
#13449=CARTESIAN_POINT('Ctrl Pts',(-46.,55.,0.));
#13450=CARTESIAN_POINT('Ctrl Pts',(-46.,54.7916666666667,-12.3256628518316));
#13451=CARTESIAN_POINT('Ctrl Pts',(-39.8371685740842,54.5833333333333,-23.));
#13452=CARTESIAN_POINT('Ctrl Pts',(-33.6743371481684,54.375,-33.6743371481684));
#13453=CARTESIAN_POINT('Ctrl Pts',(-23.,54.1666666666667,-39.8371685740842));
#13454=CARTESIAN_POINT('Ctrl Pts',(-12.3256628518317,53.9583333333333,-46.));
#13455=CARTESIAN_POINT('Ctrl Pts',(-2.81668763803891E-15,53.75,-46.));
#13456=CARTESIAN_POINT('Ctrl Pts',(12.3256628518316,53.5416666666667,-46.));
#13457=CARTESIAN_POINT('Ctrl Pts',(23.,53.3333333333333,-39.8371685740842));
#13458=CARTESIAN_POINT('Ctrl Pts',(33.6743371481683,53.125,-33.6743371481684));
#13459=CARTESIAN_POINT('Ctrl Pts',(39.8371685740842,52.9166666666667,-23.));
#13460=CARTESIAN_POINT('Ctrl Pts',(46.,52.7083333333333,-12.3256628518317));
#13461=CARTESIAN_POINT('Ctrl Pts',(46.,52.5,-5.63337527607782E-15));
#13462=CARTESIAN_POINT('Ctrl Pts',(46.,52.2916666666667,12.3256628518316));
#13463=CARTESIAN_POINT('Ctrl Pts',(39.8371685740842,52.0833333333333,23.));
#13464=CARTESIAN_POINT('Ctrl Pts',(33.6743371481684,51.875,33.6743371481683));
#13465=CARTESIAN_POINT('Ctrl Pts',(23.,51.6666666666667,39.8371685740842));
#13466=CARTESIAN_POINT('Ctrl Pts',(12.3256628518317,51.4583333333333,46.));
#13467=CARTESIAN_POINT('Ctrl Pts',(8.45006291411674E-15,51.25,46.));
#13468=CARTESIAN_POINT('Ctrl Pts',(-12.3256628518316,51.0416666666667,46.));
#13469=CARTESIAN_POINT('Ctrl Pts',(-23.,50.8333333333333,39.8371685740842));
#13470=CARTESIAN_POINT('Ctrl Pts',(-33.6743371481683,50.625,33.6743371481684));
#13471=CARTESIAN_POINT('Ctrl Pts',(-39.8371685740842,50.4166666666667,23.));
#13472=CARTESIAN_POINT('Ctrl Pts',(-46.,50.2083333333333,12.3256628518317));
#13473=CARTESIAN_POINT('Ctrl Pts',(-46.,50.,0.));
#13474=CARTESIAN_POINT('Ctrl Pts',(-46.,49.7916666666667,-12.3256628518316));
#13475=CARTESIAN_POINT('Ctrl Pts',(-39.8371685740842,49.5833333333333,-23.));
#13476=CARTESIAN_POINT('Ctrl Pts',(-33.6743371481684,49.375,-33.6743371481684));
#13477=CARTESIAN_POINT('Ctrl Pts',(-23.,49.1666666666667,-39.8371685740842));
#13478=CARTESIAN_POINT('Ctrl Pts',(-12.3256628518317,48.9583333333333,-46.));
#13479=CARTESIAN_POINT('Ctrl Pts',(-2.81668763803891E-15,48.75,-46.));
#13480=CARTESIAN_POINT('Ctrl Pts',(12.3256628518316,48.5416666666667,-46.));
#13481=CARTESIAN_POINT('Ctrl Pts',(23.,48.3333333333333,-39.8371685740842));
#13482=CARTESIAN_POINT('Ctrl Pts',(33.6743371481683,48.125,-33.6743371481684));
#13483=CARTESIAN_POINT('Ctrl Pts',(39.8371685740842,47.9166666666667,-23.));
#13484=CARTESIAN_POINT('Ctrl Pts',(46.,47.7083333333333,-12.3256628518317));
#13485=CARTESIAN_POINT('Ctrl Pts',(46.,47.5,-5.63337527607782E-15));
#13486=CARTESIAN_POINT('Ctrl Pts',(46.,47.2916666666667,12.3256628518316));
#13487=CARTESIAN_POINT('Ctrl Pts',(39.8371685740842,47.0833333333333,23.));
#13488=CARTESIAN_POINT('Ctrl Pts',(33.6743371481684,46.875,33.6743371481683));
#13489=CARTESIAN_POINT('Ctrl Pts',(23.,46.6666666666667,39.8371685740842));
#13490=CARTESIAN_POINT('Ctrl Pts',(12.3256628518317,46.4583333333333,46.));
#13491=CARTESIAN_POINT('Ctrl Pts',(8.45006291411674E-15,46.25,46.));
#13492=CARTESIAN_POINT('Ctrl Pts',(-12.3256628518316,46.0416666666667,46.));
#13493=CARTESIAN_POINT('Ctrl Pts',(-23.,45.8333333333333,39.8371685740842));
#13494=CARTESIAN_POINT('Ctrl Pts',(-33.6743371481683,45.625,33.6743371481684));
#13495=CARTESIAN_POINT('Ctrl Pts',(-39.8371685740842,45.4166666666667,23.));
#13496=CARTESIAN_POINT('Ctrl Pts',(-46.,45.2083333333333,12.3256628518317));
#13497=CARTESIAN_POINT('Ctrl Pts',(-46.,45.,0.));
#13498=CARTESIAN_POINT('Ctrl Pts',(-46.,44.7916666666667,-12.3256628518316));
#13499=CARTESIAN_POINT('Ctrl Pts',(-39.8371685740842,44.5833333333333,-23.));
#13500=CARTESIAN_POINT('Ctrl Pts',(-33.6743371481684,44.375,-33.6743371481684));
#13501=CARTESIAN_POINT('Ctrl Pts',(-23.,44.1666666666667,-39.8371685740842));
#13502=CARTESIAN_POINT('Ctrl Pts',(-12.3256628518317,43.9583333333333,-46.));
#13503=CARTESIAN_POINT('Ctrl Pts',(-2.81668763803891E-15,43.75,-46.));
#13504=CARTESIAN_POINT('Ctrl Pts',(12.3256628518316,43.5416666666667,-46.));
#13505=CARTESIAN_POINT('Ctrl Pts',(23.,43.3333333333333,-39.8371685740842));
#13506=CARTESIAN_POINT('Ctrl Pts',(33.6743371481683,43.125,-33.6743371481684));
#13507=CARTESIAN_POINT('Ctrl Pts',(39.8371685740842,42.9166666666667,-23.));
#13508=CARTESIAN_POINT('Ctrl Pts',(46.,42.7083333333333,-12.3256628518317));
#13509=CARTESIAN_POINT('Ctrl Pts',(46.,42.5,-5.63337527607782E-15));
#13510=CARTESIAN_POINT('Ctrl Pts',(46.,42.2916666666667,12.3256628518316));
#13511=CARTESIAN_POINT('Ctrl Pts',(39.8371685740842,42.0833333333333,23.));
#13512=CARTESIAN_POINT('Ctrl Pts',(33.6743371481684,41.875,33.6743371481683));
#13513=CARTESIAN_POINT('Ctrl Pts',(23.,41.6666666666667,39.8371685740842));
#13514=CARTESIAN_POINT('Ctrl Pts',(12.3256628518317,41.4583333333333,46.));
#13515=CARTESIAN_POINT('Ctrl Pts',(8.45006291411674E-15,41.25,46.));
#13516=CARTESIAN_POINT('Ctrl Pts',(-12.3256628518316,41.0416666666667,46.));
#13517=CARTESIAN_POINT('Ctrl Pts',(-23.,40.8333333333333,39.8371685740842));
#13518=CARTESIAN_POINT('Ctrl Pts',(-33.6743371481683,40.625,33.6743371481684));
#13519=CARTESIAN_POINT('Ctrl Pts',(-39.8371685740842,40.4166666666667,23.));
#13520=CARTESIAN_POINT('Ctrl Pts',(-46.,40.2083333333333,12.3256628518317));
#13521=CARTESIAN_POINT('Ctrl Pts',(-46.,40.,0.));
#13522=CARTESIAN_POINT('Ctrl Pts',(-46.,39.7916666666667,-12.3256628518316));
#13523=CARTESIAN_POINT('Ctrl Pts',(-39.8371685740842,39.5833333333333,-23.));
#13524=CARTESIAN_POINT('Ctrl Pts',(-33.6743371481684,39.375,-33.6743371481684));
#13525=CARTESIAN_POINT('Ctrl Pts',(-23.,39.1666666666667,-39.8371685740842));
#13526=CARTESIAN_POINT('Ctrl Pts',(-12.3256628518317,38.9583333333333,-46.));
#13527=CARTESIAN_POINT('Ctrl Pts',(-2.81668763803891E-15,38.75,-46.));
#13528=CARTESIAN_POINT('Ctrl Pts',(12.3256628518316,38.5416666666667,-46.));
#13529=CARTESIAN_POINT('Ctrl Pts',(23.,38.3333333333333,-39.8371685740842));
#13530=CARTESIAN_POINT('Ctrl Pts',(33.6743371481683,38.125,-33.6743371481684));
#13531=CARTESIAN_POINT('Ctrl Pts',(39.8371685740842,37.9166666666667,-23.));
#13532=CARTESIAN_POINT('Ctrl Pts',(46.,37.7083333333333,-12.3256628518317));
#13533=CARTESIAN_POINT('Ctrl Pts',(46.,37.5,-5.63337527607782E-15));
#13534=CARTESIAN_POINT('Ctrl Pts',(46.,37.2916666666667,12.3256628518316));
#13535=CARTESIAN_POINT('Ctrl Pts',(39.8371685740842,37.0833333333333,23.));
#13536=CARTESIAN_POINT('Ctrl Pts',(33.6743371481684,36.875,33.6743371481683));
#13537=CARTESIAN_POINT('Ctrl Pts',(23.,36.6666666666667,39.8371685740842));
#13538=CARTESIAN_POINT('Ctrl Pts',(12.3256628518317,36.4583333333333,46.));
#13539=CARTESIAN_POINT('Ctrl Pts',(8.45006291411674E-15,36.25,46.));
#13540=CARTESIAN_POINT('Ctrl Pts',(-12.3256628518316,36.0416666666667,46.));
#13541=CARTESIAN_POINT('Ctrl Pts',(-23.,35.8333333333333,39.8371685740842));
#13542=CARTESIAN_POINT('Ctrl Pts',(-33.6743371481683,35.625,33.6743371481684));
#13543=CARTESIAN_POINT('Ctrl Pts',(-39.8371685740842,35.4166666666667,23.));
#13544=CARTESIAN_POINT('Ctrl Pts',(-46.,35.2083333333333,12.3256628518317));
#13545=CARTESIAN_POINT('Ctrl Pts',(-46.,35.,0.));
#13546=CARTESIAN_POINT('Ctrl Pts',(-46.,34.7916666666667,-12.3256628518316));
#13547=CARTESIAN_POINT('Ctrl Pts',(-39.8371685740842,34.5833333333333,-23.));
#13548=CARTESIAN_POINT('Ctrl Pts',(-33.6743371481684,34.375,-33.6743371481684));
#13549=CARTESIAN_POINT('Ctrl Pts',(-23.,34.1666666666667,-39.8371685740842));
#13550=CARTESIAN_POINT('Ctrl Pts',(-12.3256628518317,33.9583333333333,-46.));
#13551=CARTESIAN_POINT('Ctrl Pts',(-2.81668763803891E-15,33.75,-46.));
#13552=CARTESIAN_POINT('Ctrl Pts',(12.3256628518316,33.5416666666667,-46.));
#13553=CARTESIAN_POINT('Ctrl Pts',(23.,33.3333333333333,-39.8371685740842));
#13554=CARTESIAN_POINT('Ctrl Pts',(33.6743371481683,33.125,-33.6743371481684));
#13555=CARTESIAN_POINT('Ctrl Pts',(39.8371685740842,32.9166666666667,-23.));
#13556=CARTESIAN_POINT('Ctrl Pts',(46.,32.7083333333333,-12.3256628518317));
#13557=CARTESIAN_POINT('Ctrl Pts',(46.,32.5,-5.63337527607782E-15));
#13558=CARTESIAN_POINT('Ctrl Pts',(46.,32.2916666666667,12.3256628518316));
#13559=CARTESIAN_POINT('Ctrl Pts',(39.8371685740842,32.0833333333333,23.));
#13560=CARTESIAN_POINT('Ctrl Pts',(33.6743371481684,31.875,33.6743371481683));
#13561=CARTESIAN_POINT('Ctrl Pts',(23.,31.6666666666667,39.8371685740842));
#13562=CARTESIAN_POINT('Ctrl Pts',(12.3256628518317,31.4583333333333,46.));
#13563=CARTESIAN_POINT('Ctrl Pts',(8.45006291411674E-15,31.25,46.));
#13564=CARTESIAN_POINT('Ctrl Pts',(-12.3256628518316,31.0416666666667,46.));
#13565=CARTESIAN_POINT('Ctrl Pts',(-23.,30.8333333333333,39.8371685740842));
#13566=CARTESIAN_POINT('Ctrl Pts',(-33.6743371481683,30.625,33.6743371481684));
#13567=CARTESIAN_POINT('Ctrl Pts',(-39.8371685740842,30.4166666666667,23.));
#13568=CARTESIAN_POINT('Ctrl Pts',(-46.,30.2083333333333,12.3256628518317));
#13569=CARTESIAN_POINT('Ctrl Pts',(-46.,30.,0.));
#13570=CARTESIAN_POINT('Ctrl Pts',(48.5725845633798,40.8793483229262,3.60701400320329));
#13571=CARTESIAN_POINT('Ctrl Pts',(48.3407853679392,41.0125314497137,3.60701400320329));
#13572=CARTESIAN_POINT('Ctrl Pts',(48.1089821836664,41.1457076343819,3.60701400320328));
#13573=CARTESIAN_POINT('Ctrl Pts',(47.6453674864979,41.4120455056142,3.60701400320328));
#13574=CARTESIAN_POINT('Ctrl Pts',(47.4135559734254,41.5452071923974,3.60701400320326));
#13575=CARTESIAN_POINT('Ctrl Pts',(47.1817401099609,41.6783613050641,3.60701400320326));
#13576=CARTESIAN_POINT('Ctrl Pts',(46.7406305897488,41.9317328641751,3.60701400320326));
#13577=CARTESIAN_POINT('Ctrl Pts',(46.2995053259033,42.1850770165972,3.60701400320326));
#13578=CARTESIAN_POINT('Ctrl Pts',(45.858362923034,42.438391319744,3.60701400320326));
#13579=CARTESIAN_POINT('Ctrl Pts',(3.61292728433799,41.311710737147,45.8578974271399));
#13580=CARTESIAN_POINT('Ctrl Pts',(3.61292728433799,41.178117727701,46.089460636719));
#13581=CARTESIAN_POINT('Ctrl Pts',(3.61292728433786,40.9109294856547,46.5525857733052));
#13582=CARTESIAN_POINT('Ctrl Pts',(3.61292728433808,40.6437369897944,47.0157084557285));
#13583=CARTESIAN_POINT('Ctrl Pts',(3.61292728433808,40.2553460757966,47.6888965792834));
#13584=CARTESIAN_POINT('Ctrl Pts',(3.61292728433799,40.0005487265709,48.1305218136162));
#13585=CARTESIAN_POINT('Ctrl Pts',(3.61292728433799,39.7457479656467,48.5721450795008));
#13586=CARTESIAN_POINT('Ctrl Pts',(-48.706329375,58.437500006828,-1.8898197019151E-14));
#13587=CARTESIAN_POINT('Ctrl Pts',(-48.706329375,58.2291666734946,-13.0508216223155));
#13588=CARTESIAN_POINT('Ctrl Pts',(-42.1809185638422,58.0208333401613,-24.3531646875));
#13589=CARTESIAN_POINT('Ctrl Pts',(-35.6555077526845,57.812500006828,-35.6555077526845));
#13590=CARTESIAN_POINT('Ctrl Pts',(-24.3531646875,57.6041666734946,-42.1809185638422));
#13591=CARTESIAN_POINT('Ctrl Pts',(-13.0508216223155,57.3958333401613,-48.706329375));
#13592=CARTESIAN_POINT('Ctrl Pts',(1.59157945007855E-14,57.187500006828,
-48.706329375));
#13593=CARTESIAN_POINT('Ctrl Pts',(13.0508216223155,56.9791666734946,-48.706329375));
#13594=CARTESIAN_POINT('Ctrl Pts',(24.3531646875,56.7708333401613,-42.1809185638422));
#13595=CARTESIAN_POINT('Ctrl Pts',(35.6555077526845,56.562500006828,-35.6555077526845));
#13596=CARTESIAN_POINT('Ctrl Pts',(42.1809185638422,56.3541666734946,-24.3531646875));
#13597=CARTESIAN_POINT('Ctrl Pts',(48.706329375,56.1458333401613,-13.0508216223155));
#13598=CARTESIAN_POINT('Ctrl Pts',(48.706329375,55.937500006828,1.293339198242E-14));
#13599=CARTESIAN_POINT('Ctrl Pts',(48.706329375,55.7291666734946,13.0508216223155));
#13600=CARTESIAN_POINT('Ctrl Pts',(42.1809185638422,55.5208333401613,24.3531646875));
#13601=CARTESIAN_POINT('Ctrl Pts',(35.6555077526845,55.312500006828,35.6555077526845));
#13602=CARTESIAN_POINT('Ctrl Pts',(24.3531646875,55.1041666734946,42.1809185638422));
#13603=CARTESIAN_POINT('Ctrl Pts',(13.0508216223155,54.8958333401613,48.706329375));
#13604=CARTESIAN_POINT('Ctrl Pts',(-9.95098946405443E-15,54.687500006828,
48.706329375));
#13605=CARTESIAN_POINT('Ctrl Pts',(-13.0508216223155,54.4791666734946,48.706329375));
#13606=CARTESIAN_POINT('Ctrl Pts',(-24.3531646875,54.2708333401613,42.1809185638423));
#13607=CARTESIAN_POINT('Ctrl Pts',(-35.6555077526845,54.062500006828,35.6555077526845));
#13608=CARTESIAN_POINT('Ctrl Pts',(-42.1809185638422,53.8541666734946,24.3531646875));
#13609=CARTESIAN_POINT('Ctrl Pts',(-48.706329375,53.6458333401613,13.0508216223155));
#13610=CARTESIAN_POINT('Ctrl Pts',(-48.706329375,53.437500006828,-1.8898197019151E-14));
#13611=CARTESIAN_POINT('Ctrl Pts',(-48.706329375,53.2291666734946,-13.0508216223155));
#13612=CARTESIAN_POINT('Ctrl Pts',(-42.1809185638422,53.0208333401613,-24.3531646875));
#13613=CARTESIAN_POINT('Ctrl Pts',(-35.6555077526845,52.812500006828,-35.6555077526845));
#13614=CARTESIAN_POINT('Ctrl Pts',(-24.3531646875,52.6041666734946,-42.1809185638422));
#13615=CARTESIAN_POINT('Ctrl Pts',(-13.0508216223155,52.3958333401613,-48.706329375));
#13616=CARTESIAN_POINT('Ctrl Pts',(1.59157945007855E-14,52.187500006828,
-48.706329375));
#13617=CARTESIAN_POINT('Ctrl Pts',(13.0508216223155,51.9791666734946,-48.706329375));
#13618=CARTESIAN_POINT('Ctrl Pts',(24.3531646875,51.7708333401613,-42.1809185638422));
#13619=CARTESIAN_POINT('Ctrl Pts',(35.6555077526845,51.562500006828,-35.6555077526845));
#13620=CARTESIAN_POINT('Ctrl Pts',(42.1809185638422,51.3541666734946,-24.3531646875));
#13621=CARTESIAN_POINT('Ctrl Pts',(48.706329375,51.1458333401613,-13.0508216223155));
#13622=CARTESIAN_POINT('Ctrl Pts',(48.706329375,50.937500006828,1.293339198242E-14));
#13623=CARTESIAN_POINT('Ctrl Pts',(48.706329375,50.7291666734946,13.0508216223155));
#13624=CARTESIAN_POINT('Ctrl Pts',(42.1809185638422,50.5208333401613,24.3531646875));
#13625=CARTESIAN_POINT('Ctrl Pts',(35.6555077526845,50.312500006828,35.6555077526845));
#13626=CARTESIAN_POINT('Ctrl Pts',(24.3531646875,50.1041666734946,42.1809185638422));
#13627=CARTESIAN_POINT('Ctrl Pts',(13.0508216223155,49.8958333401613,48.706329375));
#13628=CARTESIAN_POINT('Ctrl Pts',(-9.95098946405443E-15,49.687500006828,
48.706329375));
#13629=CARTESIAN_POINT('Ctrl Pts',(-13.0508216223155,49.4791666734946,48.706329375));
#13630=CARTESIAN_POINT('Ctrl Pts',(-24.3531646875,49.2708333401613,42.1809185638423));
#13631=CARTESIAN_POINT('Ctrl Pts',(-35.6555077526845,49.062500006828,35.6555077526845));
#13632=CARTESIAN_POINT('Ctrl Pts',(-42.1809185638422,48.8541666734946,24.3531646875));
#13633=CARTESIAN_POINT('Ctrl Pts',(-48.706329375,48.6458333401613,13.0508216223155));
#13634=CARTESIAN_POINT('Ctrl Pts',(-48.706329375,48.437500006828,-1.8898197019151E-14));
#13635=CARTESIAN_POINT('Ctrl Pts',(-48.706329375,48.2291666734946,-13.0508216223155));
#13636=CARTESIAN_POINT('Ctrl Pts',(-42.1809185638422,48.0208333401613,-24.3531646875));
#13637=CARTESIAN_POINT('Ctrl Pts',(-35.6555077526845,47.812500006828,-35.6555077526845));
#13638=CARTESIAN_POINT('Ctrl Pts',(-24.3531646875,47.6041666734946,-42.1809185638422));
#13639=CARTESIAN_POINT('Ctrl Pts',(-13.0508216223155,47.3958333401613,-48.706329375));
#13640=CARTESIAN_POINT('Ctrl Pts',(1.59157945007855E-14,47.187500006828,
-48.706329375));
#13641=CARTESIAN_POINT('Ctrl Pts',(13.0508216223155,46.9791666734946,-48.706329375));
#13642=CARTESIAN_POINT('Ctrl Pts',(24.3531646875,46.7708333401613,-42.1809185638422));
#13643=CARTESIAN_POINT('Ctrl Pts',(35.6555077526845,46.562500006828,-35.6555077526845));
#13644=CARTESIAN_POINT('Ctrl Pts',(42.1809185638422,46.3541666734946,-24.3531646875));
#13645=CARTESIAN_POINT('Ctrl Pts',(48.706329375,46.1458333401613,-13.0508216223155));
#13646=CARTESIAN_POINT('Ctrl Pts',(48.706329375,45.937500006828,1.293339198242E-14));
#13647=CARTESIAN_POINT('Ctrl Pts',(48.706329375,45.7291666734946,13.0508216223155));
#13648=CARTESIAN_POINT('Ctrl Pts',(42.1809185638422,45.5208333401613,24.3531646875));
#13649=CARTESIAN_POINT('Ctrl Pts',(35.6555077526845,45.312500006828,35.6555077526845));
#13650=CARTESIAN_POINT('Ctrl Pts',(24.3531646875,45.1041666734946,42.1809185638422));
#13651=CARTESIAN_POINT('Ctrl Pts',(13.0508216223155,44.8958333401613,48.706329375));
#13652=CARTESIAN_POINT('Ctrl Pts',(-9.95098946405443E-15,44.687500006828,
48.706329375));
#13653=CARTESIAN_POINT('Ctrl Pts',(-13.0508216223155,44.4791666734946,48.706329375));
#13654=CARTESIAN_POINT('Ctrl Pts',(-24.3531646875,44.2708333401613,42.1809185638423));
#13655=CARTESIAN_POINT('Ctrl Pts',(-35.6555077526845,44.062500006828,35.6555077526845));
#13656=CARTESIAN_POINT('Ctrl Pts',(-42.1809185638422,43.8541666734946,24.3531646875));
#13657=CARTESIAN_POINT('Ctrl Pts',(-48.706329375,43.6458333401613,13.0508216223155));
#13658=CARTESIAN_POINT('Ctrl Pts',(-48.706329375,43.437500006828,-1.8898197019151E-14));
#13659=CARTESIAN_POINT('Ctrl Pts',(-48.706329375,43.2291666734946,-13.0508216223155));
#13660=CARTESIAN_POINT('Ctrl Pts',(-42.1809185638422,43.0208333401613,-24.3531646875));
#13661=CARTESIAN_POINT('Ctrl Pts',(-35.6555077526845,42.812500006828,-35.6555077526845));
#13662=CARTESIAN_POINT('Ctrl Pts',(-24.3531646875,42.6041666734946,-42.1809185638422));
#13663=CARTESIAN_POINT('Ctrl Pts',(-13.0508216223155,42.3958333401613,-48.706329375));
#13664=CARTESIAN_POINT('Ctrl Pts',(1.59157945007855E-14,42.187500006828,
-48.706329375));
#13665=CARTESIAN_POINT('Ctrl Pts',(13.0508216223155,41.9791666734946,-48.706329375));
#13666=CARTESIAN_POINT('Ctrl Pts',(24.3531646875,41.7708333401613,-42.1809185638422));
#13667=CARTESIAN_POINT('Ctrl Pts',(35.6555077526845,41.562500006828,-35.6555077526845));
#13668=CARTESIAN_POINT('Ctrl Pts',(42.1809185638422,41.3541666734946,-24.3531646875));
#13669=CARTESIAN_POINT('Ctrl Pts',(48.706329375,41.1458333401613,-13.0508216223155));
#13670=CARTESIAN_POINT('Ctrl Pts',(48.706329375,40.937500006828,1.293339198242E-14));
#13671=CARTESIAN_POINT('Ctrl Pts',(48.706329375,40.7291666734946,13.0508216223155));
#13672=CARTESIAN_POINT('Ctrl Pts',(42.1809185638422,40.5208333401613,24.3531646875));
#13673=CARTESIAN_POINT('Ctrl Pts',(35.6555077526845,40.312500006828,35.6555077526845));
#13674=CARTESIAN_POINT('Ctrl Pts',(24.3531646875,40.1041666734946,42.1809185638422));
#13675=CARTESIAN_POINT('Ctrl Pts',(13.0508216223155,39.8958333401613,48.706329375));
#13676=CARTESIAN_POINT('Ctrl Pts',(-9.95098946405443E-15,39.687500006828,
48.706329375));
#13677=CARTESIAN_POINT('Ctrl Pts',(-13.0508216223155,39.4791666734946,48.706329375));
#13678=CARTESIAN_POINT('Ctrl Pts',(-24.3531646875,39.2708333401613,42.1809185638423));
#13679=CARTESIAN_POINT('Ctrl Pts',(-35.6555077526845,39.062500006828,35.6555077526845));
#13680=CARTESIAN_POINT('Ctrl Pts',(-42.1809185638422,38.8541666734946,24.3531646875));
#13681=CARTESIAN_POINT('Ctrl Pts',(-48.706329375,38.6458333401613,13.0508216223155));
#13682=CARTESIAN_POINT('Ctrl Pts',(-48.706329375,38.437500006828,-1.8898197019151E-14));
#13683=CARTESIAN_POINT('Ctrl Pts',(-48.706329375,38.2291666734946,-13.0508216223155));
#13684=CARTESIAN_POINT('Ctrl Pts',(-42.1809185638422,38.0208333401613,-24.3531646875));
#13685=CARTESIAN_POINT('Ctrl Pts',(-35.6555077526845,37.812500006828,-35.6555077526845));
#13686=CARTESIAN_POINT('Ctrl Pts',(-24.3531646875,37.6041666734946,-42.1809185638422));
#13687=CARTESIAN_POINT('Ctrl Pts',(-13.0508216223155,37.3958333401613,-48.706329375));
#13688=CARTESIAN_POINT('Ctrl Pts',(1.59157945007855E-14,37.187500006828,
-48.706329375));
#13689=CARTESIAN_POINT('Ctrl Pts',(13.0508216223155,36.9791666734946,-48.706329375));
#13690=CARTESIAN_POINT('Ctrl Pts',(24.3531646875,36.7708333401613,-42.1809185638422));
#13691=CARTESIAN_POINT('Ctrl Pts',(35.6555077526845,36.562500006828,-35.6555077526845));
#13692=CARTESIAN_POINT('Ctrl Pts',(42.1809185638422,36.3541666734946,-24.3531646875));
#13693=CARTESIAN_POINT('Ctrl Pts',(48.706329375,36.1458333401613,-13.0508216223155));
#13694=CARTESIAN_POINT('Ctrl Pts',(48.706329375,35.937500006828,1.293339198242E-14));
#13695=CARTESIAN_POINT('Ctrl Pts',(48.706329375,35.7291666734946,13.0508216223155));
#13696=CARTESIAN_POINT('Ctrl Pts',(42.1809185638422,35.5208333401613,24.3531646875));
#13697=CARTESIAN_POINT('Ctrl Pts',(35.6555077526845,35.312500006828,35.6555077526845));
#13698=CARTESIAN_POINT('Ctrl Pts',(24.3531646875,35.1041666734946,42.1809185638422));
#13699=CARTESIAN_POINT('Ctrl Pts',(13.0508216223155,34.8958333401613,48.706329375));
#13700=CARTESIAN_POINT('Ctrl Pts',(-9.95098946405443E-15,34.687500006828,
48.706329375));
#13701=CARTESIAN_POINT('Ctrl Pts',(-13.0508216223155,34.4791666734946,48.706329375));
#13702=CARTESIAN_POINT('Ctrl Pts',(-24.3531646875,34.2708333401613,42.1809185638423));
#13703=CARTESIAN_POINT('Ctrl Pts',(-35.6555077526845,34.062500006828,35.6555077526845));
#13704=CARTESIAN_POINT('Ctrl Pts',(-42.1809185638422,33.8541666734946,24.3531646875));
#13705=CARTESIAN_POINT('Ctrl Pts',(-48.706329375,33.6458333401613,13.0508216223155));
#13706=CARTESIAN_POINT('Ctrl Pts',(-48.706329375,33.437500006828,-1.8898197019151E-14));
#13707=CARTESIAN_POINT('Ctrl Pts',(-48.706329375,33.2291666734946,-13.0508216223155));
#13708=CARTESIAN_POINT('Ctrl Pts',(-42.1809185638422,33.0208333401613,-24.3531646875));
#13709=CARTESIAN_POINT('Ctrl Pts',(-35.6555077526845,32.812500006828,-35.6555077526845));
#13710=CARTESIAN_POINT('Ctrl Pts',(-24.3531646875,32.6041666734946,-42.1809185638422));
#13711=CARTESIAN_POINT('Ctrl Pts',(-13.0508216223155,32.3958333401613,-48.706329375));
#13712=CARTESIAN_POINT('Ctrl Pts',(1.59157945007855E-14,32.187500006828,
-48.706329375));
#13713=CARTESIAN_POINT('Ctrl Pts',(13.0508216223155,31.9791666734946,-48.706329375));
#13714=CARTESIAN_POINT('Ctrl Pts',(24.3531646875,31.7708333401613,-42.1809185638422));
#13715=CARTESIAN_POINT('Ctrl Pts',(35.6555077526845,31.562500006828,-35.6555077526845));
#13716=CARTESIAN_POINT('Ctrl Pts',(42.1809185638422,31.3541666734946,-24.3531646875));
#13717=CARTESIAN_POINT('Ctrl Pts',(48.706329375,31.1458333401613,-13.0508216223155));
#13718=CARTESIAN_POINT('Ctrl Pts',(48.706329375,30.937500006828,1.293339198242E-14));
#13719=CARTESIAN_POINT('Ctrl Pts',(48.706329375,30.7291666734946,13.0508216223155));
#13720=CARTESIAN_POINT('Ctrl Pts',(42.1809185638422,30.5208333401613,24.3531646875));
#13721=CARTESIAN_POINT('Ctrl Pts',(35.6555077526845,30.312500006828,35.6555077526845));
#13722=CARTESIAN_POINT('Ctrl Pts',(24.3531646875,30.1041666734946,42.1809185638422));
#13723=CARTESIAN_POINT('Ctrl Pts',(13.0508216223155,29.8958333401613,48.706329375));
#13724=CARTESIAN_POINT('Ctrl Pts',(-9.95098946405443E-15,29.687500006828,
48.706329375));
#13725=CARTESIAN_POINT('Ctrl Pts',(-13.0508216223155,29.4791666734946,48.706329375));
#13726=CARTESIAN_POINT('Ctrl Pts',(-24.3531646875,29.2708333401613,42.1809185638423));
#13727=CARTESIAN_POINT('Ctrl Pts',(-35.6555077526845,29.062500006828,35.6555077526845));
#13728=CARTESIAN_POINT('Ctrl Pts',(-42.1809185638422,28.8541666734946,24.3531646875));
#13729=CARTESIAN_POINT('Ctrl Pts',(-48.706329375,28.6458333401613,13.0508216223155));
#13730=CARTESIAN_POINT('Ctrl Pts',(-48.706329375,28.437500006828,-1.8898197019151E-14));
#13731=CARTESIAN_POINT('Ctrl Pts',(-46.,60.,0.));
#13732=CARTESIAN_POINT('Ctrl Pts',(-46.,59.7916666666667,-12.3256628518316));
#13733=CARTESIAN_POINT('Ctrl Pts',(-39.8371685740842,59.5833333333333,-23.));
#13734=CARTESIAN_POINT('Ctrl Pts',(-33.6743371481684,59.375,-33.6743371481684));
#13735=CARTESIAN_POINT('Ctrl Pts',(-23.,59.1666666666667,-39.8371685740842));
#13736=CARTESIAN_POINT('Ctrl Pts',(-12.3256628518317,58.9583333333333,-46.));
#13737=CARTESIAN_POINT('Ctrl Pts',(-2.81668763803891E-15,58.75,-46.));
#13738=CARTESIAN_POINT('Ctrl Pts',(12.3256628518316,58.5416666666667,-46.));
#13739=CARTESIAN_POINT('Ctrl Pts',(23.,58.3333333333333,-39.8371685740842));
#13740=CARTESIAN_POINT('Ctrl Pts',(33.6743371481683,58.125,-33.6743371481684));
#13741=CARTESIAN_POINT('Ctrl Pts',(39.8371685740842,57.9166666666667,-23.));
#13742=CARTESIAN_POINT('Ctrl Pts',(46.,57.7083333333333,-12.3256628518317));
#13743=CARTESIAN_POINT('Ctrl Pts',(46.,57.5,-5.63337527607782E-15));
#13744=CARTESIAN_POINT('Ctrl Pts',(46.,57.2916666666667,12.3256628518316));
#13745=CARTESIAN_POINT('Ctrl Pts',(39.8371685740842,57.0833333333333,23.));
#13746=CARTESIAN_POINT('Ctrl Pts',(33.6743371481684,56.875,33.6743371481683));
#13747=CARTESIAN_POINT('Ctrl Pts',(23.,56.6666666666667,39.8371685740842));
#13748=CARTESIAN_POINT('Ctrl Pts',(12.3256628518317,56.4583333333333,46.));
#13749=CARTESIAN_POINT('Ctrl Pts',(8.45006291411674E-15,56.25,46.));
#13750=CARTESIAN_POINT('Ctrl Pts',(-12.3256628518316,56.0416666666667,46.));
#13751=CARTESIAN_POINT('Ctrl Pts',(-23.,55.8333333333333,39.8371685740842));
#13752=CARTESIAN_POINT('Ctrl Pts',(-33.6743371481683,55.625,33.6743371481684));
#13753=CARTESIAN_POINT('Ctrl Pts',(-39.8371685740842,55.4166666666667,23.));
#13754=CARTESIAN_POINT('Ctrl Pts',(-46.,55.2083333333333,12.3256628518317));
#13755=CARTESIAN_POINT('Ctrl Pts',(-46.,55.,0.));
#13756=CARTESIAN_POINT('Ctrl Pts',(-46.,54.7916666666667,-12.3256628518316));
#13757=CARTESIAN_POINT('Ctrl Pts',(-39.8371685740842,54.5833333333333,-23.));
#13758=CARTESIAN_POINT('Ctrl Pts',(-33.6743371481684,54.375,-33.6743371481684));
#13759=CARTESIAN_POINT('Ctrl Pts',(-23.,54.1666666666667,-39.8371685740842));
#13760=CARTESIAN_POINT('Ctrl Pts',(-12.3256628518317,53.9583333333333,-46.));
#13761=CARTESIAN_POINT('Ctrl Pts',(-2.81668763803891E-15,53.75,-46.));
#13762=CARTESIAN_POINT('Ctrl Pts',(12.3256628518316,53.5416666666667,-46.));
#13763=CARTESIAN_POINT('Ctrl Pts',(23.,53.3333333333333,-39.8371685740842));
#13764=CARTESIAN_POINT('Ctrl Pts',(33.6743371481683,53.125,-33.6743371481684));
#13765=CARTESIAN_POINT('Ctrl Pts',(39.8371685740842,52.9166666666667,-23.));
#13766=CARTESIAN_POINT('Ctrl Pts',(46.,52.7083333333333,-12.3256628518317));
#13767=CARTESIAN_POINT('Ctrl Pts',(46.,52.5,-5.63337527607782E-15));
#13768=CARTESIAN_POINT('Ctrl Pts',(46.,52.2916666666667,12.3256628518316));
#13769=CARTESIAN_POINT('Ctrl Pts',(39.8371685740842,52.0833333333333,23.));
#13770=CARTESIAN_POINT('Ctrl Pts',(33.6743371481684,51.875,33.6743371481683));
#13771=CARTESIAN_POINT('Ctrl Pts',(23.,51.6666666666667,39.8371685740842));
#13772=CARTESIAN_POINT('Ctrl Pts',(12.3256628518317,51.4583333333333,46.));
#13773=CARTESIAN_POINT('Ctrl Pts',(8.45006291411674E-15,51.25,46.));
#13774=CARTESIAN_POINT('Ctrl Pts',(-12.3256628518316,51.0416666666667,46.));
#13775=CARTESIAN_POINT('Ctrl Pts',(-23.,50.8333333333333,39.8371685740842));
#13776=CARTESIAN_POINT('Ctrl Pts',(-33.6743371481683,50.625,33.6743371481684));
#13777=CARTESIAN_POINT('Ctrl Pts',(-39.8371685740842,50.4166666666667,23.));
#13778=CARTESIAN_POINT('Ctrl Pts',(-46.,50.2083333333333,12.3256628518317));
#13779=CARTESIAN_POINT('Ctrl Pts',(-46.,50.,0.));
#13780=CARTESIAN_POINT('Ctrl Pts',(-46.,49.7916666666667,-12.3256628518316));
#13781=CARTESIAN_POINT('Ctrl Pts',(-39.8371685740842,49.5833333333333,-23.));
#13782=CARTESIAN_POINT('Ctrl Pts',(-33.6743371481684,49.375,-33.6743371481684));
#13783=CARTESIAN_POINT('Ctrl Pts',(-23.,49.1666666666667,-39.8371685740842));
#13784=CARTESIAN_POINT('Ctrl Pts',(-12.3256628518317,48.9583333333333,-46.));
#13785=CARTESIAN_POINT('Ctrl Pts',(-2.81668763803891E-15,48.75,-46.));
#13786=CARTESIAN_POINT('Ctrl Pts',(12.3256628518316,48.5416666666667,-46.));
#13787=CARTESIAN_POINT('Ctrl Pts',(23.,48.3333333333333,-39.8371685740842));
#13788=CARTESIAN_POINT('Ctrl Pts',(33.6743371481683,48.125,-33.6743371481684));
#13789=CARTESIAN_POINT('Ctrl Pts',(39.8371685740842,47.9166666666667,-23.));
#13790=CARTESIAN_POINT('Ctrl Pts',(46.,47.7083333333333,-12.3256628518317));
#13791=CARTESIAN_POINT('Ctrl Pts',(46.,47.5,-5.63337527607782E-15));
#13792=CARTESIAN_POINT('Ctrl Pts',(46.,47.2916666666667,12.3256628518316));
#13793=CARTESIAN_POINT('Ctrl Pts',(39.8371685740842,47.0833333333333,23.));
#13794=CARTESIAN_POINT('Ctrl Pts',(33.6743371481684,46.875,33.6743371481683));
#13795=CARTESIAN_POINT('Ctrl Pts',(23.,46.6666666666667,39.8371685740842));
#13796=CARTESIAN_POINT('Ctrl Pts',(12.3256628518317,46.4583333333333,46.));
#13797=CARTESIAN_POINT('Ctrl Pts',(8.45006291411674E-15,46.25,46.));
#13798=CARTESIAN_POINT('Ctrl Pts',(-12.3256628518316,46.0416666666667,46.));
#13799=CARTESIAN_POINT('Ctrl Pts',(-23.,45.8333333333333,39.8371685740842));
#13800=CARTESIAN_POINT('Ctrl Pts',(-33.6743371481683,45.625,33.6743371481684));
#13801=CARTESIAN_POINT('Ctrl Pts',(-39.8371685740842,45.4166666666667,23.));
#13802=CARTESIAN_POINT('Ctrl Pts',(-46.,45.2083333333333,12.3256628518317));
#13803=CARTESIAN_POINT('Ctrl Pts',(-46.,45.,0.));
#13804=CARTESIAN_POINT('Ctrl Pts',(-46.,44.7916666666667,-12.3256628518316));
#13805=CARTESIAN_POINT('Ctrl Pts',(-39.8371685740842,44.5833333333333,-23.));
#13806=CARTESIAN_POINT('Ctrl Pts',(-33.6743371481684,44.375,-33.6743371481684));
#13807=CARTESIAN_POINT('Ctrl Pts',(-23.,44.1666666666667,-39.8371685740842));
#13808=CARTESIAN_POINT('Ctrl Pts',(-12.3256628518317,43.9583333333333,-46.));
#13809=CARTESIAN_POINT('Ctrl Pts',(-2.81668763803891E-15,43.75,-46.));
#13810=CARTESIAN_POINT('Ctrl Pts',(12.3256628518316,43.5416666666667,-46.));
#13811=CARTESIAN_POINT('Ctrl Pts',(23.,43.3333333333333,-39.8371685740842));
#13812=CARTESIAN_POINT('Ctrl Pts',(33.6743371481683,43.125,-33.6743371481684));
#13813=CARTESIAN_POINT('Ctrl Pts',(39.8371685740842,42.9166666666667,-23.));
#13814=CARTESIAN_POINT('Ctrl Pts',(46.,42.7083333333333,-12.3256628518317));
#13815=CARTESIAN_POINT('Ctrl Pts',(46.,42.5,-5.63337527607782E-15));
#13816=CARTESIAN_POINT('Ctrl Pts',(46.,42.2916666666667,12.3256628518316));
#13817=CARTESIAN_POINT('Ctrl Pts',(39.8371685740842,42.0833333333333,23.));
#13818=CARTESIAN_POINT('Ctrl Pts',(33.6743371481684,41.875,33.6743371481683));
#13819=CARTESIAN_POINT('Ctrl Pts',(23.,41.6666666666667,39.8371685740842));
#13820=CARTESIAN_POINT('Ctrl Pts',(12.3256628518317,41.4583333333333,46.));
#13821=CARTESIAN_POINT('Ctrl Pts',(8.45006291411674E-15,41.25,46.));
#13822=CARTESIAN_POINT('Ctrl Pts',(-12.3256628518316,41.0416666666667,46.));
#13823=CARTESIAN_POINT('Ctrl Pts',(-23.,40.8333333333333,39.8371685740842));
#13824=CARTESIAN_POINT('Ctrl Pts',(-33.6743371481683,40.625,33.6743371481684));
#13825=CARTESIAN_POINT('Ctrl Pts',(-39.8371685740842,40.4166666666667,23.));
#13826=CARTESIAN_POINT('Ctrl Pts',(-46.,40.2083333333333,12.3256628518317));
#13827=CARTESIAN_POINT('Ctrl Pts',(-46.,40.,0.));
#13828=CARTESIAN_POINT('Ctrl Pts',(-46.,39.7916666666667,-12.3256628518316));
#13829=CARTESIAN_POINT('Ctrl Pts',(-39.8371685740842,39.5833333333333,-23.));
#13830=CARTESIAN_POINT('Ctrl Pts',(-33.6743371481684,39.375,-33.6743371481684));
#13831=CARTESIAN_POINT('Ctrl Pts',(-23.,39.1666666666667,-39.8371685740842));
#13832=CARTESIAN_POINT('Ctrl Pts',(-12.3256628518317,38.9583333333333,-46.));
#13833=CARTESIAN_POINT('Ctrl Pts',(-2.81668763803891E-15,38.75,-46.));
#13834=CARTESIAN_POINT('Ctrl Pts',(12.3256628518316,38.5416666666667,-46.));
#13835=CARTESIAN_POINT('Ctrl Pts',(23.,38.3333333333333,-39.8371685740842));
#13836=CARTESIAN_POINT('Ctrl Pts',(33.6743371481683,38.125,-33.6743371481684));
#13837=CARTESIAN_POINT('Ctrl Pts',(39.8371685740842,37.9166666666667,-23.));
#13838=CARTESIAN_POINT('Ctrl Pts',(46.,37.7083333333333,-12.3256628518317));
#13839=CARTESIAN_POINT('Ctrl Pts',(46.,37.5,-5.63337527607782E-15));
#13840=CARTESIAN_POINT('Ctrl Pts',(46.,37.2916666666667,12.3256628518316));
#13841=CARTESIAN_POINT('Ctrl Pts',(39.8371685740842,37.0833333333333,23.));
#13842=CARTESIAN_POINT('Ctrl Pts',(33.6743371481684,36.875,33.6743371481683));
#13843=CARTESIAN_POINT('Ctrl Pts',(23.,36.6666666666667,39.8371685740842));
#13844=CARTESIAN_POINT('Ctrl Pts',(12.3256628518317,36.4583333333333,46.));
#13845=CARTESIAN_POINT('Ctrl Pts',(8.45006291411674E-15,36.25,46.));
#13846=CARTESIAN_POINT('Ctrl Pts',(-12.3256628518316,36.0416666666667,46.));
#13847=CARTESIAN_POINT('Ctrl Pts',(-23.,35.8333333333333,39.8371685740842));
#13848=CARTESIAN_POINT('Ctrl Pts',(-33.6743371481683,35.625,33.6743371481684));
#13849=CARTESIAN_POINT('Ctrl Pts',(-39.8371685740842,35.4166666666667,23.));
#13850=CARTESIAN_POINT('Ctrl Pts',(-46.,35.2083333333333,12.3256628518317));
#13851=CARTESIAN_POINT('Ctrl Pts',(-46.,35.,0.));
#13852=CARTESIAN_POINT('Ctrl Pts',(-46.,34.7916666666667,-12.3256628518316));
#13853=CARTESIAN_POINT('Ctrl Pts',(-39.8371685740842,34.5833333333333,-23.));
#13854=CARTESIAN_POINT('Ctrl Pts',(-33.6743371481684,34.375,-33.6743371481684));
#13855=CARTESIAN_POINT('Ctrl Pts',(-23.,34.1666666666667,-39.8371685740842));
#13856=CARTESIAN_POINT('Ctrl Pts',(-12.3256628518317,33.9583333333333,-46.));
#13857=CARTESIAN_POINT('Ctrl Pts',(-2.81668763803891E-15,33.75,-46.));
#13858=CARTESIAN_POINT('Ctrl Pts',(12.3256628518316,33.5416666666667,-46.));
#13859=CARTESIAN_POINT('Ctrl Pts',(23.,33.3333333333333,-39.8371685740842));
#13860=CARTESIAN_POINT('Ctrl Pts',(33.6743371481683,33.125,-33.6743371481684));
#13861=CARTESIAN_POINT('Ctrl Pts',(39.8371685740842,32.9166666666667,-23.));
#13862=CARTESIAN_POINT('Ctrl Pts',(46.,32.7083333333333,-12.3256628518317));
#13863=CARTESIAN_POINT('Ctrl Pts',(46.,32.5,-5.63337527607782E-15));
#13864=CARTESIAN_POINT('Ctrl Pts',(46.,32.2916666666667,12.3256628518316));
#13865=CARTESIAN_POINT('Ctrl Pts',(39.8371685740842,32.0833333333333,23.));
#13866=CARTESIAN_POINT('Ctrl Pts',(33.6743371481684,31.875,33.6743371481683));
#13867=CARTESIAN_POINT('Ctrl Pts',(23.,31.6666666666667,39.8371685740842));
#13868=CARTESIAN_POINT('Ctrl Pts',(12.3256628518317,31.4583333333333,46.));
#13869=CARTESIAN_POINT('Ctrl Pts',(8.45006291411674E-15,31.25,46.));
#13870=CARTESIAN_POINT('Ctrl Pts',(-12.3256628518316,31.0416666666667,46.));
#13871=CARTESIAN_POINT('Ctrl Pts',(-23.,30.8333333333333,39.8371685740842));
#13872=CARTESIAN_POINT('Ctrl Pts',(-33.6743371481683,30.625,33.6743371481684));
#13873=CARTESIAN_POINT('Ctrl Pts',(-39.8371685740842,30.4166666666667,23.));
#13874=CARTESIAN_POINT('Ctrl Pts',(-46.,30.2083333333333,12.3256628518317));
#13875=CARTESIAN_POINT('Ctrl Pts',(-46.,30.,0.));
#13876=CARTESIAN_POINT('',(-48.3871149493437,58.4400045958969,-4.33048599679673));
#13877=CARTESIAN_POINT('',(-48.5134353784345,58.3675463684955,-4.33048599679673));
#13878=CARTESIAN_POINT('',(-4.32456003949879,57.3301814056101,-48.3876449370521));
#13879=CARTESIAN_POINT('Ctrl Pts',(-48.3871149493437,58.4400045958969,-4.33048599679673));
#13880=CARTESIAN_POINT('Ctrl Pts',(-47.4315944011671,58.2650323891532,-15.0070896471195));
#13881=CARTESIAN_POINT('Ctrl Pts',(-42.0719562365133,58.0934748917139,-24.2902552584851));
#13882=CARTESIAN_POINT('Ctrl Pts',(-35.5634019560564,57.8851415583806,-35.5634019560564));
#13883=CARTESIAN_POINT('Ctrl Pts',(-24.2902552584851,57.6768082250473,-42.0719562365133));
#13884=CARTESIAN_POINT('Ctrl Pts',(-15.0043879255857,57.5052007984562,-47.4331542408219));
#13885=CARTESIAN_POINT('Ctrl Pts',(-4.32456003949879,57.3301814056101,-48.3876449370521));
#13886=CARTESIAN_POINT('',(-4.32456003949879,57.3301814056101,-48.3876449370521));
#13887=CARTESIAN_POINT('Ctrl Pts',(-48.706329375,58.437500006828,-1.8898197019151E-14));
#13888=CARTESIAN_POINT('Ctrl Pts',(-48.706329375,58.2291666734946,-13.0508216223155));
#13889=CARTESIAN_POINT('Ctrl Pts',(-42.1809185638422,58.0208333401613,-24.3531646875));
#13890=CARTESIAN_POINT('Ctrl Pts',(-35.6555077526845,57.812500006828,-35.6555077526845));
#13891=CARTESIAN_POINT('Ctrl Pts',(-24.3531646875,57.6041666734946,-42.1809185638422));
#13892=CARTESIAN_POINT('Ctrl Pts',(-13.0508216223155,57.3958333401613,-48.706329375));
#13893=CARTESIAN_POINT('Ctrl Pts',(1.59157945007855E-14,57.187500006828,
-48.706329375));
#13894=CARTESIAN_POINT('Ctrl Pts',(13.0508216223155,56.9791666734946,-48.706329375));
#13895=CARTESIAN_POINT('Ctrl Pts',(24.3531646875,56.7708333401613,-42.1809185638422));
#13896=CARTESIAN_POINT('Ctrl Pts',(35.6555077526845,56.562500006828,-35.6555077526845));
#13897=CARTESIAN_POINT('Ctrl Pts',(42.1809185638422,56.3541666734946,-24.3531646875));
#13898=CARTESIAN_POINT('Ctrl Pts',(48.706329375,56.1458333401613,-13.0508216223155));
#13899=CARTESIAN_POINT('Ctrl Pts',(48.706329375,55.937500006828,1.293339198242E-14));
#13900=CARTESIAN_POINT('Ctrl Pts',(48.706329375,55.7291666734946,13.0508216223155));
#13901=CARTESIAN_POINT('Ctrl Pts',(42.1809185638422,55.5208333401613,24.3531646875));
#13902=CARTESIAN_POINT('Ctrl Pts',(35.6555077526845,55.312500006828,35.6555077526845));
#13903=CARTESIAN_POINT('Ctrl Pts',(24.3531646875,55.1041666734946,42.1809185638422));
#13904=CARTESIAN_POINT('Ctrl Pts',(13.0508216223155,54.8958333401613,48.706329375));
#13905=CARTESIAN_POINT('Ctrl Pts',(-9.95098946405443E-15,54.687500006828,
48.706329375));
#13906=CARTESIAN_POINT('Ctrl Pts',(-13.0508216223155,54.4791666734946,48.706329375));
#13907=CARTESIAN_POINT('Ctrl Pts',(-24.3531646875,54.2708333401613,42.1809185638423));
#13908=CARTESIAN_POINT('Ctrl Pts',(-35.6555077526845,54.062500006828,35.6555077526845));
#13909=CARTESIAN_POINT('Ctrl Pts',(-42.1809185638422,53.8541666734946,24.3531646875));
#13910=CARTESIAN_POINT('Ctrl Pts',(-48.706329375,53.6458333401613,13.0508216223155));
#13911=CARTESIAN_POINT('Ctrl Pts',(-48.706329375,53.437500006828,-1.8898197019151E-14));
#13912=CARTESIAN_POINT('Ctrl Pts',(-48.706329375,53.2291666734946,-13.0508216223155));
#13913=CARTESIAN_POINT('Ctrl Pts',(-42.1809185638422,53.0208333401613,-24.3531646875));
#13914=CARTESIAN_POINT('Ctrl Pts',(-35.6555077526845,52.812500006828,-35.6555077526845));
#13915=CARTESIAN_POINT('Ctrl Pts',(-24.3531646875,52.6041666734946,-42.1809185638422));
#13916=CARTESIAN_POINT('Ctrl Pts',(-13.0508216223155,52.3958333401613,-48.706329375));
#13917=CARTESIAN_POINT('Ctrl Pts',(1.59157945007855E-14,52.187500006828,
-48.706329375));
#13918=CARTESIAN_POINT('Ctrl Pts',(13.0508216223155,51.9791666734946,-48.706329375));
#13919=CARTESIAN_POINT('Ctrl Pts',(24.3531646875,51.7708333401613,-42.1809185638422));
#13920=CARTESIAN_POINT('Ctrl Pts',(35.6555077526845,51.562500006828,-35.6555077526845));
#13921=CARTESIAN_POINT('Ctrl Pts',(42.1809185638422,51.3541666734946,-24.3531646875));
#13922=CARTESIAN_POINT('Ctrl Pts',(48.706329375,51.1458333401613,-13.0508216223155));
#13923=CARTESIAN_POINT('Ctrl Pts',(48.706329375,50.937500006828,1.293339198242E-14));
#13924=CARTESIAN_POINT('Ctrl Pts',(48.706329375,50.7291666734946,13.0508216223155));
#13925=CARTESIAN_POINT('Ctrl Pts',(42.1809185638422,50.5208333401613,24.3531646875));
#13926=CARTESIAN_POINT('Ctrl Pts',(35.6555077526845,50.312500006828,35.6555077526845));
#13927=CARTESIAN_POINT('Ctrl Pts',(24.3531646875,50.1041666734946,42.1809185638422));
#13928=CARTESIAN_POINT('Ctrl Pts',(13.0508216223155,49.8958333401613,48.706329375));
#13929=CARTESIAN_POINT('Ctrl Pts',(-9.95098946405443E-15,49.687500006828,
48.706329375));
#13930=CARTESIAN_POINT('Ctrl Pts',(-13.0508216223155,49.4791666734946,48.706329375));
#13931=CARTESIAN_POINT('Ctrl Pts',(-24.3531646875,49.2708333401613,42.1809185638423));
#13932=CARTESIAN_POINT('Ctrl Pts',(-35.6555077526845,49.062500006828,35.6555077526845));
#13933=CARTESIAN_POINT('Ctrl Pts',(-42.1809185638422,48.8541666734946,24.3531646875));
#13934=CARTESIAN_POINT('Ctrl Pts',(-48.706329375,48.6458333401613,13.0508216223155));
#13935=CARTESIAN_POINT('Ctrl Pts',(-48.706329375,48.437500006828,-1.8898197019151E-14));
#13936=CARTESIAN_POINT('Ctrl Pts',(-48.706329375,48.2291666734946,-13.0508216223155));
#13937=CARTESIAN_POINT('Ctrl Pts',(-42.1809185638422,48.0208333401613,-24.3531646875));
#13938=CARTESIAN_POINT('Ctrl Pts',(-35.6555077526845,47.812500006828,-35.6555077526845));
#13939=CARTESIAN_POINT('Ctrl Pts',(-24.3531646875,47.6041666734946,-42.1809185638422));
#13940=CARTESIAN_POINT('Ctrl Pts',(-13.0508216223155,47.3958333401613,-48.706329375));
#13941=CARTESIAN_POINT('Ctrl Pts',(1.59157945007855E-14,47.187500006828,
-48.706329375));
#13942=CARTESIAN_POINT('Ctrl Pts',(13.0508216223155,46.9791666734946,-48.706329375));
#13943=CARTESIAN_POINT('Ctrl Pts',(24.3531646875,46.7708333401613,-42.1809185638422));
#13944=CARTESIAN_POINT('Ctrl Pts',(35.6555077526845,46.562500006828,-35.6555077526845));
#13945=CARTESIAN_POINT('Ctrl Pts',(42.1809185638422,46.3541666734946,-24.3531646875));
#13946=CARTESIAN_POINT('Ctrl Pts',(48.706329375,46.1458333401613,-13.0508216223155));
#13947=CARTESIAN_POINT('Ctrl Pts',(48.706329375,45.937500006828,1.293339198242E-14));
#13948=CARTESIAN_POINT('Ctrl Pts',(48.706329375,45.7291666734946,13.0508216223155));
#13949=CARTESIAN_POINT('Ctrl Pts',(42.1809185638422,45.5208333401613,24.3531646875));
#13950=CARTESIAN_POINT('Ctrl Pts',(35.6555077526845,45.312500006828,35.6555077526845));
#13951=CARTESIAN_POINT('Ctrl Pts',(24.3531646875,45.1041666734946,42.1809185638422));
#13952=CARTESIAN_POINT('Ctrl Pts',(13.0508216223155,44.8958333401613,48.706329375));
#13953=CARTESIAN_POINT('Ctrl Pts',(-9.95098946405443E-15,44.687500006828,
48.706329375));
#13954=CARTESIAN_POINT('Ctrl Pts',(-13.0508216223155,44.4791666734946,48.706329375));
#13955=CARTESIAN_POINT('Ctrl Pts',(-24.3531646875,44.2708333401613,42.1809185638423));
#13956=CARTESIAN_POINT('Ctrl Pts',(-35.6555077526845,44.062500006828,35.6555077526845));
#13957=CARTESIAN_POINT('Ctrl Pts',(-42.1809185638422,43.8541666734946,24.3531646875));
#13958=CARTESIAN_POINT('Ctrl Pts',(-48.706329375,43.6458333401613,13.0508216223155));
#13959=CARTESIAN_POINT('Ctrl Pts',(-48.706329375,43.437500006828,-1.8898197019151E-14));
#13960=CARTESIAN_POINT('Ctrl Pts',(-48.706329375,43.2291666734946,-13.0508216223155));
#13961=CARTESIAN_POINT('Ctrl Pts',(-42.1809185638422,43.0208333401613,-24.3531646875));
#13962=CARTESIAN_POINT('Ctrl Pts',(-35.6555077526845,42.812500006828,-35.6555077526845));
#13963=CARTESIAN_POINT('Ctrl Pts',(-24.3531646875,42.6041666734946,-42.1809185638422));
#13964=CARTESIAN_POINT('Ctrl Pts',(-13.0508216223155,42.3958333401613,-48.706329375));
#13965=CARTESIAN_POINT('Ctrl Pts',(1.59157945007855E-14,42.187500006828,
-48.706329375));
#13966=CARTESIAN_POINT('Ctrl Pts',(13.0508216223155,41.9791666734946,-48.706329375));
#13967=CARTESIAN_POINT('Ctrl Pts',(24.3531646875,41.7708333401613,-42.1809185638422));
#13968=CARTESIAN_POINT('Ctrl Pts',(35.6555077526845,41.562500006828,-35.6555077526845));
#13969=CARTESIAN_POINT('Ctrl Pts',(42.1809185638422,41.3541666734946,-24.3531646875));
#13970=CARTESIAN_POINT('Ctrl Pts',(48.706329375,41.1458333401613,-13.0508216223155));
#13971=CARTESIAN_POINT('Ctrl Pts',(48.706329375,40.937500006828,1.293339198242E-14));
#13972=CARTESIAN_POINT('Ctrl Pts',(48.706329375,40.7291666734946,13.0508216223155));
#13973=CARTESIAN_POINT('Ctrl Pts',(42.1809185638422,40.5208333401613,24.3531646875));
#13974=CARTESIAN_POINT('Ctrl Pts',(35.6555077526845,40.312500006828,35.6555077526845));
#13975=CARTESIAN_POINT('Ctrl Pts',(24.3531646875,40.1041666734946,42.1809185638422));
#13976=CARTESIAN_POINT('Ctrl Pts',(13.0508216223155,39.8958333401613,48.706329375));
#13977=CARTESIAN_POINT('Ctrl Pts',(-9.95098946405443E-15,39.687500006828,
48.706329375));
#13978=CARTESIAN_POINT('Ctrl Pts',(-13.0508216223155,39.4791666734946,48.706329375));
#13979=CARTESIAN_POINT('Ctrl Pts',(-24.3531646875,39.2708333401613,42.1809185638423));
#13980=CARTESIAN_POINT('Ctrl Pts',(-35.6555077526845,39.062500006828,35.6555077526845));
#13981=CARTESIAN_POINT('Ctrl Pts',(-42.1809185638422,38.8541666734946,24.3531646875));
#13982=CARTESIAN_POINT('Ctrl Pts',(-48.706329375,38.6458333401613,13.0508216223155));
#13983=CARTESIAN_POINT('Ctrl Pts',(-48.706329375,38.437500006828,-1.8898197019151E-14));
#13984=CARTESIAN_POINT('Ctrl Pts',(-48.706329375,38.2291666734946,-13.0508216223155));
#13985=CARTESIAN_POINT('Ctrl Pts',(-42.1809185638422,38.0208333401613,-24.3531646875));
#13986=CARTESIAN_POINT('Ctrl Pts',(-35.6555077526845,37.812500006828,-35.6555077526845));
#13987=CARTESIAN_POINT('Ctrl Pts',(-24.3531646875,37.6041666734946,-42.1809185638422));
#13988=CARTESIAN_POINT('Ctrl Pts',(-13.0508216223155,37.3958333401613,-48.706329375));
#13989=CARTESIAN_POINT('Ctrl Pts',(1.59157945007855E-14,37.187500006828,
-48.706329375));
#13990=CARTESIAN_POINT('Ctrl Pts',(13.0508216223155,36.9791666734946,-48.706329375));
#13991=CARTESIAN_POINT('Ctrl Pts',(24.3531646875,36.7708333401613,-42.1809185638422));
#13992=CARTESIAN_POINT('Ctrl Pts',(35.6555077526845,36.562500006828,-35.6555077526845));
#13993=CARTESIAN_POINT('Ctrl Pts',(42.1809185638422,36.3541666734946,-24.3531646875));
#13994=CARTESIAN_POINT('Ctrl Pts',(48.706329375,36.1458333401613,-13.0508216223155));
#13995=CARTESIAN_POINT('Ctrl Pts',(48.706329375,35.937500006828,1.293339198242E-14));
#13996=CARTESIAN_POINT('Ctrl Pts',(48.706329375,35.7291666734946,13.0508216223155));
#13997=CARTESIAN_POINT('Ctrl Pts',(42.1809185638422,35.5208333401613,24.3531646875));
#13998=CARTESIAN_POINT('Ctrl Pts',(35.6555077526845,35.312500006828,35.6555077526845));
#13999=CARTESIAN_POINT('Ctrl Pts',(24.3531646875,35.1041666734946,42.1809185638422));
#14000=CARTESIAN_POINT('Ctrl Pts',(13.0508216223155,34.8958333401613,48.706329375));
#14001=CARTESIAN_POINT('Ctrl Pts',(-9.95098946405443E-15,34.687500006828,
48.706329375));
#14002=CARTESIAN_POINT('Ctrl Pts',(-13.0508216223155,34.4791666734946,48.706329375));
#14003=CARTESIAN_POINT('Ctrl Pts',(-24.3531646875,34.2708333401613,42.1809185638423));
#14004=CARTESIAN_POINT('Ctrl Pts',(-35.6555077526845,34.062500006828,35.6555077526845));
#14005=CARTESIAN_POINT('Ctrl Pts',(-42.1809185638422,33.8541666734946,24.3531646875));
#14006=CARTESIAN_POINT('Ctrl Pts',(-48.706329375,33.6458333401613,13.0508216223155));
#14007=CARTESIAN_POINT('Ctrl Pts',(-48.706329375,33.437500006828,-1.8898197019151E-14));
#14008=CARTESIAN_POINT('Ctrl Pts',(-48.706329375,33.2291666734946,-13.0508216223155));
#14009=CARTESIAN_POINT('Ctrl Pts',(-42.1809185638422,33.0208333401613,-24.3531646875));
#14010=CARTESIAN_POINT('Ctrl Pts',(-35.6555077526845,32.812500006828,-35.6555077526845));
#14011=CARTESIAN_POINT('Ctrl Pts',(-24.3531646875,32.6041666734946,-42.1809185638422));
#14012=CARTESIAN_POINT('Ctrl Pts',(-13.0508216223155,32.3958333401613,-48.706329375));
#14013=CARTESIAN_POINT('Ctrl Pts',(1.59157945007855E-14,32.187500006828,
-48.706329375));
#14014=CARTESIAN_POINT('Ctrl Pts',(13.0508216223155,31.9791666734946,-48.706329375));
#14015=CARTESIAN_POINT('Ctrl Pts',(24.3531646875,31.7708333401613,-42.1809185638422));
#14016=CARTESIAN_POINT('Ctrl Pts',(35.6555077526845,31.562500006828,-35.6555077526845));
#14017=CARTESIAN_POINT('Ctrl Pts',(42.1809185638422,31.3541666734946,-24.3531646875));
#14018=CARTESIAN_POINT('Ctrl Pts',(48.706329375,31.1458333401613,-13.0508216223155));
#14019=CARTESIAN_POINT('Ctrl Pts',(48.706329375,30.937500006828,1.293339198242E-14));
#14020=CARTESIAN_POINT('Ctrl Pts',(48.706329375,30.7291666734946,13.0508216223155));
#14021=CARTESIAN_POINT('Ctrl Pts',(42.1809185638422,30.5208333401613,24.3531646875));
#14022=CARTESIAN_POINT('Ctrl Pts',(35.6555077526845,30.312500006828,35.6555077526845));
#14023=CARTESIAN_POINT('Ctrl Pts',(24.3531646875,30.1041666734946,42.1809185638422));
#14024=CARTESIAN_POINT('Ctrl Pts',(13.0508216223155,29.8958333401613,48.706329375));
#14025=CARTESIAN_POINT('Ctrl Pts',(-9.95098946405443E-15,29.687500006828,
48.706329375));
#14026=CARTESIAN_POINT('Ctrl Pts',(-13.0508216223155,29.4791666734946,48.706329375));
#14027=CARTESIAN_POINT('Ctrl Pts',(-24.3531646875,29.2708333401613,42.1809185638423));
#14028=CARTESIAN_POINT('Ctrl Pts',(-35.6555077526845,29.062500006828,35.6555077526845));
#14029=CARTESIAN_POINT('Ctrl Pts',(-42.1809185638422,28.8541666734946,24.3531646875));
#14030=CARTESIAN_POINT('Ctrl Pts',(-48.706329375,28.6458333401613,13.0508216223155));
#14031=CARTESIAN_POINT('Ctrl Pts',(-48.706329375,28.437500006828,-1.8898197019151E-14));
#14032=CARTESIAN_POINT('Ctrl Pts',(-46.,60.,0.));
#14033=CARTESIAN_POINT('Ctrl Pts',(-46.,59.7916666666667,-12.3256628518316));
#14034=CARTESIAN_POINT('Ctrl Pts',(-39.8371685740842,59.5833333333333,-23.));
#14035=CARTESIAN_POINT('Ctrl Pts',(-33.6743371481684,59.375,-33.6743371481684));
#14036=CARTESIAN_POINT('Ctrl Pts',(-23.,59.1666666666667,-39.8371685740842));
#14037=CARTESIAN_POINT('Ctrl Pts',(-12.3256628518317,58.9583333333333,-46.));
#14038=CARTESIAN_POINT('Ctrl Pts',(-2.81668763803891E-15,58.75,-46.));
#14039=CARTESIAN_POINT('Ctrl Pts',(12.3256628518316,58.5416666666667,-46.));
#14040=CARTESIAN_POINT('Ctrl Pts',(23.,58.3333333333333,-39.8371685740842));
#14041=CARTESIAN_POINT('Ctrl Pts',(33.6743371481683,58.125,-33.6743371481684));
#14042=CARTESIAN_POINT('Ctrl Pts',(39.8371685740842,57.9166666666667,-23.));
#14043=CARTESIAN_POINT('Ctrl Pts',(46.,57.7083333333333,-12.3256628518317));
#14044=CARTESIAN_POINT('Ctrl Pts',(46.,57.5,-5.63337527607782E-15));
#14045=CARTESIAN_POINT('Ctrl Pts',(46.,57.2916666666667,12.3256628518316));
#14046=CARTESIAN_POINT('Ctrl Pts',(39.8371685740842,57.0833333333333,23.));
#14047=CARTESIAN_POINT('Ctrl Pts',(33.6743371481684,56.875,33.6743371481683));
#14048=CARTESIAN_POINT('Ctrl Pts',(23.,56.6666666666667,39.8371685740842));
#14049=CARTESIAN_POINT('Ctrl Pts',(12.3256628518317,56.4583333333333,46.));
#14050=CARTESIAN_POINT('Ctrl Pts',(8.45006291411674E-15,56.25,46.));
#14051=CARTESIAN_POINT('Ctrl Pts',(-12.3256628518316,56.0416666666667,46.));
#14052=CARTESIAN_POINT('Ctrl Pts',(-23.,55.8333333333333,39.8371685740842));
#14053=CARTESIAN_POINT('Ctrl Pts',(-33.6743371481683,55.625,33.6743371481684));
#14054=CARTESIAN_POINT('Ctrl Pts',(-39.8371685740842,55.4166666666667,23.));
#14055=CARTESIAN_POINT('Ctrl Pts',(-46.,55.2083333333333,12.3256628518317));
#14056=CARTESIAN_POINT('Ctrl Pts',(-46.,55.,0.));
#14057=CARTESIAN_POINT('Ctrl Pts',(-46.,54.7916666666667,-12.3256628518316));
#14058=CARTESIAN_POINT('Ctrl Pts',(-39.8371685740842,54.5833333333333,-23.));
#14059=CARTESIAN_POINT('Ctrl Pts',(-33.6743371481684,54.375,-33.6743371481684));
#14060=CARTESIAN_POINT('Ctrl Pts',(-23.,54.1666666666667,-39.8371685740842));
#14061=CARTESIAN_POINT('Ctrl Pts',(-12.3256628518317,53.9583333333333,-46.));
#14062=CARTESIAN_POINT('Ctrl Pts',(-2.81668763803891E-15,53.75,-46.));
#14063=CARTESIAN_POINT('Ctrl Pts',(12.3256628518316,53.5416666666667,-46.));
#14064=CARTESIAN_POINT('Ctrl Pts',(23.,53.3333333333333,-39.8371685740842));
#14065=CARTESIAN_POINT('Ctrl Pts',(33.6743371481683,53.125,-33.6743371481684));
#14066=CARTESIAN_POINT('Ctrl Pts',(39.8371685740842,52.9166666666667,-23.));
#14067=CARTESIAN_POINT('Ctrl Pts',(46.,52.7083333333333,-12.3256628518317));
#14068=CARTESIAN_POINT('Ctrl Pts',(46.,52.5,-5.63337527607782E-15));
#14069=CARTESIAN_POINT('Ctrl Pts',(46.,52.2916666666667,12.3256628518316));
#14070=CARTESIAN_POINT('Ctrl Pts',(39.8371685740842,52.0833333333333,23.));
#14071=CARTESIAN_POINT('Ctrl Pts',(33.6743371481684,51.875,33.6743371481683));
#14072=CARTESIAN_POINT('Ctrl Pts',(23.,51.6666666666667,39.8371685740842));
#14073=CARTESIAN_POINT('Ctrl Pts',(12.3256628518317,51.4583333333333,46.));
#14074=CARTESIAN_POINT('Ctrl Pts',(8.45006291411674E-15,51.25,46.));
#14075=CARTESIAN_POINT('Ctrl Pts',(-12.3256628518316,51.0416666666667,46.));
#14076=CARTESIAN_POINT('Ctrl Pts',(-23.,50.8333333333333,39.8371685740842));
#14077=CARTESIAN_POINT('Ctrl Pts',(-33.6743371481683,50.625,33.6743371481684));
#14078=CARTESIAN_POINT('Ctrl Pts',(-39.8371685740842,50.4166666666667,23.));
#14079=CARTESIAN_POINT('Ctrl Pts',(-46.,50.2083333333333,12.3256628518317));
#14080=CARTESIAN_POINT('Ctrl Pts',(-46.,50.,0.));
#14081=CARTESIAN_POINT('Ctrl Pts',(-46.,49.7916666666667,-12.3256628518316));
#14082=CARTESIAN_POINT('Ctrl Pts',(-39.8371685740842,49.5833333333333,-23.));
#14083=CARTESIAN_POINT('Ctrl Pts',(-33.6743371481684,49.375,-33.6743371481684));
#14084=CARTESIAN_POINT('Ctrl Pts',(-23.,49.1666666666667,-39.8371685740842));
#14085=CARTESIAN_POINT('Ctrl Pts',(-12.3256628518317,48.9583333333333,-46.));
#14086=CARTESIAN_POINT('Ctrl Pts',(-2.81668763803891E-15,48.75,-46.));
#14087=CARTESIAN_POINT('Ctrl Pts',(12.3256628518316,48.5416666666667,-46.));
#14088=CARTESIAN_POINT('Ctrl Pts',(23.,48.3333333333333,-39.8371685740842));
#14089=CARTESIAN_POINT('Ctrl Pts',(33.6743371481683,48.125,-33.6743371481684));
#14090=CARTESIAN_POINT('Ctrl Pts',(39.8371685740842,47.9166666666667,-23.));
#14091=CARTESIAN_POINT('Ctrl Pts',(46.,47.7083333333333,-12.3256628518317));
#14092=CARTESIAN_POINT('Ctrl Pts',(46.,47.5,-5.63337527607782E-15));
#14093=CARTESIAN_POINT('Ctrl Pts',(46.,47.2916666666667,12.3256628518316));
#14094=CARTESIAN_POINT('Ctrl Pts',(39.8371685740842,47.0833333333333,23.));
#14095=CARTESIAN_POINT('Ctrl Pts',(33.6743371481684,46.875,33.6743371481683));
#14096=CARTESIAN_POINT('Ctrl Pts',(23.,46.6666666666667,39.8371685740842));
#14097=CARTESIAN_POINT('Ctrl Pts',(12.3256628518317,46.4583333333333,46.));
#14098=CARTESIAN_POINT('Ctrl Pts',(8.45006291411674E-15,46.25,46.));
#14099=CARTESIAN_POINT('Ctrl Pts',(-12.3256628518316,46.0416666666667,46.));
#14100=CARTESIAN_POINT('Ctrl Pts',(-23.,45.8333333333333,39.8371685740842));
#14101=CARTESIAN_POINT('Ctrl Pts',(-33.6743371481683,45.625,33.6743371481684));
#14102=CARTESIAN_POINT('Ctrl Pts',(-39.8371685740842,45.4166666666667,23.));
#14103=CARTESIAN_POINT('Ctrl Pts',(-46.,45.2083333333333,12.3256628518317));
#14104=CARTESIAN_POINT('Ctrl Pts',(-46.,45.,0.));
#14105=CARTESIAN_POINT('Ctrl Pts',(-46.,44.7916666666667,-12.3256628518316));
#14106=CARTESIAN_POINT('Ctrl Pts',(-39.8371685740842,44.5833333333333,-23.));
#14107=CARTESIAN_POINT('Ctrl Pts',(-33.6743371481684,44.375,-33.6743371481684));
#14108=CARTESIAN_POINT('Ctrl Pts',(-23.,44.1666666666667,-39.8371685740842));
#14109=CARTESIAN_POINT('Ctrl Pts',(-12.3256628518317,43.9583333333333,-46.));
#14110=CARTESIAN_POINT('Ctrl Pts',(-2.81668763803891E-15,43.75,-46.));
#14111=CARTESIAN_POINT('Ctrl Pts',(12.3256628518316,43.5416666666667,-46.));
#14112=CARTESIAN_POINT('Ctrl Pts',(23.,43.3333333333333,-39.8371685740842));
#14113=CARTESIAN_POINT('Ctrl Pts',(33.6743371481683,43.125,-33.6743371481684));
#14114=CARTESIAN_POINT('Ctrl Pts',(39.8371685740842,42.9166666666667,-23.));
#14115=CARTESIAN_POINT('Ctrl Pts',(46.,42.7083333333333,-12.3256628518317));
#14116=CARTESIAN_POINT('Ctrl Pts',(46.,42.5,-5.63337527607782E-15));
#14117=CARTESIAN_POINT('Ctrl Pts',(46.,42.2916666666667,12.3256628518316));
#14118=CARTESIAN_POINT('Ctrl Pts',(39.8371685740842,42.0833333333333,23.));
#14119=CARTESIAN_POINT('Ctrl Pts',(33.6743371481684,41.875,33.6743371481683));
#14120=CARTESIAN_POINT('Ctrl Pts',(23.,41.6666666666667,39.8371685740842));
#14121=CARTESIAN_POINT('Ctrl Pts',(12.3256628518317,41.4583333333333,46.));
#14122=CARTESIAN_POINT('Ctrl Pts',(8.45006291411674E-15,41.25,46.));
#14123=CARTESIAN_POINT('Ctrl Pts',(-12.3256628518316,41.0416666666667,46.));
#14124=CARTESIAN_POINT('Ctrl Pts',(-23.,40.8333333333333,39.8371685740842));
#14125=CARTESIAN_POINT('Ctrl Pts',(-33.6743371481683,40.625,33.6743371481684));
#14126=CARTESIAN_POINT('Ctrl Pts',(-39.8371685740842,40.4166666666667,23.));
#14127=CARTESIAN_POINT('Ctrl Pts',(-46.,40.2083333333333,12.3256628518317));
#14128=CARTESIAN_POINT('Ctrl Pts',(-46.,40.,0.));
#14129=CARTESIAN_POINT('Ctrl Pts',(-46.,39.7916666666667,-12.3256628518316));
#14130=CARTESIAN_POINT('Ctrl Pts',(-39.8371685740842,39.5833333333333,-23.));
#14131=CARTESIAN_POINT('Ctrl Pts',(-33.6743371481684,39.375,-33.6743371481684));
#14132=CARTESIAN_POINT('Ctrl Pts',(-23.,39.1666666666667,-39.8371685740842));
#14133=CARTESIAN_POINT('Ctrl Pts',(-12.3256628518317,38.9583333333333,-46.));
#14134=CARTESIAN_POINT('Ctrl Pts',(-2.81668763803891E-15,38.75,-46.));
#14135=CARTESIAN_POINT('Ctrl Pts',(12.3256628518316,38.5416666666667,-46.));
#14136=CARTESIAN_POINT('Ctrl Pts',(23.,38.3333333333333,-39.8371685740842));
#14137=CARTESIAN_POINT('Ctrl Pts',(33.6743371481683,38.125,-33.6743371481684));
#14138=CARTESIAN_POINT('Ctrl Pts',(39.8371685740842,37.9166666666667,-23.));
#14139=CARTESIAN_POINT('Ctrl Pts',(46.,37.7083333333333,-12.3256628518317));
#14140=CARTESIAN_POINT('Ctrl Pts',(46.,37.5,-5.63337527607782E-15));
#14141=CARTESIAN_POINT('Ctrl Pts',(46.,37.2916666666667,12.3256628518316));
#14142=CARTESIAN_POINT('Ctrl Pts',(39.8371685740842,37.0833333333333,23.));
#14143=CARTESIAN_POINT('Ctrl Pts',(33.6743371481684,36.875,33.6743371481683));
#14144=CARTESIAN_POINT('Ctrl Pts',(23.,36.6666666666667,39.8371685740842));
#14145=CARTESIAN_POINT('Ctrl Pts',(12.3256628518317,36.4583333333333,46.));
#14146=CARTESIAN_POINT('Ctrl Pts',(8.45006291411674E-15,36.25,46.));
#14147=CARTESIAN_POINT('Ctrl Pts',(-12.3256628518316,36.0416666666667,46.));
#14148=CARTESIAN_POINT('Ctrl Pts',(-23.,35.8333333333333,39.8371685740842));
#14149=CARTESIAN_POINT('Ctrl Pts',(-33.6743371481683,35.625,33.6743371481684));
#14150=CARTESIAN_POINT('Ctrl Pts',(-39.8371685740842,35.4166666666667,23.));
#14151=CARTESIAN_POINT('Ctrl Pts',(-46.,35.2083333333333,12.3256628518317));
#14152=CARTESIAN_POINT('Ctrl Pts',(-46.,35.,0.));
#14153=CARTESIAN_POINT('Ctrl Pts',(-46.,34.7916666666667,-12.3256628518316));
#14154=CARTESIAN_POINT('Ctrl Pts',(-39.8371685740842,34.5833333333333,-23.));
#14155=CARTESIAN_POINT('Ctrl Pts',(-33.6743371481684,34.375,-33.6743371481684));
#14156=CARTESIAN_POINT('Ctrl Pts',(-23.,34.1666666666667,-39.8371685740842));
#14157=CARTESIAN_POINT('Ctrl Pts',(-12.3256628518317,33.9583333333333,-46.));
#14158=CARTESIAN_POINT('Ctrl Pts',(-2.81668763803891E-15,33.75,-46.));
#14159=CARTESIAN_POINT('Ctrl Pts',(12.3256628518316,33.5416666666667,-46.));
#14160=CARTESIAN_POINT('Ctrl Pts',(23.,33.3333333333333,-39.8371685740842));
#14161=CARTESIAN_POINT('Ctrl Pts',(33.6743371481683,33.125,-33.6743371481684));
#14162=CARTESIAN_POINT('Ctrl Pts',(39.8371685740842,32.9166666666667,-23.));
#14163=CARTESIAN_POINT('Ctrl Pts',(46.,32.7083333333333,-12.3256628518317));
#14164=CARTESIAN_POINT('Ctrl Pts',(46.,32.5,-5.63337527607782E-15));
#14165=CARTESIAN_POINT('Ctrl Pts',(46.,32.2916666666667,12.3256628518316));
#14166=CARTESIAN_POINT('Ctrl Pts',(39.8371685740842,32.0833333333333,23.));
#14167=CARTESIAN_POINT('Ctrl Pts',(33.6743371481684,31.875,33.6743371481683));
#14168=CARTESIAN_POINT('Ctrl Pts',(23.,31.6666666666667,39.8371685740842));
#14169=CARTESIAN_POINT('Ctrl Pts',(12.3256628518317,31.4583333333333,46.));
#14170=CARTESIAN_POINT('Ctrl Pts',(8.45006291411674E-15,31.25,46.));
#14171=CARTESIAN_POINT('Ctrl Pts',(-12.3256628518316,31.0416666666667,46.));
#14172=CARTESIAN_POINT('Ctrl Pts',(-23.,30.8333333333333,39.8371685740842));
#14173=CARTESIAN_POINT('Ctrl Pts',(-33.6743371481683,30.625,33.6743371481684));
#14174=CARTESIAN_POINT('Ctrl Pts',(-39.8371685740842,30.4166666666667,23.));
#14175=CARTESIAN_POINT('Ctrl Pts',(-46.,30.2083333333333,12.3256628518317));
#14176=CARTESIAN_POINT('Ctrl Pts',(-46.,30.,0.));
#14177=CARTESIAN_POINT('Origin',(4513.80899678944,-7900.15854878091,-4.33048595875475));
#14178=CARTESIAN_POINT('Ctrl Pts',(-4.32456003949879,53.8240181593938,-45.7962681936506));
#14179=CARTESIAN_POINT('Ctrl Pts',(-4.32456003949879,53.6905125468623,-46.0278818021281));
#14180=CARTESIAN_POINT('Ctrl Pts',(-4.32456003949875,53.4234964717135,-46.4911062234486));
#14181=CARTESIAN_POINT('Ctrl Pts',(-4.32456003949878,53.1564711191154,-46.954325296818));
#14182=CARTESIAN_POINT('Ctrl Pts',(-4.32456003949878,52.7677643029224,-47.6286149142205));
#14183=CARTESIAN_POINT('Ctrl Pts',(-4.32456003949881,52.5125642776457,-48.0712916022845));
#14184=CARTESIAN_POINT('Ctrl Pts',(-4.32456003949876,52.2573567866782,-48.5139639861634));
#14185=CARTESIAN_POINT('Ctrl Pts',(-48.706329375,58.437500006828,-1.8898197019151E-14));
#14186=CARTESIAN_POINT('Ctrl Pts',(-48.706329375,58.2291666734946,-13.0508216223155));
#14187=CARTESIAN_POINT('Ctrl Pts',(-42.1809185638422,58.0208333401613,-24.3531646875));
#14188=CARTESIAN_POINT('Ctrl Pts',(-35.6555077526845,57.812500006828,-35.6555077526845));
#14189=CARTESIAN_POINT('Ctrl Pts',(-24.3531646875,57.6041666734946,-42.1809185638422));
#14190=CARTESIAN_POINT('Ctrl Pts',(-13.0508216223155,57.3958333401613,-48.706329375));
#14191=CARTESIAN_POINT('Ctrl Pts',(1.59157945007855E-14,57.187500006828,
-48.706329375));
#14192=CARTESIAN_POINT('Ctrl Pts',(13.0508216223155,56.9791666734946,-48.706329375));
#14193=CARTESIAN_POINT('Ctrl Pts',(24.3531646875,56.7708333401613,-42.1809185638422));
#14194=CARTESIAN_POINT('Ctrl Pts',(35.6555077526845,56.562500006828,-35.6555077526845));
#14195=CARTESIAN_POINT('Ctrl Pts',(42.1809185638422,56.3541666734946,-24.3531646875));
#14196=CARTESIAN_POINT('Ctrl Pts',(48.706329375,56.1458333401613,-13.0508216223155));
#14197=CARTESIAN_POINT('Ctrl Pts',(48.706329375,55.937500006828,1.293339198242E-14));
#14198=CARTESIAN_POINT('Ctrl Pts',(48.706329375,55.7291666734946,13.0508216223155));
#14199=CARTESIAN_POINT('Ctrl Pts',(42.1809185638422,55.5208333401613,24.3531646875));
#14200=CARTESIAN_POINT('Ctrl Pts',(35.6555077526845,55.312500006828,35.6555077526845));
#14201=CARTESIAN_POINT('Ctrl Pts',(24.3531646875,55.1041666734946,42.1809185638422));
#14202=CARTESIAN_POINT('Ctrl Pts',(13.0508216223155,54.8958333401613,48.706329375));
#14203=CARTESIAN_POINT('Ctrl Pts',(-9.95098946405443E-15,54.687500006828,
48.706329375));
#14204=CARTESIAN_POINT('Ctrl Pts',(-13.0508216223155,54.4791666734946,48.706329375));
#14205=CARTESIAN_POINT('Ctrl Pts',(-24.3531646875,54.2708333401613,42.1809185638423));
#14206=CARTESIAN_POINT('Ctrl Pts',(-35.6555077526845,54.062500006828,35.6555077526845));
#14207=CARTESIAN_POINT('Ctrl Pts',(-42.1809185638422,53.8541666734946,24.3531646875));
#14208=CARTESIAN_POINT('Ctrl Pts',(-48.706329375,53.6458333401613,13.0508216223155));
#14209=CARTESIAN_POINT('Ctrl Pts',(-48.706329375,53.437500006828,-1.8898197019151E-14));
#14210=CARTESIAN_POINT('Ctrl Pts',(-48.706329375,53.2291666734946,-13.0508216223155));
#14211=CARTESIAN_POINT('Ctrl Pts',(-42.1809185638422,53.0208333401613,-24.3531646875));
#14212=CARTESIAN_POINT('Ctrl Pts',(-35.6555077526845,52.812500006828,-35.6555077526845));
#14213=CARTESIAN_POINT('Ctrl Pts',(-24.3531646875,52.6041666734946,-42.1809185638422));
#14214=CARTESIAN_POINT('Ctrl Pts',(-13.0508216223155,52.3958333401613,-48.706329375));
#14215=CARTESIAN_POINT('Ctrl Pts',(1.59157945007855E-14,52.187500006828,
-48.706329375));
#14216=CARTESIAN_POINT('Ctrl Pts',(13.0508216223155,51.9791666734946,-48.706329375));
#14217=CARTESIAN_POINT('Ctrl Pts',(24.3531646875,51.7708333401613,-42.1809185638422));
#14218=CARTESIAN_POINT('Ctrl Pts',(35.6555077526845,51.562500006828,-35.6555077526845));
#14219=CARTESIAN_POINT('Ctrl Pts',(42.1809185638422,51.3541666734946,-24.3531646875));
#14220=CARTESIAN_POINT('Ctrl Pts',(48.706329375,51.1458333401613,-13.0508216223155));
#14221=CARTESIAN_POINT('Ctrl Pts',(48.706329375,50.937500006828,1.293339198242E-14));
#14222=CARTESIAN_POINT('Ctrl Pts',(48.706329375,50.7291666734946,13.0508216223155));
#14223=CARTESIAN_POINT('Ctrl Pts',(42.1809185638422,50.5208333401613,24.3531646875));
#14224=CARTESIAN_POINT('Ctrl Pts',(35.6555077526845,50.312500006828,35.6555077526845));
#14225=CARTESIAN_POINT('Ctrl Pts',(24.3531646875,50.1041666734946,42.1809185638422));
#14226=CARTESIAN_POINT('Ctrl Pts',(13.0508216223155,49.8958333401613,48.706329375));
#14227=CARTESIAN_POINT('Ctrl Pts',(-9.95098946405443E-15,49.687500006828,
48.706329375));
#14228=CARTESIAN_POINT('Ctrl Pts',(-13.0508216223155,49.4791666734946,48.706329375));
#14229=CARTESIAN_POINT('Ctrl Pts',(-24.3531646875,49.2708333401613,42.1809185638423));
#14230=CARTESIAN_POINT('Ctrl Pts',(-35.6555077526845,49.062500006828,35.6555077526845));
#14231=CARTESIAN_POINT('Ctrl Pts',(-42.1809185638422,48.8541666734946,24.3531646875));
#14232=CARTESIAN_POINT('Ctrl Pts',(-48.706329375,48.6458333401613,13.0508216223155));
#14233=CARTESIAN_POINT('Ctrl Pts',(-48.706329375,48.437500006828,-1.8898197019151E-14));
#14234=CARTESIAN_POINT('Ctrl Pts',(-48.706329375,48.2291666734946,-13.0508216223155));
#14235=CARTESIAN_POINT('Ctrl Pts',(-42.1809185638422,48.0208333401613,-24.3531646875));
#14236=CARTESIAN_POINT('Ctrl Pts',(-35.6555077526845,47.812500006828,-35.6555077526845));
#14237=CARTESIAN_POINT('Ctrl Pts',(-24.3531646875,47.6041666734946,-42.1809185638422));
#14238=CARTESIAN_POINT('Ctrl Pts',(-13.0508216223155,47.3958333401613,-48.706329375));
#14239=CARTESIAN_POINT('Ctrl Pts',(1.59157945007855E-14,47.187500006828,
-48.706329375));
#14240=CARTESIAN_POINT('Ctrl Pts',(13.0508216223155,46.9791666734946,-48.706329375));
#14241=CARTESIAN_POINT('Ctrl Pts',(24.3531646875,46.7708333401613,-42.1809185638422));
#14242=CARTESIAN_POINT('Ctrl Pts',(35.6555077526845,46.562500006828,-35.6555077526845));
#14243=CARTESIAN_POINT('Ctrl Pts',(42.1809185638422,46.3541666734946,-24.3531646875));
#14244=CARTESIAN_POINT('Ctrl Pts',(48.706329375,46.1458333401613,-13.0508216223155));
#14245=CARTESIAN_POINT('Ctrl Pts',(48.706329375,45.937500006828,1.293339198242E-14));
#14246=CARTESIAN_POINT('Ctrl Pts',(48.706329375,45.7291666734946,13.0508216223155));
#14247=CARTESIAN_POINT('Ctrl Pts',(42.1809185638422,45.5208333401613,24.3531646875));
#14248=CARTESIAN_POINT('Ctrl Pts',(35.6555077526845,45.312500006828,35.6555077526845));
#14249=CARTESIAN_POINT('Ctrl Pts',(24.3531646875,45.1041666734946,42.1809185638422));
#14250=CARTESIAN_POINT('Ctrl Pts',(13.0508216223155,44.8958333401613,48.706329375));
#14251=CARTESIAN_POINT('Ctrl Pts',(-9.95098946405443E-15,44.687500006828,
48.706329375));
#14252=CARTESIAN_POINT('Ctrl Pts',(-13.0508216223155,44.4791666734946,48.706329375));
#14253=CARTESIAN_POINT('Ctrl Pts',(-24.3531646875,44.2708333401613,42.1809185638423));
#14254=CARTESIAN_POINT('Ctrl Pts',(-35.6555077526845,44.062500006828,35.6555077526845));
#14255=CARTESIAN_POINT('Ctrl Pts',(-42.1809185638422,43.8541666734946,24.3531646875));
#14256=CARTESIAN_POINT('Ctrl Pts',(-48.706329375,43.6458333401613,13.0508216223155));
#14257=CARTESIAN_POINT('Ctrl Pts',(-48.706329375,43.437500006828,-1.8898197019151E-14));
#14258=CARTESIAN_POINT('Ctrl Pts',(-48.706329375,43.2291666734946,-13.0508216223155));
#14259=CARTESIAN_POINT('Ctrl Pts',(-42.1809185638422,43.0208333401613,-24.3531646875));
#14260=CARTESIAN_POINT('Ctrl Pts',(-35.6555077526845,42.812500006828,-35.6555077526845));
#14261=CARTESIAN_POINT('Ctrl Pts',(-24.3531646875,42.6041666734946,-42.1809185638422));
#14262=CARTESIAN_POINT('Ctrl Pts',(-13.0508216223155,42.3958333401613,-48.706329375));
#14263=CARTESIAN_POINT('Ctrl Pts',(1.59157945007855E-14,42.187500006828,
-48.706329375));
#14264=CARTESIAN_POINT('Ctrl Pts',(13.0508216223155,41.9791666734946,-48.706329375));
#14265=CARTESIAN_POINT('Ctrl Pts',(24.3531646875,41.7708333401613,-42.1809185638422));
#14266=CARTESIAN_POINT('Ctrl Pts',(35.6555077526845,41.562500006828,-35.6555077526845));
#14267=CARTESIAN_POINT('Ctrl Pts',(42.1809185638422,41.3541666734946,-24.3531646875));
#14268=CARTESIAN_POINT('Ctrl Pts',(48.706329375,41.1458333401613,-13.0508216223155));
#14269=CARTESIAN_POINT('Ctrl Pts',(48.706329375,40.937500006828,1.293339198242E-14));
#14270=CARTESIAN_POINT('Ctrl Pts',(48.706329375,40.7291666734946,13.0508216223155));
#14271=CARTESIAN_POINT('Ctrl Pts',(42.1809185638422,40.5208333401613,24.3531646875));
#14272=CARTESIAN_POINT('Ctrl Pts',(35.6555077526845,40.312500006828,35.6555077526845));
#14273=CARTESIAN_POINT('Ctrl Pts',(24.3531646875,40.1041666734946,42.1809185638422));
#14274=CARTESIAN_POINT('Ctrl Pts',(13.0508216223155,39.8958333401613,48.706329375));
#14275=CARTESIAN_POINT('Ctrl Pts',(-9.95098946405443E-15,39.687500006828,
48.706329375));
#14276=CARTESIAN_POINT('Ctrl Pts',(-13.0508216223155,39.4791666734946,48.706329375));
#14277=CARTESIAN_POINT('Ctrl Pts',(-24.3531646875,39.2708333401613,42.1809185638423));
#14278=CARTESIAN_POINT('Ctrl Pts',(-35.6555077526845,39.062500006828,35.6555077526845));
#14279=CARTESIAN_POINT('Ctrl Pts',(-42.1809185638422,38.8541666734946,24.3531646875));
#14280=CARTESIAN_POINT('Ctrl Pts',(-48.706329375,38.6458333401613,13.0508216223155));
#14281=CARTESIAN_POINT('Ctrl Pts',(-48.706329375,38.437500006828,-1.8898197019151E-14));
#14282=CARTESIAN_POINT('Ctrl Pts',(-48.706329375,38.2291666734946,-13.0508216223155));
#14283=CARTESIAN_POINT('Ctrl Pts',(-42.1809185638422,38.0208333401613,-24.3531646875));
#14284=CARTESIAN_POINT('Ctrl Pts',(-35.6555077526845,37.812500006828,-35.6555077526845));
#14285=CARTESIAN_POINT('Ctrl Pts',(-24.3531646875,37.6041666734946,-42.1809185638422));
#14286=CARTESIAN_POINT('Ctrl Pts',(-13.0508216223155,37.3958333401613,-48.706329375));
#14287=CARTESIAN_POINT('Ctrl Pts',(1.59157945007855E-14,37.187500006828,
-48.706329375));
#14288=CARTESIAN_POINT('Ctrl Pts',(13.0508216223155,36.9791666734946,-48.706329375));
#14289=CARTESIAN_POINT('Ctrl Pts',(24.3531646875,36.7708333401613,-42.1809185638422));
#14290=CARTESIAN_POINT('Ctrl Pts',(35.6555077526845,36.562500006828,-35.6555077526845));
#14291=CARTESIAN_POINT('Ctrl Pts',(42.1809185638422,36.3541666734946,-24.3531646875));
#14292=CARTESIAN_POINT('Ctrl Pts',(48.706329375,36.1458333401613,-13.0508216223155));
#14293=CARTESIAN_POINT('Ctrl Pts',(48.706329375,35.937500006828,1.293339198242E-14));
#14294=CARTESIAN_POINT('Ctrl Pts',(48.706329375,35.7291666734946,13.0508216223155));
#14295=CARTESIAN_POINT('Ctrl Pts',(42.1809185638422,35.5208333401613,24.3531646875));
#14296=CARTESIAN_POINT('Ctrl Pts',(35.6555077526845,35.312500006828,35.6555077526845));
#14297=CARTESIAN_POINT('Ctrl Pts',(24.3531646875,35.1041666734946,42.1809185638422));
#14298=CARTESIAN_POINT('Ctrl Pts',(13.0508216223155,34.8958333401613,48.706329375));
#14299=CARTESIAN_POINT('Ctrl Pts',(-9.95098946405443E-15,34.687500006828,
48.706329375));
#14300=CARTESIAN_POINT('Ctrl Pts',(-13.0508216223155,34.4791666734946,48.706329375));
#14301=CARTESIAN_POINT('Ctrl Pts',(-24.3531646875,34.2708333401613,42.1809185638423));
#14302=CARTESIAN_POINT('Ctrl Pts',(-35.6555077526845,34.062500006828,35.6555077526845));
#14303=CARTESIAN_POINT('Ctrl Pts',(-42.1809185638422,33.8541666734946,24.3531646875));
#14304=CARTESIAN_POINT('Ctrl Pts',(-48.706329375,33.6458333401613,13.0508216223155));
#14305=CARTESIAN_POINT('Ctrl Pts',(-48.706329375,33.437500006828,-1.8898197019151E-14));
#14306=CARTESIAN_POINT('Ctrl Pts',(-48.706329375,33.2291666734946,-13.0508216223155));
#14307=CARTESIAN_POINT('Ctrl Pts',(-42.1809185638422,33.0208333401613,-24.3531646875));
#14308=CARTESIAN_POINT('Ctrl Pts',(-35.6555077526845,32.812500006828,-35.6555077526845));
#14309=CARTESIAN_POINT('Ctrl Pts',(-24.3531646875,32.6041666734946,-42.1809185638422));
#14310=CARTESIAN_POINT('Ctrl Pts',(-13.0508216223155,32.3958333401613,-48.706329375));
#14311=CARTESIAN_POINT('Ctrl Pts',(1.59157945007855E-14,32.187500006828,
-48.706329375));
#14312=CARTESIAN_POINT('Ctrl Pts',(13.0508216223155,31.9791666734946,-48.706329375));
#14313=CARTESIAN_POINT('Ctrl Pts',(24.3531646875,31.7708333401613,-42.1809185638422));
#14314=CARTESIAN_POINT('Ctrl Pts',(35.6555077526845,31.562500006828,-35.6555077526845));
#14315=CARTESIAN_POINT('Ctrl Pts',(42.1809185638422,31.3541666734946,-24.3531646875));
#14316=CARTESIAN_POINT('Ctrl Pts',(48.706329375,31.1458333401613,-13.0508216223155));
#14317=CARTESIAN_POINT('Ctrl Pts',(48.706329375,30.937500006828,1.293339198242E-14));
#14318=CARTESIAN_POINT('Ctrl Pts',(48.706329375,30.7291666734946,13.0508216223155));
#14319=CARTESIAN_POINT('Ctrl Pts',(42.1809185638422,30.5208333401613,24.3531646875));
#14320=CARTESIAN_POINT('Ctrl Pts',(35.6555077526845,30.312500006828,35.6555077526845));
#14321=CARTESIAN_POINT('Ctrl Pts',(24.3531646875,30.1041666734946,42.1809185638422));
#14322=CARTESIAN_POINT('Ctrl Pts',(13.0508216223155,29.8958333401613,48.706329375));
#14323=CARTESIAN_POINT('Ctrl Pts',(-9.95098946405443E-15,29.687500006828,
48.706329375));
#14324=CARTESIAN_POINT('Ctrl Pts',(-13.0508216223155,29.4791666734946,48.706329375));
#14325=CARTESIAN_POINT('Ctrl Pts',(-24.3531646875,29.2708333401613,42.1809185638423));
#14326=CARTESIAN_POINT('Ctrl Pts',(-35.6555077526845,29.062500006828,35.6555077526845));
#14327=CARTESIAN_POINT('Ctrl Pts',(-42.1809185638422,28.8541666734946,24.3531646875));
#14328=CARTESIAN_POINT('Ctrl Pts',(-48.706329375,28.6458333401613,13.0508216223155));
#14329=CARTESIAN_POINT('Ctrl Pts',(-48.706329375,28.437500006828,-1.8898197019151E-14));
#14330=CARTESIAN_POINT('Ctrl Pts',(-46.,60.,0.));
#14331=CARTESIAN_POINT('Ctrl Pts',(-46.,59.7916666666667,-12.3256628518316));
#14332=CARTESIAN_POINT('Ctrl Pts',(-39.8371685740842,59.5833333333333,-23.));
#14333=CARTESIAN_POINT('Ctrl Pts',(-33.6743371481684,59.375,-33.6743371481684));
#14334=CARTESIAN_POINT('Ctrl Pts',(-23.,59.1666666666667,-39.8371685740842));
#14335=CARTESIAN_POINT('Ctrl Pts',(-12.3256628518317,58.9583333333333,-46.));
#14336=CARTESIAN_POINT('Ctrl Pts',(-2.81668763803891E-15,58.75,-46.));
#14337=CARTESIAN_POINT('Ctrl Pts',(12.3256628518316,58.5416666666667,-46.));
#14338=CARTESIAN_POINT('Ctrl Pts',(23.,58.3333333333333,-39.8371685740842));
#14339=CARTESIAN_POINT('Ctrl Pts',(33.6743371481683,58.125,-33.6743371481684));
#14340=CARTESIAN_POINT('Ctrl Pts',(39.8371685740842,57.9166666666667,-23.));
#14341=CARTESIAN_POINT('Ctrl Pts',(46.,57.7083333333333,-12.3256628518317));
#14342=CARTESIAN_POINT('Ctrl Pts',(46.,57.5,-5.63337527607782E-15));
#14343=CARTESIAN_POINT('Ctrl Pts',(46.,57.2916666666667,12.3256628518316));
#14344=CARTESIAN_POINT('Ctrl Pts',(39.8371685740842,57.0833333333333,23.));
#14345=CARTESIAN_POINT('Ctrl Pts',(33.6743371481684,56.875,33.6743371481683));
#14346=CARTESIAN_POINT('Ctrl Pts',(23.,56.6666666666667,39.8371685740842));
#14347=CARTESIAN_POINT('Ctrl Pts',(12.3256628518317,56.4583333333333,46.));
#14348=CARTESIAN_POINT('Ctrl Pts',(8.45006291411674E-15,56.25,46.));
#14349=CARTESIAN_POINT('Ctrl Pts',(-12.3256628518316,56.0416666666667,46.));
#14350=CARTESIAN_POINT('Ctrl Pts',(-23.,55.8333333333333,39.8371685740842));
#14351=CARTESIAN_POINT('Ctrl Pts',(-33.6743371481683,55.625,33.6743371481684));
#14352=CARTESIAN_POINT('Ctrl Pts',(-39.8371685740842,55.4166666666667,23.));
#14353=CARTESIAN_POINT('Ctrl Pts',(-46.,55.2083333333333,12.3256628518317));
#14354=CARTESIAN_POINT('Ctrl Pts',(-46.,55.,0.));
#14355=CARTESIAN_POINT('Ctrl Pts',(-46.,54.7916666666667,-12.3256628518316));
#14356=CARTESIAN_POINT('Ctrl Pts',(-39.8371685740842,54.5833333333333,-23.));
#14357=CARTESIAN_POINT('Ctrl Pts',(-33.6743371481684,54.375,-33.6743371481684));
#14358=CARTESIAN_POINT('Ctrl Pts',(-23.,54.1666666666667,-39.8371685740842));
#14359=CARTESIAN_POINT('Ctrl Pts',(-12.3256628518317,53.9583333333333,-46.));
#14360=CARTESIAN_POINT('Ctrl Pts',(-2.81668763803891E-15,53.75,-46.));
#14361=CARTESIAN_POINT('Ctrl Pts',(12.3256628518316,53.5416666666667,-46.));
#14362=CARTESIAN_POINT('Ctrl Pts',(23.,53.3333333333333,-39.8371685740842));
#14363=CARTESIAN_POINT('Ctrl Pts',(33.6743371481683,53.125,-33.6743371481684));
#14364=CARTESIAN_POINT('Ctrl Pts',(39.8371685740842,52.9166666666667,-23.));
#14365=CARTESIAN_POINT('Ctrl Pts',(46.,52.7083333333333,-12.3256628518317));
#14366=CARTESIAN_POINT('Ctrl Pts',(46.,52.5,-5.63337527607782E-15));
#14367=CARTESIAN_POINT('Ctrl Pts',(46.,52.2916666666667,12.3256628518316));
#14368=CARTESIAN_POINT('Ctrl Pts',(39.8371685740842,52.0833333333333,23.));
#14369=CARTESIAN_POINT('Ctrl Pts',(33.6743371481684,51.875,33.6743371481683));
#14370=CARTESIAN_POINT('Ctrl Pts',(23.,51.6666666666667,39.8371685740842));
#14371=CARTESIAN_POINT('Ctrl Pts',(12.3256628518317,51.4583333333333,46.));
#14372=CARTESIAN_POINT('Ctrl Pts',(8.45006291411674E-15,51.25,46.));
#14373=CARTESIAN_POINT('Ctrl Pts',(-12.3256628518316,51.0416666666667,46.));
#14374=CARTESIAN_POINT('Ctrl Pts',(-23.,50.8333333333333,39.8371685740842));
#14375=CARTESIAN_POINT('Ctrl Pts',(-33.6743371481683,50.625,33.6743371481684));
#14376=CARTESIAN_POINT('Ctrl Pts',(-39.8371685740842,50.4166666666667,23.));
#14377=CARTESIAN_POINT('Ctrl Pts',(-46.,50.2083333333333,12.3256628518317));
#14378=CARTESIAN_POINT('Ctrl Pts',(-46.,50.,0.));
#14379=CARTESIAN_POINT('Ctrl Pts',(-46.,49.7916666666667,-12.3256628518316));
#14380=CARTESIAN_POINT('Ctrl Pts',(-39.8371685740842,49.5833333333333,-23.));
#14381=CARTESIAN_POINT('Ctrl Pts',(-33.6743371481684,49.375,-33.6743371481684));
#14382=CARTESIAN_POINT('Ctrl Pts',(-23.,49.1666666666667,-39.8371685740842));
#14383=CARTESIAN_POINT('Ctrl Pts',(-12.3256628518317,48.9583333333333,-46.));
#14384=CARTESIAN_POINT('Ctrl Pts',(-2.81668763803891E-15,48.75,-46.));
#14385=CARTESIAN_POINT('Ctrl Pts',(12.3256628518316,48.5416666666667,-46.));
#14386=CARTESIAN_POINT('Ctrl Pts',(23.,48.3333333333333,-39.8371685740842));
#14387=CARTESIAN_POINT('Ctrl Pts',(33.6743371481683,48.125,-33.6743371481684));
#14388=CARTESIAN_POINT('Ctrl Pts',(39.8371685740842,47.9166666666667,-23.));
#14389=CARTESIAN_POINT('Ctrl Pts',(46.,47.7083333333333,-12.3256628518317));
#14390=CARTESIAN_POINT('Ctrl Pts',(46.,47.5,-5.63337527607782E-15));
#14391=CARTESIAN_POINT('Ctrl Pts',(46.,47.2916666666667,12.3256628518316));
#14392=CARTESIAN_POINT('Ctrl Pts',(39.8371685740842,47.0833333333333,23.));
#14393=CARTESIAN_POINT('Ctrl Pts',(33.6743371481684,46.875,33.6743371481683));
#14394=CARTESIAN_POINT('Ctrl Pts',(23.,46.6666666666667,39.8371685740842));
#14395=CARTESIAN_POINT('Ctrl Pts',(12.3256628518317,46.4583333333333,46.));
#14396=CARTESIAN_POINT('Ctrl Pts',(8.45006291411674E-15,46.25,46.));
#14397=CARTESIAN_POINT('Ctrl Pts',(-12.3256628518316,46.0416666666667,46.));
#14398=CARTESIAN_POINT('Ctrl Pts',(-23.,45.8333333333333,39.8371685740842));
#14399=CARTESIAN_POINT('Ctrl Pts',(-33.6743371481683,45.625,33.6743371481684));
#14400=CARTESIAN_POINT('Ctrl Pts',(-39.8371685740842,45.4166666666667,23.));
#14401=CARTESIAN_POINT('Ctrl Pts',(-46.,45.2083333333333,12.3256628518317));
#14402=CARTESIAN_POINT('Ctrl Pts',(-46.,45.,0.));
#14403=CARTESIAN_POINT('Ctrl Pts',(-46.,44.7916666666667,-12.3256628518316));
#14404=CARTESIAN_POINT('Ctrl Pts',(-39.8371685740842,44.5833333333333,-23.));
#14405=CARTESIAN_POINT('Ctrl Pts',(-33.6743371481684,44.375,-33.6743371481684));
#14406=CARTESIAN_POINT('Ctrl Pts',(-23.,44.1666666666667,-39.8371685740842));
#14407=CARTESIAN_POINT('Ctrl Pts',(-12.3256628518317,43.9583333333333,-46.));
#14408=CARTESIAN_POINT('Ctrl Pts',(-2.81668763803891E-15,43.75,-46.));
#14409=CARTESIAN_POINT('Ctrl Pts',(12.3256628518316,43.5416666666667,-46.));
#14410=CARTESIAN_POINT('Ctrl Pts',(23.,43.3333333333333,-39.8371685740842));
#14411=CARTESIAN_POINT('Ctrl Pts',(33.6743371481683,43.125,-33.6743371481684));
#14412=CARTESIAN_POINT('Ctrl Pts',(39.8371685740842,42.9166666666667,-23.));
#14413=CARTESIAN_POINT('Ctrl Pts',(46.,42.7083333333333,-12.3256628518317));
#14414=CARTESIAN_POINT('Ctrl Pts',(46.,42.5,-5.63337527607782E-15));
#14415=CARTESIAN_POINT('Ctrl Pts',(46.,42.2916666666667,12.3256628518316));
#14416=CARTESIAN_POINT('Ctrl Pts',(39.8371685740842,42.0833333333333,23.));
#14417=CARTESIAN_POINT('Ctrl Pts',(33.6743371481684,41.875,33.6743371481683));
#14418=CARTESIAN_POINT('Ctrl Pts',(23.,41.6666666666667,39.8371685740842));
#14419=CARTESIAN_POINT('Ctrl Pts',(12.3256628518317,41.4583333333333,46.));
#14420=CARTESIAN_POINT('Ctrl Pts',(8.45006291411674E-15,41.25,46.));
#14421=CARTESIAN_POINT('Ctrl Pts',(-12.3256628518316,41.0416666666667,46.));
#14422=CARTESIAN_POINT('Ctrl Pts',(-23.,40.8333333333333,39.8371685740842));
#14423=CARTESIAN_POINT('Ctrl Pts',(-33.6743371481683,40.625,33.6743371481684));
#14424=CARTESIAN_POINT('Ctrl Pts',(-39.8371685740842,40.4166666666667,23.));
#14425=CARTESIAN_POINT('Ctrl Pts',(-46.,40.2083333333333,12.3256628518317));
#14426=CARTESIAN_POINT('Ctrl Pts',(-46.,40.,0.));
#14427=CARTESIAN_POINT('Ctrl Pts',(-46.,39.7916666666667,-12.3256628518316));
#14428=CARTESIAN_POINT('Ctrl Pts',(-39.8371685740842,39.5833333333333,-23.));
#14429=CARTESIAN_POINT('Ctrl Pts',(-33.6743371481684,39.375,-33.6743371481684));
#14430=CARTESIAN_POINT('Ctrl Pts',(-23.,39.1666666666667,-39.8371685740842));
#14431=CARTESIAN_POINT('Ctrl Pts',(-12.3256628518317,38.9583333333333,-46.));
#14432=CARTESIAN_POINT('Ctrl Pts',(-2.81668763803891E-15,38.75,-46.));
#14433=CARTESIAN_POINT('Ctrl Pts',(12.3256628518316,38.5416666666667,-46.));
#14434=CARTESIAN_POINT('Ctrl Pts',(23.,38.3333333333333,-39.8371685740842));
#14435=CARTESIAN_POINT('Ctrl Pts',(33.6743371481683,38.125,-33.6743371481684));
#14436=CARTESIAN_POINT('Ctrl Pts',(39.8371685740842,37.9166666666667,-23.));
#14437=CARTESIAN_POINT('Ctrl Pts',(46.,37.7083333333333,-12.3256628518317));
#14438=CARTESIAN_POINT('Ctrl Pts',(46.,37.5,-5.63337527607782E-15));
#14439=CARTESIAN_POINT('Ctrl Pts',(46.,37.2916666666667,12.3256628518316));
#14440=CARTESIAN_POINT('Ctrl Pts',(39.8371685740842,37.0833333333333,23.));
#14441=CARTESIAN_POINT('Ctrl Pts',(33.6743371481684,36.875,33.6743371481683));
#14442=CARTESIAN_POINT('Ctrl Pts',(23.,36.6666666666667,39.8371685740842));
#14443=CARTESIAN_POINT('Ctrl Pts',(12.3256628518317,36.4583333333333,46.));
#14444=CARTESIAN_POINT('Ctrl Pts',(8.45006291411674E-15,36.25,46.));
#14445=CARTESIAN_POINT('Ctrl Pts',(-12.3256628518316,36.0416666666667,46.));
#14446=CARTESIAN_POINT('Ctrl Pts',(-23.,35.8333333333333,39.8371685740842));
#14447=CARTESIAN_POINT('Ctrl Pts',(-33.6743371481683,35.625,33.6743371481684));
#14448=CARTESIAN_POINT('Ctrl Pts',(-39.8371685740842,35.4166666666667,23.));
#14449=CARTESIAN_POINT('Ctrl Pts',(-46.,35.2083333333333,12.3256628518317));
#14450=CARTESIAN_POINT('Ctrl Pts',(-46.,35.,0.));
#14451=CARTESIAN_POINT('Ctrl Pts',(-46.,34.7916666666667,-12.3256628518316));
#14452=CARTESIAN_POINT('Ctrl Pts',(-39.8371685740842,34.5833333333333,-23.));
#14453=CARTESIAN_POINT('Ctrl Pts',(-33.6743371481684,34.375,-33.6743371481684));
#14454=CARTESIAN_POINT('Ctrl Pts',(-23.,34.1666666666667,-39.8371685740842));
#14455=CARTESIAN_POINT('Ctrl Pts',(-12.3256628518317,33.9583333333333,-46.));
#14456=CARTESIAN_POINT('Ctrl Pts',(-2.81668763803891E-15,33.75,-46.));
#14457=CARTESIAN_POINT('Ctrl Pts',(12.3256628518316,33.5416666666667,-46.));
#14458=CARTESIAN_POINT('Ctrl Pts',(23.,33.3333333333333,-39.8371685740842));
#14459=CARTESIAN_POINT('Ctrl Pts',(33.6743371481683,33.125,-33.6743371481684));
#14460=CARTESIAN_POINT('Ctrl Pts',(39.8371685740842,32.9166666666667,-23.));
#14461=CARTESIAN_POINT('Ctrl Pts',(46.,32.7083333333333,-12.3256628518317));
#14462=CARTESIAN_POINT('Ctrl Pts',(46.,32.5,-5.63337527607782E-15));
#14463=CARTESIAN_POINT('Ctrl Pts',(46.,32.2916666666667,12.3256628518316));
#14464=CARTESIAN_POINT('Ctrl Pts',(39.8371685740842,32.0833333333333,23.));
#14465=CARTESIAN_POINT('Ctrl Pts',(33.6743371481684,31.875,33.6743371481683));
#14466=CARTESIAN_POINT('Ctrl Pts',(23.,31.6666666666667,39.8371685740842));
#14467=CARTESIAN_POINT('Ctrl Pts',(12.3256628518317,31.4583333333333,46.));
#14468=CARTESIAN_POINT('Ctrl Pts',(8.45006291411674E-15,31.25,46.));
#14469=CARTESIAN_POINT('Ctrl Pts',(-12.3256628518316,31.0416666666667,46.));
#14470=CARTESIAN_POINT('Ctrl Pts',(-23.,30.8333333333333,39.8371685740842));
#14471=CARTESIAN_POINT('Ctrl Pts',(-33.6743371481683,30.625,33.6743371481684));
#14472=CARTESIAN_POINT('Ctrl Pts',(-39.8371685740842,30.4166666666667,23.));
#14473=CARTESIAN_POINT('Ctrl Pts',(-46.,30.2083333333333,12.3256628518317));
#14474=CARTESIAN_POINT('Ctrl Pts',(-46.,30.,0.));
#14475=CARTESIAN_POINT('Ctrl Pts',(-45.858362923034,55.061608680256,3.60701400320327));
#14476=CARTESIAN_POINT('Ctrl Pts',(-46.089925771934,54.9280150456297,3.60701400320327));
#14477=CARTESIAN_POINT('Ctrl Pts',(-46.5530501979845,54.6608255719956,3.60701400320327));
#14478=CARTESIAN_POINT('Ctrl Pts',(-47.0161721905706,54.3936318804497,3.60701400320325));
#14479=CARTESIAN_POINT('Ctrl Pts',(-47.6893519862319,54.0052434879083,3.60701400320325));
#14480=CARTESIAN_POINT('Ctrl Pts',(-48.1309692507094,53.7504492807381,3.60701400320327));
#14481=CARTESIAN_POINT('Ctrl Pts',(-48.5725845633798,53.4956516907298,3.60701400320327));
#14482=CARTESIAN_POINT('Origin',(-4.32455831995572,-7916.57953929723,-4524.0108731871));
#14483=CARTESIAN_POINT('Ctrl Pts',(-48.706329375,58.437500006828,-1.8898197019151E-14));
#14484=CARTESIAN_POINT('Ctrl Pts',(-48.706329375,58.2291666734946,-13.0508216223155));
#14485=CARTESIAN_POINT('Ctrl Pts',(-42.1809185638422,58.0208333401613,-24.3531646875));
#14486=CARTESIAN_POINT('Ctrl Pts',(-35.6555077526845,57.812500006828,-35.6555077526845));
#14487=CARTESIAN_POINT('Ctrl Pts',(-24.3531646875,57.6041666734946,-42.1809185638422));
#14488=CARTESIAN_POINT('Ctrl Pts',(-13.0508216223155,57.3958333401613,-48.706329375));
#14489=CARTESIAN_POINT('Ctrl Pts',(1.59157945007855E-14,57.187500006828,
-48.706329375));
#14490=CARTESIAN_POINT('Ctrl Pts',(13.0508216223155,56.9791666734946,-48.706329375));
#14491=CARTESIAN_POINT('Ctrl Pts',(24.3531646875,56.7708333401613,-42.1809185638422));
#14492=CARTESIAN_POINT('Ctrl Pts',(35.6555077526845,56.562500006828,-35.6555077526845));
#14493=CARTESIAN_POINT('Ctrl Pts',(42.1809185638422,56.3541666734946,-24.3531646875));
#14494=CARTESIAN_POINT('Ctrl Pts',(48.706329375,56.1458333401613,-13.0508216223155));
#14495=CARTESIAN_POINT('Ctrl Pts',(48.706329375,55.937500006828,1.293339198242E-14));
#14496=CARTESIAN_POINT('Ctrl Pts',(48.706329375,55.7291666734946,13.0508216223155));
#14497=CARTESIAN_POINT('Ctrl Pts',(42.1809185638422,55.5208333401613,24.3531646875));
#14498=CARTESIAN_POINT('Ctrl Pts',(35.6555077526845,55.312500006828,35.6555077526845));
#14499=CARTESIAN_POINT('Ctrl Pts',(24.3531646875,55.1041666734946,42.1809185638422));
#14500=CARTESIAN_POINT('Ctrl Pts',(13.0508216223155,54.8958333401613,48.706329375));
#14501=CARTESIAN_POINT('Ctrl Pts',(-9.95098946405443E-15,54.687500006828,
48.706329375));
#14502=CARTESIAN_POINT('Ctrl Pts',(-13.0508216223155,54.4791666734946,48.706329375));
#14503=CARTESIAN_POINT('Ctrl Pts',(-24.3531646875,54.2708333401613,42.1809185638423));
#14504=CARTESIAN_POINT('Ctrl Pts',(-35.6555077526845,54.062500006828,35.6555077526845));
#14505=CARTESIAN_POINT('Ctrl Pts',(-42.1809185638422,53.8541666734946,24.3531646875));
#14506=CARTESIAN_POINT('Ctrl Pts',(-48.706329375,53.6458333401613,13.0508216223155));
#14507=CARTESIAN_POINT('Ctrl Pts',(-48.706329375,53.437500006828,-1.8898197019151E-14));
#14508=CARTESIAN_POINT('Ctrl Pts',(-48.706329375,53.2291666734946,-13.0508216223155));
#14509=CARTESIAN_POINT('Ctrl Pts',(-42.1809185638422,53.0208333401613,-24.3531646875));
#14510=CARTESIAN_POINT('Ctrl Pts',(-35.6555077526845,52.812500006828,-35.6555077526845));
#14511=CARTESIAN_POINT('Ctrl Pts',(-24.3531646875,52.6041666734946,-42.1809185638422));
#14512=CARTESIAN_POINT('Ctrl Pts',(-13.0508216223155,52.3958333401613,-48.706329375));
#14513=CARTESIAN_POINT('Ctrl Pts',(1.59157945007855E-14,52.187500006828,
-48.706329375));
#14514=CARTESIAN_POINT('Ctrl Pts',(13.0508216223155,51.9791666734946,-48.706329375));
#14515=CARTESIAN_POINT('Ctrl Pts',(24.3531646875,51.7708333401613,-42.1809185638422));
#14516=CARTESIAN_POINT('Ctrl Pts',(35.6555077526845,51.562500006828,-35.6555077526845));
#14517=CARTESIAN_POINT('Ctrl Pts',(42.1809185638422,51.3541666734946,-24.3531646875));
#14518=CARTESIAN_POINT('Ctrl Pts',(48.706329375,51.1458333401613,-13.0508216223155));
#14519=CARTESIAN_POINT('Ctrl Pts',(48.706329375,50.937500006828,1.293339198242E-14));
#14520=CARTESIAN_POINT('Ctrl Pts',(48.706329375,50.7291666734946,13.0508216223155));
#14521=CARTESIAN_POINT('Ctrl Pts',(42.1809185638422,50.5208333401613,24.3531646875));
#14522=CARTESIAN_POINT('Ctrl Pts',(35.6555077526845,50.312500006828,35.6555077526845));
#14523=CARTESIAN_POINT('Ctrl Pts',(24.3531646875,50.1041666734946,42.1809185638422));
#14524=CARTESIAN_POINT('Ctrl Pts',(13.0508216223155,49.8958333401613,48.706329375));
#14525=CARTESIAN_POINT('Ctrl Pts',(-9.95098946405443E-15,49.687500006828,
48.706329375));
#14526=CARTESIAN_POINT('Ctrl Pts',(-13.0508216223155,49.4791666734946,48.706329375));
#14527=CARTESIAN_POINT('Ctrl Pts',(-24.3531646875,49.2708333401613,42.1809185638423));
#14528=CARTESIAN_POINT('Ctrl Pts',(-35.6555077526845,49.062500006828,35.6555077526845));
#14529=CARTESIAN_POINT('Ctrl Pts',(-42.1809185638422,48.8541666734946,24.3531646875));
#14530=CARTESIAN_POINT('Ctrl Pts',(-48.706329375,48.6458333401613,13.0508216223155));
#14531=CARTESIAN_POINT('Ctrl Pts',(-48.706329375,48.437500006828,-1.8898197019151E-14));
#14532=CARTESIAN_POINT('Ctrl Pts',(-48.706329375,48.2291666734946,-13.0508216223155));
#14533=CARTESIAN_POINT('Ctrl Pts',(-42.1809185638422,48.0208333401613,-24.3531646875));
#14534=CARTESIAN_POINT('Ctrl Pts',(-35.6555077526845,47.812500006828,-35.6555077526845));
#14535=CARTESIAN_POINT('Ctrl Pts',(-24.3531646875,47.6041666734946,-42.1809185638422));
#14536=CARTESIAN_POINT('Ctrl Pts',(-13.0508216223155,47.3958333401613,-48.706329375));
#14537=CARTESIAN_POINT('Ctrl Pts',(1.59157945007855E-14,47.187500006828,
-48.706329375));
#14538=CARTESIAN_POINT('Ctrl Pts',(13.0508216223155,46.9791666734946,-48.706329375));
#14539=CARTESIAN_POINT('Ctrl Pts',(24.3531646875,46.7708333401613,-42.1809185638422));
#14540=CARTESIAN_POINT('Ctrl Pts',(35.6555077526845,46.562500006828,-35.6555077526845));
#14541=CARTESIAN_POINT('Ctrl Pts',(42.1809185638422,46.3541666734946,-24.3531646875));
#14542=CARTESIAN_POINT('Ctrl Pts',(48.706329375,46.1458333401613,-13.0508216223155));
#14543=CARTESIAN_POINT('Ctrl Pts',(48.706329375,45.937500006828,1.293339198242E-14));
#14544=CARTESIAN_POINT('Ctrl Pts',(48.706329375,45.7291666734946,13.0508216223155));
#14545=CARTESIAN_POINT('Ctrl Pts',(42.1809185638422,45.5208333401613,24.3531646875));
#14546=CARTESIAN_POINT('Ctrl Pts',(35.6555077526845,45.312500006828,35.6555077526845));
#14547=CARTESIAN_POINT('Ctrl Pts',(24.3531646875,45.1041666734946,42.1809185638422));
#14548=CARTESIAN_POINT('Ctrl Pts',(13.0508216223155,44.8958333401613,48.706329375));
#14549=CARTESIAN_POINT('Ctrl Pts',(-9.95098946405443E-15,44.687500006828,
48.706329375));
#14550=CARTESIAN_POINT('Ctrl Pts',(-13.0508216223155,44.4791666734946,48.706329375));
#14551=CARTESIAN_POINT('Ctrl Pts',(-24.3531646875,44.2708333401613,42.1809185638423));
#14552=CARTESIAN_POINT('Ctrl Pts',(-35.6555077526845,44.062500006828,35.6555077526845));
#14553=CARTESIAN_POINT('Ctrl Pts',(-42.1809185638422,43.8541666734946,24.3531646875));
#14554=CARTESIAN_POINT('Ctrl Pts',(-48.706329375,43.6458333401613,13.0508216223155));
#14555=CARTESIAN_POINT('Ctrl Pts',(-48.706329375,43.437500006828,-1.8898197019151E-14));
#14556=CARTESIAN_POINT('Ctrl Pts',(-48.706329375,43.2291666734946,-13.0508216223155));
#14557=CARTESIAN_POINT('Ctrl Pts',(-42.1809185638422,43.0208333401613,-24.3531646875));
#14558=CARTESIAN_POINT('Ctrl Pts',(-35.6555077526845,42.812500006828,-35.6555077526845));
#14559=CARTESIAN_POINT('Ctrl Pts',(-24.3531646875,42.6041666734946,-42.1809185638422));
#14560=CARTESIAN_POINT('Ctrl Pts',(-13.0508216223155,42.3958333401613,-48.706329375));
#14561=CARTESIAN_POINT('Ctrl Pts',(1.59157945007855E-14,42.187500006828,
-48.706329375));
#14562=CARTESIAN_POINT('Ctrl Pts',(13.0508216223155,41.9791666734946,-48.706329375));
#14563=CARTESIAN_POINT('Ctrl Pts',(24.3531646875,41.7708333401613,-42.1809185638422));
#14564=CARTESIAN_POINT('Ctrl Pts',(35.6555077526845,41.562500006828,-35.6555077526845));
#14565=CARTESIAN_POINT('Ctrl Pts',(42.1809185638422,41.3541666734946,-24.3531646875));
#14566=CARTESIAN_POINT('Ctrl Pts',(48.706329375,41.1458333401613,-13.0508216223155));
#14567=CARTESIAN_POINT('Ctrl Pts',(48.706329375,40.937500006828,1.293339198242E-14));
#14568=CARTESIAN_POINT('Ctrl Pts',(48.706329375,40.7291666734946,13.0508216223155));
#14569=CARTESIAN_POINT('Ctrl Pts',(42.1809185638422,40.5208333401613,24.3531646875));
#14570=CARTESIAN_POINT('Ctrl Pts',(35.6555077526845,40.312500006828,35.6555077526845));
#14571=CARTESIAN_POINT('Ctrl Pts',(24.3531646875,40.1041666734946,42.1809185638422));
#14572=CARTESIAN_POINT('Ctrl Pts',(13.0508216223155,39.8958333401613,48.706329375));
#14573=CARTESIAN_POINT('Ctrl Pts',(-9.95098946405443E-15,39.687500006828,
48.706329375));
#14574=CARTESIAN_POINT('Ctrl Pts',(-13.0508216223155,39.4791666734946,48.706329375));
#14575=CARTESIAN_POINT('Ctrl Pts',(-24.3531646875,39.2708333401613,42.1809185638423));
#14576=CARTESIAN_POINT('Ctrl Pts',(-35.6555077526845,39.062500006828,35.6555077526845));
#14577=CARTESIAN_POINT('Ctrl Pts',(-42.1809185638422,38.8541666734946,24.3531646875));
#14578=CARTESIAN_POINT('Ctrl Pts',(-48.706329375,38.6458333401613,13.0508216223155));
#14579=CARTESIAN_POINT('Ctrl Pts',(-48.706329375,38.437500006828,-1.8898197019151E-14));
#14580=CARTESIAN_POINT('Ctrl Pts',(-48.706329375,38.2291666734946,-13.0508216223155));
#14581=CARTESIAN_POINT('Ctrl Pts',(-42.1809185638422,38.0208333401613,-24.3531646875));
#14582=CARTESIAN_POINT('Ctrl Pts',(-35.6555077526845,37.812500006828,-35.6555077526845));
#14583=CARTESIAN_POINT('Ctrl Pts',(-24.3531646875,37.6041666734946,-42.1809185638422));
#14584=CARTESIAN_POINT('Ctrl Pts',(-13.0508216223155,37.3958333401613,-48.706329375));
#14585=CARTESIAN_POINT('Ctrl Pts',(1.59157945007855E-14,37.187500006828,
-48.706329375));
#14586=CARTESIAN_POINT('Ctrl Pts',(13.0508216223155,36.9791666734946,-48.706329375));
#14587=CARTESIAN_POINT('Ctrl Pts',(24.3531646875,36.7708333401613,-42.1809185638422));
#14588=CARTESIAN_POINT('Ctrl Pts',(35.6555077526845,36.562500006828,-35.6555077526845));
#14589=CARTESIAN_POINT('Ctrl Pts',(42.1809185638422,36.3541666734946,-24.3531646875));
#14590=CARTESIAN_POINT('Ctrl Pts',(48.706329375,36.1458333401613,-13.0508216223155));
#14591=CARTESIAN_POINT('Ctrl Pts',(48.706329375,35.937500006828,1.293339198242E-14));
#14592=CARTESIAN_POINT('Ctrl Pts',(48.706329375,35.7291666734946,13.0508216223155));
#14593=CARTESIAN_POINT('Ctrl Pts',(42.1809185638422,35.5208333401613,24.3531646875));
#14594=CARTESIAN_POINT('Ctrl Pts',(35.6555077526845,35.312500006828,35.6555077526845));
#14595=CARTESIAN_POINT('Ctrl Pts',(24.3531646875,35.1041666734946,42.1809185638422));
#14596=CARTESIAN_POINT('Ctrl Pts',(13.0508216223155,34.8958333401613,48.706329375));
#14597=CARTESIAN_POINT('Ctrl Pts',(-9.95098946405443E-15,34.687500006828,
48.706329375));
#14598=CARTESIAN_POINT('Ctrl Pts',(-13.0508216223155,34.4791666734946,48.706329375));
#14599=CARTESIAN_POINT('Ctrl Pts',(-24.3531646875,34.2708333401613,42.1809185638423));
#14600=CARTESIAN_POINT('Ctrl Pts',(-35.6555077526845,34.062500006828,35.6555077526845));
#14601=CARTESIAN_POINT('Ctrl Pts',(-42.1809185638422,33.8541666734946,24.3531646875));
#14602=CARTESIAN_POINT('Ctrl Pts',(-48.706329375,33.6458333401613,13.0508216223155));
#14603=CARTESIAN_POINT('Ctrl Pts',(-48.706329375,33.437500006828,-1.8898197019151E-14));
#14604=CARTESIAN_POINT('Ctrl Pts',(-48.706329375,33.2291666734946,-13.0508216223155));
#14605=CARTESIAN_POINT('Ctrl Pts',(-42.1809185638422,33.0208333401613,-24.3531646875));
#14606=CARTESIAN_POINT('Ctrl Pts',(-35.6555077526845,32.812500006828,-35.6555077526845));
#14607=CARTESIAN_POINT('Ctrl Pts',(-24.3531646875,32.6041666734946,-42.1809185638422));
#14608=CARTESIAN_POINT('Ctrl Pts',(-13.0508216223155,32.3958333401613,-48.706329375));
#14609=CARTESIAN_POINT('Ctrl Pts',(1.59157945007855E-14,32.187500006828,
-48.706329375));
#14610=CARTESIAN_POINT('Ctrl Pts',(13.0508216223155,31.9791666734946,-48.706329375));
#14611=CARTESIAN_POINT('Ctrl Pts',(24.3531646875,31.7708333401613,-42.1809185638422));
#14612=CARTESIAN_POINT('Ctrl Pts',(35.6555077526845,31.562500006828,-35.6555077526845));
#14613=CARTESIAN_POINT('Ctrl Pts',(42.1809185638422,31.3541666734946,-24.3531646875));
#14614=CARTESIAN_POINT('Ctrl Pts',(48.706329375,31.1458333401613,-13.0508216223155));
#14615=CARTESIAN_POINT('Ctrl Pts',(48.706329375,30.937500006828,1.293339198242E-14));
#14616=CARTESIAN_POINT('Ctrl Pts',(48.706329375,30.7291666734946,13.0508216223155));
#14617=CARTESIAN_POINT('Ctrl Pts',(42.1809185638422,30.5208333401613,24.3531646875));
#14618=CARTESIAN_POINT('Ctrl Pts',(35.6555077526845,30.312500006828,35.6555077526845));
#14619=CARTESIAN_POINT('Ctrl Pts',(24.3531646875,30.1041666734946,42.1809185638422));
#14620=CARTESIAN_POINT('Ctrl Pts',(13.0508216223155,29.8958333401613,48.706329375));
#14621=CARTESIAN_POINT('Ctrl Pts',(-9.95098946405443E-15,29.687500006828,
48.706329375));
#14622=CARTESIAN_POINT('Ctrl Pts',(-13.0508216223155,29.4791666734946,48.706329375));
#14623=CARTESIAN_POINT('Ctrl Pts',(-24.3531646875,29.2708333401613,42.1809185638423));
#14624=CARTESIAN_POINT('Ctrl Pts',(-35.6555077526845,29.062500006828,35.6555077526845));
#14625=CARTESIAN_POINT('Ctrl Pts',(-42.1809185638422,28.8541666734946,24.3531646875));
#14626=CARTESIAN_POINT('Ctrl Pts',(-48.706329375,28.6458333401613,13.0508216223155));
#14627=CARTESIAN_POINT('Ctrl Pts',(-48.706329375,28.437500006828,-1.8898197019151E-14));
#14628=CARTESIAN_POINT('Ctrl Pts',(-46.,60.,0.));
#14629=CARTESIAN_POINT('Ctrl Pts',(-46.,59.7916666666667,-12.3256628518316));
#14630=CARTESIAN_POINT('Ctrl Pts',(-39.8371685740842,59.5833333333333,-23.));
#14631=CARTESIAN_POINT('Ctrl Pts',(-33.6743371481684,59.375,-33.6743371481684));
#14632=CARTESIAN_POINT('Ctrl Pts',(-23.,59.1666666666667,-39.8371685740842));
#14633=CARTESIAN_POINT('Ctrl Pts',(-12.3256628518317,58.9583333333333,-46.));
#14634=CARTESIAN_POINT('Ctrl Pts',(-2.81668763803891E-15,58.75,-46.));
#14635=CARTESIAN_POINT('Ctrl Pts',(12.3256628518316,58.5416666666667,-46.));
#14636=CARTESIAN_POINT('Ctrl Pts',(23.,58.3333333333333,-39.8371685740842));
#14637=CARTESIAN_POINT('Ctrl Pts',(33.6743371481683,58.125,-33.6743371481684));
#14638=CARTESIAN_POINT('Ctrl Pts',(39.8371685740842,57.9166666666667,-23.));
#14639=CARTESIAN_POINT('Ctrl Pts',(46.,57.7083333333333,-12.3256628518317));
#14640=CARTESIAN_POINT('Ctrl Pts',(46.,57.5,-5.63337527607782E-15));
#14641=CARTESIAN_POINT('Ctrl Pts',(46.,57.2916666666667,12.3256628518316));
#14642=CARTESIAN_POINT('Ctrl Pts',(39.8371685740842,57.0833333333333,23.));
#14643=CARTESIAN_POINT('Ctrl Pts',(33.6743371481684,56.875,33.6743371481683));
#14644=CARTESIAN_POINT('Ctrl Pts',(23.,56.6666666666667,39.8371685740842));
#14645=CARTESIAN_POINT('Ctrl Pts',(12.3256628518317,56.4583333333333,46.));
#14646=CARTESIAN_POINT('Ctrl Pts',(8.45006291411674E-15,56.25,46.));
#14647=CARTESIAN_POINT('Ctrl Pts',(-12.3256628518316,56.0416666666667,46.));
#14648=CARTESIAN_POINT('Ctrl Pts',(-23.,55.8333333333333,39.8371685740842));
#14649=CARTESIAN_POINT('Ctrl Pts',(-33.6743371481683,55.625,33.6743371481684));
#14650=CARTESIAN_POINT('Ctrl Pts',(-39.8371685740842,55.4166666666667,23.));
#14651=CARTESIAN_POINT('Ctrl Pts',(-46.,55.2083333333333,12.3256628518317));
#14652=CARTESIAN_POINT('Ctrl Pts',(-46.,55.,0.));
#14653=CARTESIAN_POINT('Ctrl Pts',(-46.,54.7916666666667,-12.3256628518316));
#14654=CARTESIAN_POINT('Ctrl Pts',(-39.8371685740842,54.5833333333333,-23.));
#14655=CARTESIAN_POINT('Ctrl Pts',(-33.6743371481684,54.375,-33.6743371481684));
#14656=CARTESIAN_POINT('Ctrl Pts',(-23.,54.1666666666667,-39.8371685740842));
#14657=CARTESIAN_POINT('Ctrl Pts',(-12.3256628518317,53.9583333333333,-46.));
#14658=CARTESIAN_POINT('Ctrl Pts',(-2.81668763803891E-15,53.75,-46.));
#14659=CARTESIAN_POINT('Ctrl Pts',(12.3256628518316,53.5416666666667,-46.));
#14660=CARTESIAN_POINT('Ctrl Pts',(23.,53.3333333333333,-39.8371685740842));
#14661=CARTESIAN_POINT('Ctrl Pts',(33.6743371481683,53.125,-33.6743371481684));
#14662=CARTESIAN_POINT('Ctrl Pts',(39.8371685740842,52.9166666666667,-23.));
#14663=CARTESIAN_POINT('Ctrl Pts',(46.,52.7083333333333,-12.3256628518317));
#14664=CARTESIAN_POINT('Ctrl Pts',(46.,52.5,-5.63337527607782E-15));
#14665=CARTESIAN_POINT('Ctrl Pts',(46.,52.2916666666667,12.3256628518316));
#14666=CARTESIAN_POINT('Ctrl Pts',(39.8371685740842,52.0833333333333,23.));
#14667=CARTESIAN_POINT('Ctrl Pts',(33.6743371481684,51.875,33.6743371481683));
#14668=CARTESIAN_POINT('Ctrl Pts',(23.,51.6666666666667,39.8371685740842));
#14669=CARTESIAN_POINT('Ctrl Pts',(12.3256628518317,51.4583333333333,46.));
#14670=CARTESIAN_POINT('Ctrl Pts',(8.45006291411674E-15,51.25,46.));
#14671=CARTESIAN_POINT('Ctrl Pts',(-12.3256628518316,51.0416666666667,46.));
#14672=CARTESIAN_POINT('Ctrl Pts',(-23.,50.8333333333333,39.8371685740842));
#14673=CARTESIAN_POINT('Ctrl Pts',(-33.6743371481683,50.625,33.6743371481684));
#14674=CARTESIAN_POINT('Ctrl Pts',(-39.8371685740842,50.4166666666667,23.));
#14675=CARTESIAN_POINT('Ctrl Pts',(-46.,50.2083333333333,12.3256628518317));
#14676=CARTESIAN_POINT('Ctrl Pts',(-46.,50.,0.));
#14677=CARTESIAN_POINT('Ctrl Pts',(-46.,49.7916666666667,-12.3256628518316));
#14678=CARTESIAN_POINT('Ctrl Pts',(-39.8371685740842,49.5833333333333,-23.));
#14679=CARTESIAN_POINT('Ctrl Pts',(-33.6743371481684,49.375,-33.6743371481684));
#14680=CARTESIAN_POINT('Ctrl Pts',(-23.,49.1666666666667,-39.8371685740842));
#14681=CARTESIAN_POINT('Ctrl Pts',(-12.3256628518317,48.9583333333333,-46.));
#14682=CARTESIAN_POINT('Ctrl Pts',(-2.81668763803891E-15,48.75,-46.));
#14683=CARTESIAN_POINT('Ctrl Pts',(12.3256628518316,48.5416666666667,-46.));
#14684=CARTESIAN_POINT('Ctrl Pts',(23.,48.3333333333333,-39.8371685740842));
#14685=CARTESIAN_POINT('Ctrl Pts',(33.6743371481683,48.125,-33.6743371481684));
#14686=CARTESIAN_POINT('Ctrl Pts',(39.8371685740842,47.9166666666667,-23.));
#14687=CARTESIAN_POINT('Ctrl Pts',(46.,47.7083333333333,-12.3256628518317));
#14688=CARTESIAN_POINT('Ctrl Pts',(46.,47.5,-5.63337527607782E-15));
#14689=CARTESIAN_POINT('Ctrl Pts',(46.,47.2916666666667,12.3256628518316));
#14690=CARTESIAN_POINT('Ctrl Pts',(39.8371685740842,47.0833333333333,23.));
#14691=CARTESIAN_POINT('Ctrl Pts',(33.6743371481684,46.875,33.6743371481683));
#14692=CARTESIAN_POINT('Ctrl Pts',(23.,46.6666666666667,39.8371685740842));
#14693=CARTESIAN_POINT('Ctrl Pts',(12.3256628518317,46.4583333333333,46.));
#14694=CARTESIAN_POINT('Ctrl Pts',(8.45006291411674E-15,46.25,46.));
#14695=CARTESIAN_POINT('Ctrl Pts',(-12.3256628518316,46.0416666666667,46.));
#14696=CARTESIAN_POINT('Ctrl Pts',(-23.,45.8333333333333,39.8371685740842));
#14697=CARTESIAN_POINT('Ctrl Pts',(-33.6743371481683,45.625,33.6743371481684));
#14698=CARTESIAN_POINT('Ctrl Pts',(-39.8371685740842,45.4166666666667,23.));
#14699=CARTESIAN_POINT('Ctrl Pts',(-46.,45.2083333333333,12.3256628518317));
#14700=CARTESIAN_POINT('Ctrl Pts',(-46.,45.,0.));
#14701=CARTESIAN_POINT('Ctrl Pts',(-46.,44.7916666666667,-12.3256628518316));
#14702=CARTESIAN_POINT('Ctrl Pts',(-39.8371685740842,44.5833333333333,-23.));
#14703=CARTESIAN_POINT('Ctrl Pts',(-33.6743371481684,44.375,-33.6743371481684));
#14704=CARTESIAN_POINT('Ctrl Pts',(-23.,44.1666666666667,-39.8371685740842));
#14705=CARTESIAN_POINT('Ctrl Pts',(-12.3256628518317,43.9583333333333,-46.));
#14706=CARTESIAN_POINT('Ctrl Pts',(-2.81668763803891E-15,43.75,-46.));
#14707=CARTESIAN_POINT('Ctrl Pts',(12.3256628518316,43.5416666666667,-46.));
#14708=CARTESIAN_POINT('Ctrl Pts',(23.,43.3333333333333,-39.8371685740842));
#14709=CARTESIAN_POINT('Ctrl Pts',(33.6743371481683,43.125,-33.6743371481684));
#14710=CARTESIAN_POINT('Ctrl Pts',(39.8371685740842,42.9166666666667,-23.));
#14711=CARTESIAN_POINT('Ctrl Pts',(46.,42.7083333333333,-12.3256628518317));
#14712=CARTESIAN_POINT('Ctrl Pts',(46.,42.5,-5.63337527607782E-15));
#14713=CARTESIAN_POINT('Ctrl Pts',(46.,42.2916666666667,12.3256628518316));
#14714=CARTESIAN_POINT('Ctrl Pts',(39.8371685740842,42.0833333333333,23.));
#14715=CARTESIAN_POINT('Ctrl Pts',(33.6743371481684,41.875,33.6743371481683));
#14716=CARTESIAN_POINT('Ctrl Pts',(23.,41.6666666666667,39.8371685740842));
#14717=CARTESIAN_POINT('Ctrl Pts',(12.3256628518317,41.4583333333333,46.));
#14718=CARTESIAN_POINT('Ctrl Pts',(8.45006291411674E-15,41.25,46.));
#14719=CARTESIAN_POINT('Ctrl Pts',(-12.3256628518316,41.0416666666667,46.));
#14720=CARTESIAN_POINT('Ctrl Pts',(-23.,40.8333333333333,39.8371685740842));
#14721=CARTESIAN_POINT('Ctrl Pts',(-33.6743371481683,40.625,33.6743371481684));
#14722=CARTESIAN_POINT('Ctrl Pts',(-39.8371685740842,40.4166666666667,23.));
#14723=CARTESIAN_POINT('Ctrl Pts',(-46.,40.2083333333333,12.3256628518317));
#14724=CARTESIAN_POINT('Ctrl Pts',(-46.,40.,0.));
#14725=CARTESIAN_POINT('Ctrl Pts',(-46.,39.7916666666667,-12.3256628518316));
#14726=CARTESIAN_POINT('Ctrl Pts',(-39.8371685740842,39.5833333333333,-23.));
#14727=CARTESIAN_POINT('Ctrl Pts',(-33.6743371481684,39.375,-33.6743371481684));
#14728=CARTESIAN_POINT('Ctrl Pts',(-23.,39.1666666666667,-39.8371685740842));
#14729=CARTESIAN_POINT('Ctrl Pts',(-12.3256628518317,38.9583333333333,-46.));
#14730=CARTESIAN_POINT('Ctrl Pts',(-2.81668763803891E-15,38.75,-46.));
#14731=CARTESIAN_POINT('Ctrl Pts',(12.3256628518316,38.5416666666667,-46.));
#14732=CARTESIAN_POINT('Ctrl Pts',(23.,38.3333333333333,-39.8371685740842));
#14733=CARTESIAN_POINT('Ctrl Pts',(33.6743371481683,38.125,-33.6743371481684));
#14734=CARTESIAN_POINT('Ctrl Pts',(39.8371685740842,37.9166666666667,-23.));
#14735=CARTESIAN_POINT('Ctrl Pts',(46.,37.7083333333333,-12.3256628518317));
#14736=CARTESIAN_POINT('Ctrl Pts',(46.,37.5,-5.63337527607782E-15));
#14737=CARTESIAN_POINT('Ctrl Pts',(46.,37.2916666666667,12.3256628518316));
#14738=CARTESIAN_POINT('Ctrl Pts',(39.8371685740842,37.0833333333333,23.));
#14739=CARTESIAN_POINT('Ctrl Pts',(33.6743371481684,36.875,33.6743371481683));
#14740=CARTESIAN_POINT('Ctrl Pts',(23.,36.6666666666667,39.8371685740842));
#14741=CARTESIAN_POINT('Ctrl Pts',(12.3256628518317,36.4583333333333,46.));
#14742=CARTESIAN_POINT('Ctrl Pts',(8.45006291411674E-15,36.25,46.));
#14743=CARTESIAN_POINT('Ctrl Pts',(-12.3256628518316,36.0416666666667,46.));
#14744=CARTESIAN_POINT('Ctrl Pts',(-23.,35.8333333333333,39.8371685740842));
#14745=CARTESIAN_POINT('Ctrl Pts',(-33.6743371481683,35.625,33.6743371481684));
#14746=CARTESIAN_POINT('Ctrl Pts',(-39.8371685740842,35.4166666666667,23.));
#14747=CARTESIAN_POINT('Ctrl Pts',(-46.,35.2083333333333,12.3256628518317));
#14748=CARTESIAN_POINT('Ctrl Pts',(-46.,35.,0.));
#14749=CARTESIAN_POINT('Ctrl Pts',(-46.,34.7916666666667,-12.3256628518316));
#14750=CARTESIAN_POINT('Ctrl Pts',(-39.8371685740842,34.5833333333333,-23.));
#14751=CARTESIAN_POINT('Ctrl Pts',(-33.6743371481684,34.375,-33.6743371481684));
#14752=CARTESIAN_POINT('Ctrl Pts',(-23.,34.1666666666667,-39.8371685740842));
#14753=CARTESIAN_POINT('Ctrl Pts',(-12.3256628518317,33.9583333333333,-46.));
#14754=CARTESIAN_POINT('Ctrl Pts',(-2.81668763803891E-15,33.75,-46.));
#14755=CARTESIAN_POINT('Ctrl Pts',(12.3256628518316,33.5416666666667,-46.));
#14756=CARTESIAN_POINT('Ctrl Pts',(23.,33.3333333333333,-39.8371685740842));
#14757=CARTESIAN_POINT('Ctrl Pts',(33.6743371481683,33.125,-33.6743371481684));
#14758=CARTESIAN_POINT('Ctrl Pts',(39.8371685740842,32.9166666666667,-23.));
#14759=CARTESIAN_POINT('Ctrl Pts',(46.,32.7083333333333,-12.3256628518317));
#14760=CARTESIAN_POINT('Ctrl Pts',(46.,32.5,-5.63337527607782E-15));
#14761=CARTESIAN_POINT('Ctrl Pts',(46.,32.2916666666667,12.3256628518316));
#14762=CARTESIAN_POINT('Ctrl Pts',(39.8371685740842,32.0833333333333,23.));
#14763=CARTESIAN_POINT('Ctrl Pts',(33.6743371481684,31.875,33.6743371481683));
#14764=CARTESIAN_POINT('Ctrl Pts',(23.,31.6666666666667,39.8371685740842));
#14765=CARTESIAN_POINT('Ctrl Pts',(12.3256628518317,31.4583333333333,46.));
#14766=CARTESIAN_POINT('Ctrl Pts',(8.45006291411674E-15,31.25,46.));
#14767=CARTESIAN_POINT('Ctrl Pts',(-12.3256628518316,31.0416666666667,46.));
#14768=CARTESIAN_POINT('Ctrl Pts',(-23.,30.8333333333333,39.8371685740842));
#14769=CARTESIAN_POINT('Ctrl Pts',(-33.6743371481683,30.625,33.6743371481684));
#14770=CARTESIAN_POINT('Ctrl Pts',(-39.8371685740842,30.4166666666667,23.));
#14771=CARTESIAN_POINT('Ctrl Pts',(-46.,30.2083333333333,12.3256628518317));
#14772=CARTESIAN_POINT('Ctrl Pts',(-46.,30.,0.));
#14773=CARTESIAN_POINT('Origin',(4513.80899862641,-7905.15855185603,-4.33048603483869));
#14774=CARTESIAN_POINT('Ctrl Pts',(-4.32456003949879,48.8240181593938,-45.7962681936506));
#14775=CARTESIAN_POINT('Ctrl Pts',(-4.32456003949874,48.6905125468623,-46.0278818021281));
#14776=CARTESIAN_POINT('Ctrl Pts',(-4.3245600394988,48.4234964717135,-46.4911062234486));
#14777=CARTESIAN_POINT('Ctrl Pts',(-4.32456003949883,48.1564711191154,-46.954325296818));
#14778=CARTESIAN_POINT('Ctrl Pts',(-4.32456003949883,47.7677643029224,-47.6286149142205));
#14779=CARTESIAN_POINT('Ctrl Pts',(-4.32456003949881,47.5125642776457,-48.0712916022845));
#14780=CARTESIAN_POINT('Ctrl Pts',(-4.32456003949881,47.2573567866782,-48.5139639861634));
#14781=CARTESIAN_POINT('Ctrl Pts',(-48.706329375,58.437500006828,-1.8898197019151E-14));
#14782=CARTESIAN_POINT('Ctrl Pts',(-48.706329375,58.2291666734946,-13.0508216223155));
#14783=CARTESIAN_POINT('Ctrl Pts',(-42.1809185638422,58.0208333401613,-24.3531646875));
#14784=CARTESIAN_POINT('Ctrl Pts',(-35.6555077526845,57.812500006828,-35.6555077526845));
#14785=CARTESIAN_POINT('Ctrl Pts',(-24.3531646875,57.6041666734946,-42.1809185638422));
#14786=CARTESIAN_POINT('Ctrl Pts',(-13.0508216223155,57.3958333401613,-48.706329375));
#14787=CARTESIAN_POINT('Ctrl Pts',(1.59157945007855E-14,57.187500006828,
-48.706329375));
#14788=CARTESIAN_POINT('Ctrl Pts',(13.0508216223155,56.9791666734946,-48.706329375));
#14789=CARTESIAN_POINT('Ctrl Pts',(24.3531646875,56.7708333401613,-42.1809185638422));
#14790=CARTESIAN_POINT('Ctrl Pts',(35.6555077526845,56.562500006828,-35.6555077526845));
#14791=CARTESIAN_POINT('Ctrl Pts',(42.1809185638422,56.3541666734946,-24.3531646875));
#14792=CARTESIAN_POINT('Ctrl Pts',(48.706329375,56.1458333401613,-13.0508216223155));
#14793=CARTESIAN_POINT('Ctrl Pts',(48.706329375,55.937500006828,1.293339198242E-14));
#14794=CARTESIAN_POINT('Ctrl Pts',(48.706329375,55.7291666734946,13.0508216223155));
#14795=CARTESIAN_POINT('Ctrl Pts',(42.1809185638422,55.5208333401613,24.3531646875));
#14796=CARTESIAN_POINT('Ctrl Pts',(35.6555077526845,55.312500006828,35.6555077526845));
#14797=CARTESIAN_POINT('Ctrl Pts',(24.3531646875,55.1041666734946,42.1809185638422));
#14798=CARTESIAN_POINT('Ctrl Pts',(13.0508216223155,54.8958333401613,48.706329375));
#14799=CARTESIAN_POINT('Ctrl Pts',(-9.95098946405443E-15,54.687500006828,
48.706329375));
#14800=CARTESIAN_POINT('Ctrl Pts',(-13.0508216223155,54.4791666734946,48.706329375));
#14801=CARTESIAN_POINT('Ctrl Pts',(-24.3531646875,54.2708333401613,42.1809185638423));
#14802=CARTESIAN_POINT('Ctrl Pts',(-35.6555077526845,54.062500006828,35.6555077526845));
#14803=CARTESIAN_POINT('Ctrl Pts',(-42.1809185638422,53.8541666734946,24.3531646875));
#14804=CARTESIAN_POINT('Ctrl Pts',(-48.706329375,53.6458333401613,13.0508216223155));
#14805=CARTESIAN_POINT('Ctrl Pts',(-48.706329375,53.437500006828,-1.8898197019151E-14));
#14806=CARTESIAN_POINT('Ctrl Pts',(-48.706329375,53.2291666734946,-13.0508216223155));
#14807=CARTESIAN_POINT('Ctrl Pts',(-42.1809185638422,53.0208333401613,-24.3531646875));
#14808=CARTESIAN_POINT('Ctrl Pts',(-35.6555077526845,52.812500006828,-35.6555077526845));
#14809=CARTESIAN_POINT('Ctrl Pts',(-24.3531646875,52.6041666734946,-42.1809185638422));
#14810=CARTESIAN_POINT('Ctrl Pts',(-13.0508216223155,52.3958333401613,-48.706329375));
#14811=CARTESIAN_POINT('Ctrl Pts',(1.59157945007855E-14,52.187500006828,
-48.706329375));
#14812=CARTESIAN_POINT('Ctrl Pts',(13.0508216223155,51.9791666734946,-48.706329375));
#14813=CARTESIAN_POINT('Ctrl Pts',(24.3531646875,51.7708333401613,-42.1809185638422));
#14814=CARTESIAN_POINT('Ctrl Pts',(35.6555077526845,51.562500006828,-35.6555077526845));
#14815=CARTESIAN_POINT('Ctrl Pts',(42.1809185638422,51.3541666734946,-24.3531646875));
#14816=CARTESIAN_POINT('Ctrl Pts',(48.706329375,51.1458333401613,-13.0508216223155));
#14817=CARTESIAN_POINT('Ctrl Pts',(48.706329375,50.937500006828,1.293339198242E-14));
#14818=CARTESIAN_POINT('Ctrl Pts',(48.706329375,50.7291666734946,13.0508216223155));
#14819=CARTESIAN_POINT('Ctrl Pts',(42.1809185638422,50.5208333401613,24.3531646875));
#14820=CARTESIAN_POINT('Ctrl Pts',(35.6555077526845,50.312500006828,35.6555077526845));
#14821=CARTESIAN_POINT('Ctrl Pts',(24.3531646875,50.1041666734946,42.1809185638422));
#14822=CARTESIAN_POINT('Ctrl Pts',(13.0508216223155,49.8958333401613,48.706329375));
#14823=CARTESIAN_POINT('Ctrl Pts',(-9.95098946405443E-15,49.687500006828,
48.706329375));
#14824=CARTESIAN_POINT('Ctrl Pts',(-13.0508216223155,49.4791666734946,48.706329375));
#14825=CARTESIAN_POINT('Ctrl Pts',(-24.3531646875,49.2708333401613,42.1809185638423));
#14826=CARTESIAN_POINT('Ctrl Pts',(-35.6555077526845,49.062500006828,35.6555077526845));
#14827=CARTESIAN_POINT('Ctrl Pts',(-42.1809185638422,48.8541666734946,24.3531646875));
#14828=CARTESIAN_POINT('Ctrl Pts',(-48.706329375,48.6458333401613,13.0508216223155));
#14829=CARTESIAN_POINT('Ctrl Pts',(-48.706329375,48.437500006828,-1.8898197019151E-14));
#14830=CARTESIAN_POINT('Ctrl Pts',(-48.706329375,48.2291666734946,-13.0508216223155));
#14831=CARTESIAN_POINT('Ctrl Pts',(-42.1809185638422,48.0208333401613,-24.3531646875));
#14832=CARTESIAN_POINT('Ctrl Pts',(-35.6555077526845,47.812500006828,-35.6555077526845));
#14833=CARTESIAN_POINT('Ctrl Pts',(-24.3531646875,47.6041666734946,-42.1809185638422));
#14834=CARTESIAN_POINT('Ctrl Pts',(-13.0508216223155,47.3958333401613,-48.706329375));
#14835=CARTESIAN_POINT('Ctrl Pts',(1.59157945007855E-14,47.187500006828,
-48.706329375));
#14836=CARTESIAN_POINT('Ctrl Pts',(13.0508216223155,46.9791666734946,-48.706329375));
#14837=CARTESIAN_POINT('Ctrl Pts',(24.3531646875,46.7708333401613,-42.1809185638422));
#14838=CARTESIAN_POINT('Ctrl Pts',(35.6555077526845,46.562500006828,-35.6555077526845));
#14839=CARTESIAN_POINT('Ctrl Pts',(42.1809185638422,46.3541666734946,-24.3531646875));
#14840=CARTESIAN_POINT('Ctrl Pts',(48.706329375,46.1458333401613,-13.0508216223155));
#14841=CARTESIAN_POINT('Ctrl Pts',(48.706329375,45.937500006828,1.293339198242E-14));
#14842=CARTESIAN_POINT('Ctrl Pts',(48.706329375,45.7291666734946,13.0508216223155));
#14843=CARTESIAN_POINT('Ctrl Pts',(42.1809185638422,45.5208333401613,24.3531646875));
#14844=CARTESIAN_POINT('Ctrl Pts',(35.6555077526845,45.312500006828,35.6555077526845));
#14845=CARTESIAN_POINT('Ctrl Pts',(24.3531646875,45.1041666734946,42.1809185638422));
#14846=CARTESIAN_POINT('Ctrl Pts',(13.0508216223155,44.8958333401613,48.706329375));
#14847=CARTESIAN_POINT('Ctrl Pts',(-9.95098946405443E-15,44.687500006828,
48.706329375));
#14848=CARTESIAN_POINT('Ctrl Pts',(-13.0508216223155,44.4791666734946,48.706329375));
#14849=CARTESIAN_POINT('Ctrl Pts',(-24.3531646875,44.2708333401613,42.1809185638423));
#14850=CARTESIAN_POINT('Ctrl Pts',(-35.6555077526845,44.062500006828,35.6555077526845));
#14851=CARTESIAN_POINT('Ctrl Pts',(-42.1809185638422,43.8541666734946,24.3531646875));
#14852=CARTESIAN_POINT('Ctrl Pts',(-48.706329375,43.6458333401613,13.0508216223155));
#14853=CARTESIAN_POINT('Ctrl Pts',(-48.706329375,43.437500006828,-1.8898197019151E-14));
#14854=CARTESIAN_POINT('Ctrl Pts',(-48.706329375,43.2291666734946,-13.0508216223155));
#14855=CARTESIAN_POINT('Ctrl Pts',(-42.1809185638422,43.0208333401613,-24.3531646875));
#14856=CARTESIAN_POINT('Ctrl Pts',(-35.6555077526845,42.812500006828,-35.6555077526845));
#14857=CARTESIAN_POINT('Ctrl Pts',(-24.3531646875,42.6041666734946,-42.1809185638422));
#14858=CARTESIAN_POINT('Ctrl Pts',(-13.0508216223155,42.3958333401613,-48.706329375));
#14859=CARTESIAN_POINT('Ctrl Pts',(1.59157945007855E-14,42.187500006828,
-48.706329375));
#14860=CARTESIAN_POINT('Ctrl Pts',(13.0508216223155,41.9791666734946,-48.706329375));
#14861=CARTESIAN_POINT('Ctrl Pts',(24.3531646875,41.7708333401613,-42.1809185638422));
#14862=CARTESIAN_POINT('Ctrl Pts',(35.6555077526845,41.562500006828,-35.6555077526845));
#14863=CARTESIAN_POINT('Ctrl Pts',(42.1809185638422,41.3541666734946,-24.3531646875));
#14864=CARTESIAN_POINT('Ctrl Pts',(48.706329375,41.1458333401613,-13.0508216223155));
#14865=CARTESIAN_POINT('Ctrl Pts',(48.706329375,40.937500006828,1.293339198242E-14));
#14866=CARTESIAN_POINT('Ctrl Pts',(48.706329375,40.7291666734946,13.0508216223155));
#14867=CARTESIAN_POINT('Ctrl Pts',(42.1809185638422,40.5208333401613,24.3531646875));
#14868=CARTESIAN_POINT('Ctrl Pts',(35.6555077526845,40.312500006828,35.6555077526845));
#14869=CARTESIAN_POINT('Ctrl Pts',(24.3531646875,40.1041666734946,42.1809185638422));
#14870=CARTESIAN_POINT('Ctrl Pts',(13.0508216223155,39.8958333401613,48.706329375));
#14871=CARTESIAN_POINT('Ctrl Pts',(-9.95098946405443E-15,39.687500006828,
48.706329375));
#14872=CARTESIAN_POINT('Ctrl Pts',(-13.0508216223155,39.4791666734946,48.706329375));
#14873=CARTESIAN_POINT('Ctrl Pts',(-24.3531646875,39.2708333401613,42.1809185638423));
#14874=CARTESIAN_POINT('Ctrl Pts',(-35.6555077526845,39.062500006828,35.6555077526845));
#14875=CARTESIAN_POINT('Ctrl Pts',(-42.1809185638422,38.8541666734946,24.3531646875));
#14876=CARTESIAN_POINT('Ctrl Pts',(-48.706329375,38.6458333401613,13.0508216223155));
#14877=CARTESIAN_POINT('Ctrl Pts',(-48.706329375,38.437500006828,-1.8898197019151E-14));
#14878=CARTESIAN_POINT('Ctrl Pts',(-48.706329375,38.2291666734946,-13.0508216223155));
#14879=CARTESIAN_POINT('Ctrl Pts',(-42.1809185638422,38.0208333401613,-24.3531646875));
#14880=CARTESIAN_POINT('Ctrl Pts',(-35.6555077526845,37.812500006828,-35.6555077526845));
#14881=CARTESIAN_POINT('Ctrl Pts',(-24.3531646875,37.6041666734946,-42.1809185638422));
#14882=CARTESIAN_POINT('Ctrl Pts',(-13.0508216223155,37.3958333401613,-48.706329375));
#14883=CARTESIAN_POINT('Ctrl Pts',(1.59157945007855E-14,37.187500006828,
-48.706329375));
#14884=CARTESIAN_POINT('Ctrl Pts',(13.0508216223155,36.9791666734946,-48.706329375));
#14885=CARTESIAN_POINT('Ctrl Pts',(24.3531646875,36.7708333401613,-42.1809185638422));
#14886=CARTESIAN_POINT('Ctrl Pts',(35.6555077526845,36.562500006828,-35.6555077526845));
#14887=CARTESIAN_POINT('Ctrl Pts',(42.1809185638422,36.3541666734946,-24.3531646875));
#14888=CARTESIAN_POINT('Ctrl Pts',(48.706329375,36.1458333401613,-13.0508216223155));
#14889=CARTESIAN_POINT('Ctrl Pts',(48.706329375,35.937500006828,1.293339198242E-14));
#14890=CARTESIAN_POINT('Ctrl Pts',(48.706329375,35.7291666734946,13.0508216223155));
#14891=CARTESIAN_POINT('Ctrl Pts',(42.1809185638422,35.5208333401613,24.3531646875));
#14892=CARTESIAN_POINT('Ctrl Pts',(35.6555077526845,35.312500006828,35.6555077526845));
#14893=CARTESIAN_POINT('Ctrl Pts',(24.3531646875,35.1041666734946,42.1809185638422));
#14894=CARTESIAN_POINT('Ctrl Pts',(13.0508216223155,34.8958333401613,48.706329375));
#14895=CARTESIAN_POINT('Ctrl Pts',(-9.95098946405443E-15,34.687500006828,
48.706329375));
#14896=CARTESIAN_POINT('Ctrl Pts',(-13.0508216223155,34.4791666734946,48.706329375));
#14897=CARTESIAN_POINT('Ctrl Pts',(-24.3531646875,34.2708333401613,42.1809185638423));
#14898=CARTESIAN_POINT('Ctrl Pts',(-35.6555077526845,34.062500006828,35.6555077526845));
#14899=CARTESIAN_POINT('Ctrl Pts',(-42.1809185638422,33.8541666734946,24.3531646875));
#14900=CARTESIAN_POINT('Ctrl Pts',(-48.706329375,33.6458333401613,13.0508216223155));
#14901=CARTESIAN_POINT('Ctrl Pts',(-48.706329375,33.437500006828,-1.8898197019151E-14));
#14902=CARTESIAN_POINT('Ctrl Pts',(-48.706329375,33.2291666734946,-13.0508216223155));
#14903=CARTESIAN_POINT('Ctrl Pts',(-42.1809185638422,33.0208333401613,-24.3531646875));
#14904=CARTESIAN_POINT('Ctrl Pts',(-35.6555077526845,32.812500006828,-35.6555077526845));
#14905=CARTESIAN_POINT('Ctrl Pts',(-24.3531646875,32.6041666734946,-42.1809185638422));
#14906=CARTESIAN_POINT('Ctrl Pts',(-13.0508216223155,32.3958333401613,-48.706329375));
#14907=CARTESIAN_POINT('Ctrl Pts',(1.59157945007855E-14,32.187500006828,
-48.706329375));
#14908=CARTESIAN_POINT('Ctrl Pts',(13.0508216223155,31.9791666734946,-48.706329375));
#14909=CARTESIAN_POINT('Ctrl Pts',(24.3531646875,31.7708333401613,-42.1809185638422));
#14910=CARTESIAN_POINT('Ctrl Pts',(35.6555077526845,31.562500006828,-35.6555077526845));
#14911=CARTESIAN_POINT('Ctrl Pts',(42.1809185638422,31.3541666734946,-24.3531646875));
#14912=CARTESIAN_POINT('Ctrl Pts',(48.706329375,31.1458333401613,-13.0508216223155));
#14913=CARTESIAN_POINT('Ctrl Pts',(48.706329375,30.937500006828,1.293339198242E-14));
#14914=CARTESIAN_POINT('Ctrl Pts',(48.706329375,30.7291666734946,13.0508216223155));
#14915=CARTESIAN_POINT('Ctrl Pts',(42.1809185638422,30.5208333401613,24.3531646875));
#14916=CARTESIAN_POINT('Ctrl Pts',(35.6555077526845,30.312500006828,35.6555077526845));
#14917=CARTESIAN_POINT('Ctrl Pts',(24.3531646875,30.1041666734946,42.1809185638422));
#14918=CARTESIAN_POINT('Ctrl Pts',(13.0508216223155,29.8958333401613,48.706329375));
#14919=CARTESIAN_POINT('Ctrl Pts',(-9.95098946405443E-15,29.687500006828,
48.706329375));
#14920=CARTESIAN_POINT('Ctrl Pts',(-13.0508216223155,29.4791666734946,48.706329375));
#14921=CARTESIAN_POINT('Ctrl Pts',(-24.3531646875,29.2708333401613,42.1809185638423));
#14922=CARTESIAN_POINT('Ctrl Pts',(-35.6555077526845,29.062500006828,35.6555077526845));
#14923=CARTESIAN_POINT('Ctrl Pts',(-42.1809185638422,28.8541666734946,24.3531646875));
#14924=CARTESIAN_POINT('Ctrl Pts',(-48.706329375,28.6458333401613,13.0508216223155));
#14925=CARTESIAN_POINT('Ctrl Pts',(-48.706329375,28.437500006828,-1.8898197019151E-14));
#14926=CARTESIAN_POINT('Ctrl Pts',(-46.,60.,0.));
#14927=CARTESIAN_POINT('Ctrl Pts',(-46.,59.7916666666667,-12.3256628518316));
#14928=CARTESIAN_POINT('Ctrl Pts',(-39.8371685740842,59.5833333333333,-23.));
#14929=CARTESIAN_POINT('Ctrl Pts',(-33.6743371481684,59.375,-33.6743371481684));
#14930=CARTESIAN_POINT('Ctrl Pts',(-23.,59.1666666666667,-39.8371685740842));
#14931=CARTESIAN_POINT('Ctrl Pts',(-12.3256628518317,58.9583333333333,-46.));
#14932=CARTESIAN_POINT('Ctrl Pts',(-2.81668763803891E-15,58.75,-46.));
#14933=CARTESIAN_POINT('Ctrl Pts',(12.3256628518316,58.5416666666667,-46.));
#14934=CARTESIAN_POINT('Ctrl Pts',(23.,58.3333333333333,-39.8371685740842));
#14935=CARTESIAN_POINT('Ctrl Pts',(33.6743371481683,58.125,-33.6743371481684));
#14936=CARTESIAN_POINT('Ctrl Pts',(39.8371685740842,57.9166666666667,-23.));
#14937=CARTESIAN_POINT('Ctrl Pts',(46.,57.7083333333333,-12.3256628518317));
#14938=CARTESIAN_POINT('Ctrl Pts',(46.,57.5,-5.63337527607782E-15));
#14939=CARTESIAN_POINT('Ctrl Pts',(46.,57.2916666666667,12.3256628518316));
#14940=CARTESIAN_POINT('Ctrl Pts',(39.8371685740842,57.0833333333333,23.));
#14941=CARTESIAN_POINT('Ctrl Pts',(33.6743371481684,56.875,33.6743371481683));
#14942=CARTESIAN_POINT('Ctrl Pts',(23.,56.6666666666667,39.8371685740842));
#14943=CARTESIAN_POINT('Ctrl Pts',(12.3256628518317,56.4583333333333,46.));
#14944=CARTESIAN_POINT('Ctrl Pts',(8.45006291411674E-15,56.25,46.));
#14945=CARTESIAN_POINT('Ctrl Pts',(-12.3256628518316,56.0416666666667,46.));
#14946=CARTESIAN_POINT('Ctrl Pts',(-23.,55.8333333333333,39.8371685740842));
#14947=CARTESIAN_POINT('Ctrl Pts',(-33.6743371481683,55.625,33.6743371481684));
#14948=CARTESIAN_POINT('Ctrl Pts',(-39.8371685740842,55.4166666666667,23.));
#14949=CARTESIAN_POINT('Ctrl Pts',(-46.,55.2083333333333,12.3256628518317));
#14950=CARTESIAN_POINT('Ctrl Pts',(-46.,55.,0.));
#14951=CARTESIAN_POINT('Ctrl Pts',(-46.,54.7916666666667,-12.3256628518316));
#14952=CARTESIAN_POINT('Ctrl Pts',(-39.8371685740842,54.5833333333333,-23.));
#14953=CARTESIAN_POINT('Ctrl Pts',(-33.6743371481684,54.375,-33.6743371481684));
#14954=CARTESIAN_POINT('Ctrl Pts',(-23.,54.1666666666667,-39.8371685740842));
#14955=CARTESIAN_POINT('Ctrl Pts',(-12.3256628518317,53.9583333333333,-46.));
#14956=CARTESIAN_POINT('Ctrl Pts',(-2.81668763803891E-15,53.75,-46.));
#14957=CARTESIAN_POINT('Ctrl Pts',(12.3256628518316,53.5416666666667,-46.));
#14958=CARTESIAN_POINT('Ctrl Pts',(23.,53.3333333333333,-39.8371685740842));
#14959=CARTESIAN_POINT('Ctrl Pts',(33.6743371481683,53.125,-33.6743371481684));
#14960=CARTESIAN_POINT('Ctrl Pts',(39.8371685740842,52.9166666666667,-23.));
#14961=CARTESIAN_POINT('Ctrl Pts',(46.,52.7083333333333,-12.3256628518317));
#14962=CARTESIAN_POINT('Ctrl Pts',(46.,52.5,-5.63337527607782E-15));
#14963=CARTESIAN_POINT('Ctrl Pts',(46.,52.2916666666667,12.3256628518316));
#14964=CARTESIAN_POINT('Ctrl Pts',(39.8371685740842,52.0833333333333,23.));
#14965=CARTESIAN_POINT('Ctrl Pts',(33.6743371481684,51.875,33.6743371481683));
#14966=CARTESIAN_POINT('Ctrl Pts',(23.,51.6666666666667,39.8371685740842));
#14967=CARTESIAN_POINT('Ctrl Pts',(12.3256628518317,51.4583333333333,46.));
#14968=CARTESIAN_POINT('Ctrl Pts',(8.45006291411674E-15,51.25,46.));
#14969=CARTESIAN_POINT('Ctrl Pts',(-12.3256628518316,51.0416666666667,46.));
#14970=CARTESIAN_POINT('Ctrl Pts',(-23.,50.8333333333333,39.8371685740842));
#14971=CARTESIAN_POINT('Ctrl Pts',(-33.6743371481683,50.625,33.6743371481684));
#14972=CARTESIAN_POINT('Ctrl Pts',(-39.8371685740842,50.4166666666667,23.));
#14973=CARTESIAN_POINT('Ctrl Pts',(-46.,50.2083333333333,12.3256628518317));
#14974=CARTESIAN_POINT('Ctrl Pts',(-46.,50.,0.));
#14975=CARTESIAN_POINT('Ctrl Pts',(-46.,49.7916666666667,-12.3256628518316));
#14976=CARTESIAN_POINT('Ctrl Pts',(-39.8371685740842,49.5833333333333,-23.));
#14977=CARTESIAN_POINT('Ctrl Pts',(-33.6743371481684,49.375,-33.6743371481684));
#14978=CARTESIAN_POINT('Ctrl Pts',(-23.,49.1666666666667,-39.8371685740842));
#14979=CARTESIAN_POINT('Ctrl Pts',(-12.3256628518317,48.9583333333333,-46.));
#14980=CARTESIAN_POINT('Ctrl Pts',(-2.81668763803891E-15,48.75,-46.));
#14981=CARTESIAN_POINT('Ctrl Pts',(12.3256628518316,48.5416666666667,-46.));
#14982=CARTESIAN_POINT('Ctrl Pts',(23.,48.3333333333333,-39.8371685740842));
#14983=CARTESIAN_POINT('Ctrl Pts',(33.6743371481683,48.125,-33.6743371481684));
#14984=CARTESIAN_POINT('Ctrl Pts',(39.8371685740842,47.9166666666667,-23.));
#14985=CARTESIAN_POINT('Ctrl Pts',(46.,47.7083333333333,-12.3256628518317));
#14986=CARTESIAN_POINT('Ctrl Pts',(46.,47.5,-5.63337527607782E-15));
#14987=CARTESIAN_POINT('Ctrl Pts',(46.,47.2916666666667,12.3256628518316));
#14988=CARTESIAN_POINT('Ctrl Pts',(39.8371685740842,47.0833333333333,23.));
#14989=CARTESIAN_POINT('Ctrl Pts',(33.6743371481684,46.875,33.6743371481683));
#14990=CARTESIAN_POINT('Ctrl Pts',(23.,46.6666666666667,39.8371685740842));
#14991=CARTESIAN_POINT('Ctrl Pts',(12.3256628518317,46.4583333333333,46.));
#14992=CARTESIAN_POINT('Ctrl Pts',(8.45006291411674E-15,46.25,46.));
#14993=CARTESIAN_POINT('Ctrl Pts',(-12.3256628518316,46.0416666666667,46.));
#14994=CARTESIAN_POINT('Ctrl Pts',(-23.,45.8333333333333,39.8371685740842));
#14995=CARTESIAN_POINT('Ctrl Pts',(-33.6743371481683,45.625,33.6743371481684));
#14996=CARTESIAN_POINT('Ctrl Pts',(-39.8371685740842,45.4166666666667,23.));
#14997=CARTESIAN_POINT('Ctrl Pts',(-46.,45.2083333333333,12.3256628518317));
#14998=CARTESIAN_POINT('Ctrl Pts',(-46.,45.,0.));
#14999=CARTESIAN_POINT('Ctrl Pts',(-46.,44.7916666666667,-12.3256628518316));
#15000=CARTESIAN_POINT('Ctrl Pts',(-39.8371685740842,44.5833333333333,-23.));
#15001=CARTESIAN_POINT('Ctrl Pts',(-33.6743371481684,44.375,-33.6743371481684));
#15002=CARTESIAN_POINT('Ctrl Pts',(-23.,44.1666666666667,-39.8371685740842));
#15003=CARTESIAN_POINT('Ctrl Pts',(-12.3256628518317,43.9583333333333,-46.));
#15004=CARTESIAN_POINT('Ctrl Pts',(-2.81668763803891E-15,43.75,-46.));
#15005=CARTESIAN_POINT('Ctrl Pts',(12.3256628518316,43.5416666666667,-46.));
#15006=CARTESIAN_POINT('Ctrl Pts',(23.,43.3333333333333,-39.8371685740842));
#15007=CARTESIAN_POINT('Ctrl Pts',(33.6743371481683,43.125,-33.6743371481684));
#15008=CARTESIAN_POINT('Ctrl Pts',(39.8371685740842,42.9166666666667,-23.));
#15009=CARTESIAN_POINT('Ctrl Pts',(46.,42.7083333333333,-12.3256628518317));
#15010=CARTESIAN_POINT('Ctrl Pts',(46.,42.5,-5.63337527607782E-15));
#15011=CARTESIAN_POINT('Ctrl Pts',(46.,42.2916666666667,12.3256628518316));
#15012=CARTESIAN_POINT('Ctrl Pts',(39.8371685740842,42.0833333333333,23.));
#15013=CARTESIAN_POINT('Ctrl Pts',(33.6743371481684,41.875,33.6743371481683));
#15014=CARTESIAN_POINT('Ctrl Pts',(23.,41.6666666666667,39.8371685740842));
#15015=CARTESIAN_POINT('Ctrl Pts',(12.3256628518317,41.4583333333333,46.));
#15016=CARTESIAN_POINT('Ctrl Pts',(8.45006291411674E-15,41.25,46.));
#15017=CARTESIAN_POINT('Ctrl Pts',(-12.3256628518316,41.0416666666667,46.));
#15018=CARTESIAN_POINT('Ctrl Pts',(-23.,40.8333333333333,39.8371685740842));
#15019=CARTESIAN_POINT('Ctrl Pts',(-33.6743371481683,40.625,33.6743371481684));
#15020=CARTESIAN_POINT('Ctrl Pts',(-39.8371685740842,40.4166666666667,23.));
#15021=CARTESIAN_POINT('Ctrl Pts',(-46.,40.2083333333333,12.3256628518317));
#15022=CARTESIAN_POINT('Ctrl Pts',(-46.,40.,0.));
#15023=CARTESIAN_POINT('Ctrl Pts',(-46.,39.7916666666667,-12.3256628518316));
#15024=CARTESIAN_POINT('Ctrl Pts',(-39.8371685740842,39.5833333333333,-23.));
#15025=CARTESIAN_POINT('Ctrl Pts',(-33.6743371481684,39.375,-33.6743371481684));
#15026=CARTESIAN_POINT('Ctrl Pts',(-23.,39.1666666666667,-39.8371685740842));
#15027=CARTESIAN_POINT('Ctrl Pts',(-12.3256628518317,38.9583333333333,-46.));
#15028=CARTESIAN_POINT('Ctrl Pts',(-2.81668763803891E-15,38.75,-46.));
#15029=CARTESIAN_POINT('Ctrl Pts',(12.3256628518316,38.5416666666667,-46.));
#15030=CARTESIAN_POINT('Ctrl Pts',(23.,38.3333333333333,-39.8371685740842));
#15031=CARTESIAN_POINT('Ctrl Pts',(33.6743371481683,38.125,-33.6743371481684));
#15032=CARTESIAN_POINT('Ctrl Pts',(39.8371685740842,37.9166666666667,-23.));
#15033=CARTESIAN_POINT('Ctrl Pts',(46.,37.7083333333333,-12.3256628518317));
#15034=CARTESIAN_POINT('Ctrl Pts',(46.,37.5,-5.63337527607782E-15));
#15035=CARTESIAN_POINT('Ctrl Pts',(46.,37.2916666666667,12.3256628518316));
#15036=CARTESIAN_POINT('Ctrl Pts',(39.8371685740842,37.0833333333333,23.));
#15037=CARTESIAN_POINT('Ctrl Pts',(33.6743371481684,36.875,33.6743371481683));
#15038=CARTESIAN_POINT('Ctrl Pts',(23.,36.6666666666667,39.8371685740842));
#15039=CARTESIAN_POINT('Ctrl Pts',(12.3256628518317,36.4583333333333,46.));
#15040=CARTESIAN_POINT('Ctrl Pts',(8.45006291411674E-15,36.25,46.));
#15041=CARTESIAN_POINT('Ctrl Pts',(-12.3256628518316,36.0416666666667,46.));
#15042=CARTESIAN_POINT('Ctrl Pts',(-23.,35.8333333333333,39.8371685740842));
#15043=CARTESIAN_POINT('Ctrl Pts',(-33.6743371481683,35.625,33.6743371481684));
#15044=CARTESIAN_POINT('Ctrl Pts',(-39.8371685740842,35.4166666666667,23.));
#15045=CARTESIAN_POINT('Ctrl Pts',(-46.,35.2083333333333,12.3256628518317));
#15046=CARTESIAN_POINT('Ctrl Pts',(-46.,35.,0.));
#15047=CARTESIAN_POINT('Ctrl Pts',(-46.,34.7916666666667,-12.3256628518316));
#15048=CARTESIAN_POINT('Ctrl Pts',(-39.8371685740842,34.5833333333333,-23.));
#15049=CARTESIAN_POINT('Ctrl Pts',(-33.6743371481684,34.375,-33.6743371481684));
#15050=CARTESIAN_POINT('Ctrl Pts',(-23.,34.1666666666667,-39.8371685740842));
#15051=CARTESIAN_POINT('Ctrl Pts',(-12.3256628518317,33.9583333333333,-46.));
#15052=CARTESIAN_POINT('Ctrl Pts',(-2.81668763803891E-15,33.75,-46.));
#15053=CARTESIAN_POINT('Ctrl Pts',(12.3256628518316,33.5416666666667,-46.));
#15054=CARTESIAN_POINT('Ctrl Pts',(23.,33.3333333333333,-39.8371685740842));
#15055=CARTESIAN_POINT('Ctrl Pts',(33.6743371481683,33.125,-33.6743371481684));
#15056=CARTESIAN_POINT('Ctrl Pts',(39.8371685740842,32.9166666666667,-23.));
#15057=CARTESIAN_POINT('Ctrl Pts',(46.,32.7083333333333,-12.3256628518317));
#15058=CARTESIAN_POINT('Ctrl Pts',(46.,32.5,-5.63337527607782E-15));
#15059=CARTESIAN_POINT('Ctrl Pts',(46.,32.2916666666667,12.3256628518316));
#15060=CARTESIAN_POINT('Ctrl Pts',(39.8371685740842,32.0833333333333,23.));
#15061=CARTESIAN_POINT('Ctrl Pts',(33.6743371481684,31.875,33.6743371481683));
#15062=CARTESIAN_POINT('Ctrl Pts',(23.,31.6666666666667,39.8371685740842));
#15063=CARTESIAN_POINT('Ctrl Pts',(12.3256628518317,31.4583333333333,46.));
#15064=CARTESIAN_POINT('Ctrl Pts',(8.45006291411674E-15,31.25,46.));
#15065=CARTESIAN_POINT('Ctrl Pts',(-12.3256628518316,31.0416666666667,46.));
#15066=CARTESIAN_POINT('Ctrl Pts',(-23.,30.8333333333333,39.8371685740842));
#15067=CARTESIAN_POINT('Ctrl Pts',(-33.6743371481683,30.625,33.6743371481684));
#15068=CARTESIAN_POINT('Ctrl Pts',(-39.8371685740842,30.4166666666667,23.));
#15069=CARTESIAN_POINT('Ctrl Pts',(-46.,30.2083333333333,12.3256628518317));
#15070=CARTESIAN_POINT('Ctrl Pts',(-46.,30.,0.));
#15071=CARTESIAN_POINT('Ctrl Pts',(-45.858362923034,50.061608680256,3.60701400320326));
#15072=CARTESIAN_POINT('Ctrl Pts',(-46.089925771934,49.9280150456296,3.60701400320326));
#15073=CARTESIAN_POINT('Ctrl Pts',(-46.5530501979845,49.6608255719955,3.60701400320326));
#15074=CARTESIAN_POINT('Ctrl Pts',(-47.0161721905706,49.3936318804496,3.60701400320324));
#15075=CARTESIAN_POINT('Ctrl Pts',(-47.6893519862319,49.0052434879083,3.60701400320324));
#15076=CARTESIAN_POINT('Ctrl Pts',(-48.1309692507095,48.7504492807381,3.60701400320326));
#15077=CARTESIAN_POINT('Ctrl Pts',(-48.5725845633798,48.4956516907297,3.60701400320326));
#15078=CARTESIAN_POINT('Origin',(-4.32456000128674,-7921.57954027603,-4524.01087374411));
#15079=CARTESIAN_POINT('Ctrl Pts',(-48.706329375,58.437500006828,-1.8898197019151E-14));
#15080=CARTESIAN_POINT('Ctrl Pts',(-48.706329375,58.2291666734946,-13.0508216223155));
#15081=CARTESIAN_POINT('Ctrl Pts',(-42.1809185638422,58.0208333401613,-24.3531646875));
#15082=CARTESIAN_POINT('Ctrl Pts',(-35.6555077526845,57.812500006828,-35.6555077526845));
#15083=CARTESIAN_POINT('Ctrl Pts',(-24.3531646875,57.6041666734946,-42.1809185638422));
#15084=CARTESIAN_POINT('Ctrl Pts',(-13.0508216223155,57.3958333401613,-48.706329375));
#15085=CARTESIAN_POINT('Ctrl Pts',(1.59157945007855E-14,57.187500006828,
-48.706329375));
#15086=CARTESIAN_POINT('Ctrl Pts',(13.0508216223155,56.9791666734946,-48.706329375));
#15087=CARTESIAN_POINT('Ctrl Pts',(24.3531646875,56.7708333401613,-42.1809185638422));
#15088=CARTESIAN_POINT('Ctrl Pts',(35.6555077526845,56.562500006828,-35.6555077526845));
#15089=CARTESIAN_POINT('Ctrl Pts',(42.1809185638422,56.3541666734946,-24.3531646875));
#15090=CARTESIAN_POINT('Ctrl Pts',(48.706329375,56.1458333401613,-13.0508216223155));
#15091=CARTESIAN_POINT('Ctrl Pts',(48.706329375,55.937500006828,1.293339198242E-14));
#15092=CARTESIAN_POINT('Ctrl Pts',(48.706329375,55.7291666734946,13.0508216223155));
#15093=CARTESIAN_POINT('Ctrl Pts',(42.1809185638422,55.5208333401613,24.3531646875));
#15094=CARTESIAN_POINT('Ctrl Pts',(35.6555077526845,55.312500006828,35.6555077526845));
#15095=CARTESIAN_POINT('Ctrl Pts',(24.3531646875,55.1041666734946,42.1809185638422));
#15096=CARTESIAN_POINT('Ctrl Pts',(13.0508216223155,54.8958333401613,48.706329375));
#15097=CARTESIAN_POINT('Ctrl Pts',(-9.95098946405443E-15,54.687500006828,
48.706329375));
#15098=CARTESIAN_POINT('Ctrl Pts',(-13.0508216223155,54.4791666734946,48.706329375));
#15099=CARTESIAN_POINT('Ctrl Pts',(-24.3531646875,54.2708333401613,42.1809185638423));
#15100=CARTESIAN_POINT('Ctrl Pts',(-35.6555077526845,54.062500006828,35.6555077526845));
#15101=CARTESIAN_POINT('Ctrl Pts',(-42.1809185638422,53.8541666734946,24.3531646875));
#15102=CARTESIAN_POINT('Ctrl Pts',(-48.706329375,53.6458333401613,13.0508216223155));
#15103=CARTESIAN_POINT('Ctrl Pts',(-48.706329375,53.437500006828,-1.8898197019151E-14));
#15104=CARTESIAN_POINT('Ctrl Pts',(-48.706329375,53.2291666734946,-13.0508216223155));
#15105=CARTESIAN_POINT('Ctrl Pts',(-42.1809185638422,53.0208333401613,-24.3531646875));
#15106=CARTESIAN_POINT('Ctrl Pts',(-35.6555077526845,52.812500006828,-35.6555077526845));
#15107=CARTESIAN_POINT('Ctrl Pts',(-24.3531646875,52.6041666734946,-42.1809185638422));
#15108=CARTESIAN_POINT('Ctrl Pts',(-13.0508216223155,52.3958333401613,-48.706329375));
#15109=CARTESIAN_POINT('Ctrl Pts',(1.59157945007855E-14,52.187500006828,
-48.706329375));
#15110=CARTESIAN_POINT('Ctrl Pts',(13.0508216223155,51.9791666734946,-48.706329375));
#15111=CARTESIAN_POINT('Ctrl Pts',(24.3531646875,51.7708333401613,-42.1809185638422));
#15112=CARTESIAN_POINT('Ctrl Pts',(35.6555077526845,51.562500006828,-35.6555077526845));
#15113=CARTESIAN_POINT('Ctrl Pts',(42.1809185638422,51.3541666734946,-24.3531646875));
#15114=CARTESIAN_POINT('Ctrl Pts',(48.706329375,51.1458333401613,-13.0508216223155));
#15115=CARTESIAN_POINT('Ctrl Pts',(48.706329375,50.937500006828,1.293339198242E-14));
#15116=CARTESIAN_POINT('Ctrl Pts',(48.706329375,50.7291666734946,13.0508216223155));
#15117=CARTESIAN_POINT('Ctrl Pts',(42.1809185638422,50.5208333401613,24.3531646875));
#15118=CARTESIAN_POINT('Ctrl Pts',(35.6555077526845,50.312500006828,35.6555077526845));
#15119=CARTESIAN_POINT('Ctrl Pts',(24.3531646875,50.1041666734946,42.1809185638422));
#15120=CARTESIAN_POINT('Ctrl Pts',(13.0508216223155,49.8958333401613,48.706329375));
#15121=CARTESIAN_POINT('Ctrl Pts',(-9.95098946405443E-15,49.687500006828,
48.706329375));
#15122=CARTESIAN_POINT('Ctrl Pts',(-13.0508216223155,49.4791666734946,48.706329375));
#15123=CARTESIAN_POINT('Ctrl Pts',(-24.3531646875,49.2708333401613,42.1809185638423));
#15124=CARTESIAN_POINT('Ctrl Pts',(-35.6555077526845,49.062500006828,35.6555077526845));
#15125=CARTESIAN_POINT('Ctrl Pts',(-42.1809185638422,48.8541666734946,24.3531646875));
#15126=CARTESIAN_POINT('Ctrl Pts',(-48.706329375,48.6458333401613,13.0508216223155));
#15127=CARTESIAN_POINT('Ctrl Pts',(-48.706329375,48.437500006828,-1.8898197019151E-14));
#15128=CARTESIAN_POINT('Ctrl Pts',(-48.706329375,48.2291666734946,-13.0508216223155));
#15129=CARTESIAN_POINT('Ctrl Pts',(-42.1809185638422,48.0208333401613,-24.3531646875));
#15130=CARTESIAN_POINT('Ctrl Pts',(-35.6555077526845,47.812500006828,-35.6555077526845));
#15131=CARTESIAN_POINT('Ctrl Pts',(-24.3531646875,47.6041666734946,-42.1809185638422));
#15132=CARTESIAN_POINT('Ctrl Pts',(-13.0508216223155,47.3958333401613,-48.706329375));
#15133=CARTESIAN_POINT('Ctrl Pts',(1.59157945007855E-14,47.187500006828,
-48.706329375));
#15134=CARTESIAN_POINT('Ctrl Pts',(13.0508216223155,46.9791666734946,-48.706329375));
#15135=CARTESIAN_POINT('Ctrl Pts',(24.3531646875,46.7708333401613,-42.1809185638422));
#15136=CARTESIAN_POINT('Ctrl Pts',(35.6555077526845,46.562500006828,-35.6555077526845));
#15137=CARTESIAN_POINT('Ctrl Pts',(42.1809185638422,46.3541666734946,-24.3531646875));
#15138=CARTESIAN_POINT('Ctrl Pts',(48.706329375,46.1458333401613,-13.0508216223155));
#15139=CARTESIAN_POINT('Ctrl Pts',(48.706329375,45.937500006828,1.293339198242E-14));
#15140=CARTESIAN_POINT('Ctrl Pts',(48.706329375,45.7291666734946,13.0508216223155));
#15141=CARTESIAN_POINT('Ctrl Pts',(42.1809185638422,45.5208333401613,24.3531646875));
#15142=CARTESIAN_POINT('Ctrl Pts',(35.6555077526845,45.312500006828,35.6555077526845));
#15143=CARTESIAN_POINT('Ctrl Pts',(24.3531646875,45.1041666734946,42.1809185638422));
#15144=CARTESIAN_POINT('Ctrl Pts',(13.0508216223155,44.8958333401613,48.706329375));
#15145=CARTESIAN_POINT('Ctrl Pts',(-9.95098946405443E-15,44.687500006828,
48.706329375));
#15146=CARTESIAN_POINT('Ctrl Pts',(-13.0508216223155,44.4791666734946,48.706329375));
#15147=CARTESIAN_POINT('Ctrl Pts',(-24.3531646875,44.2708333401613,42.1809185638423));
#15148=CARTESIAN_POINT('Ctrl Pts',(-35.6555077526845,44.062500006828,35.6555077526845));
#15149=CARTESIAN_POINT('Ctrl Pts',(-42.1809185638422,43.8541666734946,24.3531646875));
#15150=CARTESIAN_POINT('Ctrl Pts',(-48.706329375,43.6458333401613,13.0508216223155));
#15151=CARTESIAN_POINT('Ctrl Pts',(-48.706329375,43.437500006828,-1.8898197019151E-14));
#15152=CARTESIAN_POINT('Ctrl Pts',(-48.706329375,43.2291666734946,-13.0508216223155));
#15153=CARTESIAN_POINT('Ctrl Pts',(-42.1809185638422,43.0208333401613,-24.3531646875));
#15154=CARTESIAN_POINT('Ctrl Pts',(-35.6555077526845,42.812500006828,-35.6555077526845));
#15155=CARTESIAN_POINT('Ctrl Pts',(-24.3531646875,42.6041666734946,-42.1809185638422));
#15156=CARTESIAN_POINT('Ctrl Pts',(-13.0508216223155,42.3958333401613,-48.706329375));
#15157=CARTESIAN_POINT('Ctrl Pts',(1.59157945007855E-14,42.187500006828,
-48.706329375));
#15158=CARTESIAN_POINT('Ctrl Pts',(13.0508216223155,41.9791666734946,-48.706329375));
#15159=CARTESIAN_POINT('Ctrl Pts',(24.3531646875,41.7708333401613,-42.1809185638422));
#15160=CARTESIAN_POINT('Ctrl Pts',(35.6555077526845,41.562500006828,-35.6555077526845));
#15161=CARTESIAN_POINT('Ctrl Pts',(42.1809185638422,41.3541666734946,-24.3531646875));
#15162=CARTESIAN_POINT('Ctrl Pts',(48.706329375,41.1458333401613,-13.0508216223155));
#15163=CARTESIAN_POINT('Ctrl Pts',(48.706329375,40.937500006828,1.293339198242E-14));
#15164=CARTESIAN_POINT('Ctrl Pts',(48.706329375,40.7291666734946,13.0508216223155));
#15165=CARTESIAN_POINT('Ctrl Pts',(42.1809185638422,40.5208333401613,24.3531646875));
#15166=CARTESIAN_POINT('Ctrl Pts',(35.6555077526845,40.312500006828,35.6555077526845));
#15167=CARTESIAN_POINT('Ctrl Pts',(24.3531646875,40.1041666734946,42.1809185638422));
#15168=CARTESIAN_POINT('Ctrl Pts',(13.0508216223155,39.8958333401613,48.706329375));
#15169=CARTESIAN_POINT('Ctrl Pts',(-9.95098946405443E-15,39.687500006828,
48.706329375));
#15170=CARTESIAN_POINT('Ctrl Pts',(-13.0508216223155,39.4791666734946,48.706329375));
#15171=CARTESIAN_POINT('Ctrl Pts',(-24.3531646875,39.2708333401613,42.1809185638423));
#15172=CARTESIAN_POINT('Ctrl Pts',(-35.6555077526845,39.062500006828,35.6555077526845));
#15173=CARTESIAN_POINT('Ctrl Pts',(-42.1809185638422,38.8541666734946,24.3531646875));
#15174=CARTESIAN_POINT('Ctrl Pts',(-48.706329375,38.6458333401613,13.0508216223155));
#15175=CARTESIAN_POINT('Ctrl Pts',(-48.706329375,38.437500006828,-1.8898197019151E-14));
#15176=CARTESIAN_POINT('Ctrl Pts',(-48.706329375,38.2291666734946,-13.0508216223155));
#15177=CARTESIAN_POINT('Ctrl Pts',(-42.1809185638422,38.0208333401613,-24.3531646875));
#15178=CARTESIAN_POINT('Ctrl Pts',(-35.6555077526845,37.812500006828,-35.6555077526845));
#15179=CARTESIAN_POINT('Ctrl Pts',(-24.3531646875,37.6041666734946,-42.1809185638422));
#15180=CARTESIAN_POINT('Ctrl Pts',(-13.0508216223155,37.3958333401613,-48.706329375));
#15181=CARTESIAN_POINT('Ctrl Pts',(1.59157945007855E-14,37.187500006828,
-48.706329375));
#15182=CARTESIAN_POINT('Ctrl Pts',(13.0508216223155,36.9791666734946,-48.706329375));
#15183=CARTESIAN_POINT('Ctrl Pts',(24.3531646875,36.7708333401613,-42.1809185638422));
#15184=CARTESIAN_POINT('Ctrl Pts',(35.6555077526845,36.562500006828,-35.6555077526845));
#15185=CARTESIAN_POINT('Ctrl Pts',(42.1809185638422,36.3541666734946,-24.3531646875));
#15186=CARTESIAN_POINT('Ctrl Pts',(48.706329375,36.1458333401613,-13.0508216223155));
#15187=CARTESIAN_POINT('Ctrl Pts',(48.706329375,35.937500006828,1.293339198242E-14));
#15188=CARTESIAN_POINT('Ctrl Pts',(48.706329375,35.7291666734946,13.0508216223155));
#15189=CARTESIAN_POINT('Ctrl Pts',(42.1809185638422,35.5208333401613,24.3531646875));
#15190=CARTESIAN_POINT('Ctrl Pts',(35.6555077526845,35.312500006828,35.6555077526845));
#15191=CARTESIAN_POINT('Ctrl Pts',(24.3531646875,35.1041666734946,42.1809185638422));
#15192=CARTESIAN_POINT('Ctrl Pts',(13.0508216223155,34.8958333401613,48.706329375));
#15193=CARTESIAN_POINT('Ctrl Pts',(-9.95098946405443E-15,34.687500006828,
48.706329375));
#15194=CARTESIAN_POINT('Ctrl Pts',(-13.0508216223155,34.4791666734946,48.706329375));
#15195=CARTESIAN_POINT('Ctrl Pts',(-24.3531646875,34.2708333401613,42.1809185638423));
#15196=CARTESIAN_POINT('Ctrl Pts',(-35.6555077526845,34.062500006828,35.6555077526845));
#15197=CARTESIAN_POINT('Ctrl Pts',(-42.1809185638422,33.8541666734946,24.3531646875));
#15198=CARTESIAN_POINT('Ctrl Pts',(-48.706329375,33.6458333401613,13.0508216223155));
#15199=CARTESIAN_POINT('Ctrl Pts',(-48.706329375,33.437500006828,-1.8898197019151E-14));
#15200=CARTESIAN_POINT('Ctrl Pts',(-48.706329375,33.2291666734946,-13.0508216223155));
#15201=CARTESIAN_POINT('Ctrl Pts',(-42.1809185638422,33.0208333401613,-24.3531646875));
#15202=CARTESIAN_POINT('Ctrl Pts',(-35.6555077526845,32.812500006828,-35.6555077526845));
#15203=CARTESIAN_POINT('Ctrl Pts',(-24.3531646875,32.6041666734946,-42.1809185638422));
#15204=CARTESIAN_POINT('Ctrl Pts',(-13.0508216223155,32.3958333401613,-48.706329375));
#15205=CARTESIAN_POINT('Ctrl Pts',(1.59157945007855E-14,32.187500006828,
-48.706329375));
#15206=CARTESIAN_POINT('Ctrl Pts',(13.0508216223155,31.9791666734946,-48.706329375));
#15207=CARTESIAN_POINT('Ctrl Pts',(24.3531646875,31.7708333401613,-42.1809185638422));
#15208=CARTESIAN_POINT('Ctrl Pts',(35.6555077526845,31.562500006828,-35.6555077526845));
#15209=CARTESIAN_POINT('Ctrl Pts',(42.1809185638422,31.3541666734946,-24.3531646875));
#15210=CARTESIAN_POINT('Ctrl Pts',(48.706329375,31.1458333401613,-13.0508216223155));
#15211=CARTESIAN_POINT('Ctrl Pts',(48.706329375,30.937500006828,1.293339198242E-14));
#15212=CARTESIAN_POINT('Ctrl Pts',(48.706329375,30.7291666734946,13.0508216223155));
#15213=CARTESIAN_POINT('Ctrl Pts',(42.1809185638422,30.5208333401613,24.3531646875));
#15214=CARTESIAN_POINT('Ctrl Pts',(35.6555077526845,30.312500006828,35.6555077526845));
#15215=CARTESIAN_POINT('Ctrl Pts',(24.3531646875,30.1041666734946,42.1809185638422));
#15216=CARTESIAN_POINT('Ctrl Pts',(13.0508216223155,29.8958333401613,48.706329375));
#15217=CARTESIAN_POINT('Ctrl Pts',(-9.95098946405443E-15,29.687500006828,
48.706329375));
#15218=CARTESIAN_POINT('Ctrl Pts',(-13.0508216223155,29.4791666734946,48.706329375));
#15219=CARTESIAN_POINT('Ctrl Pts',(-24.3531646875,29.2708333401613,42.1809185638423));
#15220=CARTESIAN_POINT('Ctrl Pts',(-35.6555077526845,29.062500006828,35.6555077526845));
#15221=CARTESIAN_POINT('Ctrl Pts',(-42.1809185638422,28.8541666734946,24.3531646875));
#15222=CARTESIAN_POINT('Ctrl Pts',(-48.706329375,28.6458333401613,13.0508216223155));
#15223=CARTESIAN_POINT('Ctrl Pts',(-48.706329375,28.437500006828,-1.8898197019151E-14));
#15224=CARTESIAN_POINT('Ctrl Pts',(-46.,60.,0.));
#15225=CARTESIAN_POINT('Ctrl Pts',(-46.,59.7916666666667,-12.3256628518316));
#15226=CARTESIAN_POINT('Ctrl Pts',(-39.8371685740842,59.5833333333333,-23.));
#15227=CARTESIAN_POINT('Ctrl Pts',(-33.6743371481684,59.375,-33.6743371481684));
#15228=CARTESIAN_POINT('Ctrl Pts',(-23.,59.1666666666667,-39.8371685740842));
#15229=CARTESIAN_POINT('Ctrl Pts',(-12.3256628518317,58.9583333333333,-46.));
#15230=CARTESIAN_POINT('Ctrl Pts',(-2.81668763803891E-15,58.75,-46.));
#15231=CARTESIAN_POINT('Ctrl Pts',(12.3256628518316,58.5416666666667,-46.));
#15232=CARTESIAN_POINT('Ctrl Pts',(23.,58.3333333333333,-39.8371685740842));
#15233=CARTESIAN_POINT('Ctrl Pts',(33.6743371481683,58.125,-33.6743371481684));
#15234=CARTESIAN_POINT('Ctrl Pts',(39.8371685740842,57.9166666666667,-23.));
#15235=CARTESIAN_POINT('Ctrl Pts',(46.,57.7083333333333,-12.3256628518317));
#15236=CARTESIAN_POINT('Ctrl Pts',(46.,57.5,-5.63337527607782E-15));
#15237=CARTESIAN_POINT('Ctrl Pts',(46.,57.2916666666667,12.3256628518316));
#15238=CARTESIAN_POINT('Ctrl Pts',(39.8371685740842,57.0833333333333,23.));
#15239=CARTESIAN_POINT('Ctrl Pts',(33.6743371481684,56.875,33.6743371481683));
#15240=CARTESIAN_POINT('Ctrl Pts',(23.,56.6666666666667,39.8371685740842));
#15241=CARTESIAN_POINT('Ctrl Pts',(12.3256628518317,56.4583333333333,46.));
#15242=CARTESIAN_POINT('Ctrl Pts',(8.45006291411674E-15,56.25,46.));
#15243=CARTESIAN_POINT('Ctrl Pts',(-12.3256628518316,56.0416666666667,46.));
#15244=CARTESIAN_POINT('Ctrl Pts',(-23.,55.8333333333333,39.8371685740842));
#15245=CARTESIAN_POINT('Ctrl Pts',(-33.6743371481683,55.625,33.6743371481684));
#15246=CARTESIAN_POINT('Ctrl Pts',(-39.8371685740842,55.4166666666667,23.));
#15247=CARTESIAN_POINT('Ctrl Pts',(-46.,55.2083333333333,12.3256628518317));
#15248=CARTESIAN_POINT('Ctrl Pts',(-46.,55.,0.));
#15249=CARTESIAN_POINT('Ctrl Pts',(-46.,54.7916666666667,-12.3256628518316));
#15250=CARTESIAN_POINT('Ctrl Pts',(-39.8371685740842,54.5833333333333,-23.));
#15251=CARTESIAN_POINT('Ctrl Pts',(-33.6743371481684,54.375,-33.6743371481684));
#15252=CARTESIAN_POINT('Ctrl Pts',(-23.,54.1666666666667,-39.8371685740842));
#15253=CARTESIAN_POINT('Ctrl Pts',(-12.3256628518317,53.9583333333333,-46.));
#15254=CARTESIAN_POINT('Ctrl Pts',(-2.81668763803891E-15,53.75,-46.));
#15255=CARTESIAN_POINT('Ctrl Pts',(12.3256628518316,53.5416666666667,-46.));
#15256=CARTESIAN_POINT('Ctrl Pts',(23.,53.3333333333333,-39.8371685740842));
#15257=CARTESIAN_POINT('Ctrl Pts',(33.6743371481683,53.125,-33.6743371481684));
#15258=CARTESIAN_POINT('Ctrl Pts',(39.8371685740842,52.9166666666667,-23.));
#15259=CARTESIAN_POINT('Ctrl Pts',(46.,52.7083333333333,-12.3256628518317));
#15260=CARTESIAN_POINT('Ctrl Pts',(46.,52.5,-5.63337527607782E-15));
#15261=CARTESIAN_POINT('Ctrl Pts',(46.,52.2916666666667,12.3256628518316));
#15262=CARTESIAN_POINT('Ctrl Pts',(39.8371685740842,52.0833333333333,23.));
#15263=CARTESIAN_POINT('Ctrl Pts',(33.6743371481684,51.875,33.6743371481683));
#15264=CARTESIAN_POINT('Ctrl Pts',(23.,51.6666666666667,39.8371685740842));
#15265=CARTESIAN_POINT('Ctrl Pts',(12.3256628518317,51.4583333333333,46.));
#15266=CARTESIAN_POINT('Ctrl Pts',(8.45006291411674E-15,51.25,46.));
#15267=CARTESIAN_POINT('Ctrl Pts',(-12.3256628518316,51.0416666666667,46.));
#15268=CARTESIAN_POINT('Ctrl Pts',(-23.,50.8333333333333,39.8371685740842));
#15269=CARTESIAN_POINT('Ctrl Pts',(-33.6743371481683,50.625,33.6743371481684));
#15270=CARTESIAN_POINT('Ctrl Pts',(-39.8371685740842,50.4166666666667,23.));
#15271=CARTESIAN_POINT('Ctrl Pts',(-46.,50.2083333333333,12.3256628518317));
#15272=CARTESIAN_POINT('Ctrl Pts',(-46.,50.,0.));
#15273=CARTESIAN_POINT('Ctrl Pts',(-46.,49.7916666666667,-12.3256628518316));
#15274=CARTESIAN_POINT('Ctrl Pts',(-39.8371685740842,49.5833333333333,-23.));
#15275=CARTESIAN_POINT('Ctrl Pts',(-33.6743371481684,49.375,-33.6743371481684));
#15276=CARTESIAN_POINT('Ctrl Pts',(-23.,49.1666666666667,-39.8371685740842));
#15277=CARTESIAN_POINT('Ctrl Pts',(-12.3256628518317,48.9583333333333,-46.));
#15278=CARTESIAN_POINT('Ctrl Pts',(-2.81668763803891E-15,48.75,-46.));
#15279=CARTESIAN_POINT('Ctrl Pts',(12.3256628518316,48.5416666666667,-46.));
#15280=CARTESIAN_POINT('Ctrl Pts',(23.,48.3333333333333,-39.8371685740842));
#15281=CARTESIAN_POINT('Ctrl Pts',(33.6743371481683,48.125,-33.6743371481684));
#15282=CARTESIAN_POINT('Ctrl Pts',(39.8371685740842,47.9166666666667,-23.));
#15283=CARTESIAN_POINT('Ctrl Pts',(46.,47.7083333333333,-12.3256628518317));
#15284=CARTESIAN_POINT('Ctrl Pts',(46.,47.5,-5.63337527607782E-15));
#15285=CARTESIAN_POINT('Ctrl Pts',(46.,47.2916666666667,12.3256628518316));
#15286=CARTESIAN_POINT('Ctrl Pts',(39.8371685740842,47.0833333333333,23.));
#15287=CARTESIAN_POINT('Ctrl Pts',(33.6743371481684,46.875,33.6743371481683));
#15288=CARTESIAN_POINT('Ctrl Pts',(23.,46.6666666666667,39.8371685740842));
#15289=CARTESIAN_POINT('Ctrl Pts',(12.3256628518317,46.4583333333333,46.));
#15290=CARTESIAN_POINT('Ctrl Pts',(8.45006291411674E-15,46.25,46.));
#15291=CARTESIAN_POINT('Ctrl Pts',(-12.3256628518316,46.0416666666667,46.));
#15292=CARTESIAN_POINT('Ctrl Pts',(-23.,45.8333333333333,39.8371685740842));
#15293=CARTESIAN_POINT('Ctrl Pts',(-33.6743371481683,45.625,33.6743371481684));
#15294=CARTESIAN_POINT('Ctrl Pts',(-39.8371685740842,45.4166666666667,23.));
#15295=CARTESIAN_POINT('Ctrl Pts',(-46.,45.2083333333333,12.3256628518317));
#15296=CARTESIAN_POINT('Ctrl Pts',(-46.,45.,0.));
#15297=CARTESIAN_POINT('Ctrl Pts',(-46.,44.7916666666667,-12.3256628518316));
#15298=CARTESIAN_POINT('Ctrl Pts',(-39.8371685740842,44.5833333333333,-23.));
#15299=CARTESIAN_POINT('Ctrl Pts',(-33.6743371481684,44.375,-33.6743371481684));
#15300=CARTESIAN_POINT('Ctrl Pts',(-23.,44.1666666666667,-39.8371685740842));
#15301=CARTESIAN_POINT('Ctrl Pts',(-12.3256628518317,43.9583333333333,-46.));
#15302=CARTESIAN_POINT('Ctrl Pts',(-2.81668763803891E-15,43.75,-46.));
#15303=CARTESIAN_POINT('Ctrl Pts',(12.3256628518316,43.5416666666667,-46.));
#15304=CARTESIAN_POINT('Ctrl Pts',(23.,43.3333333333333,-39.8371685740842));
#15305=CARTESIAN_POINT('Ctrl Pts',(33.6743371481683,43.125,-33.6743371481684));
#15306=CARTESIAN_POINT('Ctrl Pts',(39.8371685740842,42.9166666666667,-23.));
#15307=CARTESIAN_POINT('Ctrl Pts',(46.,42.7083333333333,-12.3256628518317));
#15308=CARTESIAN_POINT('Ctrl Pts',(46.,42.5,-5.63337527607782E-15));
#15309=CARTESIAN_POINT('Ctrl Pts',(46.,42.2916666666667,12.3256628518316));
#15310=CARTESIAN_POINT('Ctrl Pts',(39.8371685740842,42.0833333333333,23.));
#15311=CARTESIAN_POINT('Ctrl Pts',(33.6743371481684,41.875,33.6743371481683));
#15312=CARTESIAN_POINT('Ctrl Pts',(23.,41.6666666666667,39.8371685740842));
#15313=CARTESIAN_POINT('Ctrl Pts',(12.3256628518317,41.4583333333333,46.));
#15314=CARTESIAN_POINT('Ctrl Pts',(8.45006291411674E-15,41.25,46.));
#15315=CARTESIAN_POINT('Ctrl Pts',(-12.3256628518316,41.0416666666667,46.));
#15316=CARTESIAN_POINT('Ctrl Pts',(-23.,40.8333333333333,39.8371685740842));
#15317=CARTESIAN_POINT('Ctrl Pts',(-33.6743371481683,40.625,33.6743371481684));
#15318=CARTESIAN_POINT('Ctrl Pts',(-39.8371685740842,40.4166666666667,23.));
#15319=CARTESIAN_POINT('Ctrl Pts',(-46.,40.2083333333333,12.3256628518317));
#15320=CARTESIAN_POINT('Ctrl Pts',(-46.,40.,0.));
#15321=CARTESIAN_POINT('Ctrl Pts',(-46.,39.7916666666667,-12.3256628518316));
#15322=CARTESIAN_POINT('Ctrl Pts',(-39.8371685740842,39.5833333333333,-23.));
#15323=CARTESIAN_POINT('Ctrl Pts',(-33.6743371481684,39.375,-33.6743371481684));
#15324=CARTESIAN_POINT('Ctrl Pts',(-23.,39.1666666666667,-39.8371685740842));
#15325=CARTESIAN_POINT('Ctrl Pts',(-12.3256628518317,38.9583333333333,-46.));
#15326=CARTESIAN_POINT('Ctrl Pts',(-2.81668763803891E-15,38.75,-46.));
#15327=CARTESIAN_POINT('Ctrl Pts',(12.3256628518316,38.5416666666667,-46.));
#15328=CARTESIAN_POINT('Ctrl Pts',(23.,38.3333333333333,-39.8371685740842));
#15329=CARTESIAN_POINT('Ctrl Pts',(33.6743371481683,38.125,-33.6743371481684));
#15330=CARTESIAN_POINT('Ctrl Pts',(39.8371685740842,37.9166666666667,-23.));
#15331=CARTESIAN_POINT('Ctrl Pts',(46.,37.7083333333333,-12.3256628518317));
#15332=CARTESIAN_POINT('Ctrl Pts',(46.,37.5,-5.63337527607782E-15));
#15333=CARTESIAN_POINT('Ctrl Pts',(46.,37.2916666666667,12.3256628518316));
#15334=CARTESIAN_POINT('Ctrl Pts',(39.8371685740842,37.0833333333333,23.));
#15335=CARTESIAN_POINT('Ctrl Pts',(33.6743371481684,36.875,33.6743371481683));
#15336=CARTESIAN_POINT('Ctrl Pts',(23.,36.6666666666667,39.8371685740842));
#15337=CARTESIAN_POINT('Ctrl Pts',(12.3256628518317,36.4583333333333,46.));
#15338=CARTESIAN_POINT('Ctrl Pts',(8.45006291411674E-15,36.25,46.));
#15339=CARTESIAN_POINT('Ctrl Pts',(-12.3256628518316,36.0416666666667,46.));
#15340=CARTESIAN_POINT('Ctrl Pts',(-23.,35.8333333333333,39.8371685740842));
#15341=CARTESIAN_POINT('Ctrl Pts',(-33.6743371481683,35.625,33.6743371481684));
#15342=CARTESIAN_POINT('Ctrl Pts',(-39.8371685740842,35.4166666666667,23.));
#15343=CARTESIAN_POINT('Ctrl Pts',(-46.,35.2083333333333,12.3256628518317));
#15344=CARTESIAN_POINT('Ctrl Pts',(-46.,35.,0.));
#15345=CARTESIAN_POINT('Ctrl Pts',(-46.,34.7916666666667,-12.3256628518316));
#15346=CARTESIAN_POINT('Ctrl Pts',(-39.8371685740842,34.5833333333333,-23.));
#15347=CARTESIAN_POINT('Ctrl Pts',(-33.6743371481684,34.375,-33.6743371481684));
#15348=CARTESIAN_POINT('Ctrl Pts',(-23.,34.1666666666667,-39.8371685740842));
#15349=CARTESIAN_POINT('Ctrl Pts',(-12.3256628518317,33.9583333333333,-46.));
#15350=CARTESIAN_POINT('Ctrl Pts',(-2.81668763803891E-15,33.75,-46.));
#15351=CARTESIAN_POINT('Ctrl Pts',(12.3256628518316,33.5416666666667,-46.));
#15352=CARTESIAN_POINT('Ctrl Pts',(23.,33.3333333333333,-39.8371685740842));
#15353=CARTESIAN_POINT('Ctrl Pts',(33.6743371481683,33.125,-33.6743371481684));
#15354=CARTESIAN_POINT('Ctrl Pts',(39.8371685740842,32.9166666666667,-23.));
#15355=CARTESIAN_POINT('Ctrl Pts',(46.,32.7083333333333,-12.3256628518317));
#15356=CARTESIAN_POINT('Ctrl Pts',(46.,32.5,-5.63337527607782E-15));
#15357=CARTESIAN_POINT('Ctrl Pts',(46.,32.2916666666667,12.3256628518316));
#15358=CARTESIAN_POINT('Ctrl Pts',(39.8371685740842,32.0833333333333,23.));
#15359=CARTESIAN_POINT('Ctrl Pts',(33.6743371481684,31.875,33.6743371481683));
#15360=CARTESIAN_POINT('Ctrl Pts',(23.,31.6666666666667,39.8371685740842));
#15361=CARTESIAN_POINT('Ctrl Pts',(12.3256628518317,31.4583333333333,46.));
#15362=CARTESIAN_POINT('Ctrl Pts',(8.45006291411674E-15,31.25,46.));
#15363=CARTESIAN_POINT('Ctrl Pts',(-12.3256628518316,31.0416666666667,46.));
#15364=CARTESIAN_POINT('Ctrl Pts',(-23.,30.8333333333333,39.8371685740842));
#15365=CARTESIAN_POINT('Ctrl Pts',(-33.6743371481683,30.625,33.6743371481684));
#15366=CARTESIAN_POINT('Ctrl Pts',(-39.8371685740842,30.4166666666667,23.));
#15367=CARTESIAN_POINT('Ctrl Pts',(-46.,30.2083333333333,12.3256628518317));
#15368=CARTESIAN_POINT('Ctrl Pts',(-46.,30.,0.));
#15369=CARTESIAN_POINT('Origin',(4513.80899804858,-7910.15855089474,-4.33048597777576));
#15370=CARTESIAN_POINT('Ctrl Pts',(-4.32456003949879,43.8240181593938,-45.7962681936506));
#15371=CARTESIAN_POINT('Ctrl Pts',(-4.32456003949876,43.6905125468623,-46.0278818021281));
#15372=CARTESIAN_POINT('Ctrl Pts',(-4.32456003949882,43.4234964717135,-46.4911062234486));
#15373=CARTESIAN_POINT('Ctrl Pts',(-4.32456003949885,43.1564711191154,-46.954325296818));
#15374=CARTESIAN_POINT('Ctrl Pts',(-4.32456003949885,42.7677643029224,-47.6286149142205));
#15375=CARTESIAN_POINT('Ctrl Pts',(-4.32456003949873,42.5125642776457,-48.0712916022845));
#15376=CARTESIAN_POINT('Ctrl Pts',(-4.32456003949873,42.2573567866782,-48.5139639861634));
#15377=CARTESIAN_POINT('Ctrl Pts',(-48.706329375,58.437500006828,-1.8898197019151E-14));
#15378=CARTESIAN_POINT('Ctrl Pts',(-48.706329375,58.2291666734946,-13.0508216223155));
#15379=CARTESIAN_POINT('Ctrl Pts',(-42.1809185638422,58.0208333401613,-24.3531646875));
#15380=CARTESIAN_POINT('Ctrl Pts',(-35.6555077526845,57.812500006828,-35.6555077526845));
#15381=CARTESIAN_POINT('Ctrl Pts',(-24.3531646875,57.6041666734946,-42.1809185638422));
#15382=CARTESIAN_POINT('Ctrl Pts',(-13.0508216223155,57.3958333401613,-48.706329375));
#15383=CARTESIAN_POINT('Ctrl Pts',(1.59157945007855E-14,57.187500006828,
-48.706329375));
#15384=CARTESIAN_POINT('Ctrl Pts',(13.0508216223155,56.9791666734946,-48.706329375));
#15385=CARTESIAN_POINT('Ctrl Pts',(24.3531646875,56.7708333401613,-42.1809185638422));
#15386=CARTESIAN_POINT('Ctrl Pts',(35.6555077526845,56.562500006828,-35.6555077526845));
#15387=CARTESIAN_POINT('Ctrl Pts',(42.1809185638422,56.3541666734946,-24.3531646875));
#15388=CARTESIAN_POINT('Ctrl Pts',(48.706329375,56.1458333401613,-13.0508216223155));
#15389=CARTESIAN_POINT('Ctrl Pts',(48.706329375,55.937500006828,1.293339198242E-14));
#15390=CARTESIAN_POINT('Ctrl Pts',(48.706329375,55.7291666734946,13.0508216223155));
#15391=CARTESIAN_POINT('Ctrl Pts',(42.1809185638422,55.5208333401613,24.3531646875));
#15392=CARTESIAN_POINT('Ctrl Pts',(35.6555077526845,55.312500006828,35.6555077526845));
#15393=CARTESIAN_POINT('Ctrl Pts',(24.3531646875,55.1041666734946,42.1809185638422));
#15394=CARTESIAN_POINT('Ctrl Pts',(13.0508216223155,54.8958333401613,48.706329375));
#15395=CARTESIAN_POINT('Ctrl Pts',(-9.95098946405443E-15,54.687500006828,
48.706329375));
#15396=CARTESIAN_POINT('Ctrl Pts',(-13.0508216223155,54.4791666734946,48.706329375));
#15397=CARTESIAN_POINT('Ctrl Pts',(-24.3531646875,54.2708333401613,42.1809185638423));
#15398=CARTESIAN_POINT('Ctrl Pts',(-35.6555077526845,54.062500006828,35.6555077526845));
#15399=CARTESIAN_POINT('Ctrl Pts',(-42.1809185638422,53.8541666734946,24.3531646875));
#15400=CARTESIAN_POINT('Ctrl Pts',(-48.706329375,53.6458333401613,13.0508216223155));
#15401=CARTESIAN_POINT('Ctrl Pts',(-48.706329375,53.437500006828,-1.8898197019151E-14));
#15402=CARTESIAN_POINT('Ctrl Pts',(-48.706329375,53.2291666734946,-13.0508216223155));
#15403=CARTESIAN_POINT('Ctrl Pts',(-42.1809185638422,53.0208333401613,-24.3531646875));
#15404=CARTESIAN_POINT('Ctrl Pts',(-35.6555077526845,52.812500006828,-35.6555077526845));
#15405=CARTESIAN_POINT('Ctrl Pts',(-24.3531646875,52.6041666734946,-42.1809185638422));
#15406=CARTESIAN_POINT('Ctrl Pts',(-13.0508216223155,52.3958333401613,-48.706329375));
#15407=CARTESIAN_POINT('Ctrl Pts',(1.59157945007855E-14,52.187500006828,
-48.706329375));
#15408=CARTESIAN_POINT('Ctrl Pts',(13.0508216223155,51.9791666734946,-48.706329375));
#15409=CARTESIAN_POINT('Ctrl Pts',(24.3531646875,51.7708333401613,-42.1809185638422));
#15410=CARTESIAN_POINT('Ctrl Pts',(35.6555077526845,51.562500006828,-35.6555077526845));
#15411=CARTESIAN_POINT('Ctrl Pts',(42.1809185638422,51.3541666734946,-24.3531646875));
#15412=CARTESIAN_POINT('Ctrl Pts',(48.706329375,51.1458333401613,-13.0508216223155));
#15413=CARTESIAN_POINT('Ctrl Pts',(48.706329375,50.937500006828,1.293339198242E-14));
#15414=CARTESIAN_POINT('Ctrl Pts',(48.706329375,50.7291666734946,13.0508216223155));
#15415=CARTESIAN_POINT('Ctrl Pts',(42.1809185638422,50.5208333401613,24.3531646875));
#15416=CARTESIAN_POINT('Ctrl Pts',(35.6555077526845,50.312500006828,35.6555077526845));
#15417=CARTESIAN_POINT('Ctrl Pts',(24.3531646875,50.1041666734946,42.1809185638422));
#15418=CARTESIAN_POINT('Ctrl Pts',(13.0508216223155,49.8958333401613,48.706329375));
#15419=CARTESIAN_POINT('Ctrl Pts',(-9.95098946405443E-15,49.687500006828,
48.706329375));
#15420=CARTESIAN_POINT('Ctrl Pts',(-13.0508216223155,49.4791666734946,48.706329375));
#15421=CARTESIAN_POINT('Ctrl Pts',(-24.3531646875,49.2708333401613,42.1809185638423));
#15422=CARTESIAN_POINT('Ctrl Pts',(-35.6555077526845,49.062500006828,35.6555077526845));
#15423=CARTESIAN_POINT('Ctrl Pts',(-42.1809185638422,48.8541666734946,24.3531646875));
#15424=CARTESIAN_POINT('Ctrl Pts',(-48.706329375,48.6458333401613,13.0508216223155));
#15425=CARTESIAN_POINT('Ctrl Pts',(-48.706329375,48.437500006828,-1.8898197019151E-14));
#15426=CARTESIAN_POINT('Ctrl Pts',(-48.706329375,48.2291666734946,-13.0508216223155));
#15427=CARTESIAN_POINT('Ctrl Pts',(-42.1809185638422,48.0208333401613,-24.3531646875));
#15428=CARTESIAN_POINT('Ctrl Pts',(-35.6555077526845,47.812500006828,-35.6555077526845));
#15429=CARTESIAN_POINT('Ctrl Pts',(-24.3531646875,47.6041666734946,-42.1809185638422));
#15430=CARTESIAN_POINT('Ctrl Pts',(-13.0508216223155,47.3958333401613,-48.706329375));
#15431=CARTESIAN_POINT('Ctrl Pts',(1.59157945007855E-14,47.187500006828,
-48.706329375));
#15432=CARTESIAN_POINT('Ctrl Pts',(13.0508216223155,46.9791666734946,-48.706329375));
#15433=CARTESIAN_POINT('Ctrl Pts',(24.3531646875,46.7708333401613,-42.1809185638422));
#15434=CARTESIAN_POINT('Ctrl Pts',(35.6555077526845,46.562500006828,-35.6555077526845));
#15435=CARTESIAN_POINT('Ctrl Pts',(42.1809185638422,46.3541666734946,-24.3531646875));
#15436=CARTESIAN_POINT('Ctrl Pts',(48.706329375,46.1458333401613,-13.0508216223155));
#15437=CARTESIAN_POINT('Ctrl Pts',(48.706329375,45.937500006828,1.293339198242E-14));
#15438=CARTESIAN_POINT('Ctrl Pts',(48.706329375,45.7291666734946,13.0508216223155));
#15439=CARTESIAN_POINT('Ctrl Pts',(42.1809185638422,45.5208333401613,24.3531646875));
#15440=CARTESIAN_POINT('Ctrl Pts',(35.6555077526845,45.312500006828,35.6555077526845));
#15441=CARTESIAN_POINT('Ctrl Pts',(24.3531646875,45.1041666734946,42.1809185638422));
#15442=CARTESIAN_POINT('Ctrl Pts',(13.0508216223155,44.8958333401613,48.706329375));
#15443=CARTESIAN_POINT('Ctrl Pts',(-9.95098946405443E-15,44.687500006828,
48.706329375));
#15444=CARTESIAN_POINT('Ctrl Pts',(-13.0508216223155,44.4791666734946,48.706329375));
#15445=CARTESIAN_POINT('Ctrl Pts',(-24.3531646875,44.2708333401613,42.1809185638423));
#15446=CARTESIAN_POINT('Ctrl Pts',(-35.6555077526845,44.062500006828,35.6555077526845));
#15447=CARTESIAN_POINT('Ctrl Pts',(-42.1809185638422,43.8541666734946,24.3531646875));
#15448=CARTESIAN_POINT('Ctrl Pts',(-48.706329375,43.6458333401613,13.0508216223155));
#15449=CARTESIAN_POINT('Ctrl Pts',(-48.706329375,43.437500006828,-1.8898197019151E-14));
#15450=CARTESIAN_POINT('Ctrl Pts',(-48.706329375,43.2291666734946,-13.0508216223155));
#15451=CARTESIAN_POINT('Ctrl Pts',(-42.1809185638422,43.0208333401613,-24.3531646875));
#15452=CARTESIAN_POINT('Ctrl Pts',(-35.6555077526845,42.812500006828,-35.6555077526845));
#15453=CARTESIAN_POINT('Ctrl Pts',(-24.3531646875,42.6041666734946,-42.1809185638422));
#15454=CARTESIAN_POINT('Ctrl Pts',(-13.0508216223155,42.3958333401613,-48.706329375));
#15455=CARTESIAN_POINT('Ctrl Pts',(1.59157945007855E-14,42.187500006828,
-48.706329375));
#15456=CARTESIAN_POINT('Ctrl Pts',(13.0508216223155,41.9791666734946,-48.706329375));
#15457=CARTESIAN_POINT('Ctrl Pts',(24.3531646875,41.7708333401613,-42.1809185638422));
#15458=CARTESIAN_POINT('Ctrl Pts',(35.6555077526845,41.562500006828,-35.6555077526845));
#15459=CARTESIAN_POINT('Ctrl Pts',(42.1809185638422,41.3541666734946,-24.3531646875));
#15460=CARTESIAN_POINT('Ctrl Pts',(48.706329375,41.1458333401613,-13.0508216223155));
#15461=CARTESIAN_POINT('Ctrl Pts',(48.706329375,40.937500006828,1.293339198242E-14));
#15462=CARTESIAN_POINT('Ctrl Pts',(48.706329375,40.7291666734946,13.0508216223155));
#15463=CARTESIAN_POINT('Ctrl Pts',(42.1809185638422,40.5208333401613,24.3531646875));
#15464=CARTESIAN_POINT('Ctrl Pts',(35.6555077526845,40.312500006828,35.6555077526845));
#15465=CARTESIAN_POINT('Ctrl Pts',(24.3531646875,40.1041666734946,42.1809185638422));
#15466=CARTESIAN_POINT('Ctrl Pts',(13.0508216223155,39.8958333401613,48.706329375));
#15467=CARTESIAN_POINT('Ctrl Pts',(-9.95098946405443E-15,39.687500006828,
48.706329375));
#15468=CARTESIAN_POINT('Ctrl Pts',(-13.0508216223155,39.4791666734946,48.706329375));
#15469=CARTESIAN_POINT('Ctrl Pts',(-24.3531646875,39.2708333401613,42.1809185638423));
#15470=CARTESIAN_POINT('Ctrl Pts',(-35.6555077526845,39.062500006828,35.6555077526845));
#15471=CARTESIAN_POINT('Ctrl Pts',(-42.1809185638422,38.8541666734946,24.3531646875));
#15472=CARTESIAN_POINT('Ctrl Pts',(-48.706329375,38.6458333401613,13.0508216223155));
#15473=CARTESIAN_POINT('Ctrl Pts',(-48.706329375,38.437500006828,-1.8898197019151E-14));
#15474=CARTESIAN_POINT('Ctrl Pts',(-48.706329375,38.2291666734946,-13.0508216223155));
#15475=CARTESIAN_POINT('Ctrl Pts',(-42.1809185638422,38.0208333401613,-24.3531646875));
#15476=CARTESIAN_POINT('Ctrl Pts',(-35.6555077526845,37.812500006828,-35.6555077526845));
#15477=CARTESIAN_POINT('Ctrl Pts',(-24.3531646875,37.6041666734946,-42.1809185638422));
#15478=CARTESIAN_POINT('Ctrl Pts',(-13.0508216223155,37.3958333401613,-48.706329375));
#15479=CARTESIAN_POINT('Ctrl Pts',(1.59157945007855E-14,37.187500006828,
-48.706329375));
#15480=CARTESIAN_POINT('Ctrl Pts',(13.0508216223155,36.9791666734946,-48.706329375));
#15481=CARTESIAN_POINT('Ctrl Pts',(24.3531646875,36.7708333401613,-42.1809185638422));
#15482=CARTESIAN_POINT('Ctrl Pts',(35.6555077526845,36.562500006828,-35.6555077526845));
#15483=CARTESIAN_POINT('Ctrl Pts',(42.1809185638422,36.3541666734946,-24.3531646875));
#15484=CARTESIAN_POINT('Ctrl Pts',(48.706329375,36.1458333401613,-13.0508216223155));
#15485=CARTESIAN_POINT('Ctrl Pts',(48.706329375,35.937500006828,1.293339198242E-14));
#15486=CARTESIAN_POINT('Ctrl Pts',(48.706329375,35.7291666734946,13.0508216223155));
#15487=CARTESIAN_POINT('Ctrl Pts',(42.1809185638422,35.5208333401613,24.3531646875));
#15488=CARTESIAN_POINT('Ctrl Pts',(35.6555077526845,35.312500006828,35.6555077526845));
#15489=CARTESIAN_POINT('Ctrl Pts',(24.3531646875,35.1041666734946,42.1809185638422));
#15490=CARTESIAN_POINT('Ctrl Pts',(13.0508216223155,34.8958333401613,48.706329375));
#15491=CARTESIAN_POINT('Ctrl Pts',(-9.95098946405443E-15,34.687500006828,
48.706329375));
#15492=CARTESIAN_POINT('Ctrl Pts',(-13.0508216223155,34.4791666734946,48.706329375));
#15493=CARTESIAN_POINT('Ctrl Pts',(-24.3531646875,34.2708333401613,42.1809185638423));
#15494=CARTESIAN_POINT('Ctrl Pts',(-35.6555077526845,34.062500006828,35.6555077526845));
#15495=CARTESIAN_POINT('Ctrl Pts',(-42.1809185638422,33.8541666734946,24.3531646875));
#15496=CARTESIAN_POINT('Ctrl Pts',(-48.706329375,33.6458333401613,13.0508216223155));
#15497=CARTESIAN_POINT('Ctrl Pts',(-48.706329375,33.437500006828,-1.8898197019151E-14));
#15498=CARTESIAN_POINT('Ctrl Pts',(-48.706329375,33.2291666734946,-13.0508216223155));
#15499=CARTESIAN_POINT('Ctrl Pts',(-42.1809185638422,33.0208333401613,-24.3531646875));
#15500=CARTESIAN_POINT('Ctrl Pts',(-35.6555077526845,32.812500006828,-35.6555077526845));
#15501=CARTESIAN_POINT('Ctrl Pts',(-24.3531646875,32.6041666734946,-42.1809185638422));
#15502=CARTESIAN_POINT('Ctrl Pts',(-13.0508216223155,32.3958333401613,-48.706329375));
#15503=CARTESIAN_POINT('Ctrl Pts',(1.59157945007855E-14,32.187500006828,
-48.706329375));
#15504=CARTESIAN_POINT('Ctrl Pts',(13.0508216223155,31.9791666734946,-48.706329375));
#15505=CARTESIAN_POINT('Ctrl Pts',(24.3531646875,31.7708333401613,-42.1809185638422));
#15506=CARTESIAN_POINT('Ctrl Pts',(35.6555077526845,31.562500006828,-35.6555077526845));
#15507=CARTESIAN_POINT('Ctrl Pts',(42.1809185638422,31.3541666734946,-24.3531646875));
#15508=CARTESIAN_POINT('Ctrl Pts',(48.706329375,31.1458333401613,-13.0508216223155));
#15509=CARTESIAN_POINT('Ctrl Pts',(48.706329375,30.937500006828,1.293339198242E-14));
#15510=CARTESIAN_POINT('Ctrl Pts',(48.706329375,30.7291666734946,13.0508216223155));
#15511=CARTESIAN_POINT('Ctrl Pts',(42.1809185638422,30.5208333401613,24.3531646875));
#15512=CARTESIAN_POINT('Ctrl Pts',(35.6555077526845,30.312500006828,35.6555077526845));
#15513=CARTESIAN_POINT('Ctrl Pts',(24.3531646875,30.1041666734946,42.1809185638422));
#15514=CARTESIAN_POINT('Ctrl Pts',(13.0508216223155,29.8958333401613,48.706329375));
#15515=CARTESIAN_POINT('Ctrl Pts',(-9.95098946405443E-15,29.687500006828,
48.706329375));
#15516=CARTESIAN_POINT('Ctrl Pts',(-13.0508216223155,29.4791666734946,48.706329375));
#15517=CARTESIAN_POINT('Ctrl Pts',(-24.3531646875,29.2708333401613,42.1809185638423));
#15518=CARTESIAN_POINT('Ctrl Pts',(-35.6555077526845,29.062500006828,35.6555077526845));
#15519=CARTESIAN_POINT('Ctrl Pts',(-42.1809185638422,28.8541666734946,24.3531646875));
#15520=CARTESIAN_POINT('Ctrl Pts',(-48.706329375,28.6458333401613,13.0508216223155));
#15521=CARTESIAN_POINT('Ctrl Pts',(-48.706329375,28.437500006828,-1.8898197019151E-14));
#15522=CARTESIAN_POINT('Ctrl Pts',(-46.,60.,0.));
#15523=CARTESIAN_POINT('Ctrl Pts',(-46.,59.7916666666667,-12.3256628518316));
#15524=CARTESIAN_POINT('Ctrl Pts',(-39.8371685740842,59.5833333333333,-23.));
#15525=CARTESIAN_POINT('Ctrl Pts',(-33.6743371481684,59.375,-33.6743371481684));
#15526=CARTESIAN_POINT('Ctrl Pts',(-23.,59.1666666666667,-39.8371685740842));
#15527=CARTESIAN_POINT('Ctrl Pts',(-12.3256628518317,58.9583333333333,-46.));
#15528=CARTESIAN_POINT('Ctrl Pts',(-2.81668763803891E-15,58.75,-46.));
#15529=CARTESIAN_POINT('Ctrl Pts',(12.3256628518316,58.5416666666667,-46.));
#15530=CARTESIAN_POINT('Ctrl Pts',(23.,58.3333333333333,-39.8371685740842));
#15531=CARTESIAN_POINT('Ctrl Pts',(33.6743371481683,58.125,-33.6743371481684));
#15532=CARTESIAN_POINT('Ctrl Pts',(39.8371685740842,57.9166666666667,-23.));
#15533=CARTESIAN_POINT('Ctrl Pts',(46.,57.7083333333333,-12.3256628518317));
#15534=CARTESIAN_POINT('Ctrl Pts',(46.,57.5,-5.63337527607782E-15));
#15535=CARTESIAN_POINT('Ctrl Pts',(46.,57.2916666666667,12.3256628518316));
#15536=CARTESIAN_POINT('Ctrl Pts',(39.8371685740842,57.0833333333333,23.));
#15537=CARTESIAN_POINT('Ctrl Pts',(33.6743371481684,56.875,33.6743371481683));
#15538=CARTESIAN_POINT('Ctrl Pts',(23.,56.6666666666667,39.8371685740842));
#15539=CARTESIAN_POINT('Ctrl Pts',(12.3256628518317,56.4583333333333,46.));
#15540=CARTESIAN_POINT('Ctrl Pts',(8.45006291411674E-15,56.25,46.));
#15541=CARTESIAN_POINT('Ctrl Pts',(-12.3256628518316,56.0416666666667,46.));
#15542=CARTESIAN_POINT('Ctrl Pts',(-23.,55.8333333333333,39.8371685740842));
#15543=CARTESIAN_POINT('Ctrl Pts',(-33.6743371481683,55.625,33.6743371481684));
#15544=CARTESIAN_POINT('Ctrl Pts',(-39.8371685740842,55.4166666666667,23.));
#15545=CARTESIAN_POINT('Ctrl Pts',(-46.,55.2083333333333,12.3256628518317));
#15546=CARTESIAN_POINT('Ctrl Pts',(-46.,55.,0.));
#15547=CARTESIAN_POINT('Ctrl Pts',(-46.,54.7916666666667,-12.3256628518316));
#15548=CARTESIAN_POINT('Ctrl Pts',(-39.8371685740842,54.5833333333333,-23.));
#15549=CARTESIAN_POINT('Ctrl Pts',(-33.6743371481684,54.375,-33.6743371481684));
#15550=CARTESIAN_POINT('Ctrl Pts',(-23.,54.1666666666667,-39.8371685740842));
#15551=CARTESIAN_POINT('Ctrl Pts',(-12.3256628518317,53.9583333333333,-46.));
#15552=CARTESIAN_POINT('Ctrl Pts',(-2.81668763803891E-15,53.75,-46.));
#15553=CARTESIAN_POINT('Ctrl Pts',(12.3256628518316,53.5416666666667,-46.));
#15554=CARTESIAN_POINT('Ctrl Pts',(23.,53.3333333333333,-39.8371685740842));
#15555=CARTESIAN_POINT('Ctrl Pts',(33.6743371481683,53.125,-33.6743371481684));
#15556=CARTESIAN_POINT('Ctrl Pts',(39.8371685740842,52.9166666666667,-23.));
#15557=CARTESIAN_POINT('Ctrl Pts',(46.,52.7083333333333,-12.3256628518317));
#15558=CARTESIAN_POINT('Ctrl Pts',(46.,52.5,-5.63337527607782E-15));
#15559=CARTESIAN_POINT('Ctrl Pts',(46.,52.2916666666667,12.3256628518316));
#15560=CARTESIAN_POINT('Ctrl Pts',(39.8371685740842,52.0833333333333,23.));
#15561=CARTESIAN_POINT('Ctrl Pts',(33.6743371481684,51.875,33.6743371481683));
#15562=CARTESIAN_POINT('Ctrl Pts',(23.,51.6666666666667,39.8371685740842));
#15563=CARTESIAN_POINT('Ctrl Pts',(12.3256628518317,51.4583333333333,46.));
#15564=CARTESIAN_POINT('Ctrl Pts',(8.45006291411674E-15,51.25,46.));
#15565=CARTESIAN_POINT('Ctrl Pts',(-12.3256628518316,51.0416666666667,46.));
#15566=CARTESIAN_POINT('Ctrl Pts',(-23.,50.8333333333333,39.8371685740842));
#15567=CARTESIAN_POINT('Ctrl Pts',(-33.6743371481683,50.625,33.6743371481684));
#15568=CARTESIAN_POINT('Ctrl Pts',(-39.8371685740842,50.4166666666667,23.));
#15569=CARTESIAN_POINT('Ctrl Pts',(-46.,50.2083333333333,12.3256628518317));
#15570=CARTESIAN_POINT('Ctrl Pts',(-46.,50.,0.));
#15571=CARTESIAN_POINT('Ctrl Pts',(-46.,49.7916666666667,-12.3256628518316));
#15572=CARTESIAN_POINT('Ctrl Pts',(-39.8371685740842,49.5833333333333,-23.));
#15573=CARTESIAN_POINT('Ctrl Pts',(-33.6743371481684,49.375,-33.6743371481684));
#15574=CARTESIAN_POINT('Ctrl Pts',(-23.,49.1666666666667,-39.8371685740842));
#15575=CARTESIAN_POINT('Ctrl Pts',(-12.3256628518317,48.9583333333333,-46.));
#15576=CARTESIAN_POINT('Ctrl Pts',(-2.81668763803891E-15,48.75,-46.));
#15577=CARTESIAN_POINT('Ctrl Pts',(12.3256628518316,48.5416666666667,-46.));
#15578=CARTESIAN_POINT('Ctrl Pts',(23.,48.3333333333333,-39.8371685740842));
#15579=CARTESIAN_POINT('Ctrl Pts',(33.6743371481683,48.125,-33.6743371481684));
#15580=CARTESIAN_POINT('Ctrl Pts',(39.8371685740842,47.9166666666667,-23.));
#15581=CARTESIAN_POINT('Ctrl Pts',(46.,47.7083333333333,-12.3256628518317));
#15582=CARTESIAN_POINT('Ctrl Pts',(46.,47.5,-5.63337527607782E-15));
#15583=CARTESIAN_POINT('Ctrl Pts',(46.,47.2916666666667,12.3256628518316));
#15584=CARTESIAN_POINT('Ctrl Pts',(39.8371685740842,47.0833333333333,23.));
#15585=CARTESIAN_POINT('Ctrl Pts',(33.6743371481684,46.875,33.6743371481683));
#15586=CARTESIAN_POINT('Ctrl Pts',(23.,46.6666666666667,39.8371685740842));
#15587=CARTESIAN_POINT('Ctrl Pts',(12.3256628518317,46.4583333333333,46.));
#15588=CARTESIAN_POINT('Ctrl Pts',(8.45006291411674E-15,46.25,46.));
#15589=CARTESIAN_POINT('Ctrl Pts',(-12.3256628518316,46.0416666666667,46.));
#15590=CARTESIAN_POINT('Ctrl Pts',(-23.,45.8333333333333,39.8371685740842));
#15591=CARTESIAN_POINT('Ctrl Pts',(-33.6743371481683,45.625,33.6743371481684));
#15592=CARTESIAN_POINT('Ctrl Pts',(-39.8371685740842,45.4166666666667,23.));
#15593=CARTESIAN_POINT('Ctrl Pts',(-46.,45.2083333333333,12.3256628518317));
#15594=CARTESIAN_POINT('Ctrl Pts',(-46.,45.,0.));
#15595=CARTESIAN_POINT('Ctrl Pts',(-46.,44.7916666666667,-12.3256628518316));
#15596=CARTESIAN_POINT('Ctrl Pts',(-39.8371685740842,44.5833333333333,-23.));
#15597=CARTESIAN_POINT('Ctrl Pts',(-33.6743371481684,44.375,-33.6743371481684));
#15598=CARTESIAN_POINT('Ctrl Pts',(-23.,44.1666666666667,-39.8371685740842));
#15599=CARTESIAN_POINT('Ctrl Pts',(-12.3256628518317,43.9583333333333,-46.));
#15600=CARTESIAN_POINT('Ctrl Pts',(-2.81668763803891E-15,43.75,-46.));
#15601=CARTESIAN_POINT('Ctrl Pts',(12.3256628518316,43.5416666666667,-46.));
#15602=CARTESIAN_POINT('Ctrl Pts',(23.,43.3333333333333,-39.8371685740842));
#15603=CARTESIAN_POINT('Ctrl Pts',(33.6743371481683,43.125,-33.6743371481684));
#15604=CARTESIAN_POINT('Ctrl Pts',(39.8371685740842,42.9166666666667,-23.));
#15605=CARTESIAN_POINT('Ctrl Pts',(46.,42.7083333333333,-12.3256628518317));
#15606=CARTESIAN_POINT('Ctrl Pts',(46.,42.5,-5.63337527607782E-15));
#15607=CARTESIAN_POINT('Ctrl Pts',(46.,42.2916666666667,12.3256628518316));
#15608=CARTESIAN_POINT('Ctrl Pts',(39.8371685740842,42.0833333333333,23.));
#15609=CARTESIAN_POINT('Ctrl Pts',(33.6743371481684,41.875,33.6743371481683));
#15610=CARTESIAN_POINT('Ctrl Pts',(23.,41.6666666666667,39.8371685740842));
#15611=CARTESIAN_POINT('Ctrl Pts',(12.3256628518317,41.4583333333333,46.));
#15612=CARTESIAN_POINT('Ctrl Pts',(8.45006291411674E-15,41.25,46.));
#15613=CARTESIAN_POINT('Ctrl Pts',(-12.3256628518316,41.0416666666667,46.));
#15614=CARTESIAN_POINT('Ctrl Pts',(-23.,40.8333333333333,39.8371685740842));
#15615=CARTESIAN_POINT('Ctrl Pts',(-33.6743371481683,40.625,33.6743371481684));
#15616=CARTESIAN_POINT('Ctrl Pts',(-39.8371685740842,40.4166666666667,23.));
#15617=CARTESIAN_POINT('Ctrl Pts',(-46.,40.2083333333333,12.3256628518317));
#15618=CARTESIAN_POINT('Ctrl Pts',(-46.,40.,0.));
#15619=CARTESIAN_POINT('Ctrl Pts',(-46.,39.7916666666667,-12.3256628518316));
#15620=CARTESIAN_POINT('Ctrl Pts',(-39.8371685740842,39.5833333333333,-23.));
#15621=CARTESIAN_POINT('Ctrl Pts',(-33.6743371481684,39.375,-33.6743371481684));
#15622=CARTESIAN_POINT('Ctrl Pts',(-23.,39.1666666666667,-39.8371685740842));
#15623=CARTESIAN_POINT('Ctrl Pts',(-12.3256628518317,38.9583333333333,-46.));
#15624=CARTESIAN_POINT('Ctrl Pts',(-2.81668763803891E-15,38.75,-46.));
#15625=CARTESIAN_POINT('Ctrl Pts',(12.3256628518316,38.5416666666667,-46.));
#15626=CARTESIAN_POINT('Ctrl Pts',(23.,38.3333333333333,-39.8371685740842));
#15627=CARTESIAN_POINT('Ctrl Pts',(33.6743371481683,38.125,-33.6743371481684));
#15628=CARTESIAN_POINT('Ctrl Pts',(39.8371685740842,37.9166666666667,-23.));
#15629=CARTESIAN_POINT('Ctrl Pts',(46.,37.7083333333333,-12.3256628518317));
#15630=CARTESIAN_POINT('Ctrl Pts',(46.,37.5,-5.63337527607782E-15));
#15631=CARTESIAN_POINT('Ctrl Pts',(46.,37.2916666666667,12.3256628518316));
#15632=CARTESIAN_POINT('Ctrl Pts',(39.8371685740842,37.0833333333333,23.));
#15633=CARTESIAN_POINT('Ctrl Pts',(33.6743371481684,36.875,33.6743371481683));
#15634=CARTESIAN_POINT('Ctrl Pts',(23.,36.6666666666667,39.8371685740842));
#15635=CARTESIAN_POINT('Ctrl Pts',(12.3256628518317,36.4583333333333,46.));
#15636=CARTESIAN_POINT('Ctrl Pts',(8.45006291411674E-15,36.25,46.));
#15637=CARTESIAN_POINT('Ctrl Pts',(-12.3256628518316,36.0416666666667,46.));
#15638=CARTESIAN_POINT('Ctrl Pts',(-23.,35.8333333333333,39.8371685740842));
#15639=CARTESIAN_POINT('Ctrl Pts',(-33.6743371481683,35.625,33.6743371481684));
#15640=CARTESIAN_POINT('Ctrl Pts',(-39.8371685740842,35.4166666666667,23.));
#15641=CARTESIAN_POINT('Ctrl Pts',(-46.,35.2083333333333,12.3256628518317));
#15642=CARTESIAN_POINT('Ctrl Pts',(-46.,35.,0.));
#15643=CARTESIAN_POINT('Ctrl Pts',(-46.,34.7916666666667,-12.3256628518316));
#15644=CARTESIAN_POINT('Ctrl Pts',(-39.8371685740842,34.5833333333333,-23.));
#15645=CARTESIAN_POINT('Ctrl Pts',(-33.6743371481684,34.375,-33.6743371481684));
#15646=CARTESIAN_POINT('Ctrl Pts',(-23.,34.1666666666667,-39.8371685740842));
#15647=CARTESIAN_POINT('Ctrl Pts',(-12.3256628518317,33.9583333333333,-46.));
#15648=CARTESIAN_POINT('Ctrl Pts',(-2.81668763803891E-15,33.75,-46.));
#15649=CARTESIAN_POINT('Ctrl Pts',(12.3256628518316,33.5416666666667,-46.));
#15650=CARTESIAN_POINT('Ctrl Pts',(23.,33.3333333333333,-39.8371685740842));
#15651=CARTESIAN_POINT('Ctrl Pts',(33.6743371481683,33.125,-33.6743371481684));
#15652=CARTESIAN_POINT('Ctrl Pts',(39.8371685740842,32.9166666666667,-23.));
#15653=CARTESIAN_POINT('Ctrl Pts',(46.,32.7083333333333,-12.3256628518317));
#15654=CARTESIAN_POINT('Ctrl Pts',(46.,32.5,-5.63337527607782E-15));
#15655=CARTESIAN_POINT('Ctrl Pts',(46.,32.2916666666667,12.3256628518316));
#15656=CARTESIAN_POINT('Ctrl Pts',(39.8371685740842,32.0833333333333,23.));
#15657=CARTESIAN_POINT('Ctrl Pts',(33.6743371481684,31.875,33.6743371481683));
#15658=CARTESIAN_POINT('Ctrl Pts',(23.,31.6666666666667,39.8371685740842));
#15659=CARTESIAN_POINT('Ctrl Pts',(12.3256628518317,31.4583333333333,46.));
#15660=CARTESIAN_POINT('Ctrl Pts',(8.45006291411674E-15,31.25,46.));
#15661=CARTESIAN_POINT('Ctrl Pts',(-12.3256628518316,31.0416666666667,46.));
#15662=CARTESIAN_POINT('Ctrl Pts',(-23.,30.8333333333333,39.8371685740842));
#15663=CARTESIAN_POINT('Ctrl Pts',(-33.6743371481683,30.625,33.6743371481684));
#15664=CARTESIAN_POINT('Ctrl Pts',(-39.8371685740842,30.4166666666667,23.));
#15665=CARTESIAN_POINT('Ctrl Pts',(-46.,30.2083333333333,12.3256628518317));
#15666=CARTESIAN_POINT('Ctrl Pts',(-46.,30.,0.));
#15667=CARTESIAN_POINT('Ctrl Pts',(-45.858362923034,45.061608680256,3.60701400320326));
#15668=CARTESIAN_POINT('Ctrl Pts',(-46.089925771934,44.9280150456296,3.60701400320326));
#15669=CARTESIAN_POINT('Ctrl Pts',(-46.5530501979845,44.6608255719955,3.60701400320326));
#15670=CARTESIAN_POINT('Ctrl Pts',(-47.0161721905706,44.3936318804496,3.60701400320324));
#15671=CARTESIAN_POINT('Ctrl Pts',(-47.6893519862319,44.0052434879083,3.60701400320324));
#15672=CARTESIAN_POINT('Ctrl Pts',(-48.1309692507095,43.7504492807381,3.60701400320326));
#15673=CARTESIAN_POINT('Ctrl Pts',(-48.5725845633798,43.4956516907297,3.60701400320326));
#15674=CARTESIAN_POINT('Origin',(-4.32455996307467,-7926.57953929723,-4524.0108731871));
#15675=CARTESIAN_POINT('Ctrl Pts',(-48.706329375,58.437500006828,-1.8898197019151E-14));
#15676=CARTESIAN_POINT('Ctrl Pts',(-48.706329375,58.2291666734946,-13.0508216223155));
#15677=CARTESIAN_POINT('Ctrl Pts',(-42.1809185638422,58.0208333401613,-24.3531646875));
#15678=CARTESIAN_POINT('Ctrl Pts',(-35.6555077526845,57.812500006828,-35.6555077526845));
#15679=CARTESIAN_POINT('Ctrl Pts',(-24.3531646875,57.6041666734946,-42.1809185638422));
#15680=CARTESIAN_POINT('Ctrl Pts',(-13.0508216223155,57.3958333401613,-48.706329375));
#15681=CARTESIAN_POINT('Ctrl Pts',(1.59157945007855E-14,57.187500006828,
-48.706329375));
#15682=CARTESIAN_POINT('Ctrl Pts',(13.0508216223155,56.9791666734946,-48.706329375));
#15683=CARTESIAN_POINT('Ctrl Pts',(24.3531646875,56.7708333401613,-42.1809185638422));
#15684=CARTESIAN_POINT('Ctrl Pts',(35.6555077526845,56.562500006828,-35.6555077526845));
#15685=CARTESIAN_POINT('Ctrl Pts',(42.1809185638422,56.3541666734946,-24.3531646875));
#15686=CARTESIAN_POINT('Ctrl Pts',(48.706329375,56.1458333401613,-13.0508216223155));
#15687=CARTESIAN_POINT('Ctrl Pts',(48.706329375,55.937500006828,1.293339198242E-14));
#15688=CARTESIAN_POINT('Ctrl Pts',(48.706329375,55.7291666734946,13.0508216223155));
#15689=CARTESIAN_POINT('Ctrl Pts',(42.1809185638422,55.5208333401613,24.3531646875));
#15690=CARTESIAN_POINT('Ctrl Pts',(35.6555077526845,55.312500006828,35.6555077526845));
#15691=CARTESIAN_POINT('Ctrl Pts',(24.3531646875,55.1041666734946,42.1809185638422));
#15692=CARTESIAN_POINT('Ctrl Pts',(13.0508216223155,54.8958333401613,48.706329375));
#15693=CARTESIAN_POINT('Ctrl Pts',(-9.95098946405443E-15,54.687500006828,
48.706329375));
#15694=CARTESIAN_POINT('Ctrl Pts',(-13.0508216223155,54.4791666734946,48.706329375));
#15695=CARTESIAN_POINT('Ctrl Pts',(-24.3531646875,54.2708333401613,42.1809185638423));
#15696=CARTESIAN_POINT('Ctrl Pts',(-35.6555077526845,54.062500006828,35.6555077526845));
#15697=CARTESIAN_POINT('Ctrl Pts',(-42.1809185638422,53.8541666734946,24.3531646875));
#15698=CARTESIAN_POINT('Ctrl Pts',(-48.706329375,53.6458333401613,13.0508216223155));
#15699=CARTESIAN_POINT('Ctrl Pts',(-48.706329375,53.437500006828,-1.8898197019151E-14));
#15700=CARTESIAN_POINT('Ctrl Pts',(-48.706329375,53.2291666734946,-13.0508216223155));
#15701=CARTESIAN_POINT('Ctrl Pts',(-42.1809185638422,53.0208333401613,-24.3531646875));
#15702=CARTESIAN_POINT('Ctrl Pts',(-35.6555077526845,52.812500006828,-35.6555077526845));
#15703=CARTESIAN_POINT('Ctrl Pts',(-24.3531646875,52.6041666734946,-42.1809185638422));
#15704=CARTESIAN_POINT('Ctrl Pts',(-13.0508216223155,52.3958333401613,-48.706329375));
#15705=CARTESIAN_POINT('Ctrl Pts',(1.59157945007855E-14,52.187500006828,
-48.706329375));
#15706=CARTESIAN_POINT('Ctrl Pts',(13.0508216223155,51.9791666734946,-48.706329375));
#15707=CARTESIAN_POINT('Ctrl Pts',(24.3531646875,51.7708333401613,-42.1809185638422));
#15708=CARTESIAN_POINT('Ctrl Pts',(35.6555077526845,51.562500006828,-35.6555077526845));
#15709=CARTESIAN_POINT('Ctrl Pts',(42.1809185638422,51.3541666734946,-24.3531646875));
#15710=CARTESIAN_POINT('Ctrl Pts',(48.706329375,51.1458333401613,-13.0508216223155));
#15711=CARTESIAN_POINT('Ctrl Pts',(48.706329375,50.937500006828,1.293339198242E-14));
#15712=CARTESIAN_POINT('Ctrl Pts',(48.706329375,50.7291666734946,13.0508216223155));
#15713=CARTESIAN_POINT('Ctrl Pts',(42.1809185638422,50.5208333401613,24.3531646875));
#15714=CARTESIAN_POINT('Ctrl Pts',(35.6555077526845,50.312500006828,35.6555077526845));
#15715=CARTESIAN_POINT('Ctrl Pts',(24.3531646875,50.1041666734946,42.1809185638422));
#15716=CARTESIAN_POINT('Ctrl Pts',(13.0508216223155,49.8958333401613,48.706329375));
#15717=CARTESIAN_POINT('Ctrl Pts',(-9.95098946405443E-15,49.687500006828,
48.706329375));
#15718=CARTESIAN_POINT('Ctrl Pts',(-13.0508216223155,49.4791666734946,48.706329375));
#15719=CARTESIAN_POINT('Ctrl Pts',(-24.3531646875,49.2708333401613,42.1809185638423));
#15720=CARTESIAN_POINT('Ctrl Pts',(-35.6555077526845,49.062500006828,35.6555077526845));
#15721=CARTESIAN_POINT('Ctrl Pts',(-42.1809185638422,48.8541666734946,24.3531646875));
#15722=CARTESIAN_POINT('Ctrl Pts',(-48.706329375,48.6458333401613,13.0508216223155));
#15723=CARTESIAN_POINT('Ctrl Pts',(-48.706329375,48.437500006828,-1.8898197019151E-14));
#15724=CARTESIAN_POINT('Ctrl Pts',(-48.706329375,48.2291666734946,-13.0508216223155));
#15725=CARTESIAN_POINT('Ctrl Pts',(-42.1809185638422,48.0208333401613,-24.3531646875));
#15726=CARTESIAN_POINT('Ctrl Pts',(-35.6555077526845,47.812500006828,-35.6555077526845));
#15727=CARTESIAN_POINT('Ctrl Pts',(-24.3531646875,47.6041666734946,-42.1809185638422));
#15728=CARTESIAN_POINT('Ctrl Pts',(-13.0508216223155,47.3958333401613,-48.706329375));
#15729=CARTESIAN_POINT('Ctrl Pts',(1.59157945007855E-14,47.187500006828,
-48.706329375));
#15730=CARTESIAN_POINT('Ctrl Pts',(13.0508216223155,46.9791666734946,-48.706329375));
#15731=CARTESIAN_POINT('Ctrl Pts',(24.3531646875,46.7708333401613,-42.1809185638422));
#15732=CARTESIAN_POINT('Ctrl Pts',(35.6555077526845,46.562500006828,-35.6555077526845));
#15733=CARTESIAN_POINT('Ctrl Pts',(42.1809185638422,46.3541666734946,-24.3531646875));
#15734=CARTESIAN_POINT('Ctrl Pts',(48.706329375,46.1458333401613,-13.0508216223155));
#15735=CARTESIAN_POINT('Ctrl Pts',(48.706329375,45.937500006828,1.293339198242E-14));
#15736=CARTESIAN_POINT('Ctrl Pts',(48.706329375,45.7291666734946,13.0508216223155));
#15737=CARTESIAN_POINT('Ctrl Pts',(42.1809185638422,45.5208333401613,24.3531646875));
#15738=CARTESIAN_POINT('Ctrl Pts',(35.6555077526845,45.312500006828,35.6555077526845));
#15739=CARTESIAN_POINT('Ctrl Pts',(24.3531646875,45.1041666734946,42.1809185638422));
#15740=CARTESIAN_POINT('Ctrl Pts',(13.0508216223155,44.8958333401613,48.706329375));
#15741=CARTESIAN_POINT('Ctrl Pts',(-9.95098946405443E-15,44.687500006828,
48.706329375));
#15742=CARTESIAN_POINT('Ctrl Pts',(-13.0508216223155,44.4791666734946,48.706329375));
#15743=CARTESIAN_POINT('Ctrl Pts',(-24.3531646875,44.2708333401613,42.1809185638423));
#15744=CARTESIAN_POINT('Ctrl Pts',(-35.6555077526845,44.062500006828,35.6555077526845));
#15745=CARTESIAN_POINT('Ctrl Pts',(-42.1809185638422,43.8541666734946,24.3531646875));
#15746=CARTESIAN_POINT('Ctrl Pts',(-48.706329375,43.6458333401613,13.0508216223155));
#15747=CARTESIAN_POINT('Ctrl Pts',(-48.706329375,43.437500006828,-1.8898197019151E-14));
#15748=CARTESIAN_POINT('Ctrl Pts',(-48.706329375,43.2291666734946,-13.0508216223155));
#15749=CARTESIAN_POINT('Ctrl Pts',(-42.1809185638422,43.0208333401613,-24.3531646875));
#15750=CARTESIAN_POINT('Ctrl Pts',(-35.6555077526845,42.812500006828,-35.6555077526845));
#15751=CARTESIAN_POINT('Ctrl Pts',(-24.3531646875,42.6041666734946,-42.1809185638422));
#15752=CARTESIAN_POINT('Ctrl Pts',(-13.0508216223155,42.3958333401613,-48.706329375));
#15753=CARTESIAN_POINT('Ctrl Pts',(1.59157945007855E-14,42.187500006828,
-48.706329375));
#15754=CARTESIAN_POINT('Ctrl Pts',(13.0508216223155,41.9791666734946,-48.706329375));
#15755=CARTESIAN_POINT('Ctrl Pts',(24.3531646875,41.7708333401613,-42.1809185638422));
#15756=CARTESIAN_POINT('Ctrl Pts',(35.6555077526845,41.562500006828,-35.6555077526845));
#15757=CARTESIAN_POINT('Ctrl Pts',(42.1809185638422,41.3541666734946,-24.3531646875));
#15758=CARTESIAN_POINT('Ctrl Pts',(48.706329375,41.1458333401613,-13.0508216223155));
#15759=CARTESIAN_POINT('Ctrl Pts',(48.706329375,40.937500006828,1.293339198242E-14));
#15760=CARTESIAN_POINT('Ctrl Pts',(48.706329375,40.7291666734946,13.0508216223155));
#15761=CARTESIAN_POINT('Ctrl Pts',(42.1809185638422,40.5208333401613,24.3531646875));
#15762=CARTESIAN_POINT('Ctrl Pts',(35.6555077526845,40.312500006828,35.6555077526845));
#15763=CARTESIAN_POINT('Ctrl Pts',(24.3531646875,40.1041666734946,42.1809185638422));
#15764=CARTESIAN_POINT('Ctrl Pts',(13.0508216223155,39.8958333401613,48.706329375));
#15765=CARTESIAN_POINT('Ctrl Pts',(-9.95098946405443E-15,39.687500006828,
48.706329375));
#15766=CARTESIAN_POINT('Ctrl Pts',(-13.0508216223155,39.4791666734946,48.706329375));
#15767=CARTESIAN_POINT('Ctrl Pts',(-24.3531646875,39.2708333401613,42.1809185638423));
#15768=CARTESIAN_POINT('Ctrl Pts',(-35.6555077526845,39.062500006828,35.6555077526845));
#15769=CARTESIAN_POINT('Ctrl Pts',(-42.1809185638422,38.8541666734946,24.3531646875));
#15770=CARTESIAN_POINT('Ctrl Pts',(-48.706329375,38.6458333401613,13.0508216223155));
#15771=CARTESIAN_POINT('Ctrl Pts',(-48.706329375,38.437500006828,-1.8898197019151E-14));
#15772=CARTESIAN_POINT('Ctrl Pts',(-48.706329375,38.2291666734946,-13.0508216223155));
#15773=CARTESIAN_POINT('Ctrl Pts',(-42.1809185638422,38.0208333401613,-24.3531646875));
#15774=CARTESIAN_POINT('Ctrl Pts',(-35.6555077526845,37.812500006828,-35.6555077526845));
#15775=CARTESIAN_POINT('Ctrl Pts',(-24.3531646875,37.6041666734946,-42.1809185638422));
#15776=CARTESIAN_POINT('Ctrl Pts',(-13.0508216223155,37.3958333401613,-48.706329375));
#15777=CARTESIAN_POINT('Ctrl Pts',(1.59157945007855E-14,37.187500006828,
-48.706329375));
#15778=CARTESIAN_POINT('Ctrl Pts',(13.0508216223155,36.9791666734946,-48.706329375));
#15779=CARTESIAN_POINT('Ctrl Pts',(24.3531646875,36.7708333401613,-42.1809185638422));
#15780=CARTESIAN_POINT('Ctrl Pts',(35.6555077526845,36.562500006828,-35.6555077526845));
#15781=CARTESIAN_POINT('Ctrl Pts',(42.1809185638422,36.3541666734946,-24.3531646875));
#15782=CARTESIAN_POINT('Ctrl Pts',(48.706329375,36.1458333401613,-13.0508216223155));
#15783=CARTESIAN_POINT('Ctrl Pts',(48.706329375,35.937500006828,1.293339198242E-14));
#15784=CARTESIAN_POINT('Ctrl Pts',(48.706329375,35.7291666734946,13.0508216223155));
#15785=CARTESIAN_POINT('Ctrl Pts',(42.1809185638422,35.5208333401613,24.3531646875));
#15786=CARTESIAN_POINT('Ctrl Pts',(35.6555077526845,35.312500006828,35.6555077526845));
#15787=CARTESIAN_POINT('Ctrl Pts',(24.3531646875,35.1041666734946,42.1809185638422));
#15788=CARTESIAN_POINT('Ctrl Pts',(13.0508216223155,34.8958333401613,48.706329375));
#15789=CARTESIAN_POINT('Ctrl Pts',(-9.95098946405443E-15,34.687500006828,
48.706329375));
#15790=CARTESIAN_POINT('Ctrl Pts',(-13.0508216223155,34.4791666734946,48.706329375));
#15791=CARTESIAN_POINT('Ctrl Pts',(-24.3531646875,34.2708333401613,42.1809185638423));
#15792=CARTESIAN_POINT('Ctrl Pts',(-35.6555077526845,34.062500006828,35.6555077526845));
#15793=CARTESIAN_POINT('Ctrl Pts',(-42.1809185638422,33.8541666734946,24.3531646875));
#15794=CARTESIAN_POINT('Ctrl Pts',(-48.706329375,33.6458333401613,13.0508216223155));
#15795=CARTESIAN_POINT('Ctrl Pts',(-48.706329375,33.437500006828,-1.8898197019151E-14));
#15796=CARTESIAN_POINT('Ctrl Pts',(-48.706329375,33.2291666734946,-13.0508216223155));
#15797=CARTESIAN_POINT('Ctrl Pts',(-42.1809185638422,33.0208333401613,-24.3531646875));
#15798=CARTESIAN_POINT('Ctrl Pts',(-35.6555077526845,32.812500006828,-35.6555077526845));
#15799=CARTESIAN_POINT('Ctrl Pts',(-24.3531646875,32.6041666734946,-42.1809185638422));
#15800=CARTESIAN_POINT('Ctrl Pts',(-13.0508216223155,32.3958333401613,-48.706329375));
#15801=CARTESIAN_POINT('Ctrl Pts',(1.59157945007855E-14,32.187500006828,
-48.706329375));
#15802=CARTESIAN_POINT('Ctrl Pts',(13.0508216223155,31.9791666734946,-48.706329375));
#15803=CARTESIAN_POINT('Ctrl Pts',(24.3531646875,31.7708333401613,-42.1809185638422));
#15804=CARTESIAN_POINT('Ctrl Pts',(35.6555077526845,31.562500006828,-35.6555077526845));
#15805=CARTESIAN_POINT('Ctrl Pts',(42.1809185638422,31.3541666734946,-24.3531646875));
#15806=CARTESIAN_POINT('Ctrl Pts',(48.706329375,31.1458333401613,-13.0508216223155));
#15807=CARTESIAN_POINT('Ctrl Pts',(48.706329375,30.937500006828,1.293339198242E-14));
#15808=CARTESIAN_POINT('Ctrl Pts',(48.706329375,30.7291666734946,13.0508216223155));
#15809=CARTESIAN_POINT('Ctrl Pts',(42.1809185638422,30.5208333401613,24.3531646875));
#15810=CARTESIAN_POINT('Ctrl Pts',(35.6555077526845,30.312500006828,35.6555077526845));
#15811=CARTESIAN_POINT('Ctrl Pts',(24.3531646875,30.1041666734946,42.1809185638422));
#15812=CARTESIAN_POINT('Ctrl Pts',(13.0508216223155,29.8958333401613,48.706329375));
#15813=CARTESIAN_POINT('Ctrl Pts',(-9.95098946405443E-15,29.687500006828,
48.706329375));
#15814=CARTESIAN_POINT('Ctrl Pts',(-13.0508216223155,29.4791666734946,48.706329375));
#15815=CARTESIAN_POINT('Ctrl Pts',(-24.3531646875,29.2708333401613,42.1809185638423));
#15816=CARTESIAN_POINT('Ctrl Pts',(-35.6555077526845,29.062500006828,35.6555077526845));
#15817=CARTESIAN_POINT('Ctrl Pts',(-42.1809185638422,28.8541666734946,24.3531646875));
#15818=CARTESIAN_POINT('Ctrl Pts',(-48.706329375,28.6458333401613,13.0508216223155));
#15819=CARTESIAN_POINT('Ctrl Pts',(-48.706329375,28.437500006828,-1.8898197019151E-14));
#15820=CARTESIAN_POINT('Ctrl Pts',(-46.,60.,0.));
#15821=CARTESIAN_POINT('Ctrl Pts',(-46.,59.7916666666667,-12.3256628518316));
#15822=CARTESIAN_POINT('Ctrl Pts',(-39.8371685740842,59.5833333333333,-23.));
#15823=CARTESIAN_POINT('Ctrl Pts',(-33.6743371481684,59.375,-33.6743371481684));
#15824=CARTESIAN_POINT('Ctrl Pts',(-23.,59.1666666666667,-39.8371685740842));
#15825=CARTESIAN_POINT('Ctrl Pts',(-12.3256628518317,58.9583333333333,-46.));
#15826=CARTESIAN_POINT('Ctrl Pts',(-2.81668763803891E-15,58.75,-46.));
#15827=CARTESIAN_POINT('Ctrl Pts',(12.3256628518316,58.5416666666667,-46.));
#15828=CARTESIAN_POINT('Ctrl Pts',(23.,58.3333333333333,-39.8371685740842));
#15829=CARTESIAN_POINT('Ctrl Pts',(33.6743371481683,58.125,-33.6743371481684));
#15830=CARTESIAN_POINT('Ctrl Pts',(39.8371685740842,57.9166666666667,-23.));
#15831=CARTESIAN_POINT('Ctrl Pts',(46.,57.7083333333333,-12.3256628518317));
#15832=CARTESIAN_POINT('Ctrl Pts',(46.,57.5,-5.63337527607782E-15));
#15833=CARTESIAN_POINT('Ctrl Pts',(46.,57.2916666666667,12.3256628518316));
#15834=CARTESIAN_POINT('Ctrl Pts',(39.8371685740842,57.0833333333333,23.));
#15835=CARTESIAN_POINT('Ctrl Pts',(33.6743371481684,56.875,33.6743371481683));
#15836=CARTESIAN_POINT('Ctrl Pts',(23.,56.6666666666667,39.8371685740842));
#15837=CARTESIAN_POINT('Ctrl Pts',(12.3256628518317,56.4583333333333,46.));
#15838=CARTESIAN_POINT('Ctrl Pts',(8.45006291411674E-15,56.25,46.));
#15839=CARTESIAN_POINT('Ctrl Pts',(-12.3256628518316,56.0416666666667,46.));
#15840=CARTESIAN_POINT('Ctrl Pts',(-23.,55.8333333333333,39.8371685740842));
#15841=CARTESIAN_POINT('Ctrl Pts',(-33.6743371481683,55.625,33.6743371481684));
#15842=CARTESIAN_POINT('Ctrl Pts',(-39.8371685740842,55.4166666666667,23.));
#15843=CARTESIAN_POINT('Ctrl Pts',(-46.,55.2083333333333,12.3256628518317));
#15844=CARTESIAN_POINT('Ctrl Pts',(-46.,55.,0.));
#15845=CARTESIAN_POINT('Ctrl Pts',(-46.,54.7916666666667,-12.3256628518316));
#15846=CARTESIAN_POINT('Ctrl Pts',(-39.8371685740842,54.5833333333333,-23.));
#15847=CARTESIAN_POINT('Ctrl Pts',(-33.6743371481684,54.375,-33.6743371481684));
#15848=CARTESIAN_POINT('Ctrl Pts',(-23.,54.1666666666667,-39.8371685740842));
#15849=CARTESIAN_POINT('Ctrl Pts',(-12.3256628518317,53.9583333333333,-46.));
#15850=CARTESIAN_POINT('Ctrl Pts',(-2.81668763803891E-15,53.75,-46.));
#15851=CARTESIAN_POINT('Ctrl Pts',(12.3256628518316,53.5416666666667,-46.));
#15852=CARTESIAN_POINT('Ctrl Pts',(23.,53.3333333333333,-39.8371685740842));
#15853=CARTESIAN_POINT('Ctrl Pts',(33.6743371481683,53.125,-33.6743371481684));
#15854=CARTESIAN_POINT('Ctrl Pts',(39.8371685740842,52.9166666666667,-23.));
#15855=CARTESIAN_POINT('Ctrl Pts',(46.,52.7083333333333,-12.3256628518317));
#15856=CARTESIAN_POINT('Ctrl Pts',(46.,52.5,-5.63337527607782E-15));
#15857=CARTESIAN_POINT('Ctrl Pts',(46.,52.2916666666667,12.3256628518316));
#15858=CARTESIAN_POINT('Ctrl Pts',(39.8371685740842,52.0833333333333,23.));
#15859=CARTESIAN_POINT('Ctrl Pts',(33.6743371481684,51.875,33.6743371481683));
#15860=CARTESIAN_POINT('Ctrl Pts',(23.,51.6666666666667,39.8371685740842));
#15861=CARTESIAN_POINT('Ctrl Pts',(12.3256628518317,51.4583333333333,46.));
#15862=CARTESIAN_POINT('Ctrl Pts',(8.45006291411674E-15,51.25,46.));
#15863=CARTESIAN_POINT('Ctrl Pts',(-12.3256628518316,51.0416666666667,46.));
#15864=CARTESIAN_POINT('Ctrl Pts',(-23.,50.8333333333333,39.8371685740842));
#15865=CARTESIAN_POINT('Ctrl Pts',(-33.6743371481683,50.625,33.6743371481684));
#15866=CARTESIAN_POINT('Ctrl Pts',(-39.8371685740842,50.4166666666667,23.));
#15867=CARTESIAN_POINT('Ctrl Pts',(-46.,50.2083333333333,12.3256628518317));
#15868=CARTESIAN_POINT('Ctrl Pts',(-46.,50.,0.));
#15869=CARTESIAN_POINT('Ctrl Pts',(-46.,49.7916666666667,-12.3256628518316));
#15870=CARTESIAN_POINT('Ctrl Pts',(-39.8371685740842,49.5833333333333,-23.));
#15871=CARTESIAN_POINT('Ctrl Pts',(-33.6743371481684,49.375,-33.6743371481684));
#15872=CARTESIAN_POINT('Ctrl Pts',(-23.,49.1666666666667,-39.8371685740842));
#15873=CARTESIAN_POINT('Ctrl Pts',(-12.3256628518317,48.9583333333333,-46.));
#15874=CARTESIAN_POINT('Ctrl Pts',(-2.81668763803891E-15,48.75,-46.));
#15875=CARTESIAN_POINT('Ctrl Pts',(12.3256628518316,48.5416666666667,-46.));
#15876=CARTESIAN_POINT('Ctrl Pts',(23.,48.3333333333333,-39.8371685740842));
#15877=CARTESIAN_POINT('Ctrl Pts',(33.6743371481683,48.125,-33.6743371481684));
#15878=CARTESIAN_POINT('Ctrl Pts',(39.8371685740842,47.9166666666667,-23.));
#15879=CARTESIAN_POINT('Ctrl Pts',(46.,47.7083333333333,-12.3256628518317));
#15880=CARTESIAN_POINT('Ctrl Pts',(46.,47.5,-5.63337527607782E-15));
#15881=CARTESIAN_POINT('Ctrl Pts',(46.,47.2916666666667,12.3256628518316));
#15882=CARTESIAN_POINT('Ctrl Pts',(39.8371685740842,47.0833333333333,23.));
#15883=CARTESIAN_POINT('Ctrl Pts',(33.6743371481684,46.875,33.6743371481683));
#15884=CARTESIAN_POINT('Ctrl Pts',(23.,46.6666666666667,39.8371685740842));
#15885=CARTESIAN_POINT('Ctrl Pts',(12.3256628518317,46.4583333333333,46.));
#15886=CARTESIAN_POINT('Ctrl Pts',(8.45006291411674E-15,46.25,46.));
#15887=CARTESIAN_POINT('Ctrl Pts',(-12.3256628518316,46.0416666666667,46.));
#15888=CARTESIAN_POINT('Ctrl Pts',(-23.,45.8333333333333,39.8371685740842));
#15889=CARTESIAN_POINT('Ctrl Pts',(-33.6743371481683,45.625,33.6743371481684));
#15890=CARTESIAN_POINT('Ctrl Pts',(-39.8371685740842,45.4166666666667,23.));
#15891=CARTESIAN_POINT('Ctrl Pts',(-46.,45.2083333333333,12.3256628518317));
#15892=CARTESIAN_POINT('Ctrl Pts',(-46.,45.,0.));
#15893=CARTESIAN_POINT('Ctrl Pts',(-46.,44.7916666666667,-12.3256628518316));
#15894=CARTESIAN_POINT('Ctrl Pts',(-39.8371685740842,44.5833333333333,-23.));
#15895=CARTESIAN_POINT('Ctrl Pts',(-33.6743371481684,44.375,-33.6743371481684));
#15896=CARTESIAN_POINT('Ctrl Pts',(-23.,44.1666666666667,-39.8371685740842));
#15897=CARTESIAN_POINT('Ctrl Pts',(-12.3256628518317,43.9583333333333,-46.));
#15898=CARTESIAN_POINT('Ctrl Pts',(-2.81668763803891E-15,43.75,-46.));
#15899=CARTESIAN_POINT('Ctrl Pts',(12.3256628518316,43.5416666666667,-46.));
#15900=CARTESIAN_POINT('Ctrl Pts',(23.,43.3333333333333,-39.8371685740842));
#15901=CARTESIAN_POINT('Ctrl Pts',(33.6743371481683,43.125,-33.6743371481684));
#15902=CARTESIAN_POINT('Ctrl Pts',(39.8371685740842,42.9166666666667,-23.));
#15903=CARTESIAN_POINT('Ctrl Pts',(46.,42.7083333333333,-12.3256628518317));
#15904=CARTESIAN_POINT('Ctrl Pts',(46.,42.5,-5.63337527607782E-15));
#15905=CARTESIAN_POINT('Ctrl Pts',(46.,42.2916666666667,12.3256628518316));
#15906=CARTESIAN_POINT('Ctrl Pts',(39.8371685740842,42.0833333333333,23.));
#15907=CARTESIAN_POINT('Ctrl Pts',(33.6743371481684,41.875,33.6743371481683));
#15908=CARTESIAN_POINT('Ctrl Pts',(23.,41.6666666666667,39.8371685740842));
#15909=CARTESIAN_POINT('Ctrl Pts',(12.3256628518317,41.4583333333333,46.));
#15910=CARTESIAN_POINT('Ctrl Pts',(8.45006291411674E-15,41.25,46.));
#15911=CARTESIAN_POINT('Ctrl Pts',(-12.3256628518316,41.0416666666667,46.));
#15912=CARTESIAN_POINT('Ctrl Pts',(-23.,40.8333333333333,39.8371685740842));
#15913=CARTESIAN_POINT('Ctrl Pts',(-33.6743371481683,40.625,33.6743371481684));
#15914=CARTESIAN_POINT('Ctrl Pts',(-39.8371685740842,40.4166666666667,23.));
#15915=CARTESIAN_POINT('Ctrl Pts',(-46.,40.2083333333333,12.3256628518317));
#15916=CARTESIAN_POINT('Ctrl Pts',(-46.,40.,0.));
#15917=CARTESIAN_POINT('Ctrl Pts',(-46.,39.7916666666667,-12.3256628518316));
#15918=CARTESIAN_POINT('Ctrl Pts',(-39.8371685740842,39.5833333333333,-23.));
#15919=CARTESIAN_POINT('Ctrl Pts',(-33.6743371481684,39.375,-33.6743371481684));
#15920=CARTESIAN_POINT('Ctrl Pts',(-23.,39.1666666666667,-39.8371685740842));
#15921=CARTESIAN_POINT('Ctrl Pts',(-12.3256628518317,38.9583333333333,-46.));
#15922=CARTESIAN_POINT('Ctrl Pts',(-2.81668763803891E-15,38.75,-46.));
#15923=CARTESIAN_POINT('Ctrl Pts',(12.3256628518316,38.5416666666667,-46.));
#15924=CARTESIAN_POINT('Ctrl Pts',(23.,38.3333333333333,-39.8371685740842));
#15925=CARTESIAN_POINT('Ctrl Pts',(33.6743371481683,38.125,-33.6743371481684));
#15926=CARTESIAN_POINT('Ctrl Pts',(39.8371685740842,37.9166666666667,-23.));
#15927=CARTESIAN_POINT('Ctrl Pts',(46.,37.7083333333333,-12.3256628518317));
#15928=CARTESIAN_POINT('Ctrl Pts',(46.,37.5,-5.63337527607782E-15));
#15929=CARTESIAN_POINT('Ctrl Pts',(46.,37.2916666666667,12.3256628518316));
#15930=CARTESIAN_POINT('Ctrl Pts',(39.8371685740842,37.0833333333333,23.));
#15931=CARTESIAN_POINT('Ctrl Pts',(33.6743371481684,36.875,33.6743371481683));
#15932=CARTESIAN_POINT('Ctrl Pts',(23.,36.6666666666667,39.8371685740842));
#15933=CARTESIAN_POINT('Ctrl Pts',(12.3256628518317,36.4583333333333,46.));
#15934=CARTESIAN_POINT('Ctrl Pts',(8.45006291411674E-15,36.25,46.));
#15935=CARTESIAN_POINT('Ctrl Pts',(-12.3256628518316,36.0416666666667,46.));
#15936=CARTESIAN_POINT('Ctrl Pts',(-23.,35.8333333333333,39.8371685740842));
#15937=CARTESIAN_POINT('Ctrl Pts',(-33.6743371481683,35.625,33.6743371481684));
#15938=CARTESIAN_POINT('Ctrl Pts',(-39.8371685740842,35.4166666666667,23.));
#15939=CARTESIAN_POINT('Ctrl Pts',(-46.,35.2083333333333,12.3256628518317));
#15940=CARTESIAN_POINT('Ctrl Pts',(-46.,35.,0.));
#15941=CARTESIAN_POINT('Ctrl Pts',(-46.,34.7916666666667,-12.3256628518316));
#15942=CARTESIAN_POINT('Ctrl Pts',(-39.8371685740842,34.5833333333333,-23.));
#15943=CARTESIAN_POINT('Ctrl Pts',(-33.6743371481684,34.375,-33.6743371481684));
#15944=CARTESIAN_POINT('Ctrl Pts',(-23.,34.1666666666667,-39.8371685740842));
#15945=CARTESIAN_POINT('Ctrl Pts',(-12.3256628518317,33.9583333333333,-46.));
#15946=CARTESIAN_POINT('Ctrl Pts',(-2.81668763803891E-15,33.75,-46.));
#15947=CARTESIAN_POINT('Ctrl Pts',(12.3256628518316,33.5416666666667,-46.));
#15948=CARTESIAN_POINT('Ctrl Pts',(23.,33.3333333333333,-39.8371685740842));
#15949=CARTESIAN_POINT('Ctrl Pts',(33.6743371481683,33.125,-33.6743371481684));
#15950=CARTESIAN_POINT('Ctrl Pts',(39.8371685740842,32.9166666666667,-23.));
#15951=CARTESIAN_POINT('Ctrl Pts',(46.,32.7083333333333,-12.3256628518317));
#15952=CARTESIAN_POINT('Ctrl Pts',(46.,32.5,-5.63337527607782E-15));
#15953=CARTESIAN_POINT('Ctrl Pts',(46.,32.2916666666667,12.3256628518316));
#15954=CARTESIAN_POINT('Ctrl Pts',(39.8371685740842,32.0833333333333,23.));
#15955=CARTESIAN_POINT('Ctrl Pts',(33.6743371481684,31.875,33.6743371481683));
#15956=CARTESIAN_POINT('Ctrl Pts',(23.,31.6666666666667,39.8371685740842));
#15957=CARTESIAN_POINT('Ctrl Pts',(12.3256628518317,31.4583333333333,46.));
#15958=CARTESIAN_POINT('Ctrl Pts',(8.45006291411674E-15,31.25,46.));
#15959=CARTESIAN_POINT('Ctrl Pts',(-12.3256628518316,31.0416666666667,46.));
#15960=CARTESIAN_POINT('Ctrl Pts',(-23.,30.8333333333333,39.8371685740842));
#15961=CARTESIAN_POINT('Ctrl Pts',(-33.6743371481683,30.625,33.6743371481684));
#15962=CARTESIAN_POINT('Ctrl Pts',(-39.8371685740842,30.4166666666667,23.));
#15963=CARTESIAN_POINT('Ctrl Pts',(-46.,30.2083333333333,12.3256628518317));
#15964=CARTESIAN_POINT('Ctrl Pts',(-46.,30.,0.));
#15965=CARTESIAN_POINT('Origin',(4513.80899817375,-7915.1585511582,-4.33049284435178));
#15966=CARTESIAN_POINT('Ctrl Pts',(-4.32456003949879,38.8240181593937,-45.7962681936506));
#15967=CARTESIAN_POINT('Ctrl Pts',(-4.32456003949872,38.6905125468623,-46.0278818021281));
#15968=CARTESIAN_POINT('Ctrl Pts',(-4.32456003949878,38.4234964717135,-46.4911062234486));
#15969=CARTESIAN_POINT('Ctrl Pts',(-4.32456003949881,38.1564711191154,-46.954325296818));
#15970=CARTESIAN_POINT('Ctrl Pts',(-4.32456003949881,37.7677643029224,-47.6286149142205));
#15971=CARTESIAN_POINT('Ctrl Pts',(-4.32456003949869,37.5125642776457,-48.0712916022845));
#15972=CARTESIAN_POINT('Ctrl Pts',(-4.32456003949869,37.2573567866782,-48.5139639861634));
#15973=CARTESIAN_POINT('Ctrl Pts',(-48.706329375,58.437500006828,-1.8898197019151E-14));
#15974=CARTESIAN_POINT('Ctrl Pts',(-48.706329375,58.2291666734946,-13.0508216223155));
#15975=CARTESIAN_POINT('Ctrl Pts',(-42.1809185638422,58.0208333401613,-24.3531646875));
#15976=CARTESIAN_POINT('Ctrl Pts',(-35.6555077526845,57.812500006828,-35.6555077526845));
#15977=CARTESIAN_POINT('Ctrl Pts',(-24.3531646875,57.6041666734946,-42.1809185638422));
#15978=CARTESIAN_POINT('Ctrl Pts',(-13.0508216223155,57.3958333401613,-48.706329375));
#15979=CARTESIAN_POINT('Ctrl Pts',(1.59157945007855E-14,57.187500006828,
-48.706329375));
#15980=CARTESIAN_POINT('Ctrl Pts',(13.0508216223155,56.9791666734946,-48.706329375));
#15981=CARTESIAN_POINT('Ctrl Pts',(24.3531646875,56.7708333401613,-42.1809185638422));
#15982=CARTESIAN_POINT('Ctrl Pts',(35.6555077526845,56.562500006828,-35.6555077526845));
#15983=CARTESIAN_POINT('Ctrl Pts',(42.1809185638422,56.3541666734946,-24.3531646875));
#15984=CARTESIAN_POINT('Ctrl Pts',(48.706329375,56.1458333401613,-13.0508216223155));
#15985=CARTESIAN_POINT('Ctrl Pts',(48.706329375,55.937500006828,1.293339198242E-14));
#15986=CARTESIAN_POINT('Ctrl Pts',(48.706329375,55.7291666734946,13.0508216223155));
#15987=CARTESIAN_POINT('Ctrl Pts',(42.1809185638422,55.5208333401613,24.3531646875));
#15988=CARTESIAN_POINT('Ctrl Pts',(35.6555077526845,55.312500006828,35.6555077526845));
#15989=CARTESIAN_POINT('Ctrl Pts',(24.3531646875,55.1041666734946,42.1809185638422));
#15990=CARTESIAN_POINT('Ctrl Pts',(13.0508216223155,54.8958333401613,48.706329375));
#15991=CARTESIAN_POINT('Ctrl Pts',(-9.95098946405443E-15,54.687500006828,
48.706329375));
#15992=CARTESIAN_POINT('Ctrl Pts',(-13.0508216223155,54.4791666734946,48.706329375));
#15993=CARTESIAN_POINT('Ctrl Pts',(-24.3531646875,54.2708333401613,42.1809185638423));
#15994=CARTESIAN_POINT('Ctrl Pts',(-35.6555077526845,54.062500006828,35.6555077526845));
#15995=CARTESIAN_POINT('Ctrl Pts',(-42.1809185638422,53.8541666734946,24.3531646875));
#15996=CARTESIAN_POINT('Ctrl Pts',(-48.706329375,53.6458333401613,13.0508216223155));
#15997=CARTESIAN_POINT('Ctrl Pts',(-48.706329375,53.437500006828,-1.8898197019151E-14));
#15998=CARTESIAN_POINT('Ctrl Pts',(-48.706329375,53.2291666734946,-13.0508216223155));
#15999=CARTESIAN_POINT('Ctrl Pts',(-42.1809185638422,53.0208333401613,-24.3531646875));
#16000=CARTESIAN_POINT('Ctrl Pts',(-35.6555077526845,52.812500006828,-35.6555077526845));
#16001=CARTESIAN_POINT('Ctrl Pts',(-24.3531646875,52.6041666734946,-42.1809185638422));
#16002=CARTESIAN_POINT('Ctrl Pts',(-13.0508216223155,52.3958333401613,-48.706329375));
#16003=CARTESIAN_POINT('Ctrl Pts',(1.59157945007855E-14,52.187500006828,
-48.706329375));
#16004=CARTESIAN_POINT('Ctrl Pts',(13.0508216223155,51.9791666734946,-48.706329375));
#16005=CARTESIAN_POINT('Ctrl Pts',(24.3531646875,51.7708333401613,-42.1809185638422));
#16006=CARTESIAN_POINT('Ctrl Pts',(35.6555077526845,51.562500006828,-35.6555077526845));
#16007=CARTESIAN_POINT('Ctrl Pts',(42.1809185638422,51.3541666734946,-24.3531646875));
#16008=CARTESIAN_POINT('Ctrl Pts',(48.706329375,51.1458333401613,-13.0508216223155));
#16009=CARTESIAN_POINT('Ctrl Pts',(48.706329375,50.937500006828,1.293339198242E-14));
#16010=CARTESIAN_POINT('Ctrl Pts',(48.706329375,50.7291666734946,13.0508216223155));
#16011=CARTESIAN_POINT('Ctrl Pts',(42.1809185638422,50.5208333401613,24.3531646875));
#16012=CARTESIAN_POINT('Ctrl Pts',(35.6555077526845,50.312500006828,35.6555077526845));
#16013=CARTESIAN_POINT('Ctrl Pts',(24.3531646875,50.1041666734946,42.1809185638422));
#16014=CARTESIAN_POINT('Ctrl Pts',(13.0508216223155,49.8958333401613,48.706329375));
#16015=CARTESIAN_POINT('Ctrl Pts',(-9.95098946405443E-15,49.687500006828,
48.706329375));
#16016=CARTESIAN_POINT('Ctrl Pts',(-13.0508216223155,49.4791666734946,48.706329375));
#16017=CARTESIAN_POINT('Ctrl Pts',(-24.3531646875,49.2708333401613,42.1809185638423));
#16018=CARTESIAN_POINT('Ctrl Pts',(-35.6555077526845,49.062500006828,35.6555077526845));
#16019=CARTESIAN_POINT('Ctrl Pts',(-42.1809185638422,48.8541666734946,24.3531646875));
#16020=CARTESIAN_POINT('Ctrl Pts',(-48.706329375,48.6458333401613,13.0508216223155));
#16021=CARTESIAN_POINT('Ctrl Pts',(-48.706329375,48.437500006828,-1.8898197019151E-14));
#16022=CARTESIAN_POINT('Ctrl Pts',(-48.706329375,48.2291666734946,-13.0508216223155));
#16023=CARTESIAN_POINT('Ctrl Pts',(-42.1809185638422,48.0208333401613,-24.3531646875));
#16024=CARTESIAN_POINT('Ctrl Pts',(-35.6555077526845,47.812500006828,-35.6555077526845));
#16025=CARTESIAN_POINT('Ctrl Pts',(-24.3531646875,47.6041666734946,-42.1809185638422));
#16026=CARTESIAN_POINT('Ctrl Pts',(-13.0508216223155,47.3958333401613,-48.706329375));
#16027=CARTESIAN_POINT('Ctrl Pts',(1.59157945007855E-14,47.187500006828,
-48.706329375));
#16028=CARTESIAN_POINT('Ctrl Pts',(13.0508216223155,46.9791666734946,-48.706329375));
#16029=CARTESIAN_POINT('Ctrl Pts',(24.3531646875,46.7708333401613,-42.1809185638422));
#16030=CARTESIAN_POINT('Ctrl Pts',(35.6555077526845,46.562500006828,-35.6555077526845));
#16031=CARTESIAN_POINT('Ctrl Pts',(42.1809185638422,46.3541666734946,-24.3531646875));
#16032=CARTESIAN_POINT('Ctrl Pts',(48.706329375,46.1458333401613,-13.0508216223155));
#16033=CARTESIAN_POINT('Ctrl Pts',(48.706329375,45.937500006828,1.293339198242E-14));
#16034=CARTESIAN_POINT('Ctrl Pts',(48.706329375,45.7291666734946,13.0508216223155));
#16035=CARTESIAN_POINT('Ctrl Pts',(42.1809185638422,45.5208333401613,24.3531646875));
#16036=CARTESIAN_POINT('Ctrl Pts',(35.6555077526845,45.312500006828,35.6555077526845));
#16037=CARTESIAN_POINT('Ctrl Pts',(24.3531646875,45.1041666734946,42.1809185638422));
#16038=CARTESIAN_POINT('Ctrl Pts',(13.0508216223155,44.8958333401613,48.706329375));
#16039=CARTESIAN_POINT('Ctrl Pts',(-9.95098946405443E-15,44.687500006828,
48.706329375));
#16040=CARTESIAN_POINT('Ctrl Pts',(-13.0508216223155,44.4791666734946,48.706329375));
#16041=CARTESIAN_POINT('Ctrl Pts',(-24.3531646875,44.2708333401613,42.1809185638423));
#16042=CARTESIAN_POINT('Ctrl Pts',(-35.6555077526845,44.062500006828,35.6555077526845));
#16043=CARTESIAN_POINT('Ctrl Pts',(-42.1809185638422,43.8541666734946,24.3531646875));
#16044=CARTESIAN_POINT('Ctrl Pts',(-48.706329375,43.6458333401613,13.0508216223155));
#16045=CARTESIAN_POINT('Ctrl Pts',(-48.706329375,43.437500006828,-1.8898197019151E-14));
#16046=CARTESIAN_POINT('Ctrl Pts',(-48.706329375,43.2291666734946,-13.0508216223155));
#16047=CARTESIAN_POINT('Ctrl Pts',(-42.1809185638422,43.0208333401613,-24.3531646875));
#16048=CARTESIAN_POINT('Ctrl Pts',(-35.6555077526845,42.812500006828,-35.6555077526845));
#16049=CARTESIAN_POINT('Ctrl Pts',(-24.3531646875,42.6041666734946,-42.1809185638422));
#16050=CARTESIAN_POINT('Ctrl Pts',(-13.0508216223155,42.3958333401613,-48.706329375));
#16051=CARTESIAN_POINT('Ctrl Pts',(1.59157945007855E-14,42.187500006828,
-48.706329375));
#16052=CARTESIAN_POINT('Ctrl Pts',(13.0508216223155,41.9791666734946,-48.706329375));
#16053=CARTESIAN_POINT('Ctrl Pts',(24.3531646875,41.7708333401613,-42.1809185638422));
#16054=CARTESIAN_POINT('Ctrl Pts',(35.6555077526845,41.562500006828,-35.6555077526845));
#16055=CARTESIAN_POINT('Ctrl Pts',(42.1809185638422,41.3541666734946,-24.3531646875));
#16056=CARTESIAN_POINT('Ctrl Pts',(48.706329375,41.1458333401613,-13.0508216223155));
#16057=CARTESIAN_POINT('Ctrl Pts',(48.706329375,40.937500006828,1.293339198242E-14));
#16058=CARTESIAN_POINT('Ctrl Pts',(48.706329375,40.7291666734946,13.0508216223155));
#16059=CARTESIAN_POINT('Ctrl Pts',(42.1809185638422,40.5208333401613,24.3531646875));
#16060=CARTESIAN_POINT('Ctrl Pts',(35.6555077526845,40.312500006828,35.6555077526845));
#16061=CARTESIAN_POINT('Ctrl Pts',(24.3531646875,40.1041666734946,42.1809185638422));
#16062=CARTESIAN_POINT('Ctrl Pts',(13.0508216223155,39.8958333401613,48.706329375));
#16063=CARTESIAN_POINT('Ctrl Pts',(-9.95098946405443E-15,39.687500006828,
48.706329375));
#16064=CARTESIAN_POINT('Ctrl Pts',(-13.0508216223155,39.4791666734946,48.706329375));
#16065=CARTESIAN_POINT('Ctrl Pts',(-24.3531646875,39.2708333401613,42.1809185638423));
#16066=CARTESIAN_POINT('Ctrl Pts',(-35.6555077526845,39.062500006828,35.6555077526845));
#16067=CARTESIAN_POINT('Ctrl Pts',(-42.1809185638422,38.8541666734946,24.3531646875));
#16068=CARTESIAN_POINT('Ctrl Pts',(-48.706329375,38.6458333401613,13.0508216223155));
#16069=CARTESIAN_POINT('Ctrl Pts',(-48.706329375,38.437500006828,-1.8898197019151E-14));
#16070=CARTESIAN_POINT('Ctrl Pts',(-48.706329375,38.2291666734946,-13.0508216223155));
#16071=CARTESIAN_POINT('Ctrl Pts',(-42.1809185638422,38.0208333401613,-24.3531646875));
#16072=CARTESIAN_POINT('Ctrl Pts',(-35.6555077526845,37.812500006828,-35.6555077526845));
#16073=CARTESIAN_POINT('Ctrl Pts',(-24.3531646875,37.6041666734946,-42.1809185638422));
#16074=CARTESIAN_POINT('Ctrl Pts',(-13.0508216223155,37.3958333401613,-48.706329375));
#16075=CARTESIAN_POINT('Ctrl Pts',(1.59157945007855E-14,37.187500006828,
-48.706329375));
#16076=CARTESIAN_POINT('Ctrl Pts',(13.0508216223155,36.9791666734946,-48.706329375));
#16077=CARTESIAN_POINT('Ctrl Pts',(24.3531646875,36.7708333401613,-42.1809185638422));
#16078=CARTESIAN_POINT('Ctrl Pts',(35.6555077526845,36.562500006828,-35.6555077526845));
#16079=CARTESIAN_POINT('Ctrl Pts',(42.1809185638422,36.3541666734946,-24.3531646875));
#16080=CARTESIAN_POINT('Ctrl Pts',(48.706329375,36.1458333401613,-13.0508216223155));
#16081=CARTESIAN_POINT('Ctrl Pts',(48.706329375,35.937500006828,1.293339198242E-14));
#16082=CARTESIAN_POINT('Ctrl Pts',(48.706329375,35.7291666734946,13.0508216223155));
#16083=CARTESIAN_POINT('Ctrl Pts',(42.1809185638422,35.5208333401613,24.3531646875));
#16084=CARTESIAN_POINT('Ctrl Pts',(35.6555077526845,35.312500006828,35.6555077526845));
#16085=CARTESIAN_POINT('Ctrl Pts',(24.3531646875,35.1041666734946,42.1809185638422));
#16086=CARTESIAN_POINT('Ctrl Pts',(13.0508216223155,34.8958333401613,48.706329375));
#16087=CARTESIAN_POINT('Ctrl Pts',(-9.95098946405443E-15,34.687500006828,
48.706329375));
#16088=CARTESIAN_POINT('Ctrl Pts',(-13.0508216223155,34.4791666734946,48.706329375));
#16089=CARTESIAN_POINT('Ctrl Pts',(-24.3531646875,34.2708333401613,42.1809185638423));
#16090=CARTESIAN_POINT('Ctrl Pts',(-35.6555077526845,34.062500006828,35.6555077526845));
#16091=CARTESIAN_POINT('Ctrl Pts',(-42.1809185638422,33.8541666734946,24.3531646875));
#16092=CARTESIAN_POINT('Ctrl Pts',(-48.706329375,33.6458333401613,13.0508216223155));
#16093=CARTESIAN_POINT('Ctrl Pts',(-48.706329375,33.437500006828,-1.8898197019151E-14));
#16094=CARTESIAN_POINT('Ctrl Pts',(-48.706329375,33.2291666734946,-13.0508216223155));
#16095=CARTESIAN_POINT('Ctrl Pts',(-42.1809185638422,33.0208333401613,-24.3531646875));
#16096=CARTESIAN_POINT('Ctrl Pts',(-35.6555077526845,32.812500006828,-35.6555077526845));
#16097=CARTESIAN_POINT('Ctrl Pts',(-24.3531646875,32.6041666734946,-42.1809185638422));
#16098=CARTESIAN_POINT('Ctrl Pts',(-13.0508216223155,32.3958333401613,-48.706329375));
#16099=CARTESIAN_POINT('Ctrl Pts',(1.59157945007855E-14,32.187500006828,
-48.706329375));
#16100=CARTESIAN_POINT('Ctrl Pts',(13.0508216223155,31.9791666734946,-48.706329375));
#16101=CARTESIAN_POINT('Ctrl Pts',(24.3531646875,31.7708333401613,-42.1809185638422));
#16102=CARTESIAN_POINT('Ctrl Pts',(35.6555077526845,31.562500006828,-35.6555077526845));
#16103=CARTESIAN_POINT('Ctrl Pts',(42.1809185638422,31.3541666734946,-24.3531646875));
#16104=CARTESIAN_POINT('Ctrl Pts',(48.706329375,31.1458333401613,-13.0508216223155));
#16105=CARTESIAN_POINT('Ctrl Pts',(48.706329375,30.937500006828,1.293339198242E-14));
#16106=CARTESIAN_POINT('Ctrl Pts',(48.706329375,30.7291666734946,13.0508216223155));
#16107=CARTESIAN_POINT('Ctrl Pts',(42.1809185638422,30.5208333401613,24.3531646875));
#16108=CARTESIAN_POINT('Ctrl Pts',(35.6555077526845,30.312500006828,35.6555077526845));
#16109=CARTESIAN_POINT('Ctrl Pts',(24.3531646875,30.1041666734946,42.1809185638422));
#16110=CARTESIAN_POINT('Ctrl Pts',(13.0508216223155,29.8958333401613,48.706329375));
#16111=CARTESIAN_POINT('Ctrl Pts',(-9.95098946405443E-15,29.687500006828,
48.706329375));
#16112=CARTESIAN_POINT('Ctrl Pts',(-13.0508216223155,29.4791666734946,48.706329375));
#16113=CARTESIAN_POINT('Ctrl Pts',(-24.3531646875,29.2708333401613,42.1809185638423));
#16114=CARTESIAN_POINT('Ctrl Pts',(-35.6555077526845,29.062500006828,35.6555077526845));
#16115=CARTESIAN_POINT('Ctrl Pts',(-42.1809185638422,28.8541666734946,24.3531646875));
#16116=CARTESIAN_POINT('Ctrl Pts',(-48.706329375,28.6458333401613,13.0508216223155));
#16117=CARTESIAN_POINT('Ctrl Pts',(-48.706329375,28.437500006828,-1.8898197019151E-14));
#16118=CARTESIAN_POINT('Ctrl Pts',(-46.,60.,0.));
#16119=CARTESIAN_POINT('Ctrl Pts',(-46.,59.7916666666667,-12.3256628518316));
#16120=CARTESIAN_POINT('Ctrl Pts',(-39.8371685740842,59.5833333333333,-23.));
#16121=CARTESIAN_POINT('Ctrl Pts',(-33.6743371481684,59.375,-33.6743371481684));
#16122=CARTESIAN_POINT('Ctrl Pts',(-23.,59.1666666666667,-39.8371685740842));
#16123=CARTESIAN_POINT('Ctrl Pts',(-12.3256628518317,58.9583333333333,-46.));
#16124=CARTESIAN_POINT('Ctrl Pts',(-2.81668763803891E-15,58.75,-46.));
#16125=CARTESIAN_POINT('Ctrl Pts',(12.3256628518316,58.5416666666667,-46.));
#16126=CARTESIAN_POINT('Ctrl Pts',(23.,58.3333333333333,-39.8371685740842));
#16127=CARTESIAN_POINT('Ctrl Pts',(33.6743371481683,58.125,-33.6743371481684));
#16128=CARTESIAN_POINT('Ctrl Pts',(39.8371685740842,57.9166666666667,-23.));
#16129=CARTESIAN_POINT('Ctrl Pts',(46.,57.7083333333333,-12.3256628518317));
#16130=CARTESIAN_POINT('Ctrl Pts',(46.,57.5,-5.63337527607782E-15));
#16131=CARTESIAN_POINT('Ctrl Pts',(46.,57.2916666666667,12.3256628518316));
#16132=CARTESIAN_POINT('Ctrl Pts',(39.8371685740842,57.0833333333333,23.));
#16133=CARTESIAN_POINT('Ctrl Pts',(33.6743371481684,56.875,33.6743371481683));
#16134=CARTESIAN_POINT('Ctrl Pts',(23.,56.6666666666667,39.8371685740842));
#16135=CARTESIAN_POINT('Ctrl Pts',(12.3256628518317,56.4583333333333,46.));
#16136=CARTESIAN_POINT('Ctrl Pts',(8.45006291411674E-15,56.25,46.));
#16137=CARTESIAN_POINT('Ctrl Pts',(-12.3256628518316,56.0416666666667,46.));
#16138=CARTESIAN_POINT('Ctrl Pts',(-23.,55.8333333333333,39.8371685740842));
#16139=CARTESIAN_POINT('Ctrl Pts',(-33.6743371481683,55.625,33.6743371481684));
#16140=CARTESIAN_POINT('Ctrl Pts',(-39.8371685740842,55.4166666666667,23.));
#16141=CARTESIAN_POINT('Ctrl Pts',(-46.,55.2083333333333,12.3256628518317));
#16142=CARTESIAN_POINT('Ctrl Pts',(-46.,55.,0.));
#16143=CARTESIAN_POINT('Ctrl Pts',(-46.,54.7916666666667,-12.3256628518316));
#16144=CARTESIAN_POINT('Ctrl Pts',(-39.8371685740842,54.5833333333333,-23.));
#16145=CARTESIAN_POINT('Ctrl Pts',(-33.6743371481684,54.375,-33.6743371481684));
#16146=CARTESIAN_POINT('Ctrl Pts',(-23.,54.1666666666667,-39.8371685740842));
#16147=CARTESIAN_POINT('Ctrl Pts',(-12.3256628518317,53.9583333333333,-46.));
#16148=CARTESIAN_POINT('Ctrl Pts',(-2.81668763803891E-15,53.75,-46.));
#16149=CARTESIAN_POINT('Ctrl Pts',(12.3256628518316,53.5416666666667,-46.));
#16150=CARTESIAN_POINT('Ctrl Pts',(23.,53.3333333333333,-39.8371685740842));
#16151=CARTESIAN_POINT('Ctrl Pts',(33.6743371481683,53.125,-33.6743371481684));
#16152=CARTESIAN_POINT('Ctrl Pts',(39.8371685740842,52.9166666666667,-23.));
#16153=CARTESIAN_POINT('Ctrl Pts',(46.,52.7083333333333,-12.3256628518317));
#16154=CARTESIAN_POINT('Ctrl Pts',(46.,52.5,-5.63337527607782E-15));
#16155=CARTESIAN_POINT('Ctrl Pts',(46.,52.2916666666667,12.3256628518316));
#16156=CARTESIAN_POINT('Ctrl Pts',(39.8371685740842,52.0833333333333,23.));
#16157=CARTESIAN_POINT('Ctrl Pts',(33.6743371481684,51.875,33.6743371481683));
#16158=CARTESIAN_POINT('Ctrl Pts',(23.,51.6666666666667,39.8371685740842));
#16159=CARTESIAN_POINT('Ctrl Pts',(12.3256628518317,51.4583333333333,46.));
#16160=CARTESIAN_POINT('Ctrl Pts',(8.45006291411674E-15,51.25,46.));
#16161=CARTESIAN_POINT('Ctrl Pts',(-12.3256628518316,51.0416666666667,46.));
#16162=CARTESIAN_POINT('Ctrl Pts',(-23.,50.8333333333333,39.8371685740842));
#16163=CARTESIAN_POINT('Ctrl Pts',(-33.6743371481683,50.625,33.6743371481684));
#16164=CARTESIAN_POINT('Ctrl Pts',(-39.8371685740842,50.4166666666667,23.));
#16165=CARTESIAN_POINT('Ctrl Pts',(-46.,50.2083333333333,12.3256628518317));
#16166=CARTESIAN_POINT('Ctrl Pts',(-46.,50.,0.));
#16167=CARTESIAN_POINT('Ctrl Pts',(-46.,49.7916666666667,-12.3256628518316));
#16168=CARTESIAN_POINT('Ctrl Pts',(-39.8371685740842,49.5833333333333,-23.));
#16169=CARTESIAN_POINT('Ctrl Pts',(-33.6743371481684,49.375,-33.6743371481684));
#16170=CARTESIAN_POINT('Ctrl Pts',(-23.,49.1666666666667,-39.8371685740842));
#16171=CARTESIAN_POINT('Ctrl Pts',(-12.3256628518317,48.9583333333333,-46.));
#16172=CARTESIAN_POINT('Ctrl Pts',(-2.81668763803891E-15,48.75,-46.));
#16173=CARTESIAN_POINT('Ctrl Pts',(12.3256628518316,48.5416666666667,-46.));
#16174=CARTESIAN_POINT('Ctrl Pts',(23.,48.3333333333333,-39.8371685740842));
#16175=CARTESIAN_POINT('Ctrl Pts',(33.6743371481683,48.125,-33.6743371481684));
#16176=CARTESIAN_POINT('Ctrl Pts',(39.8371685740842,47.9166666666667,-23.));
#16177=CARTESIAN_POINT('Ctrl Pts',(46.,47.7083333333333,-12.3256628518317));
#16178=CARTESIAN_POINT('Ctrl Pts',(46.,47.5,-5.63337527607782E-15));
#16179=CARTESIAN_POINT('Ctrl Pts',(46.,47.2916666666667,12.3256628518316));
#16180=CARTESIAN_POINT('Ctrl Pts',(39.8371685740842,47.0833333333333,23.));
#16181=CARTESIAN_POINT('Ctrl Pts',(33.6743371481684,46.875,33.6743371481683));
#16182=CARTESIAN_POINT('Ctrl Pts',(23.,46.6666666666667,39.8371685740842));
#16183=CARTESIAN_POINT('Ctrl Pts',(12.3256628518317,46.4583333333333,46.));
#16184=CARTESIAN_POINT('Ctrl Pts',(8.45006291411674E-15,46.25,46.));
#16185=CARTESIAN_POINT('Ctrl Pts',(-12.3256628518316,46.0416666666667,46.));
#16186=CARTESIAN_POINT('Ctrl Pts',(-23.,45.8333333333333,39.8371685740842));
#16187=CARTESIAN_POINT('Ctrl Pts',(-33.6743371481683,45.625,33.6743371481684));
#16188=CARTESIAN_POINT('Ctrl Pts',(-39.8371685740842,45.4166666666667,23.));
#16189=CARTESIAN_POINT('Ctrl Pts',(-46.,45.2083333333333,12.3256628518317));
#16190=CARTESIAN_POINT('Ctrl Pts',(-46.,45.,0.));
#16191=CARTESIAN_POINT('Ctrl Pts',(-46.,44.7916666666667,-12.3256628518316));
#16192=CARTESIAN_POINT('Ctrl Pts',(-39.8371685740842,44.5833333333333,-23.));
#16193=CARTESIAN_POINT('Ctrl Pts',(-33.6743371481684,44.375,-33.6743371481684));
#16194=CARTESIAN_POINT('Ctrl Pts',(-23.,44.1666666666667,-39.8371685740842));
#16195=CARTESIAN_POINT('Ctrl Pts',(-12.3256628518317,43.9583333333333,-46.));
#16196=CARTESIAN_POINT('Ctrl Pts',(-2.81668763803891E-15,43.75,-46.));
#16197=CARTESIAN_POINT('Ctrl Pts',(12.3256628518316,43.5416666666667,-46.));
#16198=CARTESIAN_POINT('Ctrl Pts',(23.,43.3333333333333,-39.8371685740842));
#16199=CARTESIAN_POINT('Ctrl Pts',(33.6743371481683,43.125,-33.6743371481684));
#16200=CARTESIAN_POINT('Ctrl Pts',(39.8371685740842,42.9166666666667,-23.));
#16201=CARTESIAN_POINT('Ctrl Pts',(46.,42.7083333333333,-12.3256628518317));
#16202=CARTESIAN_POINT('Ctrl Pts',(46.,42.5,-5.63337527607782E-15));
#16203=CARTESIAN_POINT('Ctrl Pts',(46.,42.2916666666667,12.3256628518316));
#16204=CARTESIAN_POINT('Ctrl Pts',(39.8371685740842,42.0833333333333,23.));
#16205=CARTESIAN_POINT('Ctrl Pts',(33.6743371481684,41.875,33.6743371481683));
#16206=CARTESIAN_POINT('Ctrl Pts',(23.,41.6666666666667,39.8371685740842));
#16207=CARTESIAN_POINT('Ctrl Pts',(12.3256628518317,41.4583333333333,46.));
#16208=CARTESIAN_POINT('Ctrl Pts',(8.45006291411674E-15,41.25,46.));
#16209=CARTESIAN_POINT('Ctrl Pts',(-12.3256628518316,41.0416666666667,46.));
#16210=CARTESIAN_POINT('Ctrl Pts',(-23.,40.8333333333333,39.8371685740842));
#16211=CARTESIAN_POINT('Ctrl Pts',(-33.6743371481683,40.625,33.6743371481684));
#16212=CARTESIAN_POINT('Ctrl Pts',(-39.8371685740842,40.4166666666667,23.));
#16213=CARTESIAN_POINT('Ctrl Pts',(-46.,40.2083333333333,12.3256628518317));
#16214=CARTESIAN_POINT('Ctrl Pts',(-46.,40.,0.));
#16215=CARTESIAN_POINT('Ctrl Pts',(-46.,39.7916666666667,-12.3256628518316));
#16216=CARTESIAN_POINT('Ctrl Pts',(-39.8371685740842,39.5833333333333,-23.));
#16217=CARTESIAN_POINT('Ctrl Pts',(-33.6743371481684,39.375,-33.6743371481684));
#16218=CARTESIAN_POINT('Ctrl Pts',(-23.,39.1666666666667,-39.8371685740842));
#16219=CARTESIAN_POINT('Ctrl Pts',(-12.3256628518317,38.9583333333333,-46.));
#16220=CARTESIAN_POINT('Ctrl Pts',(-2.81668763803891E-15,38.75,-46.));
#16221=CARTESIAN_POINT('Ctrl Pts',(12.3256628518316,38.5416666666667,-46.));
#16222=CARTESIAN_POINT('Ctrl Pts',(23.,38.3333333333333,-39.8371685740842));
#16223=CARTESIAN_POINT('Ctrl Pts',(33.6743371481683,38.125,-33.6743371481684));
#16224=CARTESIAN_POINT('Ctrl Pts',(39.8371685740842,37.9166666666667,-23.));
#16225=CARTESIAN_POINT('Ctrl Pts',(46.,37.7083333333333,-12.3256628518317));
#16226=CARTESIAN_POINT('Ctrl Pts',(46.,37.5,-5.63337527607782E-15));
#16227=CARTESIAN_POINT('Ctrl Pts',(46.,37.2916666666667,12.3256628518316));
#16228=CARTESIAN_POINT('Ctrl Pts',(39.8371685740842,37.0833333333333,23.));
#16229=CARTESIAN_POINT('Ctrl Pts',(33.6743371481684,36.875,33.6743371481683));
#16230=CARTESIAN_POINT('Ctrl Pts',(23.,36.6666666666667,39.8371685740842));
#16231=CARTESIAN_POINT('Ctrl Pts',(12.3256628518317,36.4583333333333,46.));
#16232=CARTESIAN_POINT('Ctrl Pts',(8.45006291411674E-15,36.25,46.));
#16233=CARTESIAN_POINT('Ctrl Pts',(-12.3256628518316,36.0416666666667,46.));
#16234=CARTESIAN_POINT('Ctrl Pts',(-23.,35.8333333333333,39.8371685740842));
#16235=CARTESIAN_POINT('Ctrl Pts',(-33.6743371481683,35.625,33.6743371481684));
#16236=CARTESIAN_POINT('Ctrl Pts',(-39.8371685740842,35.4166666666667,23.));
#16237=CARTESIAN_POINT('Ctrl Pts',(-46.,35.2083333333333,12.3256628518317));
#16238=CARTESIAN_POINT('Ctrl Pts',(-46.,35.,0.));
#16239=CARTESIAN_POINT('Ctrl Pts',(-46.,34.7916666666667,-12.3256628518316));
#16240=CARTESIAN_POINT('Ctrl Pts',(-39.8371685740842,34.5833333333333,-23.));
#16241=CARTESIAN_POINT('Ctrl Pts',(-33.6743371481684,34.375,-33.6743371481684));
#16242=CARTESIAN_POINT('Ctrl Pts',(-23.,34.1666666666667,-39.8371685740842));
#16243=CARTESIAN_POINT('Ctrl Pts',(-12.3256628518317,33.9583333333333,-46.));
#16244=CARTESIAN_POINT('Ctrl Pts',(-2.81668763803891E-15,33.75,-46.));
#16245=CARTESIAN_POINT('Ctrl Pts',(12.3256628518316,33.5416666666667,-46.));
#16246=CARTESIAN_POINT('Ctrl Pts',(23.,33.3333333333333,-39.8371685740842));
#16247=CARTESIAN_POINT('Ctrl Pts',(33.6743371481683,33.125,-33.6743371481684));
#16248=CARTESIAN_POINT('Ctrl Pts',(39.8371685740842,32.9166666666667,-23.));
#16249=CARTESIAN_POINT('Ctrl Pts',(46.,32.7083333333333,-12.3256628518317));
#16250=CARTESIAN_POINT('Ctrl Pts',(46.,32.5,-5.63337527607782E-15));
#16251=CARTESIAN_POINT('Ctrl Pts',(46.,32.2916666666667,12.3256628518316));
#16252=CARTESIAN_POINT('Ctrl Pts',(39.8371685740842,32.0833333333333,23.));
#16253=CARTESIAN_POINT('Ctrl Pts',(33.6743371481684,31.875,33.6743371481683));
#16254=CARTESIAN_POINT('Ctrl Pts',(23.,31.6666666666667,39.8371685740842));
#16255=CARTESIAN_POINT('Ctrl Pts',(12.3256628518317,31.4583333333333,46.));
#16256=CARTESIAN_POINT('Ctrl Pts',(8.45006291411674E-15,31.25,46.));
#16257=CARTESIAN_POINT('Ctrl Pts',(-12.3256628518316,31.0416666666667,46.));
#16258=CARTESIAN_POINT('Ctrl Pts',(-23.,30.8333333333333,39.8371685740842));
#16259=CARTESIAN_POINT('Ctrl Pts',(-33.6743371481683,30.625,33.6743371481684));
#16260=CARTESIAN_POINT('Ctrl Pts',(-39.8371685740842,30.4166666666667,23.));
#16261=CARTESIAN_POINT('Ctrl Pts',(-46.,30.2083333333333,12.3256628518317));
#16262=CARTESIAN_POINT('Ctrl Pts',(-46.,30.,0.));
#16263=CARTESIAN_POINT('Ctrl Pts',(-45.858362923034,40.061608680256,3.60701400320328));
#16264=CARTESIAN_POINT('Ctrl Pts',(-46.089925771934,39.9280150456296,3.60701400320328));
#16265=CARTESIAN_POINT('Ctrl Pts',(-46.5530501979845,39.6608255719955,3.60701400320308));
#16266=CARTESIAN_POINT('Ctrl Pts',(-47.0161721905706,39.3936318804496,3.60701400320335));
#16267=CARTESIAN_POINT('Ctrl Pts',(-47.6893519862319,39.0052434879083,3.60701400320335));
#16268=CARTESIAN_POINT('Ctrl Pts',(-48.1309692507094,38.7504492807381,3.60701400320327));
#16269=CARTESIAN_POINT('Ctrl Pts',(-48.5725845633798,38.4956516907297,3.60701400320327));
#16270=CARTESIAN_POINT('Origin',(-4.32456261881337,-7931.57954062375,-4524.0108739909));
#16271=CARTESIAN_POINT('Ctrl Pts',(-48.706329375,58.437500006828,-1.8898197019151E-14));
#16272=CARTESIAN_POINT('Ctrl Pts',(-48.706329375,58.2291666734946,-13.0508216223155));
#16273=CARTESIAN_POINT('Ctrl Pts',(-42.1809185638422,58.0208333401613,-24.3531646875));
#16274=CARTESIAN_POINT('Ctrl Pts',(-35.6555077526845,57.812500006828,-35.6555077526845));
#16275=CARTESIAN_POINT('Ctrl Pts',(-24.3531646875,57.6041666734946,-42.1809185638422));
#16276=CARTESIAN_POINT('Ctrl Pts',(-13.0508216223155,57.3958333401613,-48.706329375));
#16277=CARTESIAN_POINT('Ctrl Pts',(1.59157945007855E-14,57.187500006828,
-48.706329375));
#16278=CARTESIAN_POINT('Ctrl Pts',(13.0508216223155,56.9791666734946,-48.706329375));
#16279=CARTESIAN_POINT('Ctrl Pts',(24.3531646875,56.7708333401613,-42.1809185638422));
#16280=CARTESIAN_POINT('Ctrl Pts',(35.6555077526845,56.562500006828,-35.6555077526845));
#16281=CARTESIAN_POINT('Ctrl Pts',(42.1809185638422,56.3541666734946,-24.3531646875));
#16282=CARTESIAN_POINT('Ctrl Pts',(48.706329375,56.1458333401613,-13.0508216223155));
#16283=CARTESIAN_POINT('Ctrl Pts',(48.706329375,55.937500006828,1.293339198242E-14));
#16284=CARTESIAN_POINT('Ctrl Pts',(48.706329375,55.7291666734946,13.0508216223155));
#16285=CARTESIAN_POINT('Ctrl Pts',(42.1809185638422,55.5208333401613,24.3531646875));
#16286=CARTESIAN_POINT('Ctrl Pts',(35.6555077526845,55.312500006828,35.6555077526845));
#16287=CARTESIAN_POINT('Ctrl Pts',(24.3531646875,55.1041666734946,42.1809185638422));
#16288=CARTESIAN_POINT('Ctrl Pts',(13.0508216223155,54.8958333401613,48.706329375));
#16289=CARTESIAN_POINT('Ctrl Pts',(-9.95098946405443E-15,54.687500006828,
48.706329375));
#16290=CARTESIAN_POINT('Ctrl Pts',(-13.0508216223155,54.4791666734946,48.706329375));
#16291=CARTESIAN_POINT('Ctrl Pts',(-24.3531646875,54.2708333401613,42.1809185638423));
#16292=CARTESIAN_POINT('Ctrl Pts',(-35.6555077526845,54.062500006828,35.6555077526845));
#16293=CARTESIAN_POINT('Ctrl Pts',(-42.1809185638422,53.8541666734946,24.3531646875));
#16294=CARTESIAN_POINT('Ctrl Pts',(-48.706329375,53.6458333401613,13.0508216223155));
#16295=CARTESIAN_POINT('Ctrl Pts',(-48.706329375,53.437500006828,-1.8898197019151E-14));
#16296=CARTESIAN_POINT('Ctrl Pts',(-48.706329375,53.2291666734946,-13.0508216223155));
#16297=CARTESIAN_POINT('Ctrl Pts',(-42.1809185638422,53.0208333401613,-24.3531646875));
#16298=CARTESIAN_POINT('Ctrl Pts',(-35.6555077526845,52.812500006828,-35.6555077526845));
#16299=CARTESIAN_POINT('Ctrl Pts',(-24.3531646875,52.6041666734946,-42.1809185638422));
#16300=CARTESIAN_POINT('Ctrl Pts',(-13.0508216223155,52.3958333401613,-48.706329375));
#16301=CARTESIAN_POINT('Ctrl Pts',(1.59157945007855E-14,52.187500006828,
-48.706329375));
#16302=CARTESIAN_POINT('Ctrl Pts',(13.0508216223155,51.9791666734946,-48.706329375));
#16303=CARTESIAN_POINT('Ctrl Pts',(24.3531646875,51.7708333401613,-42.1809185638422));
#16304=CARTESIAN_POINT('Ctrl Pts',(35.6555077526845,51.562500006828,-35.6555077526845));
#16305=CARTESIAN_POINT('Ctrl Pts',(42.1809185638422,51.3541666734946,-24.3531646875));
#16306=CARTESIAN_POINT('Ctrl Pts',(48.706329375,51.1458333401613,-13.0508216223155));
#16307=CARTESIAN_POINT('Ctrl Pts',(48.706329375,50.937500006828,1.293339198242E-14));
#16308=CARTESIAN_POINT('Ctrl Pts',(48.706329375,50.7291666734946,13.0508216223155));
#16309=CARTESIAN_POINT('Ctrl Pts',(42.1809185638422,50.5208333401613,24.3531646875));
#16310=CARTESIAN_POINT('Ctrl Pts',(35.6555077526845,50.312500006828,35.6555077526845));
#16311=CARTESIAN_POINT('Ctrl Pts',(24.3531646875,50.1041666734946,42.1809185638422));
#16312=CARTESIAN_POINT('Ctrl Pts',(13.0508216223155,49.8958333401613,48.706329375));
#16313=CARTESIAN_POINT('Ctrl Pts',(-9.95098946405443E-15,49.687500006828,
48.706329375));
#16314=CARTESIAN_POINT('Ctrl Pts',(-13.0508216223155,49.4791666734946,48.706329375));
#16315=CARTESIAN_POINT('Ctrl Pts',(-24.3531646875,49.2708333401613,42.1809185638423));
#16316=CARTESIAN_POINT('Ctrl Pts',(-35.6555077526845,49.062500006828,35.6555077526845));
#16317=CARTESIAN_POINT('Ctrl Pts',(-42.1809185638422,48.8541666734946,24.3531646875));
#16318=CARTESIAN_POINT('Ctrl Pts',(-48.706329375,48.6458333401613,13.0508216223155));
#16319=CARTESIAN_POINT('Ctrl Pts',(-48.706329375,48.437500006828,-1.8898197019151E-14));
#16320=CARTESIAN_POINT('Ctrl Pts',(-48.706329375,48.2291666734946,-13.0508216223155));
#16321=CARTESIAN_POINT('Ctrl Pts',(-42.1809185638422,48.0208333401613,-24.3531646875));
#16322=CARTESIAN_POINT('Ctrl Pts',(-35.6555077526845,47.812500006828,-35.6555077526845));
#16323=CARTESIAN_POINT('Ctrl Pts',(-24.3531646875,47.6041666734946,-42.1809185638422));
#16324=CARTESIAN_POINT('Ctrl Pts',(-13.0508216223155,47.3958333401613,-48.706329375));
#16325=CARTESIAN_POINT('Ctrl Pts',(1.59157945007855E-14,47.187500006828,
-48.706329375));
#16326=CARTESIAN_POINT('Ctrl Pts',(13.0508216223155,46.9791666734946,-48.706329375));
#16327=CARTESIAN_POINT('Ctrl Pts',(24.3531646875,46.7708333401613,-42.1809185638422));
#16328=CARTESIAN_POINT('Ctrl Pts',(35.6555077526845,46.562500006828,-35.6555077526845));
#16329=CARTESIAN_POINT('Ctrl Pts',(42.1809185638422,46.3541666734946,-24.3531646875));
#16330=CARTESIAN_POINT('Ctrl Pts',(48.706329375,46.1458333401613,-13.0508216223155));
#16331=CARTESIAN_POINT('Ctrl Pts',(48.706329375,45.937500006828,1.293339198242E-14));
#16332=CARTESIAN_POINT('Ctrl Pts',(48.706329375,45.7291666734946,13.0508216223155));
#16333=CARTESIAN_POINT('Ctrl Pts',(42.1809185638422,45.5208333401613,24.3531646875));
#16334=CARTESIAN_POINT('Ctrl Pts',(35.6555077526845,45.312500006828,35.6555077526845));
#16335=CARTESIAN_POINT('Ctrl Pts',(24.3531646875,45.1041666734946,42.1809185638422));
#16336=CARTESIAN_POINT('Ctrl Pts',(13.0508216223155,44.8958333401613,48.706329375));
#16337=CARTESIAN_POINT('Ctrl Pts',(-9.95098946405443E-15,44.687500006828,
48.706329375));
#16338=CARTESIAN_POINT('Ctrl Pts',(-13.0508216223155,44.4791666734946,48.706329375));
#16339=CARTESIAN_POINT('Ctrl Pts',(-24.3531646875,44.2708333401613,42.1809185638423));
#16340=CARTESIAN_POINT('Ctrl Pts',(-35.6555077526845,44.062500006828,35.6555077526845));
#16341=CARTESIAN_POINT('Ctrl Pts',(-42.1809185638422,43.8541666734946,24.3531646875));
#16342=CARTESIAN_POINT('Ctrl Pts',(-48.706329375,43.6458333401613,13.0508216223155));
#16343=CARTESIAN_POINT('Ctrl Pts',(-48.706329375,43.437500006828,-1.8898197019151E-14));
#16344=CARTESIAN_POINT('Ctrl Pts',(-48.706329375,43.2291666734946,-13.0508216223155));
#16345=CARTESIAN_POINT('Ctrl Pts',(-42.1809185638422,43.0208333401613,-24.3531646875));
#16346=CARTESIAN_POINT('Ctrl Pts',(-35.6555077526845,42.812500006828,-35.6555077526845));
#16347=CARTESIAN_POINT('Ctrl Pts',(-24.3531646875,42.6041666734946,-42.1809185638422));
#16348=CARTESIAN_POINT('Ctrl Pts',(-13.0508216223155,42.3958333401613,-48.706329375));
#16349=CARTESIAN_POINT('Ctrl Pts',(1.59157945007855E-14,42.187500006828,
-48.706329375));
#16350=CARTESIAN_POINT('Ctrl Pts',(13.0508216223155,41.9791666734946,-48.706329375));
#16351=CARTESIAN_POINT('Ctrl Pts',(24.3531646875,41.7708333401613,-42.1809185638422));
#16352=CARTESIAN_POINT('Ctrl Pts',(35.6555077526845,41.562500006828,-35.6555077526845));
#16353=CARTESIAN_POINT('Ctrl Pts',(42.1809185638422,41.3541666734946,-24.3531646875));
#16354=CARTESIAN_POINT('Ctrl Pts',(48.706329375,41.1458333401613,-13.0508216223155));
#16355=CARTESIAN_POINT('Ctrl Pts',(48.706329375,40.937500006828,1.293339198242E-14));
#16356=CARTESIAN_POINT('Ctrl Pts',(48.706329375,40.7291666734946,13.0508216223155));
#16357=CARTESIAN_POINT('Ctrl Pts',(42.1809185638422,40.5208333401613,24.3531646875));
#16358=CARTESIAN_POINT('Ctrl Pts',(35.6555077526845,40.312500006828,35.6555077526845));
#16359=CARTESIAN_POINT('Ctrl Pts',(24.3531646875,40.1041666734946,42.1809185638422));
#16360=CARTESIAN_POINT('Ctrl Pts',(13.0508216223155,39.8958333401613,48.706329375));
#16361=CARTESIAN_POINT('Ctrl Pts',(-9.95098946405443E-15,39.687500006828,
48.706329375));
#16362=CARTESIAN_POINT('Ctrl Pts',(-13.0508216223155,39.4791666734946,48.706329375));
#16363=CARTESIAN_POINT('Ctrl Pts',(-24.3531646875,39.2708333401613,42.1809185638423));
#16364=CARTESIAN_POINT('Ctrl Pts',(-35.6555077526845,39.062500006828,35.6555077526845));
#16365=CARTESIAN_POINT('Ctrl Pts',(-42.1809185638422,38.8541666734946,24.3531646875));
#16366=CARTESIAN_POINT('Ctrl Pts',(-48.706329375,38.6458333401613,13.0508216223155));
#16367=CARTESIAN_POINT('Ctrl Pts',(-48.706329375,38.437500006828,-1.8898197019151E-14));
#16368=CARTESIAN_POINT('Ctrl Pts',(-48.706329375,38.2291666734946,-13.0508216223155));
#16369=CARTESIAN_POINT('Ctrl Pts',(-42.1809185638422,38.0208333401613,-24.3531646875));
#16370=CARTESIAN_POINT('Ctrl Pts',(-35.6555077526845,37.812500006828,-35.6555077526845));
#16371=CARTESIAN_POINT('Ctrl Pts',(-24.3531646875,37.6041666734946,-42.1809185638422));
#16372=CARTESIAN_POINT('Ctrl Pts',(-13.0508216223155,37.3958333401613,-48.706329375));
#16373=CARTESIAN_POINT('Ctrl Pts',(1.59157945007855E-14,37.187500006828,
-48.706329375));
#16374=CARTESIAN_POINT('Ctrl Pts',(13.0508216223155,36.9791666734946,-48.706329375));
#16375=CARTESIAN_POINT('Ctrl Pts',(24.3531646875,36.7708333401613,-42.1809185638422));
#16376=CARTESIAN_POINT('Ctrl Pts',(35.6555077526845,36.562500006828,-35.6555077526845));
#16377=CARTESIAN_POINT('Ctrl Pts',(42.1809185638422,36.3541666734946,-24.3531646875));
#16378=CARTESIAN_POINT('Ctrl Pts',(48.706329375,36.1458333401613,-13.0508216223155));
#16379=CARTESIAN_POINT('Ctrl Pts',(48.706329375,35.937500006828,1.293339198242E-14));
#16380=CARTESIAN_POINT('Ctrl Pts',(48.706329375,35.7291666734946,13.0508216223155));
#16381=CARTESIAN_POINT('Ctrl Pts',(42.1809185638422,35.5208333401613,24.3531646875));
#16382=CARTESIAN_POINT('Ctrl Pts',(35.6555077526845,35.312500006828,35.6555077526845));
#16383=CARTESIAN_POINT('Ctrl Pts',(24.3531646875,35.1041666734946,42.1809185638422));
#16384=CARTESIAN_POINT('Ctrl Pts',(13.0508216223155,34.8958333401613,48.706329375));
#16385=CARTESIAN_POINT('Ctrl Pts',(-9.95098946405443E-15,34.687500006828,
48.706329375));
#16386=CARTESIAN_POINT('Ctrl Pts',(-13.0508216223155,34.4791666734946,48.706329375));
#16387=CARTESIAN_POINT('Ctrl Pts',(-24.3531646875,34.2708333401613,42.1809185638423));
#16388=CARTESIAN_POINT('Ctrl Pts',(-35.6555077526845,34.062500006828,35.6555077526845));
#16389=CARTESIAN_POINT('Ctrl Pts',(-42.1809185638422,33.8541666734946,24.3531646875));
#16390=CARTESIAN_POINT('Ctrl Pts',(-48.706329375,33.6458333401613,13.0508216223155));
#16391=CARTESIAN_POINT('Ctrl Pts',(-48.706329375,33.437500006828,-1.8898197019151E-14));
#16392=CARTESIAN_POINT('Ctrl Pts',(-48.706329375,33.2291666734946,-13.0508216223155));
#16393=CARTESIAN_POINT('Ctrl Pts',(-42.1809185638422,33.0208333401613,-24.3531646875));
#16394=CARTESIAN_POINT('Ctrl Pts',(-35.6555077526845,32.812500006828,-35.6555077526845));
#16395=CARTESIAN_POINT('Ctrl Pts',(-24.3531646875,32.6041666734946,-42.1809185638422));
#16396=CARTESIAN_POINT('Ctrl Pts',(-13.0508216223155,32.3958333401613,-48.706329375));
#16397=CARTESIAN_POINT('Ctrl Pts',(1.59157945007855E-14,32.187500006828,
-48.706329375));
#16398=CARTESIAN_POINT('Ctrl Pts',(13.0508216223155,31.9791666734946,-48.706329375));
#16399=CARTESIAN_POINT('Ctrl Pts',(24.3531646875,31.7708333401613,-42.1809185638422));
#16400=CARTESIAN_POINT('Ctrl Pts',(35.6555077526845,31.562500006828,-35.6555077526845));
#16401=CARTESIAN_POINT('Ctrl Pts',(42.1809185638422,31.3541666734946,-24.3531646875));
#16402=CARTESIAN_POINT('Ctrl Pts',(48.706329375,31.1458333401613,-13.0508216223155));
#16403=CARTESIAN_POINT('Ctrl Pts',(48.706329375,30.937500006828,1.293339198242E-14));
#16404=CARTESIAN_POINT('Ctrl Pts',(48.706329375,30.7291666734946,13.0508216223155));
#16405=CARTESIAN_POINT('Ctrl Pts',(42.1809185638422,30.5208333401613,24.3531646875));
#16406=CARTESIAN_POINT('Ctrl Pts',(35.6555077526845,30.312500006828,35.6555077526845));
#16407=CARTESIAN_POINT('Ctrl Pts',(24.3531646875,30.1041666734946,42.1809185638422));
#16408=CARTESIAN_POINT('Ctrl Pts',(13.0508216223155,29.8958333401613,48.706329375));
#16409=CARTESIAN_POINT('Ctrl Pts',(-9.95098946405443E-15,29.687500006828,
48.706329375));
#16410=CARTESIAN_POINT('Ctrl Pts',(-13.0508216223155,29.4791666734946,48.706329375));
#16411=CARTESIAN_POINT('Ctrl Pts',(-24.3531646875,29.2708333401613,42.1809185638423));
#16412=CARTESIAN_POINT('Ctrl Pts',(-35.6555077526845,29.062500006828,35.6555077526845));
#16413=CARTESIAN_POINT('Ctrl Pts',(-42.1809185638422,28.8541666734946,24.3531646875));
#16414=CARTESIAN_POINT('Ctrl Pts',(-48.706329375,28.6458333401613,13.0508216223155));
#16415=CARTESIAN_POINT('Ctrl Pts',(-48.706329375,28.437500006828,-1.8898197019151E-14));
#16416=CARTESIAN_POINT('Ctrl Pts',(-46.,60.,0.));
#16417=CARTESIAN_POINT('Ctrl Pts',(-46.,59.7916666666667,-12.3256628518316));
#16418=CARTESIAN_POINT('Ctrl Pts',(-39.8371685740842,59.5833333333333,-23.));
#16419=CARTESIAN_POINT('Ctrl Pts',(-33.6743371481684,59.375,-33.6743371481684));
#16420=CARTESIAN_POINT('Ctrl Pts',(-23.,59.1666666666667,-39.8371685740842));
#16421=CARTESIAN_POINT('Ctrl Pts',(-12.3256628518317,58.9583333333333,-46.));
#16422=CARTESIAN_POINT('Ctrl Pts',(-2.81668763803891E-15,58.75,-46.));
#16423=CARTESIAN_POINT('Ctrl Pts',(12.3256628518316,58.5416666666667,-46.));
#16424=CARTESIAN_POINT('Ctrl Pts',(23.,58.3333333333333,-39.8371685740842));
#16425=CARTESIAN_POINT('Ctrl Pts',(33.6743371481683,58.125,-33.6743371481684));
#16426=CARTESIAN_POINT('Ctrl Pts',(39.8371685740842,57.9166666666667,-23.));
#16427=CARTESIAN_POINT('Ctrl Pts',(46.,57.7083333333333,-12.3256628518317));
#16428=CARTESIAN_POINT('Ctrl Pts',(46.,57.5,-5.63337527607782E-15));
#16429=CARTESIAN_POINT('Ctrl Pts',(46.,57.2916666666667,12.3256628518316));
#16430=CARTESIAN_POINT('Ctrl Pts',(39.8371685740842,57.0833333333333,23.));
#16431=CARTESIAN_POINT('Ctrl Pts',(33.6743371481684,56.875,33.6743371481683));
#16432=CARTESIAN_POINT('Ctrl Pts',(23.,56.6666666666667,39.8371685740842));
#16433=CARTESIAN_POINT('Ctrl Pts',(12.3256628518317,56.4583333333333,46.));
#16434=CARTESIAN_POINT('Ctrl Pts',(8.45006291411674E-15,56.25,46.));
#16435=CARTESIAN_POINT('Ctrl Pts',(-12.3256628518316,56.0416666666667,46.));
#16436=CARTESIAN_POINT('Ctrl Pts',(-23.,55.8333333333333,39.8371685740842));
#16437=CARTESIAN_POINT('Ctrl Pts',(-33.6743371481683,55.625,33.6743371481684));
#16438=CARTESIAN_POINT('Ctrl Pts',(-39.8371685740842,55.4166666666667,23.));
#16439=CARTESIAN_POINT('Ctrl Pts',(-46.,55.2083333333333,12.3256628518317));
#16440=CARTESIAN_POINT('Ctrl Pts',(-46.,55.,0.));
#16441=CARTESIAN_POINT('Ctrl Pts',(-46.,54.7916666666667,-12.3256628518316));
#16442=CARTESIAN_POINT('Ctrl Pts',(-39.8371685740842,54.5833333333333,-23.));
#16443=CARTESIAN_POINT('Ctrl Pts',(-33.6743371481684,54.375,-33.6743371481684));
#16444=CARTESIAN_POINT('Ctrl Pts',(-23.,54.1666666666667,-39.8371685740842));
#16445=CARTESIAN_POINT('Ctrl Pts',(-12.3256628518317,53.9583333333333,-46.));
#16446=CARTESIAN_POINT('Ctrl Pts',(-2.81668763803891E-15,53.75,-46.));
#16447=CARTESIAN_POINT('Ctrl Pts',(12.3256628518316,53.5416666666667,-46.));
#16448=CARTESIAN_POINT('Ctrl Pts',(23.,53.3333333333333,-39.8371685740842));
#16449=CARTESIAN_POINT('Ctrl Pts',(33.6743371481683,53.125,-33.6743371481684));
#16450=CARTESIAN_POINT('Ctrl Pts',(39.8371685740842,52.9166666666667,-23.));
#16451=CARTESIAN_POINT('Ctrl Pts',(46.,52.7083333333333,-12.3256628518317));
#16452=CARTESIAN_POINT('Ctrl Pts',(46.,52.5,-5.63337527607782E-15));
#16453=CARTESIAN_POINT('Ctrl Pts',(46.,52.2916666666667,12.3256628518316));
#16454=CARTESIAN_POINT('Ctrl Pts',(39.8371685740842,52.0833333333333,23.));
#16455=CARTESIAN_POINT('Ctrl Pts',(33.6743371481684,51.875,33.6743371481683));
#16456=CARTESIAN_POINT('Ctrl Pts',(23.,51.6666666666667,39.8371685740842));
#16457=CARTESIAN_POINT('Ctrl Pts',(12.3256628518317,51.4583333333333,46.));
#16458=CARTESIAN_POINT('Ctrl Pts',(8.45006291411674E-15,51.25,46.));
#16459=CARTESIAN_POINT('Ctrl Pts',(-12.3256628518316,51.0416666666667,46.));
#16460=CARTESIAN_POINT('Ctrl Pts',(-23.,50.8333333333333,39.8371685740842));
#16461=CARTESIAN_POINT('Ctrl Pts',(-33.6743371481683,50.625,33.6743371481684));
#16462=CARTESIAN_POINT('Ctrl Pts',(-39.8371685740842,50.4166666666667,23.));
#16463=CARTESIAN_POINT('Ctrl Pts',(-46.,50.2083333333333,12.3256628518317));
#16464=CARTESIAN_POINT('Ctrl Pts',(-46.,50.,0.));
#16465=CARTESIAN_POINT('Ctrl Pts',(-46.,49.7916666666667,-12.3256628518316));
#16466=CARTESIAN_POINT('Ctrl Pts',(-39.8371685740842,49.5833333333333,-23.));
#16467=CARTESIAN_POINT('Ctrl Pts',(-33.6743371481684,49.375,-33.6743371481684));
#16468=CARTESIAN_POINT('Ctrl Pts',(-23.,49.1666666666667,-39.8371685740842));
#16469=CARTESIAN_POINT('Ctrl Pts',(-12.3256628518317,48.9583333333333,-46.));
#16470=CARTESIAN_POINT('Ctrl Pts',(-2.81668763803891E-15,48.75,-46.));
#16471=CARTESIAN_POINT('Ctrl Pts',(12.3256628518316,48.5416666666667,-46.));
#16472=CARTESIAN_POINT('Ctrl Pts',(23.,48.3333333333333,-39.8371685740842));
#16473=CARTESIAN_POINT('Ctrl Pts',(33.6743371481683,48.125,-33.6743371481684));
#16474=CARTESIAN_POINT('Ctrl Pts',(39.8371685740842,47.9166666666667,-23.));
#16475=CARTESIAN_POINT('Ctrl Pts',(46.,47.7083333333333,-12.3256628518317));
#16476=CARTESIAN_POINT('Ctrl Pts',(46.,47.5,-5.63337527607782E-15));
#16477=CARTESIAN_POINT('Ctrl Pts',(46.,47.2916666666667,12.3256628518316));
#16478=CARTESIAN_POINT('Ctrl Pts',(39.8371685740842,47.0833333333333,23.));
#16479=CARTESIAN_POINT('Ctrl Pts',(33.6743371481684,46.875,33.6743371481683));
#16480=CARTESIAN_POINT('Ctrl Pts',(23.,46.6666666666667,39.8371685740842));
#16481=CARTESIAN_POINT('Ctrl Pts',(12.3256628518317,46.4583333333333,46.));
#16482=CARTESIAN_POINT('Ctrl Pts',(8.45006291411674E-15,46.25,46.));
#16483=CARTESIAN_POINT('Ctrl Pts',(-12.3256628518316,46.0416666666667,46.));
#16484=CARTESIAN_POINT('Ctrl Pts',(-23.,45.8333333333333,39.8371685740842));
#16485=CARTESIAN_POINT('Ctrl Pts',(-33.6743371481683,45.625,33.6743371481684));
#16486=CARTESIAN_POINT('Ctrl Pts',(-39.8371685740842,45.4166666666667,23.));
#16487=CARTESIAN_POINT('Ctrl Pts',(-46.,45.2083333333333,12.3256628518317));
#16488=CARTESIAN_POINT('Ctrl Pts',(-46.,45.,0.));
#16489=CARTESIAN_POINT('Ctrl Pts',(-46.,44.7916666666667,-12.3256628518316));
#16490=CARTESIAN_POINT('Ctrl Pts',(-39.8371685740842,44.5833333333333,-23.));
#16491=CARTESIAN_POINT('Ctrl Pts',(-33.6743371481684,44.375,-33.6743371481684));
#16492=CARTESIAN_POINT('Ctrl Pts',(-23.,44.1666666666667,-39.8371685740842));
#16493=CARTESIAN_POINT('Ctrl Pts',(-12.3256628518317,43.9583333333333,-46.));
#16494=CARTESIAN_POINT('Ctrl Pts',(-2.81668763803891E-15,43.75,-46.));
#16495=CARTESIAN_POINT('Ctrl Pts',(12.3256628518316,43.5416666666667,-46.));
#16496=CARTESIAN_POINT('Ctrl Pts',(23.,43.3333333333333,-39.8371685740842));
#16497=CARTESIAN_POINT('Ctrl Pts',(33.6743371481683,43.125,-33.6743371481684));
#16498=CARTESIAN_POINT('Ctrl Pts',(39.8371685740842,42.9166666666667,-23.));
#16499=CARTESIAN_POINT('Ctrl Pts',(46.,42.7083333333333,-12.3256628518317));
#16500=CARTESIAN_POINT('Ctrl Pts',(46.,42.5,-5.63337527607782E-15));
#16501=CARTESIAN_POINT('Ctrl Pts',(46.,42.2916666666667,12.3256628518316));
#16502=CARTESIAN_POINT('Ctrl Pts',(39.8371685740842,42.0833333333333,23.));
#16503=CARTESIAN_POINT('Ctrl Pts',(33.6743371481684,41.875,33.6743371481683));
#16504=CARTESIAN_POINT('Ctrl Pts',(23.,41.6666666666667,39.8371685740842));
#16505=CARTESIAN_POINT('Ctrl Pts',(12.3256628518317,41.4583333333333,46.));
#16506=CARTESIAN_POINT('Ctrl Pts',(8.45006291411674E-15,41.25,46.));
#16507=CARTESIAN_POINT('Ctrl Pts',(-12.3256628518316,41.0416666666667,46.));
#16508=CARTESIAN_POINT('Ctrl Pts',(-23.,40.8333333333333,39.8371685740842));
#16509=CARTESIAN_POINT('Ctrl Pts',(-33.6743371481683,40.625,33.6743371481684));
#16510=CARTESIAN_POINT('Ctrl Pts',(-39.8371685740842,40.4166666666667,23.));
#16511=CARTESIAN_POINT('Ctrl Pts',(-46.,40.2083333333333,12.3256628518317));
#16512=CARTESIAN_POINT('Ctrl Pts',(-46.,40.,0.));
#16513=CARTESIAN_POINT('Ctrl Pts',(-46.,39.7916666666667,-12.3256628518316));
#16514=CARTESIAN_POINT('Ctrl Pts',(-39.8371685740842,39.5833333333333,-23.));
#16515=CARTESIAN_POINT('Ctrl Pts',(-33.6743371481684,39.375,-33.6743371481684));
#16516=CARTESIAN_POINT('Ctrl Pts',(-23.,39.1666666666667,-39.8371685740842));
#16517=CARTESIAN_POINT('Ctrl Pts',(-12.3256628518317,38.9583333333333,-46.));
#16518=CARTESIAN_POINT('Ctrl Pts',(-2.81668763803891E-15,38.75,-46.));
#16519=CARTESIAN_POINT('Ctrl Pts',(12.3256628518316,38.5416666666667,-46.));
#16520=CARTESIAN_POINT('Ctrl Pts',(23.,38.3333333333333,-39.8371685740842));
#16521=CARTESIAN_POINT('Ctrl Pts',(33.6743371481683,38.125,-33.6743371481684));
#16522=CARTESIAN_POINT('Ctrl Pts',(39.8371685740842,37.9166666666667,-23.));
#16523=CARTESIAN_POINT('Ctrl Pts',(46.,37.7083333333333,-12.3256628518317));
#16524=CARTESIAN_POINT('Ctrl Pts',(46.,37.5,-5.63337527607782E-15));
#16525=CARTESIAN_POINT('Ctrl Pts',(46.,37.2916666666667,12.3256628518316));
#16526=CARTESIAN_POINT('Ctrl Pts',(39.8371685740842,37.0833333333333,23.));
#16527=CARTESIAN_POINT('Ctrl Pts',(33.6743371481684,36.875,33.6743371481683));
#16528=CARTESIAN_POINT('Ctrl Pts',(23.,36.6666666666667,39.8371685740842));
#16529=CARTESIAN_POINT('Ctrl Pts',(12.3256628518317,36.4583333333333,46.));
#16530=CARTESIAN_POINT('Ctrl Pts',(8.45006291411674E-15,36.25,46.));
#16531=CARTESIAN_POINT('Ctrl Pts',(-12.3256628518316,36.0416666666667,46.));
#16532=CARTESIAN_POINT('Ctrl Pts',(-23.,35.8333333333333,39.8371685740842));
#16533=CARTESIAN_POINT('Ctrl Pts',(-33.6743371481683,35.625,33.6743371481684));
#16534=CARTESIAN_POINT('Ctrl Pts',(-39.8371685740842,35.4166666666667,23.));
#16535=CARTESIAN_POINT('Ctrl Pts',(-46.,35.2083333333333,12.3256628518317));
#16536=CARTESIAN_POINT('Ctrl Pts',(-46.,35.,0.));
#16537=CARTESIAN_POINT('Ctrl Pts',(-46.,34.7916666666667,-12.3256628518316));
#16538=CARTESIAN_POINT('Ctrl Pts',(-39.8371685740842,34.5833333333333,-23.));
#16539=CARTESIAN_POINT('Ctrl Pts',(-33.6743371481684,34.375,-33.6743371481684));
#16540=CARTESIAN_POINT('Ctrl Pts',(-23.,34.1666666666667,-39.8371685740842));
#16541=CARTESIAN_POINT('Ctrl Pts',(-12.3256628518317,33.9583333333333,-46.));
#16542=CARTESIAN_POINT('Ctrl Pts',(-2.81668763803891E-15,33.75,-46.));
#16543=CARTESIAN_POINT('Ctrl Pts',(12.3256628518316,33.5416666666667,-46.));
#16544=CARTESIAN_POINT('Ctrl Pts',(23.,33.3333333333333,-39.8371685740842));
#16545=CARTESIAN_POINT('Ctrl Pts',(33.6743371481683,33.125,-33.6743371481684));
#16546=CARTESIAN_POINT('Ctrl Pts',(39.8371685740842,32.9166666666667,-23.));
#16547=CARTESIAN_POINT('Ctrl Pts',(46.,32.7083333333333,-12.3256628518317));
#16548=CARTESIAN_POINT('Ctrl Pts',(46.,32.5,-5.63337527607782E-15));
#16549=CARTESIAN_POINT('Ctrl Pts',(46.,32.2916666666667,12.3256628518316));
#16550=CARTESIAN_POINT('Ctrl Pts',(39.8371685740842,32.0833333333333,23.));
#16551=CARTESIAN_POINT('Ctrl Pts',(33.6743371481684,31.875,33.6743371481683));
#16552=CARTESIAN_POINT('Ctrl Pts',(23.,31.6666666666667,39.8371685740842));
#16553=CARTESIAN_POINT('Ctrl Pts',(12.3256628518317,31.4583333333333,46.));
#16554=CARTESIAN_POINT('Ctrl Pts',(8.45006291411674E-15,31.25,46.));
#16555=CARTESIAN_POINT('Ctrl Pts',(-12.3256628518316,31.0416666666667,46.));
#16556=CARTESIAN_POINT('Ctrl Pts',(-23.,30.8333333333333,39.8371685740842));
#16557=CARTESIAN_POINT('Ctrl Pts',(-33.6743371481683,30.625,33.6743371481684));
#16558=CARTESIAN_POINT('Ctrl Pts',(-39.8371685740842,30.4166666666667,23.));
#16559=CARTESIAN_POINT('Ctrl Pts',(-46.,30.2083333333333,12.3256628518317));
#16560=CARTESIAN_POINT('Ctrl Pts',(-46.,30.,0.));
#16561=CARTESIAN_POINT('Ctrl Pts',(45.7957082162897,37.5741208584476,-4.33048599679664));
#16562=CARTESIAN_POINT('Ctrl Pts',(46.027322302781,37.4406160752063,-4.33048599679664));
#16563=CARTESIAN_POINT('Ctrl Pts',(46.4905476657728,37.1736016336912,-4.33048599679679));
#16564=CARTESIAN_POINT('Ctrl Pts',(46.9537676533565,36.9065778670208,-4.33048599679665));
#16565=CARTESIAN_POINT('Ctrl Pts',(47.6280672732221,36.5178683162597,-4.33048599679665));
#16566=CARTESIAN_POINT('Ctrl Pts',(48.0707534890442,36.2626647328764,-4.33048599679682));
#16567=CARTESIAN_POINT('Ctrl Pts',(48.5134353784344,36.0074536451604,-4.33048599679682));
#16568=CARTESIAN_POINT('Ctrl Pts',(3.61292728433801,37.1292520480092,-48.5721450795008));
#16569=CARTESIAN_POINT('Ctrl Pts',(3.61292728433801,37.2624339185675,-48.3403451622817));
#16570=CARTESIAN_POINT('Ctrl Pts',(3.61292728433802,37.395608829009,-48.1085412459393));
#16571=CARTESIAN_POINT('Ctrl Pts',(3.61292728433802,37.6619441142016,-47.6449250631479));
#16572=CARTESIAN_POINT('Ctrl Pts',(3.61292728433795,37.7951044891727,-47.4131127965212));
#16573=CARTESIAN_POINT('Ctrl Pts',(3.61292728433795,37.9282572703914,-47.1812961682826));
#16574=CARTESIAN_POINT('Ctrl Pts',(3.61292728433795,38.1816295626638,-46.7401795055578));
#16575=CARTESIAN_POINT('Ctrl Pts',(3.61292728433797,38.4349743764897,-46.2990470581854));
#16576=CARTESIAN_POINT('Ctrl Pts',(3.61292728433797,38.688289262853,-45.8578974271399));
#16577=CARTESIAN_POINT('Ctrl Pts',(-48.706329375,58.437500006828,-1.8898197019151E-14));
#16578=CARTESIAN_POINT('Ctrl Pts',(-48.706329375,58.2291666734946,-13.0508216223155));
#16579=CARTESIAN_POINT('Ctrl Pts',(-42.1809185638422,58.0208333401613,-24.3531646875));
#16580=CARTESIAN_POINT('Ctrl Pts',(-35.6555077526845,57.812500006828,-35.6555077526845));
#16581=CARTESIAN_POINT('Ctrl Pts',(-24.3531646875,57.6041666734946,-42.1809185638422));
#16582=CARTESIAN_POINT('Ctrl Pts',(-13.0508216223155,57.3958333401613,-48.706329375));
#16583=CARTESIAN_POINT('Ctrl Pts',(1.59157945007855E-14,57.187500006828,
-48.706329375));
#16584=CARTESIAN_POINT('Ctrl Pts',(13.0508216223155,56.9791666734946,-48.706329375));
#16585=CARTESIAN_POINT('Ctrl Pts',(24.3531646875,56.7708333401613,-42.1809185638422));
#16586=CARTESIAN_POINT('Ctrl Pts',(35.6555077526845,56.562500006828,-35.6555077526845));
#16587=CARTESIAN_POINT('Ctrl Pts',(42.1809185638422,56.3541666734946,-24.3531646875));
#16588=CARTESIAN_POINT('Ctrl Pts',(48.706329375,56.1458333401613,-13.0508216223155));
#16589=CARTESIAN_POINT('Ctrl Pts',(48.706329375,55.937500006828,1.293339198242E-14));
#16590=CARTESIAN_POINT('Ctrl Pts',(48.706329375,55.7291666734946,13.0508216223155));
#16591=CARTESIAN_POINT('Ctrl Pts',(42.1809185638422,55.5208333401613,24.3531646875));
#16592=CARTESIAN_POINT('Ctrl Pts',(35.6555077526845,55.312500006828,35.6555077526845));
#16593=CARTESIAN_POINT('Ctrl Pts',(24.3531646875,55.1041666734946,42.1809185638422));
#16594=CARTESIAN_POINT('Ctrl Pts',(13.0508216223155,54.8958333401613,48.706329375));
#16595=CARTESIAN_POINT('Ctrl Pts',(-9.95098946405443E-15,54.687500006828,
48.706329375));
#16596=CARTESIAN_POINT('Ctrl Pts',(-13.0508216223155,54.4791666734946,48.706329375));
#16597=CARTESIAN_POINT('Ctrl Pts',(-24.3531646875,54.2708333401613,42.1809185638423));
#16598=CARTESIAN_POINT('Ctrl Pts',(-35.6555077526845,54.062500006828,35.6555077526845));
#16599=CARTESIAN_POINT('Ctrl Pts',(-42.1809185638422,53.8541666734946,24.3531646875));
#16600=CARTESIAN_POINT('Ctrl Pts',(-48.706329375,53.6458333401613,13.0508216223155));
#16601=CARTESIAN_POINT('Ctrl Pts',(-48.706329375,53.437500006828,-1.8898197019151E-14));
#16602=CARTESIAN_POINT('Ctrl Pts',(-48.706329375,53.2291666734946,-13.0508216223155));
#16603=CARTESIAN_POINT('Ctrl Pts',(-42.1809185638422,53.0208333401613,-24.3531646875));
#16604=CARTESIAN_POINT('Ctrl Pts',(-35.6555077526845,52.812500006828,-35.6555077526845));
#16605=CARTESIAN_POINT('Ctrl Pts',(-24.3531646875,52.6041666734946,-42.1809185638422));
#16606=CARTESIAN_POINT('Ctrl Pts',(-13.0508216223155,52.3958333401613,-48.706329375));
#16607=CARTESIAN_POINT('Ctrl Pts',(1.59157945007855E-14,52.187500006828,
-48.706329375));
#16608=CARTESIAN_POINT('Ctrl Pts',(13.0508216223155,51.9791666734946,-48.706329375));
#16609=CARTESIAN_POINT('Ctrl Pts',(24.3531646875,51.7708333401613,-42.1809185638422));
#16610=CARTESIAN_POINT('Ctrl Pts',(35.6555077526845,51.562500006828,-35.6555077526845));
#16611=CARTESIAN_POINT('Ctrl Pts',(42.1809185638422,51.3541666734946,-24.3531646875));
#16612=CARTESIAN_POINT('Ctrl Pts',(48.706329375,51.1458333401613,-13.0508216223155));
#16613=CARTESIAN_POINT('Ctrl Pts',(48.706329375,50.937500006828,1.293339198242E-14));
#16614=CARTESIAN_POINT('Ctrl Pts',(48.706329375,50.7291666734946,13.0508216223155));
#16615=CARTESIAN_POINT('Ctrl Pts',(42.1809185638422,50.5208333401613,24.3531646875));
#16616=CARTESIAN_POINT('Ctrl Pts',(35.6555077526845,50.312500006828,35.6555077526845));
#16617=CARTESIAN_POINT('Ctrl Pts',(24.3531646875,50.1041666734946,42.1809185638422));
#16618=CARTESIAN_POINT('Ctrl Pts',(13.0508216223155,49.8958333401613,48.706329375));
#16619=CARTESIAN_POINT('Ctrl Pts',(-9.95098946405443E-15,49.687500006828,
48.706329375));
#16620=CARTESIAN_POINT('Ctrl Pts',(-13.0508216223155,49.4791666734946,48.706329375));
#16621=CARTESIAN_POINT('Ctrl Pts',(-24.3531646875,49.2708333401613,42.1809185638423));
#16622=CARTESIAN_POINT('Ctrl Pts',(-35.6555077526845,49.062500006828,35.6555077526845));
#16623=CARTESIAN_POINT('Ctrl Pts',(-42.1809185638422,48.8541666734946,24.3531646875));
#16624=CARTESIAN_POINT('Ctrl Pts',(-48.706329375,48.6458333401613,13.0508216223155));
#16625=CARTESIAN_POINT('Ctrl Pts',(-48.706329375,48.437500006828,-1.8898197019151E-14));
#16626=CARTESIAN_POINT('Ctrl Pts',(-48.706329375,48.2291666734946,-13.0508216223155));
#16627=CARTESIAN_POINT('Ctrl Pts',(-42.1809185638422,48.0208333401613,-24.3531646875));
#16628=CARTESIAN_POINT('Ctrl Pts',(-35.6555077526845,47.812500006828,-35.6555077526845));
#16629=CARTESIAN_POINT('Ctrl Pts',(-24.3531646875,47.6041666734946,-42.1809185638422));
#16630=CARTESIAN_POINT('Ctrl Pts',(-13.0508216223155,47.3958333401613,-48.706329375));
#16631=CARTESIAN_POINT('Ctrl Pts',(1.59157945007855E-14,47.187500006828,
-48.706329375));
#16632=CARTESIAN_POINT('Ctrl Pts',(13.0508216223155,46.9791666734946,-48.706329375));
#16633=CARTESIAN_POINT('Ctrl Pts',(24.3531646875,46.7708333401613,-42.1809185638422));
#16634=CARTESIAN_POINT('Ctrl Pts',(35.6555077526845,46.562500006828,-35.6555077526845));
#16635=CARTESIAN_POINT('Ctrl Pts',(42.1809185638422,46.3541666734946,-24.3531646875));
#16636=CARTESIAN_POINT('Ctrl Pts',(48.706329375,46.1458333401613,-13.0508216223155));
#16637=CARTESIAN_POINT('Ctrl Pts',(48.706329375,45.937500006828,1.293339198242E-14));
#16638=CARTESIAN_POINT('Ctrl Pts',(48.706329375,45.7291666734946,13.0508216223155));
#16639=CARTESIAN_POINT('Ctrl Pts',(42.1809185638422,45.5208333401613,24.3531646875));
#16640=CARTESIAN_POINT('Ctrl Pts',(35.6555077526845,45.312500006828,35.6555077526845));
#16641=CARTESIAN_POINT('Ctrl Pts',(24.3531646875,45.1041666734946,42.1809185638422));
#16642=CARTESIAN_POINT('Ctrl Pts',(13.0508216223155,44.8958333401613,48.706329375));
#16643=CARTESIAN_POINT('Ctrl Pts',(-9.95098946405443E-15,44.687500006828,
48.706329375));
#16644=CARTESIAN_POINT('Ctrl Pts',(-13.0508216223155,44.4791666734946,48.706329375));
#16645=CARTESIAN_POINT('Ctrl Pts',(-24.3531646875,44.2708333401613,42.1809185638423));
#16646=CARTESIAN_POINT('Ctrl Pts',(-35.6555077526845,44.062500006828,35.6555077526845));
#16647=CARTESIAN_POINT('Ctrl Pts',(-42.1809185638422,43.8541666734946,24.3531646875));
#16648=CARTESIAN_POINT('Ctrl Pts',(-48.706329375,43.6458333401613,13.0508216223155));
#16649=CARTESIAN_POINT('Ctrl Pts',(-48.706329375,43.437500006828,-1.8898197019151E-14));
#16650=CARTESIAN_POINT('Ctrl Pts',(-48.706329375,43.2291666734946,-13.0508216223155));
#16651=CARTESIAN_POINT('Ctrl Pts',(-42.1809185638422,43.0208333401613,-24.3531646875));
#16652=CARTESIAN_POINT('Ctrl Pts',(-35.6555077526845,42.812500006828,-35.6555077526845));
#16653=CARTESIAN_POINT('Ctrl Pts',(-24.3531646875,42.6041666734946,-42.1809185638422));
#16654=CARTESIAN_POINT('Ctrl Pts',(-13.0508216223155,42.3958333401613,-48.706329375));
#16655=CARTESIAN_POINT('Ctrl Pts',(1.59157945007855E-14,42.187500006828,
-48.706329375));
#16656=CARTESIAN_POINT('Ctrl Pts',(13.0508216223155,41.9791666734946,-48.706329375));
#16657=CARTESIAN_POINT('Ctrl Pts',(24.3531646875,41.7708333401613,-42.1809185638422));
#16658=CARTESIAN_POINT('Ctrl Pts',(35.6555077526845,41.562500006828,-35.6555077526845));
#16659=CARTESIAN_POINT('Ctrl Pts',(42.1809185638422,41.3541666734946,-24.3531646875));
#16660=CARTESIAN_POINT('Ctrl Pts',(48.706329375,41.1458333401613,-13.0508216223155));
#16661=CARTESIAN_POINT('Ctrl Pts',(48.706329375,40.937500006828,1.293339198242E-14));
#16662=CARTESIAN_POINT('Ctrl Pts',(48.706329375,40.7291666734946,13.0508216223155));
#16663=CARTESIAN_POINT('Ctrl Pts',(42.1809185638422,40.5208333401613,24.3531646875));
#16664=CARTESIAN_POINT('Ctrl Pts',(35.6555077526845,40.312500006828,35.6555077526845));
#16665=CARTESIAN_POINT('Ctrl Pts',(24.3531646875,40.1041666734946,42.1809185638422));
#16666=CARTESIAN_POINT('Ctrl Pts',(13.0508216223155,39.8958333401613,48.706329375));
#16667=CARTESIAN_POINT('Ctrl Pts',(-9.95098946405443E-15,39.687500006828,
48.706329375));
#16668=CARTESIAN_POINT('Ctrl Pts',(-13.0508216223155,39.4791666734946,48.706329375));
#16669=CARTESIAN_POINT('Ctrl Pts',(-24.3531646875,39.2708333401613,42.1809185638423));
#16670=CARTESIAN_POINT('Ctrl Pts',(-35.6555077526845,39.062500006828,35.6555077526845));
#16671=CARTESIAN_POINT('Ctrl Pts',(-42.1809185638422,38.8541666734946,24.3531646875));
#16672=CARTESIAN_POINT('Ctrl Pts',(-48.706329375,38.6458333401613,13.0508216223155));
#16673=CARTESIAN_POINT('Ctrl Pts',(-48.706329375,38.437500006828,-1.8898197019151E-14));
#16674=CARTESIAN_POINT('Ctrl Pts',(-48.706329375,38.2291666734946,-13.0508216223155));
#16675=CARTESIAN_POINT('Ctrl Pts',(-42.1809185638422,38.0208333401613,-24.3531646875));
#16676=CARTESIAN_POINT('Ctrl Pts',(-35.6555077526845,37.812500006828,-35.6555077526845));
#16677=CARTESIAN_POINT('Ctrl Pts',(-24.3531646875,37.6041666734946,-42.1809185638422));
#16678=CARTESIAN_POINT('Ctrl Pts',(-13.0508216223155,37.3958333401613,-48.706329375));
#16679=CARTESIAN_POINT('Ctrl Pts',(1.59157945007855E-14,37.187500006828,
-48.706329375));
#16680=CARTESIAN_POINT('Ctrl Pts',(13.0508216223155,36.9791666734946,-48.706329375));
#16681=CARTESIAN_POINT('Ctrl Pts',(24.3531646875,36.7708333401613,-42.1809185638422));
#16682=CARTESIAN_POINT('Ctrl Pts',(35.6555077526845,36.562500006828,-35.6555077526845));
#16683=CARTESIAN_POINT('Ctrl Pts',(42.1809185638422,36.3541666734946,-24.3531646875));
#16684=CARTESIAN_POINT('Ctrl Pts',(48.706329375,36.1458333401613,-13.0508216223155));
#16685=CARTESIAN_POINT('Ctrl Pts',(48.706329375,35.937500006828,1.293339198242E-14));
#16686=CARTESIAN_POINT('Ctrl Pts',(48.706329375,35.7291666734946,13.0508216223155));
#16687=CARTESIAN_POINT('Ctrl Pts',(42.1809185638422,35.5208333401613,24.3531646875));
#16688=CARTESIAN_POINT('Ctrl Pts',(35.6555077526845,35.312500006828,35.6555077526845));
#16689=CARTESIAN_POINT('Ctrl Pts',(24.3531646875,35.1041666734946,42.1809185638422));
#16690=CARTESIAN_POINT('Ctrl Pts',(13.0508216223155,34.8958333401613,48.706329375));
#16691=CARTESIAN_POINT('Ctrl Pts',(-9.95098946405443E-15,34.687500006828,
48.706329375));
#16692=CARTESIAN_POINT('Ctrl Pts',(-13.0508216223155,34.4791666734946,48.706329375));
#16693=CARTESIAN_POINT('Ctrl Pts',(-24.3531646875,34.2708333401613,42.1809185638423));
#16694=CARTESIAN_POINT('Ctrl Pts',(-35.6555077526845,34.062500006828,35.6555077526845));
#16695=CARTESIAN_POINT('Ctrl Pts',(-42.1809185638422,33.8541666734946,24.3531646875));
#16696=CARTESIAN_POINT('Ctrl Pts',(-48.706329375,33.6458333401613,13.0508216223155));
#16697=CARTESIAN_POINT('Ctrl Pts',(-48.706329375,33.437500006828,-1.8898197019151E-14));
#16698=CARTESIAN_POINT('Ctrl Pts',(-48.706329375,33.2291666734946,-13.0508216223155));
#16699=CARTESIAN_POINT('Ctrl Pts',(-42.1809185638422,33.0208333401613,-24.3531646875));
#16700=CARTESIAN_POINT('Ctrl Pts',(-35.6555077526845,32.812500006828,-35.6555077526845));
#16701=CARTESIAN_POINT('Ctrl Pts',(-24.3531646875,32.6041666734946,-42.1809185638422));
#16702=CARTESIAN_POINT('Ctrl Pts',(-13.0508216223155,32.3958333401613,-48.706329375));
#16703=CARTESIAN_POINT('Ctrl Pts',(1.59157945007855E-14,32.187500006828,
-48.706329375));
#16704=CARTESIAN_POINT('Ctrl Pts',(13.0508216223155,31.9791666734946,-48.706329375));
#16705=CARTESIAN_POINT('Ctrl Pts',(24.3531646875,31.7708333401613,-42.1809185638422));
#16706=CARTESIAN_POINT('Ctrl Pts',(35.6555077526845,31.562500006828,-35.6555077526845));
#16707=CARTESIAN_POINT('Ctrl Pts',(42.1809185638422,31.3541666734946,-24.3531646875));
#16708=CARTESIAN_POINT('Ctrl Pts',(48.706329375,31.1458333401613,-13.0508216223155));
#16709=CARTESIAN_POINT('Ctrl Pts',(48.706329375,30.937500006828,1.293339198242E-14));
#16710=CARTESIAN_POINT('Ctrl Pts',(48.706329375,30.7291666734946,13.0508216223155));
#16711=CARTESIAN_POINT('Ctrl Pts',(42.1809185638422,30.5208333401613,24.3531646875));
#16712=CARTESIAN_POINT('Ctrl Pts',(35.6555077526845,30.312500006828,35.6555077526845));
#16713=CARTESIAN_POINT('Ctrl Pts',(24.3531646875,30.1041666734946,42.1809185638422));
#16714=CARTESIAN_POINT('Ctrl Pts',(13.0508216223155,29.8958333401613,48.706329375));
#16715=CARTESIAN_POINT('Ctrl Pts',(-9.95098946405443E-15,29.687500006828,
48.706329375));
#16716=CARTESIAN_POINT('Ctrl Pts',(-13.0508216223155,29.4791666734946,48.706329375));
#16717=CARTESIAN_POINT('Ctrl Pts',(-24.3531646875,29.2708333401613,42.1809185638423));
#16718=CARTESIAN_POINT('Ctrl Pts',(-35.6555077526845,29.062500006828,35.6555077526845));
#16719=CARTESIAN_POINT('Ctrl Pts',(-42.1809185638422,28.8541666734946,24.3531646875));
#16720=CARTESIAN_POINT('Ctrl Pts',(-48.706329375,28.6458333401613,13.0508216223155));
#16721=CARTESIAN_POINT('Ctrl Pts',(-48.706329375,28.437500006828,-1.8898197019151E-14));
#16722=CARTESIAN_POINT('Ctrl Pts',(-46.,60.,0.));
#16723=CARTESIAN_POINT('Ctrl Pts',(-46.,59.7916666666667,-12.3256628518316));
#16724=CARTESIAN_POINT('Ctrl Pts',(-39.8371685740842,59.5833333333333,-23.));
#16725=CARTESIAN_POINT('Ctrl Pts',(-33.6743371481684,59.375,-33.6743371481684));
#16726=CARTESIAN_POINT('Ctrl Pts',(-23.,59.1666666666667,-39.8371685740842));
#16727=CARTESIAN_POINT('Ctrl Pts',(-12.3256628518317,58.9583333333333,-46.));
#16728=CARTESIAN_POINT('Ctrl Pts',(-2.81668763803891E-15,58.75,-46.));
#16729=CARTESIAN_POINT('Ctrl Pts',(12.3256628518316,58.5416666666667,-46.));
#16730=CARTESIAN_POINT('Ctrl Pts',(23.,58.3333333333333,-39.8371685740842));
#16731=CARTESIAN_POINT('Ctrl Pts',(33.6743371481683,58.125,-33.6743371481684));
#16732=CARTESIAN_POINT('Ctrl Pts',(39.8371685740842,57.9166666666667,-23.));
#16733=CARTESIAN_POINT('Ctrl Pts',(46.,57.7083333333333,-12.3256628518317));
#16734=CARTESIAN_POINT('Ctrl Pts',(46.,57.5,-5.63337527607782E-15));
#16735=CARTESIAN_POINT('Ctrl Pts',(46.,57.2916666666667,12.3256628518316));
#16736=CARTESIAN_POINT('Ctrl Pts',(39.8371685740842,57.0833333333333,23.));
#16737=CARTESIAN_POINT('Ctrl Pts',(33.6743371481684,56.875,33.6743371481683));
#16738=CARTESIAN_POINT('Ctrl Pts',(23.,56.6666666666667,39.8371685740842));
#16739=CARTESIAN_POINT('Ctrl Pts',(12.3256628518317,56.4583333333333,46.));
#16740=CARTESIAN_POINT('Ctrl Pts',(8.45006291411674E-15,56.25,46.));
#16741=CARTESIAN_POINT('Ctrl Pts',(-12.3256628518316,56.0416666666667,46.));
#16742=CARTESIAN_POINT('Ctrl Pts',(-23.,55.8333333333333,39.8371685740842));
#16743=CARTESIAN_POINT('Ctrl Pts',(-33.6743371481683,55.625,33.6743371481684));
#16744=CARTESIAN_POINT('Ctrl Pts',(-39.8371685740842,55.4166666666667,23.));
#16745=CARTESIAN_POINT('Ctrl Pts',(-46.,55.2083333333333,12.3256628518317));
#16746=CARTESIAN_POINT('Ctrl Pts',(-46.,55.,0.));
#16747=CARTESIAN_POINT('Ctrl Pts',(-46.,54.7916666666667,-12.3256628518316));
#16748=CARTESIAN_POINT('Ctrl Pts',(-39.8371685740842,54.5833333333333,-23.));
#16749=CARTESIAN_POINT('Ctrl Pts',(-33.6743371481684,54.375,-33.6743371481684));
#16750=CARTESIAN_POINT('Ctrl Pts',(-23.,54.1666666666667,-39.8371685740842));
#16751=CARTESIAN_POINT('Ctrl Pts',(-12.3256628518317,53.9583333333333,-46.));
#16752=CARTESIAN_POINT('Ctrl Pts',(-2.81668763803891E-15,53.75,-46.));
#16753=CARTESIAN_POINT('Ctrl Pts',(12.3256628518316,53.5416666666667,-46.));
#16754=CARTESIAN_POINT('Ctrl Pts',(23.,53.3333333333333,-39.8371685740842));
#16755=CARTESIAN_POINT('Ctrl Pts',(33.6743371481683,53.125,-33.6743371481684));
#16756=CARTESIAN_POINT('Ctrl Pts',(39.8371685740842,52.9166666666667,-23.));
#16757=CARTESIAN_POINT('Ctrl Pts',(46.,52.7083333333333,-12.3256628518317));
#16758=CARTESIAN_POINT('Ctrl Pts',(46.,52.5,-5.63337527607782E-15));
#16759=CARTESIAN_POINT('Ctrl Pts',(46.,52.2916666666667,12.3256628518316));
#16760=CARTESIAN_POINT('Ctrl Pts',(39.8371685740842,52.0833333333333,23.));
#16761=CARTESIAN_POINT('Ctrl Pts',(33.6743371481684,51.875,33.6743371481683));
#16762=CARTESIAN_POINT('Ctrl Pts',(23.,51.6666666666667,39.8371685740842));
#16763=CARTESIAN_POINT('Ctrl Pts',(12.3256628518317,51.4583333333333,46.));
#16764=CARTESIAN_POINT('Ctrl Pts',(8.45006291411674E-15,51.25,46.));
#16765=CARTESIAN_POINT('Ctrl Pts',(-12.3256628518316,51.0416666666667,46.));
#16766=CARTESIAN_POINT('Ctrl Pts',(-23.,50.8333333333333,39.8371685740842));
#16767=CARTESIAN_POINT('Ctrl Pts',(-33.6743371481683,50.625,33.6743371481684));
#16768=CARTESIAN_POINT('Ctrl Pts',(-39.8371685740842,50.4166666666667,23.));
#16769=CARTESIAN_POINT('Ctrl Pts',(-46.,50.2083333333333,12.3256628518317));
#16770=CARTESIAN_POINT('Ctrl Pts',(-46.,50.,0.));
#16771=CARTESIAN_POINT('Ctrl Pts',(-46.,49.7916666666667,-12.3256628518316));
#16772=CARTESIAN_POINT('Ctrl Pts',(-39.8371685740842,49.5833333333333,-23.));
#16773=CARTESIAN_POINT('Ctrl Pts',(-33.6743371481684,49.375,-33.6743371481684));
#16774=CARTESIAN_POINT('Ctrl Pts',(-23.,49.1666666666667,-39.8371685740842));
#16775=CARTESIAN_POINT('Ctrl Pts',(-12.3256628518317,48.9583333333333,-46.));
#16776=CARTESIAN_POINT('Ctrl Pts',(-2.81668763803891E-15,48.75,-46.));
#16777=CARTESIAN_POINT('Ctrl Pts',(12.3256628518316,48.5416666666667,-46.));
#16778=CARTESIAN_POINT('Ctrl Pts',(23.,48.3333333333333,-39.8371685740842));
#16779=CARTESIAN_POINT('Ctrl Pts',(33.6743371481683,48.125,-33.6743371481684));
#16780=CARTESIAN_POINT('Ctrl Pts',(39.8371685740842,47.9166666666667,-23.));
#16781=CARTESIAN_POINT('Ctrl Pts',(46.,47.7083333333333,-12.3256628518317));
#16782=CARTESIAN_POINT('Ctrl Pts',(46.,47.5,-5.63337527607782E-15));
#16783=CARTESIAN_POINT('Ctrl Pts',(46.,47.2916666666667,12.3256628518316));
#16784=CARTESIAN_POINT('Ctrl Pts',(39.8371685740842,47.0833333333333,23.));
#16785=CARTESIAN_POINT('Ctrl Pts',(33.6743371481684,46.875,33.6743371481683));
#16786=CARTESIAN_POINT('Ctrl Pts',(23.,46.6666666666667,39.8371685740842));
#16787=CARTESIAN_POINT('Ctrl Pts',(12.3256628518317,46.4583333333333,46.));
#16788=CARTESIAN_POINT('Ctrl Pts',(8.45006291411674E-15,46.25,46.));
#16789=CARTESIAN_POINT('Ctrl Pts',(-12.3256628518316,46.0416666666667,46.));
#16790=CARTESIAN_POINT('Ctrl Pts',(-23.,45.8333333333333,39.8371685740842));
#16791=CARTESIAN_POINT('Ctrl Pts',(-33.6743371481683,45.625,33.6743371481684));
#16792=CARTESIAN_POINT('Ctrl Pts',(-39.8371685740842,45.4166666666667,23.));
#16793=CARTESIAN_POINT('Ctrl Pts',(-46.,45.2083333333333,12.3256628518317));
#16794=CARTESIAN_POINT('Ctrl Pts',(-46.,45.,0.));
#16795=CARTESIAN_POINT('Ctrl Pts',(-46.,44.7916666666667,-12.3256628518316));
#16796=CARTESIAN_POINT('Ctrl Pts',(-39.8371685740842,44.5833333333333,-23.));
#16797=CARTESIAN_POINT('Ctrl Pts',(-33.6743371481684,44.375,-33.6743371481684));
#16798=CARTESIAN_POINT('Ctrl Pts',(-23.,44.1666666666667,-39.8371685740842));
#16799=CARTESIAN_POINT('Ctrl Pts',(-12.3256628518317,43.9583333333333,-46.));
#16800=CARTESIAN_POINT('Ctrl Pts',(-2.81668763803891E-15,43.75,-46.));
#16801=CARTESIAN_POINT('Ctrl Pts',(12.3256628518316,43.5416666666667,-46.));
#16802=CARTESIAN_POINT('Ctrl Pts',(23.,43.3333333333333,-39.8371685740842));
#16803=CARTESIAN_POINT('Ctrl Pts',(33.6743371481683,43.125,-33.6743371481684));
#16804=CARTESIAN_POINT('Ctrl Pts',(39.8371685740842,42.9166666666667,-23.));
#16805=CARTESIAN_POINT('Ctrl Pts',(46.,42.7083333333333,-12.3256628518317));
#16806=CARTESIAN_POINT('Ctrl Pts',(46.,42.5,-5.63337527607782E-15));
#16807=CARTESIAN_POINT('Ctrl Pts',(46.,42.2916666666667,12.3256628518316));
#16808=CARTESIAN_POINT('Ctrl Pts',(39.8371685740842,42.0833333333333,23.));
#16809=CARTESIAN_POINT('Ctrl Pts',(33.6743371481684,41.875,33.6743371481683));
#16810=CARTESIAN_POINT('Ctrl Pts',(23.,41.6666666666667,39.8371685740842));
#16811=CARTESIAN_POINT('Ctrl Pts',(12.3256628518317,41.4583333333333,46.));
#16812=CARTESIAN_POINT('Ctrl Pts',(8.45006291411674E-15,41.25,46.));
#16813=CARTESIAN_POINT('Ctrl Pts',(-12.3256628518316,41.0416666666667,46.));
#16814=CARTESIAN_POINT('Ctrl Pts',(-23.,40.8333333333333,39.8371685740842));
#16815=CARTESIAN_POINT('Ctrl Pts',(-33.6743371481683,40.625,33.6743371481684));
#16816=CARTESIAN_POINT('Ctrl Pts',(-39.8371685740842,40.4166666666667,23.));
#16817=CARTESIAN_POINT('Ctrl Pts',(-46.,40.2083333333333,12.3256628518317));
#16818=CARTESIAN_POINT('Ctrl Pts',(-46.,40.,0.));
#16819=CARTESIAN_POINT('Ctrl Pts',(-46.,39.7916666666667,-12.3256628518316));
#16820=CARTESIAN_POINT('Ctrl Pts',(-39.8371685740842,39.5833333333333,-23.));
#16821=CARTESIAN_POINT('Ctrl Pts',(-33.6743371481684,39.375,-33.6743371481684));
#16822=CARTESIAN_POINT('Ctrl Pts',(-23.,39.1666666666667,-39.8371685740842));
#16823=CARTESIAN_POINT('Ctrl Pts',(-12.3256628518317,38.9583333333333,-46.));
#16824=CARTESIAN_POINT('Ctrl Pts',(-2.81668763803891E-15,38.75,-46.));
#16825=CARTESIAN_POINT('Ctrl Pts',(12.3256628518316,38.5416666666667,-46.));
#16826=CARTESIAN_POINT('Ctrl Pts',(23.,38.3333333333333,-39.8371685740842));
#16827=CARTESIAN_POINT('Ctrl Pts',(33.6743371481683,38.125,-33.6743371481684));
#16828=CARTESIAN_POINT('Ctrl Pts',(39.8371685740842,37.9166666666667,-23.));
#16829=CARTESIAN_POINT('Ctrl Pts',(46.,37.7083333333333,-12.3256628518317));
#16830=CARTESIAN_POINT('Ctrl Pts',(46.,37.5,-5.63337527607782E-15));
#16831=CARTESIAN_POINT('Ctrl Pts',(46.,37.2916666666667,12.3256628518316));
#16832=CARTESIAN_POINT('Ctrl Pts',(39.8371685740842,37.0833333333333,23.));
#16833=CARTESIAN_POINT('Ctrl Pts',(33.6743371481684,36.875,33.6743371481683));
#16834=CARTESIAN_POINT('Ctrl Pts',(23.,36.6666666666667,39.8371685740842));
#16835=CARTESIAN_POINT('Ctrl Pts',(12.3256628518317,36.4583333333333,46.));
#16836=CARTESIAN_POINT('Ctrl Pts',(8.45006291411674E-15,36.25,46.));
#16837=CARTESIAN_POINT('Ctrl Pts',(-12.3256628518316,36.0416666666667,46.));
#16838=CARTESIAN_POINT('Ctrl Pts',(-23.,35.8333333333333,39.8371685740842));
#16839=CARTESIAN_POINT('Ctrl Pts',(-33.6743371481683,35.625,33.6743371481684));
#16840=CARTESIAN_POINT('Ctrl Pts',(-39.8371685740842,35.4166666666667,23.));
#16841=CARTESIAN_POINT('Ctrl Pts',(-46.,35.2083333333333,12.3256628518317));
#16842=CARTESIAN_POINT('Ctrl Pts',(-46.,35.,0.));
#16843=CARTESIAN_POINT('Ctrl Pts',(-46.,34.7916666666667,-12.3256628518316));
#16844=CARTESIAN_POINT('Ctrl Pts',(-39.8371685740842,34.5833333333333,-23.));
#16845=CARTESIAN_POINT('Ctrl Pts',(-33.6743371481684,34.375,-33.6743371481684));
#16846=CARTESIAN_POINT('Ctrl Pts',(-23.,34.1666666666667,-39.8371685740842));
#16847=CARTESIAN_POINT('Ctrl Pts',(-12.3256628518317,33.9583333333333,-46.));
#16848=CARTESIAN_POINT('Ctrl Pts',(-2.81668763803891E-15,33.75,-46.));
#16849=CARTESIAN_POINT('Ctrl Pts',(12.3256628518316,33.5416666666667,-46.));
#16850=CARTESIAN_POINT('Ctrl Pts',(23.,33.3333333333333,-39.8371685740842));
#16851=CARTESIAN_POINT('Ctrl Pts',(33.6743371481683,33.125,-33.6743371481684));
#16852=CARTESIAN_POINT('Ctrl Pts',(39.8371685740842,32.9166666666667,-23.));
#16853=CARTESIAN_POINT('Ctrl Pts',(46.,32.7083333333333,-12.3256628518317));
#16854=CARTESIAN_POINT('Ctrl Pts',(46.,32.5,-5.63337527607782E-15));
#16855=CARTESIAN_POINT('Ctrl Pts',(46.,32.2916666666667,12.3256628518316));
#16856=CARTESIAN_POINT('Ctrl Pts',(39.8371685740842,32.0833333333333,23.));
#16857=CARTESIAN_POINT('Ctrl Pts',(33.6743371481684,31.875,33.6743371481683));
#16858=CARTESIAN_POINT('Ctrl Pts',(23.,31.6666666666667,39.8371685740842));
#16859=CARTESIAN_POINT('Ctrl Pts',(12.3256628518317,31.4583333333333,46.));
#16860=CARTESIAN_POINT('Ctrl Pts',(8.45006291411674E-15,31.25,46.));
#16861=CARTESIAN_POINT('Ctrl Pts',(-12.3256628518316,31.0416666666667,46.));
#16862=CARTESIAN_POINT('Ctrl Pts',(-23.,30.8333333333333,39.8371685740842));
#16863=CARTESIAN_POINT('Ctrl Pts',(-33.6743371481683,30.625,33.6743371481684));
#16864=CARTESIAN_POINT('Ctrl Pts',(-39.8371685740842,30.4166666666667,23.));
#16865=CARTESIAN_POINT('Ctrl Pts',(-46.,30.2083333333333,12.3256628518317));
#16866=CARTESIAN_POINT('Ctrl Pts',(-46.,30.,0.));
#16867=CARTESIAN_POINT('Ctrl Pts',(48.5725845633798,35.8793483229262,3.60701400320329));
#16868=CARTESIAN_POINT('Ctrl Pts',(48.3407853679392,36.0125314497137,3.60701400320329));
#16869=CARTESIAN_POINT('Ctrl Pts',(48.1089821836664,36.1457076343818,3.60701400320328));
#16870=CARTESIAN_POINT('Ctrl Pts',(47.6453674864979,36.4120455056142,3.60701400320328));
#16871=CARTESIAN_POINT('Ctrl Pts',(47.4135559734254,36.5452071923974,3.60701400320326));
#16872=CARTESIAN_POINT('Ctrl Pts',(47.1817401099609,36.6783613050641,3.60701400320326));
#16873=CARTESIAN_POINT('Ctrl Pts',(46.7406305897488,36.9317328641751,3.60701400320326));
#16874=CARTESIAN_POINT('Ctrl Pts',(46.2995053259033,37.1850770165972,3.60701400320326));
#16875=CARTESIAN_POINT('Ctrl Pts',(45.858362923034,37.438391319744,3.60701400320326));
#16876=CARTESIAN_POINT('Ctrl Pts',(3.56213286848821,36.3108341932625,45.8618709760874));
#16877=CARTESIAN_POINT('Ctrl Pts',(3.51887378961017,36.0430694733184,46.3280421398764));
#16878=CARTESIAN_POINT('Ctrl Pts',(3.44742574291548,35.7751733418289,46.795680048244));
#16879=CARTESIAN_POINT('Ctrl Pts',(3.24428578910431,35.2498476701132,47.7144823615628));
#16880=CARTESIAN_POINT('Ctrl Pts',(3.11082194025322,34.987765723523,48.1737954859953));
#16881=CARTESIAN_POINT('Ctrl Pts',(2.94136876951423,34.7348340040708,48.6174338169726));
#16882=CARTESIAN_POINT('Origin',(0.,57.,0.));
#16883=CARTESIAN_POINT('',(-48.3871149493437,57.,-4.33048599679673));
#16884=CARTESIAN_POINT('',(-4.32456003949879,57.,-48.3876449370521));
#16885=CARTESIAN_POINT('Origin',(0.,57.,0.));
#16886=CARTESIAN_POINT('',(-4.32456003949879,57.,-48.3876449370521));
#16887=CARTESIAN_POINT('Origin',(0.,57.,0.));
#16888=CARTESIAN_POINT('',(0.,57.,-4.33048599679673));
#16889=CARTESIAN_POINT('',(3.61292728433799,57.,-48.4459777332189));
#16890=CARTESIAN_POINT('Origin',(0.,57.,0.));
#16891=CARTESIAN_POINT('',(3.61292728433799,57.,0.));
#16892=CARTESIAN_POINT('Origin',(0.,57.,0.));
#16893=CARTESIAN_POINT('',(0.,57.,3.60701400320327));
#16894=CARTESIAN_POINT('',(3.61292728433799,57.,45.8578974271399));
#16895=CARTESIAN_POINT('',(3.61292728433799,57.,0.));
#16896=CARTESIAN_POINT('Origin',(0.,57.,0.));
#16897=CARTESIAN_POINT('Origin',(0.,57.,0.));
#16898=CARTESIAN_POINT('',(0.,57.,-4.33048599679673));
#16899=CARTESIAN_POINT('',(-4.32456003949879,57.,0.));
#16900=CARTESIAN_POINT('Origin',(0.,57.,0.));
#16901=CARTESIAN_POINT('',(0.,57.,3.60701400320327));
#16902=CARTESIAN_POINT('',(-4.32456003949879,57.,0.));
#16903=CARTESIAN_POINT('Origin',(0.,60.,0.));
#16904=CARTESIAN_POINT('',(45.858362923034,33.0633913333999,3.60701400320327));
#16905=CARTESIAN_POINT('',(45.858362923034,32.438391319744,3.60701400320325));
#16906=CARTESIAN_POINT('',(45.858362923034,60.,3.60701400320327));
#16907=CARTESIAN_POINT('',(-45.858362923034,30.686608693912,3.60701400320327));
#16908=CARTESIAN_POINT('Ctrl Pts',(45.858362923034,33.0633913333999,3.60701400320327));
#16909=CARTESIAN_POINT('Ctrl Pts',(45.0420919829705,32.8842847836873,13.9848082063042));
#16910=CARTESIAN_POINT('Ctrl Pts',(39.8371685740842,32.7083333469893,23.));
#16911=CARTESIAN_POINT('Ctrl Pts',(33.6743371481684,32.5000000136559,33.6743371481683));
#16912=CARTESIAN_POINT('Ctrl Pts',(23.,32.2916666803226,39.8371685740842));
#16913=CARTESIAN_POINT('Ctrl Pts',(12.3256628518317,32.0833333469893,46.));
#16914=CARTESIAN_POINT('Ctrl Pts',(8.45006291411674E-15,31.8750000136559,
46.));
#16915=CARTESIAN_POINT('Ctrl Pts',(-12.3256628518316,31.6666666803226,46.));
#16916=CARTESIAN_POINT('Ctrl Pts',(-23.,31.4583333469893,39.8371685740842));
#16917=CARTESIAN_POINT('Ctrl Pts',(-33.6743371481683,31.2500000136559,33.6743371481684));
#16918=CARTESIAN_POINT('Ctrl Pts',(-39.8371685740842,31.0416666803226,23.));
#16919=CARTESIAN_POINT('Ctrl Pts',(-45.0420919829705,30.8657152436245,13.9848082063043));
#16920=CARTESIAN_POINT('Ctrl Pts',(-45.858362923034,30.686608693912,3.60701400320327));
#16921=CARTESIAN_POINT('',(-45.858362923034,30.061608680256,3.60701400320318));
#16922=CARTESIAN_POINT('',(-45.858362923034,60.,3.60701400320327));
#16923=CARTESIAN_POINT('Ctrl Pts',(45.858362923034,32.438391319744,3.60701400320325));
#16924=CARTESIAN_POINT('Ctrl Pts',(45.0420919829705,32.2592847700314,13.9848082063042));
#16925=CARTESIAN_POINT('Ctrl Pts',(39.8371685740842,32.0833333333333,23.));
#16926=CARTESIAN_POINT('Ctrl Pts',(33.6743371481684,31.875,33.6743371481683));
#16927=CARTESIAN_POINT('Ctrl Pts',(23.,31.6666666666667,39.8371685740842));
#16928=CARTESIAN_POINT('Ctrl Pts',(12.3256628518317,31.4583333333333,46.));
#16929=CARTESIAN_POINT('Ctrl Pts',(8.45006291411674E-15,31.25,46.));
#16930=CARTESIAN_POINT('Ctrl Pts',(-12.3256628518316,31.0416666666667,46.));
#16931=CARTESIAN_POINT('Ctrl Pts',(-23.,30.8333333333333,39.8371685740842));
#16932=CARTESIAN_POINT('Ctrl Pts',(-33.6743371481683,30.625,33.6743371481684));
#16933=CARTESIAN_POINT('Ctrl Pts',(-39.8371685740842,30.4166666666667,23.));
#16934=CARTESIAN_POINT('Ctrl Pts',(-45.0420919829705,30.2407152299686,13.9848082063043));
#16935=CARTESIAN_POINT('Ctrl Pts',(-45.858362923034,30.061608680256,3.60701400320318));
#16936=CARTESIAN_POINT('Origin',(0.,60.,0.));
#16937=CARTESIAN_POINT('',(45.7957082162897,32.5741208584476,-4.33048599679664));
#16938=CARTESIAN_POINT('',(45.7957082162897,33.1991208721035,-4.33048599679673));
#16939=CARTESIAN_POINT('',(45.7957082162897,60.,-4.33048599679673));
#16940=CARTESIAN_POINT('',(1.95443836226898,33.7167771652757,-45.9584613611911));
#16941=CARTESIAN_POINT('Ctrl Pts',(1.95443836226898,33.7167771652757,-45.9584613611911));
#16942=CARTESIAN_POINT('Ctrl Pts',(13.2279919463142,33.5240557157094,-45.4790400544029));
#16943=CARTESIAN_POINT('Ctrl Pts',(23.,33.3333333333333,-39.8371685740842));
#16944=CARTESIAN_POINT('Ctrl Pts',(33.6743371481683,33.125,-33.6743371481684));
#16945=CARTESIAN_POINT('Ctrl Pts',(39.8371685740842,32.9166666666667,-23.));
#16946=CARTESIAN_POINT('Ctrl Pts',(44.8515840435634,32.7471553142902,-14.3147776366026));
#16947=CARTESIAN_POINT('Ctrl Pts',(45.7957082162897,32.5741208584476,-4.33048599679664));
#16948=CARTESIAN_POINT('',(2.63082218623052,34.3301917962911,-45.9247076705387));
#16949=CARTESIAN_POINT('Ctrl Pts',(2.6308221862305,34.3301917962911,-45.9247076705387));
#16950=CARTESIAN_POINT('Ctrl Pts',(2.56921791197849,34.2597950751581,-45.928236705337));
#16951=CARTESIAN_POINT('Ctrl Pts',(2.50510731292546,34.1915500441504,-45.9317853835034));
#16952=CARTESIAN_POINT('Ctrl Pts',(2.43846309439405,34.1254745197606,-45.9353231235497));
#16953=CARTESIAN_POINT('Ctrl Pts',(2.3971217800392,34.0844859826429,-45.9375176848572));
#16954=CARTESIAN_POINT('Ctrl Pts',(2.35480478224494,34.0443330034482,-45.9397080370933));
#16955=CARTESIAN_POINT('Ctrl Pts',(2.31149948807074,34.0050278948341,-45.9418868802387));
#16956=CARTESIAN_POINT('Ctrl Pts',(2.26335270074926,33.9613285102397,-45.9443093160985));
#16957=CARTESIAN_POINT('Ctrl Pts',(2.21394822234029,33.9186513826451,-45.946718418332));
#16958=CARTESIAN_POINT('Ctrl Pts',(2.16351946109064,33.8772218703134,-45.9490927134335));
#16959=CARTESIAN_POINT('Ctrl Pts',(2.11305915068249,33.8357664389186,-45.9514684939376));
#16960=CARTESIAN_POINT('Ctrl Pts',(2.06157358891504,33.7955604486027,-45.9538094237443));
#16961=CARTESIAN_POINT('Ctrl Pts',(2.00932978732685,33.7567892931775,-45.95609398902));
#16962=CARTESIAN_POINT('Ctrl Pts',(1.99112044191851,33.7432757788551,-45.9568902641177));
#16963=CARTESIAN_POINT('Ctrl Pts',(1.97281925470307,33.7299361972055,-45.9576796918261));
#16964=CARTESIAN_POINT('Ctrl Pts',(1.95443836226869,33.7167771652761,-45.9584613611911));
#16965=CARTESIAN_POINT('Ctrl Pts',(2.63082218623052,34.3301917962911,-45.9247076705387));
#16966=CARTESIAN_POINT('Ctrl Pts',(13.5383323474866,34.1429987490258,-45.2998649402456));
#16967=CARTESIAN_POINT('Ctrl Pts',(23.,33.9583333469893,-39.8371685740842));
#16968=CARTESIAN_POINT('Ctrl Pts',(33.6743371481683,33.7500000136559,-33.6743371481684));
#16969=CARTESIAN_POINT('Ctrl Pts',(39.8371685740842,33.5416666803226,-23.));
#16970=CARTESIAN_POINT('Ctrl Pts',(44.8515840435634,33.3721553279462,-14.3147776366027));
#16971=CARTESIAN_POINT('Ctrl Pts',(45.7957082162897,33.1991208721035,-4.33048599679673));
#16972=CARTESIAN_POINT('Origin',(0.,60.,0.));
#16973=CARTESIAN_POINT('',(-45.7957082162897,34.9258791415524,-4.33048599679682));
#16974=CARTESIAN_POINT('',(-45.7957082162897,60.,-4.33048599679673));
#16975=CARTESIAN_POINT('',(-2.77456427460704,33.7972761197826,-45.9162475937012));
#16976=CARTESIAN_POINT('Ctrl Pts',(-2.77456427460705,33.7972761197826,-45.9162475937012));
#16977=CARTESIAN_POINT('Ctrl Pts',(-2.8485761476615,33.8541693341362,-45.9117753053581));
#16978=CARTESIAN_POINT('Ctrl Pts',(-2.92014445685112,33.9133331099627,-45.9072715943004));
#16979=CARTESIAN_POINT('Ctrl Pts',(-2.98933369598369,33.9747022029095,-45.9027657035543));
#16980=CARTESIAN_POINT('Ctrl Pts',(-3.03440838807543,34.0146823067985,-45.8998302523118));
#16981=CARTESIAN_POINT('Ctrl Pts',(-3.07847297023139,34.0555994041398,-45.8968938759819));
#16982=CARTESIAN_POINT('Ctrl Pts',(-3.12153932925008,34.0974457295403,-45.8939646600285));
#16983=CARTESIAN_POINT('Ctrl Pts',(-3.1893556202593,34.1633408422383,-45.8893520443803));
#16984=CARTESIAN_POINT('Ctrl Pts',(-3.25469619442314,34.2315362288938,-45.8847569569152));
#16985=CARTESIAN_POINT('Ctrl Pts',(-3.31757026199471,34.3020256949546,-45.8802105832609));
#16986=CARTESIAN_POINT('Ctrl Pts',(-3.35591287101332,34.3450124165315,-45.8774380597992));
#16987=CARTESIAN_POINT('Ctrl Pts',(-3.39333752726835,34.3888530647444,-45.8746836527545));
#16988=CARTESIAN_POINT('Ctrl Pts',(-3.42983911135813,34.4335524565479,-45.87195443482));
#16989=CARTESIAN_POINT('Ctrl Pts',(-45.7957082162897,34.9258791415524,-4.33048599679682));
#16990=CARTESIAN_POINT('Ctrl Pts',(-44.8515840435634,34.7528446857097,-14.3147776366027));
#16991=CARTESIAN_POINT('Ctrl Pts',(-39.8371685740842,34.5833333333333,-23.));
#16992=CARTESIAN_POINT('Ctrl Pts',(-33.6743371481684,34.375,-33.6743371481684));
#16993=CARTESIAN_POINT('Ctrl Pts',(-23.,34.1666666666667,-39.8371685740842));
#16994=CARTESIAN_POINT('Ctrl Pts',(-13.6041749881978,33.9832863296065,-45.2618506739068));
#16995=CARTESIAN_POINT('Ctrl Pts',(-2.77456427460704,33.7972761197826,-45.9162475937012));
#16996=CARTESIAN_POINT('Origin',(0.,60.,0.));
#16997=CARTESIAN_POINT('',(-45.858362923034,35.061608680256,3.60701400320325));
#16998=CARTESIAN_POINT('',(-45.858362923034,60.,3.60701400320327));
#16999=CARTESIAN_POINT('',(-4.24983907177925,36.1772764823076,45.8032626333974));
#17000=CARTESIAN_POINT('Ctrl Pts',(-4.24983907177925,36.1772764823076,45.8032626333974));
#17001=CARTESIAN_POINT('Ctrl Pts',(-14.2780294172147,36.0035619086092,44.8728006379193));
#17002=CARTESIAN_POINT('Ctrl Pts',(-23.,35.8333333333333,39.8371685740842));
#17003=CARTESIAN_POINT('Ctrl Pts',(-33.6743371481683,35.625,33.6743371481684));
#17004=CARTESIAN_POINT('Ctrl Pts',(-39.8371685740842,35.4166666666667,23.));
#17005=CARTESIAN_POINT('Ctrl Pts',(-45.0420919829705,35.2407152299686,13.9848082063043));
#17006=CARTESIAN_POINT('Ctrl Pts',(-45.858362923034,35.061608680256,3.60701400320325));
#17007=CARTESIAN_POINT('Ctrl Pts',(-4.32199731091473,36.8010262662206,45.796510120799));
#17008=CARTESIAN_POINT('Ctrl Pts',(-4.31460736934614,36.5957426618924,45.7972075387355));
#17009=CARTESIAN_POINT('Ctrl Pts',(-4.29092724654331,36.3860078913526,45.7994502820394));
#17010=CARTESIAN_POINT('Ctrl Pts',(-4.24983907177925,36.1772764823076,45.8032626333974));
#17011=CARTESIAN_POINT('Ctrl Pts',(-46.,55.6250000136559,0.));
#17012=CARTESIAN_POINT('Ctrl Pts',(-46.,55.4166666803226,-12.3256628518316));
#17013=CARTESIAN_POINT('Ctrl Pts',(-39.8371685740842,55.2083333469893,-23.));
#17014=CARTESIAN_POINT('Ctrl Pts',(-33.6743371481684,55.0000000136559,-33.6743371481684));
#17015=CARTESIAN_POINT('Ctrl Pts',(-23.,54.7916666803226,-39.8371685740842));
#17016=CARTESIAN_POINT('Ctrl Pts',(-12.3256628518317,54.5833333469893,-46.));
#17017=CARTESIAN_POINT('Ctrl Pts',(-2.81668763803891E-15,54.3750000136559,
-46.));
#17018=CARTESIAN_POINT('Ctrl Pts',(12.3256628518316,54.1666666803226,-46.));
#17019=CARTESIAN_POINT('Ctrl Pts',(23.,53.9583333469893,-39.8371685740842));
#17020=CARTESIAN_POINT('Ctrl Pts',(33.6743371481683,53.7500000136559,-33.6743371481684));
#17021=CARTESIAN_POINT('Ctrl Pts',(39.8371685740842,53.5416666803226,-23.));
#17022=CARTESIAN_POINT('Ctrl Pts',(46.,53.3333333469893,-12.3256628518317));
#17023=CARTESIAN_POINT('Ctrl Pts',(46.,53.1250000136559,-5.63337527607782E-15));
#17024=CARTESIAN_POINT('Ctrl Pts',(46.,52.9166666803226,12.3256628518316));
#17025=CARTESIAN_POINT('Ctrl Pts',(39.8371685740842,52.7083333469893,23.));
#17026=CARTESIAN_POINT('Ctrl Pts',(33.6743371481684,52.5000000136559,33.6743371481683));
#17027=CARTESIAN_POINT('Ctrl Pts',(23.,52.2916666803226,39.8371685740842));
#17028=CARTESIAN_POINT('Ctrl Pts',(12.3256628518317,52.0833333469893,46.));
#17029=CARTESIAN_POINT('Ctrl Pts',(8.45006291411674E-15,51.8750000136559,
46.));
#17030=CARTESIAN_POINT('Ctrl Pts',(-12.3256628518316,51.6666666803226,46.));
#17031=CARTESIAN_POINT('Ctrl Pts',(-23.,51.4583333469893,39.8371685740842));
#17032=CARTESIAN_POINT('Ctrl Pts',(-33.6743371481683,51.2500000136559,33.6743371481684));
#17033=CARTESIAN_POINT('Ctrl Pts',(-39.8371685740842,51.0416666803226,23.));
#17034=CARTESIAN_POINT('Ctrl Pts',(-46.,50.8333333469893,12.3256628518317));
#17035=CARTESIAN_POINT('Ctrl Pts',(-46.,50.6250000136559,0.));
#17036=CARTESIAN_POINT('Ctrl Pts',(-46.,50.4166666803226,-12.3256628518316));
#17037=CARTESIAN_POINT('Ctrl Pts',(-39.8371685740842,50.2083333469893,-23.));
#17038=CARTESIAN_POINT('Ctrl Pts',(-33.6743371481684,50.0000000136559,-33.6743371481684));
#17039=CARTESIAN_POINT('Ctrl Pts',(-23.,49.7916666803226,-39.8371685740842));
#17040=CARTESIAN_POINT('Ctrl Pts',(-12.3256628518317,49.5833333469893,-46.));
#17041=CARTESIAN_POINT('Ctrl Pts',(-2.81668763803891E-15,49.3750000136559,
-46.));
#17042=CARTESIAN_POINT('Ctrl Pts',(12.3256628518316,49.1666666803226,-46.));
#17043=CARTESIAN_POINT('Ctrl Pts',(23.,48.9583333469893,-39.8371685740842));
#17044=CARTESIAN_POINT('Ctrl Pts',(33.6743371481683,48.7500000136559,-33.6743371481684));
#17045=CARTESIAN_POINT('Ctrl Pts',(39.8371685740842,48.5416666803226,-23.));
#17046=CARTESIAN_POINT('Ctrl Pts',(46.,48.3333333469893,-12.3256628518317));
#17047=CARTESIAN_POINT('Ctrl Pts',(46.,48.1250000136559,-5.63337527607782E-15));
#17048=CARTESIAN_POINT('Ctrl Pts',(46.,47.9166666803226,12.3256628518316));
#17049=CARTESIAN_POINT('Ctrl Pts',(39.8371685740842,47.7083333469893,23.));
#17050=CARTESIAN_POINT('Ctrl Pts',(33.6743371481684,47.5000000136559,33.6743371481683));
#17051=CARTESIAN_POINT('Ctrl Pts',(23.,47.2916666803226,39.8371685740842));
#17052=CARTESIAN_POINT('Ctrl Pts',(12.3256628518317,47.0833333469893,46.));
#17053=CARTESIAN_POINT('Ctrl Pts',(8.45006291411674E-15,46.8750000136559,
46.));
#17054=CARTESIAN_POINT('Ctrl Pts',(-12.3256628518316,46.6666666803226,46.));
#17055=CARTESIAN_POINT('Ctrl Pts',(-23.,46.4583333469893,39.8371685740842));
#17056=CARTESIAN_POINT('Ctrl Pts',(-33.6743371481683,46.2500000136559,33.6743371481684));
#17057=CARTESIAN_POINT('Ctrl Pts',(-39.8371685740842,46.0416666803226,23.));
#17058=CARTESIAN_POINT('Ctrl Pts',(-46.,45.8333333469892,12.3256628518317));
#17059=CARTESIAN_POINT('Ctrl Pts',(-46.,45.6250000136559,0.));
#17060=CARTESIAN_POINT('Ctrl Pts',(-46.,45.4166666803226,-12.3256628518316));
#17061=CARTESIAN_POINT('Ctrl Pts',(-39.8371685740842,45.2083333469893,-23.));
#17062=CARTESIAN_POINT('Ctrl Pts',(-33.6743371481684,45.0000000136559,-33.6743371481684));
#17063=CARTESIAN_POINT('Ctrl Pts',(-23.,44.7916666803226,-39.8371685740842));
#17064=CARTESIAN_POINT('Ctrl Pts',(-12.3256628518317,44.5833333469893,-46.));
#17065=CARTESIAN_POINT('Ctrl Pts',(-2.81668763803891E-15,44.3750000136559,
-46.));
#17066=CARTESIAN_POINT('Ctrl Pts',(12.3256628518316,44.1666666803226,-46.));
#17067=CARTESIAN_POINT('Ctrl Pts',(23.,43.9583333469893,-39.8371685740842));
#17068=CARTESIAN_POINT('Ctrl Pts',(33.6743371481683,43.7500000136559,-33.6743371481684));
#17069=CARTESIAN_POINT('Ctrl Pts',(39.8371685740842,43.5416666803226,-23.));
#17070=CARTESIAN_POINT('Ctrl Pts',(46.,43.3333333469893,-12.3256628518317));
#17071=CARTESIAN_POINT('Ctrl Pts',(46.,43.1250000136559,-5.63337527607782E-15));
#17072=CARTESIAN_POINT('Ctrl Pts',(46.,42.9166666803226,12.3256628518316));
#17073=CARTESIAN_POINT('Ctrl Pts',(39.8371685740842,42.7083333469893,23.));
#17074=CARTESIAN_POINT('Ctrl Pts',(33.6743371481684,42.5000000136559,33.6743371481683));
#17075=CARTESIAN_POINT('Ctrl Pts',(23.,42.2916666803226,39.8371685740842));
#17076=CARTESIAN_POINT('Ctrl Pts',(12.3256628518317,42.0833333469893,46.));
#17077=CARTESIAN_POINT('Ctrl Pts',(8.45006291411674E-15,41.8750000136559,
46.));
#17078=CARTESIAN_POINT('Ctrl Pts',(-12.3256628518316,41.6666666803226,46.));
#17079=CARTESIAN_POINT('Ctrl Pts',(-23.,41.4583333469893,39.8371685740842));
#17080=CARTESIAN_POINT('Ctrl Pts',(-33.6743371481683,41.2500000136559,33.6743371481684));
#17081=CARTESIAN_POINT('Ctrl Pts',(-39.8371685740842,41.0416666803226,23.));
#17082=CARTESIAN_POINT('Ctrl Pts',(-46.,40.8333333469893,12.3256628518317));
#17083=CARTESIAN_POINT('Ctrl Pts',(-46.,40.6250000136559,0.));
#17084=CARTESIAN_POINT('Ctrl Pts',(-46.,40.4166666803226,-12.3256628518316));
#17085=CARTESIAN_POINT('Ctrl Pts',(-39.8371685740842,40.2083333469893,-23.));
#17086=CARTESIAN_POINT('Ctrl Pts',(-33.6743371481684,40.0000000136559,-33.6743371481684));
#17087=CARTESIAN_POINT('Ctrl Pts',(-23.,39.7916666803226,-39.8371685740842));
#17088=CARTESIAN_POINT('Ctrl Pts',(-12.3256628518317,39.5833333469893,-46.));
#17089=CARTESIAN_POINT('Ctrl Pts',(-2.81668763803891E-15,39.3750000136559,
-46.));
#17090=CARTESIAN_POINT('Ctrl Pts',(12.3256628518316,39.1666666803226,-46.));
#17091=CARTESIAN_POINT('Ctrl Pts',(23.,38.9583333469893,-39.8371685740842));
#17092=CARTESIAN_POINT('Ctrl Pts',(33.6743371481683,38.7500000136559,-33.6743371481684));
#17093=CARTESIAN_POINT('Ctrl Pts',(39.8371685740842,38.5416666803226,-23.));
#17094=CARTESIAN_POINT('Ctrl Pts',(46.,38.3333333469893,-12.3256628518317));
#17095=CARTESIAN_POINT('Ctrl Pts',(46.,38.1250000136559,-5.63337527607782E-15));
#17096=CARTESIAN_POINT('Ctrl Pts',(46.,37.9166666803226,12.3256628518316));
#17097=CARTESIAN_POINT('Ctrl Pts',(39.8371685740842,37.7083333469893,23.));
#17098=CARTESIAN_POINT('Ctrl Pts',(33.6743371481684,37.5000000136559,33.6743371481683));
#17099=CARTESIAN_POINT('Ctrl Pts',(23.,37.2916666803226,39.8371685740842));
#17100=CARTESIAN_POINT('Ctrl Pts',(12.3256628518317,37.0833333469893,46.));
#17101=CARTESIAN_POINT('Ctrl Pts',(8.45006291411674E-15,36.8750000136559,
46.));
#17102=CARTESIAN_POINT('Ctrl Pts',(-12.3256628518316,36.6666666803226,46.));
#17103=CARTESIAN_POINT('Ctrl Pts',(-23.,36.4583333469893,39.8371685740842));
#17104=CARTESIAN_POINT('Ctrl Pts',(-33.6743371481683,36.2500000136559,33.6743371481684));
#17105=CARTESIAN_POINT('Ctrl Pts',(-39.8371685740842,36.0416666803226,23.));
#17106=CARTESIAN_POINT('Ctrl Pts',(-46.,35.8333333469893,12.3256628518317));
#17107=CARTESIAN_POINT('Ctrl Pts',(-46.,35.6250000136559,0.));
#17108=CARTESIAN_POINT('Ctrl Pts',(-46.,35.4166666803226,-12.3256628518316));
#17109=CARTESIAN_POINT('Ctrl Pts',(-39.8371685740842,35.2083333469893,-23.));
#17110=CARTESIAN_POINT('Ctrl Pts',(-33.6743371481684,35.0000000136559,-33.6743371481684));
#17111=CARTESIAN_POINT('Ctrl Pts',(-23.,34.7916666803226,-39.8371685740842));
#17112=CARTESIAN_POINT('Ctrl Pts',(-12.3256628518317,34.5833333469893,-46.));
#17113=CARTESIAN_POINT('Ctrl Pts',(-2.81668763803891E-15,34.3750000136559,
-46.));
#17114=CARTESIAN_POINT('Ctrl Pts',(12.3256628518316,34.1666666803226,-46.));
#17115=CARTESIAN_POINT('Ctrl Pts',(23.,33.9583333469893,-39.8371685740842));
#17116=CARTESIAN_POINT('Ctrl Pts',(33.6743371481683,33.7500000136559,-33.6743371481684));
#17117=CARTESIAN_POINT('Ctrl Pts',(39.8371685740842,33.5416666803226,-23.));
#17118=CARTESIAN_POINT('Ctrl Pts',(46.,33.3333333469893,-12.3256628518317));
#17119=CARTESIAN_POINT('Ctrl Pts',(46.,33.1250000136559,-5.63337527607782E-15));
#17120=CARTESIAN_POINT('Ctrl Pts',(46.,32.9166666803226,12.3256628518316));
#17121=CARTESIAN_POINT('Ctrl Pts',(39.8371685740842,32.7083333469893,23.));
#17122=CARTESIAN_POINT('Ctrl Pts',(33.6743371481684,32.5000000136559,33.6743371481683));
#17123=CARTESIAN_POINT('Ctrl Pts',(23.,32.2916666803226,39.8371685740842));
#17124=CARTESIAN_POINT('Ctrl Pts',(12.3256628518317,32.0833333469893,46.));
#17125=CARTESIAN_POINT('Ctrl Pts',(8.45006291411674E-15,31.8750000136559,
46.));
#17126=CARTESIAN_POINT('Ctrl Pts',(-12.3256628518316,31.6666666803226,46.));
#17127=CARTESIAN_POINT('Ctrl Pts',(-23.,31.4583333469893,39.8371685740842));
#17128=CARTESIAN_POINT('Ctrl Pts',(-33.6743371481683,31.2500000136559,33.6743371481684));
#17129=CARTESIAN_POINT('Ctrl Pts',(-39.8371685740842,31.0416666803226,23.));
#17130=CARTESIAN_POINT('Ctrl Pts',(-46.,30.8333333469893,12.3256628518317));
#17131=CARTESIAN_POINT('Ctrl Pts',(-46.,30.6250000136559,0.));
#17132=CARTESIAN_POINT('Ctrl Pts',(-46.,30.4166666803226,-12.3256628518316));
#17133=CARTESIAN_POINT('Ctrl Pts',(-39.8371685740842,30.2083333469893,-23.));
#17134=CARTESIAN_POINT('Ctrl Pts',(-33.6743371481684,30.0000000136559,-33.6743371481684));
#17135=CARTESIAN_POINT('Ctrl Pts',(-23.,29.7916666803226,-39.8371685740842));
#17136=CARTESIAN_POINT('Ctrl Pts',(-12.3256628518317,29.5833333469893,-46.));
#17137=CARTESIAN_POINT('Ctrl Pts',(-2.81668763803891E-15,29.3750000136559,
-46.));
#17138=CARTESIAN_POINT('Ctrl Pts',(12.3256628518316,29.1666666803226,-46.));
#17139=CARTESIAN_POINT('Ctrl Pts',(23.,28.9583333469893,-39.8371685740842));
#17140=CARTESIAN_POINT('Ctrl Pts',(33.6743371481683,28.7500000136559,-33.6743371481684));
#17141=CARTESIAN_POINT('Ctrl Pts',(39.8371685740842,28.5416666803226,-23.));
#17142=CARTESIAN_POINT('Ctrl Pts',(46.,28.3333333469893,-12.3256628518317));
#17143=CARTESIAN_POINT('Ctrl Pts',(46.,28.1250000136559,-5.63337527607782E-15));
#17144=CARTESIAN_POINT('Ctrl Pts',(46.,27.9166666803226,12.3256628518316));
#17145=CARTESIAN_POINT('Ctrl Pts',(39.8371685740842,27.7083333469893,23.));
#17146=CARTESIAN_POINT('Ctrl Pts',(33.6743371481684,27.5000000136559,33.6743371481683));
#17147=CARTESIAN_POINT('Ctrl Pts',(23.,27.2916666803226,39.8371685740842));
#17148=CARTESIAN_POINT('Ctrl Pts',(12.3256628518317,27.0833333469893,46.));
#17149=CARTESIAN_POINT('Ctrl Pts',(8.45006291411674E-15,26.8750000136559,
46.));
#17150=CARTESIAN_POINT('Ctrl Pts',(-12.3256628518316,26.6666666803226,46.));
#17151=CARTESIAN_POINT('Ctrl Pts',(-23.,26.4583333469893,39.8371685740842));
#17152=CARTESIAN_POINT('Ctrl Pts',(-33.6743371481683,26.2500000136559,33.6743371481684));
#17153=CARTESIAN_POINT('Ctrl Pts',(-39.8371685740842,26.0416666803226,23.));
#17154=CARTESIAN_POINT('Ctrl Pts',(-46.,25.8333333469893,12.3256628518317));
#17155=CARTESIAN_POINT('Ctrl Pts',(-46.,25.6250000136559,0.));
#17156=CARTESIAN_POINT('Ctrl Pts',(-48.706329375,57.187500006828,-1.8898197019151E-14));
#17157=CARTESIAN_POINT('Ctrl Pts',(-48.706329375,56.9791666734946,-13.0508216223155));
#17158=CARTESIAN_POINT('Ctrl Pts',(-42.1809185638422,56.7708333401613,-24.3531646875));
#17159=CARTESIAN_POINT('Ctrl Pts',(-35.6555077526845,56.562500006828,-35.6555077526845));
#17160=CARTESIAN_POINT('Ctrl Pts',(-24.3531646875,56.3541666734946,-42.1809185638423));
#17161=CARTESIAN_POINT('Ctrl Pts',(-13.0508216223155,56.1458333401613,-48.706329375));
#17162=CARTESIAN_POINT('Ctrl Pts',(1.59157945007855E-14,55.937500006828,
-48.706329375));
#17163=CARTESIAN_POINT('Ctrl Pts',(13.0508216223155,55.7291666734946,-48.706329375));
#17164=CARTESIAN_POINT('Ctrl Pts',(24.3531646875,55.5208333401613,-42.1809185638422));
#17165=CARTESIAN_POINT('Ctrl Pts',(35.6555077526845,55.312500006828,-35.6555077526845));
#17166=CARTESIAN_POINT('Ctrl Pts',(42.1809185638422,55.1041666734946,-24.3531646875));
#17167=CARTESIAN_POINT('Ctrl Pts',(48.706329375,54.8958333401613,-13.0508216223155));
#17168=CARTESIAN_POINT('Ctrl Pts',(48.706329375,54.687500006828,1.293339198242E-14));
#17169=CARTESIAN_POINT('Ctrl Pts',(48.706329375,54.4791666734946,13.0508216223155));
#17170=CARTESIAN_POINT('Ctrl Pts',(42.1809185638422,54.2708333401613,24.3531646875));
#17171=CARTESIAN_POINT('Ctrl Pts',(35.6555077526845,54.062500006828,35.6555077526845));
#17172=CARTESIAN_POINT('Ctrl Pts',(24.3531646875,53.8541666734946,42.1809185638422));
#17173=CARTESIAN_POINT('Ctrl Pts',(13.0508216223155,53.6458333401613,48.706329375));
#17174=CARTESIAN_POINT('Ctrl Pts',(-9.95098946405443E-15,53.437500006828,
48.706329375));
#17175=CARTESIAN_POINT('Ctrl Pts',(-13.0508216223155,53.2291666734946,48.706329375));
#17176=CARTESIAN_POINT('Ctrl Pts',(-24.3531646875,53.0208333401613,42.1809185638423));
#17177=CARTESIAN_POINT('Ctrl Pts',(-35.6555077526845,52.812500006828,35.6555077526845));
#17178=CARTESIAN_POINT('Ctrl Pts',(-42.1809185638422,52.6041666734946,24.3531646875));
#17179=CARTESIAN_POINT('Ctrl Pts',(-48.706329375,52.3958333401613,13.0508216223155));
#17180=CARTESIAN_POINT('Ctrl Pts',(-48.706329375,52.187500006828,-1.8898197019151E-14));
#17181=CARTESIAN_POINT('Ctrl Pts',(-48.706329375,51.9791666734946,-13.0508216223155));
#17182=CARTESIAN_POINT('Ctrl Pts',(-42.1809185638422,51.7708333401613,-24.3531646875));
#17183=CARTESIAN_POINT('Ctrl Pts',(-35.6555077526845,51.562500006828,-35.6555077526845));
#17184=CARTESIAN_POINT('Ctrl Pts',(-24.3531646875,51.3541666734946,-42.1809185638423));
#17185=CARTESIAN_POINT('Ctrl Pts',(-13.0508216223155,51.1458333401613,-48.706329375));
#17186=CARTESIAN_POINT('Ctrl Pts',(1.59157945007855E-14,50.937500006828,
-48.706329375));
#17187=CARTESIAN_POINT('Ctrl Pts',(13.0508216223155,50.7291666734946,-48.706329375));
#17188=CARTESIAN_POINT('Ctrl Pts',(24.3531646875,50.5208333401613,-42.1809185638422));
#17189=CARTESIAN_POINT('Ctrl Pts',(35.6555077526845,50.312500006828,-35.6555077526845));
#17190=CARTESIAN_POINT('Ctrl Pts',(42.1809185638422,50.1041666734946,-24.3531646875));
#17191=CARTESIAN_POINT('Ctrl Pts',(48.706329375,49.8958333401613,-13.0508216223155));
#17192=CARTESIAN_POINT('Ctrl Pts',(48.706329375,49.687500006828,1.293339198242E-14));
#17193=CARTESIAN_POINT('Ctrl Pts',(48.706329375,49.4791666734946,13.0508216223155));
#17194=CARTESIAN_POINT('Ctrl Pts',(42.1809185638422,49.2708333401613,24.3531646875));
#17195=CARTESIAN_POINT('Ctrl Pts',(35.6555077526845,49.062500006828,35.6555077526845));
#17196=CARTESIAN_POINT('Ctrl Pts',(24.3531646875,48.8541666734946,42.1809185638422));
#17197=CARTESIAN_POINT('Ctrl Pts',(13.0508216223155,48.6458333401613,48.706329375));
#17198=CARTESIAN_POINT('Ctrl Pts',(-9.95098946405443E-15,48.437500006828,
48.706329375));
#17199=CARTESIAN_POINT('Ctrl Pts',(-13.0508216223155,48.2291666734946,48.706329375));
#17200=CARTESIAN_POINT('Ctrl Pts',(-24.3531646875,48.0208333401613,42.1809185638423));
#17201=CARTESIAN_POINT('Ctrl Pts',(-35.6555077526845,47.812500006828,35.6555077526845));
#17202=CARTESIAN_POINT('Ctrl Pts',(-42.1809185638422,47.6041666734946,24.3531646875));
#17203=CARTESIAN_POINT('Ctrl Pts',(-48.706329375,47.3958333401613,13.0508216223155));
#17204=CARTESIAN_POINT('Ctrl Pts',(-48.706329375,47.187500006828,-1.8898197019151E-14));
#17205=CARTESIAN_POINT('Ctrl Pts',(-48.706329375,46.9791666734946,-13.0508216223155));
#17206=CARTESIAN_POINT('Ctrl Pts',(-42.1809185638422,46.7708333401613,-24.3531646875));
#17207=CARTESIAN_POINT('Ctrl Pts',(-35.6555077526845,46.562500006828,-35.6555077526845));
#17208=CARTESIAN_POINT('Ctrl Pts',(-24.3531646875,46.3541666734946,-42.1809185638423));
#17209=CARTESIAN_POINT('Ctrl Pts',(-13.0508216223155,46.1458333401613,-48.706329375));
#17210=CARTESIAN_POINT('Ctrl Pts',(1.59157945007855E-14,45.937500006828,
-48.706329375));
#17211=CARTESIAN_POINT('Ctrl Pts',(13.0508216223155,45.7291666734946,-48.706329375));
#17212=CARTESIAN_POINT('Ctrl Pts',(24.3531646875,45.5208333401613,-42.1809185638422));
#17213=CARTESIAN_POINT('Ctrl Pts',(35.6555077526845,45.312500006828,-35.6555077526845));
#17214=CARTESIAN_POINT('Ctrl Pts',(42.1809185638422,45.1041666734946,-24.3531646875));
#17215=CARTESIAN_POINT('Ctrl Pts',(48.706329375,44.8958333401613,-13.0508216223155));
#17216=CARTESIAN_POINT('Ctrl Pts',(48.706329375,44.687500006828,1.293339198242E-14));
#17217=CARTESIAN_POINT('Ctrl Pts',(48.706329375,44.4791666734946,13.0508216223155));
#17218=CARTESIAN_POINT('Ctrl Pts',(42.1809185638422,44.2708333401613,24.3531646875));
#17219=CARTESIAN_POINT('Ctrl Pts',(35.6555077526845,44.062500006828,35.6555077526845));
#17220=CARTESIAN_POINT('Ctrl Pts',(24.3531646875,43.8541666734946,42.1809185638422));
#17221=CARTESIAN_POINT('Ctrl Pts',(13.0508216223155,43.6458333401613,48.706329375));
#17222=CARTESIAN_POINT('Ctrl Pts',(-9.95098946405443E-15,43.437500006828,
48.706329375));
#17223=CARTESIAN_POINT('Ctrl Pts',(-13.0508216223155,43.2291666734946,48.706329375));
#17224=CARTESIAN_POINT('Ctrl Pts',(-24.3531646875,43.0208333401613,42.1809185638423));
#17225=CARTESIAN_POINT('Ctrl Pts',(-35.6555077526845,42.812500006828,35.6555077526845));
#17226=CARTESIAN_POINT('Ctrl Pts',(-42.1809185638422,42.6041666734946,24.3531646875));
#17227=CARTESIAN_POINT('Ctrl Pts',(-48.706329375,42.3958333401613,13.0508216223155));
#17228=CARTESIAN_POINT('Ctrl Pts',(-48.706329375,42.187500006828,-1.8898197019151E-14));
#17229=CARTESIAN_POINT('Ctrl Pts',(-48.706329375,41.9791666734946,-13.0508216223155));
#17230=CARTESIAN_POINT('Ctrl Pts',(-42.1809185638422,41.7708333401613,-24.3531646875));
#17231=CARTESIAN_POINT('Ctrl Pts',(-35.6555077526845,41.562500006828,-35.6555077526845));
#17232=CARTESIAN_POINT('Ctrl Pts',(-24.3531646875,41.3541666734946,-42.1809185638423));
#17233=CARTESIAN_POINT('Ctrl Pts',(-13.0508216223155,41.1458333401613,-48.706329375));
#17234=CARTESIAN_POINT('Ctrl Pts',(1.59157945007855E-14,40.937500006828,
-48.706329375));
#17235=CARTESIAN_POINT('Ctrl Pts',(13.0508216223155,40.7291666734946,-48.706329375));
#17236=CARTESIAN_POINT('Ctrl Pts',(24.3531646875,40.5208333401613,-42.1809185638422));
#17237=CARTESIAN_POINT('Ctrl Pts',(35.6555077526845,40.312500006828,-35.6555077526845));
#17238=CARTESIAN_POINT('Ctrl Pts',(42.1809185638422,40.1041666734946,-24.3531646875));
#17239=CARTESIAN_POINT('Ctrl Pts',(48.706329375,39.8958333401613,-13.0508216223155));
#17240=CARTESIAN_POINT('Ctrl Pts',(48.706329375,39.687500006828,1.293339198242E-14));
#17241=CARTESIAN_POINT('Ctrl Pts',(48.706329375,39.4791666734946,13.0508216223155));
#17242=CARTESIAN_POINT('Ctrl Pts',(42.1809185638422,39.2708333401613,24.3531646875));
#17243=CARTESIAN_POINT('Ctrl Pts',(35.6555077526845,39.062500006828,35.6555077526845));
#17244=CARTESIAN_POINT('Ctrl Pts',(24.3531646875,38.8541666734946,42.1809185638422));
#17245=CARTESIAN_POINT('Ctrl Pts',(13.0508216223155,38.6458333401613,48.706329375));
#17246=CARTESIAN_POINT('Ctrl Pts',(-9.95098946405443E-15,38.437500006828,
48.706329375));
#17247=CARTESIAN_POINT('Ctrl Pts',(-13.0508216223155,38.2291666734946,48.706329375));
#17248=CARTESIAN_POINT('Ctrl Pts',(-24.3531646875,38.0208333401613,42.1809185638423));
#17249=CARTESIAN_POINT('Ctrl Pts',(-35.6555077526845,37.812500006828,35.6555077526845));
#17250=CARTESIAN_POINT('Ctrl Pts',(-42.1809185638422,37.6041666734946,24.3531646875));
#17251=CARTESIAN_POINT('Ctrl Pts',(-48.706329375,37.3958333401613,13.0508216223155));
#17252=CARTESIAN_POINT('Ctrl Pts',(-48.706329375,37.187500006828,-1.8898197019151E-14));
#17253=CARTESIAN_POINT('Ctrl Pts',(-48.706329375,36.9791666734946,-13.0508216223155));
#17254=CARTESIAN_POINT('Ctrl Pts',(-42.1809185638422,36.7708333401613,-24.3531646875));
#17255=CARTESIAN_POINT('Ctrl Pts',(-35.6555077526845,36.562500006828,-35.6555077526845));
#17256=CARTESIAN_POINT('Ctrl Pts',(-24.3531646875,36.3541666734946,-42.1809185638423));
#17257=CARTESIAN_POINT('Ctrl Pts',(-13.0508216223155,36.1458333401613,-48.706329375));
#17258=CARTESIAN_POINT('Ctrl Pts',(1.59157945007855E-14,35.937500006828,
-48.706329375));
#17259=CARTESIAN_POINT('Ctrl Pts',(13.0508216223155,35.7291666734946,-48.706329375));
#17260=CARTESIAN_POINT('Ctrl Pts',(24.3531646875,35.5208333401613,-42.1809185638422));
#17261=CARTESIAN_POINT('Ctrl Pts',(35.6555077526845,35.312500006828,-35.6555077526845));
#17262=CARTESIAN_POINT('Ctrl Pts',(42.1809185638422,35.1041666734946,-24.3531646875));
#17263=CARTESIAN_POINT('Ctrl Pts',(48.706329375,34.8958333401613,-13.0508216223155));
#17264=CARTESIAN_POINT('Ctrl Pts',(48.706329375,34.687500006828,1.293339198242E-14));
#17265=CARTESIAN_POINT('Ctrl Pts',(48.706329375,34.4791666734946,13.0508216223155));
#17266=CARTESIAN_POINT('Ctrl Pts',(42.1809185638422,34.2708333401613,24.3531646875));
#17267=CARTESIAN_POINT('Ctrl Pts',(35.6555077526845,34.062500006828,35.6555077526845));
#17268=CARTESIAN_POINT('Ctrl Pts',(24.3531646875,33.8541666734946,42.1809185638422));
#17269=CARTESIAN_POINT('Ctrl Pts',(13.0508216223155,33.6458333401613,48.706329375));
#17270=CARTESIAN_POINT('Ctrl Pts',(-9.95098946405443E-15,33.437500006828,
48.706329375));
#17271=CARTESIAN_POINT('Ctrl Pts',(-13.0508216223155,33.2291666734946,48.706329375));
#17272=CARTESIAN_POINT('Ctrl Pts',(-24.3531646875,33.0208333401613,42.1809185638423));
#17273=CARTESIAN_POINT('Ctrl Pts',(-35.6555077526845,32.812500006828,35.6555077526845));
#17274=CARTESIAN_POINT('Ctrl Pts',(-42.1809185638422,32.6041666734946,24.3531646875));
#17275=CARTESIAN_POINT('Ctrl Pts',(-48.706329375,32.3958333401613,13.0508216223155));
#17276=CARTESIAN_POINT('Ctrl Pts',(-48.706329375,32.187500006828,-1.8898197019151E-14));
#17277=CARTESIAN_POINT('Ctrl Pts',(-48.706329375,31.9791666734946,-13.0508216223155));
#17278=CARTESIAN_POINT('Ctrl Pts',(-42.1809185638422,31.7708333401613,-24.3531646875));
#17279=CARTESIAN_POINT('Ctrl Pts',(-35.6555077526845,31.562500006828,-35.6555077526845));
#17280=CARTESIAN_POINT('Ctrl Pts',(-24.3531646875,31.3541666734946,-42.1809185638423));
#17281=CARTESIAN_POINT('Ctrl Pts',(-13.0508216223155,31.1458333401613,-48.706329375));
#17282=CARTESIAN_POINT('Ctrl Pts',(1.59157945007855E-14,30.937500006828,
-48.706329375));
#17283=CARTESIAN_POINT('Ctrl Pts',(13.0508216223155,30.7291666734946,-48.706329375));
#17284=CARTESIAN_POINT('Ctrl Pts',(24.3531646875,30.5208333401613,-42.1809185638422));
#17285=CARTESIAN_POINT('Ctrl Pts',(35.6555077526845,30.312500006828,-35.6555077526845));
#17286=CARTESIAN_POINT('Ctrl Pts',(42.1809185638422,30.1041666734946,-24.3531646875));
#17287=CARTESIAN_POINT('Ctrl Pts',(48.706329375,29.8958333401613,-13.0508216223155));
#17288=CARTESIAN_POINT('Ctrl Pts',(48.706329375,29.687500006828,1.293339198242E-14));
#17289=CARTESIAN_POINT('Ctrl Pts',(48.706329375,29.4791666734946,13.0508216223155));
#17290=CARTESIAN_POINT('Ctrl Pts',(42.1809185638422,29.2708333401613,24.3531646875));
#17291=CARTESIAN_POINT('Ctrl Pts',(35.6555077526845,29.062500006828,35.6555077526845));
#17292=CARTESIAN_POINT('Ctrl Pts',(24.3531646875,28.8541666734946,42.1809185638422));
#17293=CARTESIAN_POINT('Ctrl Pts',(13.0508216223155,28.6458333401613,48.706329375));
#17294=CARTESIAN_POINT('Ctrl Pts',(-9.95098946405443E-15,28.437500006828,
48.706329375));
#17295=CARTESIAN_POINT('Ctrl Pts',(-13.0508216223155,28.2291666734946,48.706329375));
#17296=CARTESIAN_POINT('Ctrl Pts',(-24.3531646875,28.0208333401613,42.1809185638423));
#17297=CARTESIAN_POINT('Ctrl Pts',(-35.6555077526845,27.812500006828,35.6555077526845));
#17298=CARTESIAN_POINT('Ctrl Pts',(-42.1809185638422,27.6041666734946,24.3531646875));
#17299=CARTESIAN_POINT('Ctrl Pts',(-48.706329375,27.3958333401613,13.0508216223155));
#17300=CARTESIAN_POINT('Ctrl Pts',(-48.706329375,27.187500006828,-1.8898197019151E-14));
#17301=CARTESIAN_POINT('Origin',(-4513.80899805517,7988.28355096199,-4.33048917330144));
#17302=CARTESIAN_POINT('Ctrl Pts',(2.6308221862305,34.3301917962911,-45.9247076705387));
#17303=CARTESIAN_POINT('Ctrl Pts',(2.84524895812375,34.5752225485839,-46.3431776594255));
#17304=CARTESIAN_POINT('Ctrl Pts',(3.01791080422552,34.8332332645741,-46.7840354195864));
#17305=CARTESIAN_POINT('Ctrl Pts',(3.29117134372613,35.3512038226748,-47.6711182012495));
#17306=CARTESIAN_POINT('Ctrl Pts',(3.39456512521887,35.6166989155655,-48.1267924420204));
#17307=CARTESIAN_POINT('Ctrl Pts',(3.4681498498003,35.8816082987783,-48.5826971030357));
#17308=CARTESIAN_POINT('Ctrl Pts',(-46.,55.6250000136559,0.));
#17309=CARTESIAN_POINT('Ctrl Pts',(-46.,55.4166666803226,-12.3256628518316));
#17310=CARTESIAN_POINT('Ctrl Pts',(-39.8371685740842,55.2083333469893,-23.));
#17311=CARTESIAN_POINT('Ctrl Pts',(-33.6743371481684,55.0000000136559,-33.6743371481684));
#17312=CARTESIAN_POINT('Ctrl Pts',(-23.,54.7916666803226,-39.8371685740842));
#17313=CARTESIAN_POINT('Ctrl Pts',(-12.3256628518317,54.5833333469893,-46.));
#17314=CARTESIAN_POINT('Ctrl Pts',(-2.81668763803891E-15,54.3750000136559,
-46.));
#17315=CARTESIAN_POINT('Ctrl Pts',(12.3256628518316,54.1666666803226,-46.));
#17316=CARTESIAN_POINT('Ctrl Pts',(23.,53.9583333469893,-39.8371685740842));
#17317=CARTESIAN_POINT('Ctrl Pts',(33.6743371481683,53.7500000136559,-33.6743371481684));
#17318=CARTESIAN_POINT('Ctrl Pts',(39.8371685740842,53.5416666803226,-23.));
#17319=CARTESIAN_POINT('Ctrl Pts',(46.,53.3333333469893,-12.3256628518317));
#17320=CARTESIAN_POINT('Ctrl Pts',(46.,53.1250000136559,-5.63337527607782E-15));
#17321=CARTESIAN_POINT('Ctrl Pts',(46.,52.9166666803226,12.3256628518316));
#17322=CARTESIAN_POINT('Ctrl Pts',(39.8371685740842,52.7083333469893,23.));
#17323=CARTESIAN_POINT('Ctrl Pts',(33.6743371481684,52.5000000136559,33.6743371481683));
#17324=CARTESIAN_POINT('Ctrl Pts',(23.,52.2916666803226,39.8371685740842));
#17325=CARTESIAN_POINT('Ctrl Pts',(12.3256628518317,52.0833333469893,46.));
#17326=CARTESIAN_POINT('Ctrl Pts',(8.45006291411674E-15,51.8750000136559,
46.));
#17327=CARTESIAN_POINT('Ctrl Pts',(-12.3256628518316,51.6666666803226,46.));
#17328=CARTESIAN_POINT('Ctrl Pts',(-23.,51.4583333469893,39.8371685740842));
#17329=CARTESIAN_POINT('Ctrl Pts',(-33.6743371481683,51.2500000136559,33.6743371481684));
#17330=CARTESIAN_POINT('Ctrl Pts',(-39.8371685740842,51.0416666803226,23.));
#17331=CARTESIAN_POINT('Ctrl Pts',(-46.,50.8333333469893,12.3256628518317));
#17332=CARTESIAN_POINT('Ctrl Pts',(-46.,50.6250000136559,0.));
#17333=CARTESIAN_POINT('Ctrl Pts',(-46.,50.4166666803226,-12.3256628518316));
#17334=CARTESIAN_POINT('Ctrl Pts',(-39.8371685740842,50.2083333469893,-23.));
#17335=CARTESIAN_POINT('Ctrl Pts',(-33.6743371481684,50.0000000136559,-33.6743371481684));
#17336=CARTESIAN_POINT('Ctrl Pts',(-23.,49.7916666803226,-39.8371685740842));
#17337=CARTESIAN_POINT('Ctrl Pts',(-12.3256628518317,49.5833333469893,-46.));
#17338=CARTESIAN_POINT('Ctrl Pts',(-2.81668763803891E-15,49.3750000136559,
-46.));
#17339=CARTESIAN_POINT('Ctrl Pts',(12.3256628518316,49.1666666803226,-46.));
#17340=CARTESIAN_POINT('Ctrl Pts',(23.,48.9583333469893,-39.8371685740842));
#17341=CARTESIAN_POINT('Ctrl Pts',(33.6743371481683,48.7500000136559,-33.6743371481684));
#17342=CARTESIAN_POINT('Ctrl Pts',(39.8371685740842,48.5416666803226,-23.));
#17343=CARTESIAN_POINT('Ctrl Pts',(46.,48.3333333469893,-12.3256628518317));
#17344=CARTESIAN_POINT('Ctrl Pts',(46.,48.1250000136559,-5.63337527607782E-15));
#17345=CARTESIAN_POINT('Ctrl Pts',(46.,47.9166666803226,12.3256628518316));
#17346=CARTESIAN_POINT('Ctrl Pts',(39.8371685740842,47.7083333469893,23.));
#17347=CARTESIAN_POINT('Ctrl Pts',(33.6743371481684,47.5000000136559,33.6743371481683));
#17348=CARTESIAN_POINT('Ctrl Pts',(23.,47.2916666803226,39.8371685740842));
#17349=CARTESIAN_POINT('Ctrl Pts',(12.3256628518317,47.0833333469893,46.));
#17350=CARTESIAN_POINT('Ctrl Pts',(8.45006291411674E-15,46.8750000136559,
46.));
#17351=CARTESIAN_POINT('Ctrl Pts',(-12.3256628518316,46.6666666803226,46.));
#17352=CARTESIAN_POINT('Ctrl Pts',(-23.,46.4583333469893,39.8371685740842));
#17353=CARTESIAN_POINT('Ctrl Pts',(-33.6743371481683,46.2500000136559,33.6743371481684));
#17354=CARTESIAN_POINT('Ctrl Pts',(-39.8371685740842,46.0416666803226,23.));
#17355=CARTESIAN_POINT('Ctrl Pts',(-46.,45.8333333469892,12.3256628518317));
#17356=CARTESIAN_POINT('Ctrl Pts',(-46.,45.6250000136559,0.));
#17357=CARTESIAN_POINT('Ctrl Pts',(-46.,45.4166666803226,-12.3256628518316));
#17358=CARTESIAN_POINT('Ctrl Pts',(-39.8371685740842,45.2083333469893,-23.));
#17359=CARTESIAN_POINT('Ctrl Pts',(-33.6743371481684,45.0000000136559,-33.6743371481684));
#17360=CARTESIAN_POINT('Ctrl Pts',(-23.,44.7916666803226,-39.8371685740842));
#17361=CARTESIAN_POINT('Ctrl Pts',(-12.3256628518317,44.5833333469893,-46.));
#17362=CARTESIAN_POINT('Ctrl Pts',(-2.81668763803891E-15,44.3750000136559,
-46.));
#17363=CARTESIAN_POINT('Ctrl Pts',(12.3256628518316,44.1666666803226,-46.));
#17364=CARTESIAN_POINT('Ctrl Pts',(23.,43.9583333469893,-39.8371685740842));
#17365=CARTESIAN_POINT('Ctrl Pts',(33.6743371481683,43.7500000136559,-33.6743371481684));
#17366=CARTESIAN_POINT('Ctrl Pts',(39.8371685740842,43.5416666803226,-23.));
#17367=CARTESIAN_POINT('Ctrl Pts',(46.,43.3333333469893,-12.3256628518317));
#17368=CARTESIAN_POINT('Ctrl Pts',(46.,43.1250000136559,-5.63337527607782E-15));
#17369=CARTESIAN_POINT('Ctrl Pts',(46.,42.9166666803226,12.3256628518316));
#17370=CARTESIAN_POINT('Ctrl Pts',(39.8371685740842,42.7083333469893,23.));
#17371=CARTESIAN_POINT('Ctrl Pts',(33.6743371481684,42.5000000136559,33.6743371481683));
#17372=CARTESIAN_POINT('Ctrl Pts',(23.,42.2916666803226,39.8371685740842));
#17373=CARTESIAN_POINT('Ctrl Pts',(12.3256628518317,42.0833333469893,46.));
#17374=CARTESIAN_POINT('Ctrl Pts',(8.45006291411674E-15,41.8750000136559,
46.));
#17375=CARTESIAN_POINT('Ctrl Pts',(-12.3256628518316,41.6666666803226,46.));
#17376=CARTESIAN_POINT('Ctrl Pts',(-23.,41.4583333469893,39.8371685740842));
#17377=CARTESIAN_POINT('Ctrl Pts',(-33.6743371481683,41.2500000136559,33.6743371481684));
#17378=CARTESIAN_POINT('Ctrl Pts',(-39.8371685740842,41.0416666803226,23.));
#17379=CARTESIAN_POINT('Ctrl Pts',(-46.,40.8333333469893,12.3256628518317));
#17380=CARTESIAN_POINT('Ctrl Pts',(-46.,40.6250000136559,0.));
#17381=CARTESIAN_POINT('Ctrl Pts',(-46.,40.4166666803226,-12.3256628518316));
#17382=CARTESIAN_POINT('Ctrl Pts',(-39.8371685740842,40.2083333469893,-23.));
#17383=CARTESIAN_POINT('Ctrl Pts',(-33.6743371481684,40.0000000136559,-33.6743371481684));
#17384=CARTESIAN_POINT('Ctrl Pts',(-23.,39.7916666803226,-39.8371685740842));
#17385=CARTESIAN_POINT('Ctrl Pts',(-12.3256628518317,39.5833333469893,-46.));
#17386=CARTESIAN_POINT('Ctrl Pts',(-2.81668763803891E-15,39.3750000136559,
-46.));
#17387=CARTESIAN_POINT('Ctrl Pts',(12.3256628518316,39.1666666803226,-46.));
#17388=CARTESIAN_POINT('Ctrl Pts',(23.,38.9583333469893,-39.8371685740842));
#17389=CARTESIAN_POINT('Ctrl Pts',(33.6743371481683,38.7500000136559,-33.6743371481684));
#17390=CARTESIAN_POINT('Ctrl Pts',(39.8371685740842,38.5416666803226,-23.));
#17391=CARTESIAN_POINT('Ctrl Pts',(46.,38.3333333469893,-12.3256628518317));
#17392=CARTESIAN_POINT('Ctrl Pts',(46.,38.1250000136559,-5.63337527607782E-15));
#17393=CARTESIAN_POINT('Ctrl Pts',(46.,37.9166666803226,12.3256628518316));
#17394=CARTESIAN_POINT('Ctrl Pts',(39.8371685740842,37.7083333469893,23.));
#17395=CARTESIAN_POINT('Ctrl Pts',(33.6743371481684,37.5000000136559,33.6743371481683));
#17396=CARTESIAN_POINT('Ctrl Pts',(23.,37.2916666803226,39.8371685740842));
#17397=CARTESIAN_POINT('Ctrl Pts',(12.3256628518317,37.0833333469893,46.));
#17398=CARTESIAN_POINT('Ctrl Pts',(8.45006291411674E-15,36.8750000136559,
46.));
#17399=CARTESIAN_POINT('Ctrl Pts',(-12.3256628518316,36.6666666803226,46.));
#17400=CARTESIAN_POINT('Ctrl Pts',(-23.,36.4583333469893,39.8371685740842));
#17401=CARTESIAN_POINT('Ctrl Pts',(-33.6743371481683,36.2500000136559,33.6743371481684));
#17402=CARTESIAN_POINT('Ctrl Pts',(-39.8371685740842,36.0416666803226,23.));
#17403=CARTESIAN_POINT('Ctrl Pts',(-46.,35.8333333469893,12.3256628518317));
#17404=CARTESIAN_POINT('Ctrl Pts',(-46.,35.6250000136559,0.));
#17405=CARTESIAN_POINT('Ctrl Pts',(-46.,35.4166666803226,-12.3256628518316));
#17406=CARTESIAN_POINT('Ctrl Pts',(-39.8371685740842,35.2083333469893,-23.));
#17407=CARTESIAN_POINT('Ctrl Pts',(-33.6743371481684,35.0000000136559,-33.6743371481684));
#17408=CARTESIAN_POINT('Ctrl Pts',(-23.,34.7916666803226,-39.8371685740842));
#17409=CARTESIAN_POINT('Ctrl Pts',(-12.3256628518317,34.5833333469893,-46.));
#17410=CARTESIAN_POINT('Ctrl Pts',(-2.81668763803891E-15,34.3750000136559,
-46.));
#17411=CARTESIAN_POINT('Ctrl Pts',(12.3256628518316,34.1666666803226,-46.));
#17412=CARTESIAN_POINT('Ctrl Pts',(23.,33.9583333469893,-39.8371685740842));
#17413=CARTESIAN_POINT('Ctrl Pts',(33.6743371481683,33.7500000136559,-33.6743371481684));
#17414=CARTESIAN_POINT('Ctrl Pts',(39.8371685740842,33.5416666803226,-23.));
#17415=CARTESIAN_POINT('Ctrl Pts',(46.,33.3333333469893,-12.3256628518317));
#17416=CARTESIAN_POINT('Ctrl Pts',(46.,33.1250000136559,-5.63337527607782E-15));
#17417=CARTESIAN_POINT('Ctrl Pts',(46.,32.9166666803226,12.3256628518316));
#17418=CARTESIAN_POINT('Ctrl Pts',(39.8371685740842,32.7083333469893,23.));
#17419=CARTESIAN_POINT('Ctrl Pts',(33.6743371481684,32.5000000136559,33.6743371481683));
#17420=CARTESIAN_POINT('Ctrl Pts',(23.,32.2916666803226,39.8371685740842));
#17421=CARTESIAN_POINT('Ctrl Pts',(12.3256628518317,32.0833333469893,46.));
#17422=CARTESIAN_POINT('Ctrl Pts',(8.45006291411674E-15,31.8750000136559,
46.));
#17423=CARTESIAN_POINT('Ctrl Pts',(-12.3256628518316,31.6666666803226,46.));
#17424=CARTESIAN_POINT('Ctrl Pts',(-23.,31.4583333469893,39.8371685740842));
#17425=CARTESIAN_POINT('Ctrl Pts',(-33.6743371481683,31.2500000136559,33.6743371481684));
#17426=CARTESIAN_POINT('Ctrl Pts',(-39.8371685740842,31.0416666803226,23.));
#17427=CARTESIAN_POINT('Ctrl Pts',(-46.,30.8333333469893,12.3256628518317));
#17428=CARTESIAN_POINT('Ctrl Pts',(-46.,30.6250000136559,0.));
#17429=CARTESIAN_POINT('Ctrl Pts',(-46.,30.4166666803226,-12.3256628518316));
#17430=CARTESIAN_POINT('Ctrl Pts',(-39.8371685740842,30.2083333469893,-23.));
#17431=CARTESIAN_POINT('Ctrl Pts',(-33.6743371481684,30.0000000136559,-33.6743371481684));
#17432=CARTESIAN_POINT('Ctrl Pts',(-23.,29.7916666803226,-39.8371685740842));
#17433=CARTESIAN_POINT('Ctrl Pts',(-12.3256628518317,29.5833333469893,-46.));
#17434=CARTESIAN_POINT('Ctrl Pts',(-2.81668763803891E-15,29.3750000136559,
-46.));
#17435=CARTESIAN_POINT('Ctrl Pts',(12.3256628518316,29.1666666803226,-46.));
#17436=CARTESIAN_POINT('Ctrl Pts',(23.,28.9583333469893,-39.8371685740842));
#17437=CARTESIAN_POINT('Ctrl Pts',(33.6743371481683,28.7500000136559,-33.6743371481684));
#17438=CARTESIAN_POINT('Ctrl Pts',(39.8371685740842,28.5416666803226,-23.));
#17439=CARTESIAN_POINT('Ctrl Pts',(46.,28.3333333469893,-12.3256628518317));
#17440=CARTESIAN_POINT('Ctrl Pts',(46.,28.1250000136559,-5.63337527607782E-15));
#17441=CARTESIAN_POINT('Ctrl Pts',(46.,27.9166666803226,12.3256628518316));
#17442=CARTESIAN_POINT('Ctrl Pts',(39.8371685740842,27.7083333469893,23.));
#17443=CARTESIAN_POINT('Ctrl Pts',(33.6743371481684,27.5000000136559,33.6743371481683));
#17444=CARTESIAN_POINT('Ctrl Pts',(23.,27.2916666803226,39.8371685740842));
#17445=CARTESIAN_POINT('Ctrl Pts',(12.3256628518317,27.0833333469893,46.));
#17446=CARTESIAN_POINT('Ctrl Pts',(8.45006291411674E-15,26.8750000136559,
46.));
#17447=CARTESIAN_POINT('Ctrl Pts',(-12.3256628518316,26.6666666803226,46.));
#17448=CARTESIAN_POINT('Ctrl Pts',(-23.,26.4583333469893,39.8371685740842));
#17449=CARTESIAN_POINT('Ctrl Pts',(-33.6743371481683,26.2500000136559,33.6743371481684));
#17450=CARTESIAN_POINT('Ctrl Pts',(-39.8371685740842,26.0416666803226,23.));
#17451=CARTESIAN_POINT('Ctrl Pts',(-46.,25.8333333469893,12.3256628518317));
#17452=CARTESIAN_POINT('Ctrl Pts',(-46.,25.6250000136559,0.));
#17453=CARTESIAN_POINT('Ctrl Pts',(-48.706329375,57.187500006828,-1.8898197019151E-14));
#17454=CARTESIAN_POINT('Ctrl Pts',(-48.706329375,56.9791666734946,-13.0508216223155));
#17455=CARTESIAN_POINT('Ctrl Pts',(-42.1809185638422,56.7708333401613,-24.3531646875));
#17456=CARTESIAN_POINT('Ctrl Pts',(-35.6555077526845,56.562500006828,-35.6555077526845));
#17457=CARTESIAN_POINT('Ctrl Pts',(-24.3531646875,56.3541666734946,-42.1809185638423));
#17458=CARTESIAN_POINT('Ctrl Pts',(-13.0508216223155,56.1458333401613,-48.706329375));
#17459=CARTESIAN_POINT('Ctrl Pts',(1.59157945007855E-14,55.937500006828,
-48.706329375));
#17460=CARTESIAN_POINT('Ctrl Pts',(13.0508216223155,55.7291666734946,-48.706329375));
#17461=CARTESIAN_POINT('Ctrl Pts',(24.3531646875,55.5208333401613,-42.1809185638422));
#17462=CARTESIAN_POINT('Ctrl Pts',(35.6555077526845,55.312500006828,-35.6555077526845));
#17463=CARTESIAN_POINT('Ctrl Pts',(42.1809185638422,55.1041666734946,-24.3531646875));
#17464=CARTESIAN_POINT('Ctrl Pts',(48.706329375,54.8958333401613,-13.0508216223155));
#17465=CARTESIAN_POINT('Ctrl Pts',(48.706329375,54.687500006828,1.293339198242E-14));
#17466=CARTESIAN_POINT('Ctrl Pts',(48.706329375,54.4791666734946,13.0508216223155));
#17467=CARTESIAN_POINT('Ctrl Pts',(42.1809185638422,54.2708333401613,24.3531646875));
#17468=CARTESIAN_POINT('Ctrl Pts',(35.6555077526845,54.062500006828,35.6555077526845));
#17469=CARTESIAN_POINT('Ctrl Pts',(24.3531646875,53.8541666734946,42.1809185638422));
#17470=CARTESIAN_POINT('Ctrl Pts',(13.0508216223155,53.6458333401613,48.706329375));
#17471=CARTESIAN_POINT('Ctrl Pts',(-9.95098946405443E-15,53.437500006828,
48.706329375));
#17472=CARTESIAN_POINT('Ctrl Pts',(-13.0508216223155,53.2291666734946,48.706329375));
#17473=CARTESIAN_POINT('Ctrl Pts',(-24.3531646875,53.0208333401613,42.1809185638423));
#17474=CARTESIAN_POINT('Ctrl Pts',(-35.6555077526845,52.812500006828,35.6555077526845));
#17475=CARTESIAN_POINT('Ctrl Pts',(-42.1809185638422,52.6041666734946,24.3531646875));
#17476=CARTESIAN_POINT('Ctrl Pts',(-48.706329375,52.3958333401613,13.0508216223155));
#17477=CARTESIAN_POINT('Ctrl Pts',(-48.706329375,52.187500006828,-1.8898197019151E-14));
#17478=CARTESIAN_POINT('Ctrl Pts',(-48.706329375,51.9791666734946,-13.0508216223155));
#17479=CARTESIAN_POINT('Ctrl Pts',(-42.1809185638422,51.7708333401613,-24.3531646875));
#17480=CARTESIAN_POINT('Ctrl Pts',(-35.6555077526845,51.562500006828,-35.6555077526845));
#17481=CARTESIAN_POINT('Ctrl Pts',(-24.3531646875,51.3541666734946,-42.1809185638423));
#17482=CARTESIAN_POINT('Ctrl Pts',(-13.0508216223155,51.1458333401613,-48.706329375));
#17483=CARTESIAN_POINT('Ctrl Pts',(1.59157945007855E-14,50.937500006828,
-48.706329375));
#17484=CARTESIAN_POINT('Ctrl Pts',(13.0508216223155,50.7291666734946,-48.706329375));
#17485=CARTESIAN_POINT('Ctrl Pts',(24.3531646875,50.5208333401613,-42.1809185638422));
#17486=CARTESIAN_POINT('Ctrl Pts',(35.6555077526845,50.312500006828,-35.6555077526845));
#17487=CARTESIAN_POINT('Ctrl Pts',(42.1809185638422,50.1041666734946,-24.3531646875));
#17488=CARTESIAN_POINT('Ctrl Pts',(48.706329375,49.8958333401613,-13.0508216223155));
#17489=CARTESIAN_POINT('Ctrl Pts',(48.706329375,49.687500006828,1.293339198242E-14));
#17490=CARTESIAN_POINT('Ctrl Pts',(48.706329375,49.4791666734946,13.0508216223155));
#17491=CARTESIAN_POINT('Ctrl Pts',(42.1809185638422,49.2708333401613,24.3531646875));
#17492=CARTESIAN_POINT('Ctrl Pts',(35.6555077526845,49.062500006828,35.6555077526845));
#17493=CARTESIAN_POINT('Ctrl Pts',(24.3531646875,48.8541666734946,42.1809185638422));
#17494=CARTESIAN_POINT('Ctrl Pts',(13.0508216223155,48.6458333401613,48.706329375));
#17495=CARTESIAN_POINT('Ctrl Pts',(-9.95098946405443E-15,48.437500006828,
48.706329375));
#17496=CARTESIAN_POINT('Ctrl Pts',(-13.0508216223155,48.2291666734946,48.706329375));
#17497=CARTESIAN_POINT('Ctrl Pts',(-24.3531646875,48.0208333401613,42.1809185638423));
#17498=CARTESIAN_POINT('Ctrl Pts',(-35.6555077526845,47.812500006828,35.6555077526845));
#17499=CARTESIAN_POINT('Ctrl Pts',(-42.1809185638422,47.6041666734946,24.3531646875));
#17500=CARTESIAN_POINT('Ctrl Pts',(-48.706329375,47.3958333401613,13.0508216223155));
#17501=CARTESIAN_POINT('Ctrl Pts',(-48.706329375,47.187500006828,-1.8898197019151E-14));
#17502=CARTESIAN_POINT('Ctrl Pts',(-48.706329375,46.9791666734946,-13.0508216223155));
#17503=CARTESIAN_POINT('Ctrl Pts',(-42.1809185638422,46.7708333401613,-24.3531646875));
#17504=CARTESIAN_POINT('Ctrl Pts',(-35.6555077526845,46.562500006828,-35.6555077526845));
#17505=CARTESIAN_POINT('Ctrl Pts',(-24.3531646875,46.3541666734946,-42.1809185638423));
#17506=CARTESIAN_POINT('Ctrl Pts',(-13.0508216223155,46.1458333401613,-48.706329375));
#17507=CARTESIAN_POINT('Ctrl Pts',(1.59157945007855E-14,45.937500006828,
-48.706329375));
#17508=CARTESIAN_POINT('Ctrl Pts',(13.0508216223155,45.7291666734946,-48.706329375));
#17509=CARTESIAN_POINT('Ctrl Pts',(24.3531646875,45.5208333401613,-42.1809185638422));
#17510=CARTESIAN_POINT('Ctrl Pts',(35.6555077526845,45.312500006828,-35.6555077526845));
#17511=CARTESIAN_POINT('Ctrl Pts',(42.1809185638422,45.1041666734946,-24.3531646875));
#17512=CARTESIAN_POINT('Ctrl Pts',(48.706329375,44.8958333401613,-13.0508216223155));
#17513=CARTESIAN_POINT('Ctrl Pts',(48.706329375,44.687500006828,1.293339198242E-14));
#17514=CARTESIAN_POINT('Ctrl Pts',(48.706329375,44.4791666734946,13.0508216223155));
#17515=CARTESIAN_POINT('Ctrl Pts',(42.1809185638422,44.2708333401613,24.3531646875));
#17516=CARTESIAN_POINT('Ctrl Pts',(35.6555077526845,44.062500006828,35.6555077526845));
#17517=CARTESIAN_POINT('Ctrl Pts',(24.3531646875,43.8541666734946,42.1809185638422));
#17518=CARTESIAN_POINT('Ctrl Pts',(13.0508216223155,43.6458333401613,48.706329375));
#17519=CARTESIAN_POINT('Ctrl Pts',(-9.95098946405443E-15,43.437500006828,
48.706329375));
#17520=CARTESIAN_POINT('Ctrl Pts',(-13.0508216223155,43.2291666734946,48.706329375));
#17521=CARTESIAN_POINT('Ctrl Pts',(-24.3531646875,43.0208333401613,42.1809185638423));
#17522=CARTESIAN_POINT('Ctrl Pts',(-35.6555077526845,42.812500006828,35.6555077526845));
#17523=CARTESIAN_POINT('Ctrl Pts',(-42.1809185638422,42.6041666734946,24.3531646875));
#17524=CARTESIAN_POINT('Ctrl Pts',(-48.706329375,42.3958333401613,13.0508216223155));
#17525=CARTESIAN_POINT('Ctrl Pts',(-48.706329375,42.187500006828,-1.8898197019151E-14));
#17526=CARTESIAN_POINT('Ctrl Pts',(-48.706329375,41.9791666734946,-13.0508216223155));
#17527=CARTESIAN_POINT('Ctrl Pts',(-42.1809185638422,41.7708333401613,-24.3531646875));
#17528=CARTESIAN_POINT('Ctrl Pts',(-35.6555077526845,41.562500006828,-35.6555077526845));
#17529=CARTESIAN_POINT('Ctrl Pts',(-24.3531646875,41.3541666734946,-42.1809185638423));
#17530=CARTESIAN_POINT('Ctrl Pts',(-13.0508216223155,41.1458333401613,-48.706329375));
#17531=CARTESIAN_POINT('Ctrl Pts',(1.59157945007855E-14,40.937500006828,
-48.706329375));
#17532=CARTESIAN_POINT('Ctrl Pts',(13.0508216223155,40.7291666734946,-48.706329375));
#17533=CARTESIAN_POINT('Ctrl Pts',(24.3531646875,40.5208333401613,-42.1809185638422));
#17534=CARTESIAN_POINT('Ctrl Pts',(35.6555077526845,40.312500006828,-35.6555077526845));
#17535=CARTESIAN_POINT('Ctrl Pts',(42.1809185638422,40.1041666734946,-24.3531646875));
#17536=CARTESIAN_POINT('Ctrl Pts',(48.706329375,39.8958333401613,-13.0508216223155));
#17537=CARTESIAN_POINT('Ctrl Pts',(48.706329375,39.687500006828,1.293339198242E-14));
#17538=CARTESIAN_POINT('Ctrl Pts',(48.706329375,39.4791666734946,13.0508216223155));
#17539=CARTESIAN_POINT('Ctrl Pts',(42.1809185638422,39.2708333401613,24.3531646875));
#17540=CARTESIAN_POINT('Ctrl Pts',(35.6555077526845,39.062500006828,35.6555077526845));
#17541=CARTESIAN_POINT('Ctrl Pts',(24.3531646875,38.8541666734946,42.1809185638422));
#17542=CARTESIAN_POINT('Ctrl Pts',(13.0508216223155,38.6458333401613,48.706329375));
#17543=CARTESIAN_POINT('Ctrl Pts',(-9.95098946405443E-15,38.437500006828,
48.706329375));
#17544=CARTESIAN_POINT('Ctrl Pts',(-13.0508216223155,38.2291666734946,48.706329375));
#17545=CARTESIAN_POINT('Ctrl Pts',(-24.3531646875,38.0208333401613,42.1809185638423));
#17546=CARTESIAN_POINT('Ctrl Pts',(-35.6555077526845,37.812500006828,35.6555077526845));
#17547=CARTESIAN_POINT('Ctrl Pts',(-42.1809185638422,37.6041666734946,24.3531646875));
#17548=CARTESIAN_POINT('Ctrl Pts',(-48.706329375,37.3958333401613,13.0508216223155));
#17549=CARTESIAN_POINT('Ctrl Pts',(-48.706329375,37.187500006828,-1.8898197019151E-14));
#17550=CARTESIAN_POINT('Ctrl Pts',(-48.706329375,36.9791666734946,-13.0508216223155));
#17551=CARTESIAN_POINT('Ctrl Pts',(-42.1809185638422,36.7708333401613,-24.3531646875));
#17552=CARTESIAN_POINT('Ctrl Pts',(-35.6555077526845,36.562500006828,-35.6555077526845));
#17553=CARTESIAN_POINT('Ctrl Pts',(-24.3531646875,36.3541666734946,-42.1809185638423));
#17554=CARTESIAN_POINT('Ctrl Pts',(-13.0508216223155,36.1458333401613,-48.706329375));
#17555=CARTESIAN_POINT('Ctrl Pts',(1.59157945007855E-14,35.937500006828,
-48.706329375));
#17556=CARTESIAN_POINT('Ctrl Pts',(13.0508216223155,35.7291666734946,-48.706329375));
#17557=CARTESIAN_POINT('Ctrl Pts',(24.3531646875,35.5208333401613,-42.1809185638422));
#17558=CARTESIAN_POINT('Ctrl Pts',(35.6555077526845,35.312500006828,-35.6555077526845));
#17559=CARTESIAN_POINT('Ctrl Pts',(42.1809185638422,35.1041666734946,-24.3531646875));
#17560=CARTESIAN_POINT('Ctrl Pts',(48.706329375,34.8958333401613,-13.0508216223155));
#17561=CARTESIAN_POINT('Ctrl Pts',(48.706329375,34.687500006828,1.293339198242E-14));
#17562=CARTESIAN_POINT('Ctrl Pts',(48.706329375,34.4791666734946,13.0508216223155));
#17563=CARTESIAN_POINT('Ctrl Pts',(42.1809185638422,34.2708333401613,24.3531646875));
#17564=CARTESIAN_POINT('Ctrl Pts',(35.6555077526845,34.062500006828,35.6555077526845));
#17565=CARTESIAN_POINT('Ctrl Pts',(24.3531646875,33.8541666734946,42.1809185638422));
#17566=CARTESIAN_POINT('Ctrl Pts',(13.0508216223155,33.6458333401613,48.706329375));
#17567=CARTESIAN_POINT('Ctrl Pts',(-9.95098946405443E-15,33.437500006828,
48.706329375));
#17568=CARTESIAN_POINT('Ctrl Pts',(-13.0508216223155,33.2291666734946,48.706329375));
#17569=CARTESIAN_POINT('Ctrl Pts',(-24.3531646875,33.0208333401613,42.1809185638423));
#17570=CARTESIAN_POINT('Ctrl Pts',(-35.6555077526845,32.812500006828,35.6555077526845));
#17571=CARTESIAN_POINT('Ctrl Pts',(-42.1809185638422,32.6041666734946,24.3531646875));
#17572=CARTESIAN_POINT('Ctrl Pts',(-48.706329375,32.3958333401613,13.0508216223155));
#17573=CARTESIAN_POINT('Ctrl Pts',(-48.706329375,32.187500006828,-1.8898197019151E-14));
#17574=CARTESIAN_POINT('Ctrl Pts',(-48.706329375,31.9791666734946,-13.0508216223155));
#17575=CARTESIAN_POINT('Ctrl Pts',(-42.1809185638422,31.7708333401613,-24.3531646875));
#17576=CARTESIAN_POINT('Ctrl Pts',(-35.6555077526845,31.562500006828,-35.6555077526845));
#17577=CARTESIAN_POINT('Ctrl Pts',(-24.3531646875,31.3541666734946,-42.1809185638423));
#17578=CARTESIAN_POINT('Ctrl Pts',(-13.0508216223155,31.1458333401613,-48.706329375));
#17579=CARTESIAN_POINT('Ctrl Pts',(1.59157945007855E-14,30.937500006828,
-48.706329375));
#17580=CARTESIAN_POINT('Ctrl Pts',(13.0508216223155,30.7291666734946,-48.706329375));
#17581=CARTESIAN_POINT('Ctrl Pts',(24.3531646875,30.5208333401613,-42.1809185638422));
#17582=CARTESIAN_POINT('Ctrl Pts',(35.6555077526845,30.312500006828,-35.6555077526845));
#17583=CARTESIAN_POINT('Ctrl Pts',(42.1809185638422,30.1041666734946,-24.3531646875));
#17584=CARTESIAN_POINT('Ctrl Pts',(48.706329375,29.8958333401613,-13.0508216223155));
#17585=CARTESIAN_POINT('Ctrl Pts',(48.706329375,29.687500006828,1.293339198242E-14));
#17586=CARTESIAN_POINT('Ctrl Pts',(48.706329375,29.4791666734946,13.0508216223155));
#17587=CARTESIAN_POINT('Ctrl Pts',(42.1809185638422,29.2708333401613,24.3531646875));
#17588=CARTESIAN_POINT('Ctrl Pts',(35.6555077526845,29.062500006828,35.6555077526845));
#17589=CARTESIAN_POINT('Ctrl Pts',(24.3531646875,28.8541666734946,42.1809185638422));
#17590=CARTESIAN_POINT('Ctrl Pts',(13.0508216223155,28.6458333401613,48.706329375));
#17591=CARTESIAN_POINT('Ctrl Pts',(-9.95098946405443E-15,28.437500006828,
48.706329375));
#17592=CARTESIAN_POINT('Ctrl Pts',(-13.0508216223155,28.2291666734946,48.706329375));
#17593=CARTESIAN_POINT('Ctrl Pts',(-24.3531646875,28.0208333401613,42.1809185638423));
#17594=CARTESIAN_POINT('Ctrl Pts',(-35.6555077526845,27.812500006828,35.6555077526845));
#17595=CARTESIAN_POINT('Ctrl Pts',(-42.1809185638422,27.6041666734946,24.3531646875));
#17596=CARTESIAN_POINT('Ctrl Pts',(-48.706329375,27.3958333401613,13.0508216223155));
#17597=CARTESIAN_POINT('Ctrl Pts',(-48.706329375,27.187500006828,-1.8898197019151E-14));
#17598=CARTESIAN_POINT('',(-2.14849279754675,33.4030003256338,48.658920044375));
#17599=CARTESIAN_POINT('',(-48.5725845633798,32.2456516907297,3.60701400320324));
#17600=CARTESIAN_POINT('Ctrl Pts',(-2.14849279754675,33.4030003256338,48.658920044375));
#17601=CARTESIAN_POINT('Ctrl Pts',(-14.0425623011786,33.2108861594244,48.1337476270921));
#17602=CARTESIAN_POINT('Ctrl Pts',(-24.3531646875,33.0208333401613,42.1809185638423));
#17603=CARTESIAN_POINT('Ctrl Pts',(-35.6555077526845,32.812500006828,35.6555077526845));
#17604=CARTESIAN_POINT('Ctrl Pts',(-42.1809185638422,32.6041666734946,24.3531646875));
#17605=CARTESIAN_POINT('Ctrl Pts',(-47.7480251419552,32.4264286116308,14.7106532430575));
#17606=CARTESIAN_POINT('Ctrl Pts',(-48.5725845633798,32.2456516907297,3.60701400320324));
#17607=CARTESIAN_POINT('Ctrl Pts',(-48.5725845633798,32.2456516907297,3.60701400320324));
#17608=CARTESIAN_POINT('Ctrl Pts',(-48.3407853679392,32.1124685639422,3.60701400320324));
#17609=CARTESIAN_POINT('Ctrl Pts',(-48.1089821836664,31.9792923792741,3.60701400320324));
#17610=CARTESIAN_POINT('Ctrl Pts',(-47.6453674864979,31.7129545080418,3.60701400320324));
#17611=CARTESIAN_POINT('Ctrl Pts',(-47.4135559734253,31.5797928212585,3.60701400320323));
#17612=CARTESIAN_POINT('Ctrl Pts',(-47.1817401099609,31.4466387085919,3.60701400320323));
#17613=CARTESIAN_POINT('Ctrl Pts',(-46.7406305897488,31.1932671494809,3.60701400320323));
#17614=CARTESIAN_POINT('Ctrl Pts',(-46.2995053259033,30.9399229970588,3.60701400320325));
#17615=CARTESIAN_POINT('Ctrl Pts',(-45.858362923034,30.686608693912,3.60701400320327));
#17616=CARTESIAN_POINT('Ctrl Pts',(45.858362923034,33.0633913333999,3.60701400320327));
#17617=CARTESIAN_POINT('Ctrl Pts',(46.0899257719339,33.1969849680263,3.60701400320326));
#17618=CARTESIAN_POINT('Ctrl Pts',(46.5530501979845,33.4641744416604,3.60701400320347));
#17619=CARTESIAN_POINT('Ctrl Pts',(47.0161721905706,33.7313681332063,3.60701400320335));
#17620=CARTESIAN_POINT('Ctrl Pts',(47.6893519862319,34.1197565257476,3.60701400320335));
#17621=CARTESIAN_POINT('Ctrl Pts',(48.1309692507095,34.3745507329179,3.60701400320329));
#17622=CARTESIAN_POINT('Ctrl Pts',(48.5725845633798,34.6293483229262,3.60701400320329));
#17623=CARTESIAN_POINT('Ctrl Pts',(1.54954344745633,33.4623411901214,48.6816745427932));
#17624=CARTESIAN_POINT('Ctrl Pts',(1.37917007070576,33.3690980212298,48.5301278551423));
#17625=CARTESIAN_POINT('Ctrl Pts',(1.19203308366643,33.282927635968,48.3910568573769));
#17626=CARTESIAN_POINT('Ctrl Pts',(0.805625630179277,33.1438388130886,48.1687150028693));
#17627=CARTESIAN_POINT('Ctrl Pts',(0.609847947224847,33.0885120549907,48.08133053428));
#17628=CARTESIAN_POINT('Ctrl Pts',(0.260777891394813,33.0206023207758,47.9764123934958));
#17629=CARTESIAN_POINT('Ctrl Pts',(0.115525945788527,33.0003237004996,47.9459618456904));
#17630=CARTESIAN_POINT('Ctrl Pts',(-0.115776397631957,32.9814498550727,
47.9196126328073));
#17631=CARTESIAN_POINT('Ctrl Pts',(-0.198964591777061,32.9772746441304,
47.9144499859977));
#17632=CARTESIAN_POINT('Ctrl Pts',(-0.284246351598831,32.9756985844503,
47.9136181470705));
#17633=CARTESIAN_POINT('Ctrl Pts',(-0.28600879736358,32.9756671879154,47.9136028937503));
#17634=CARTESIAN_POINT('Ctrl Pts',(-0.288399652950703,32.9756261901408,
47.9135848302284));
#17635=CARTESIAN_POINT('Ctrl Pts',(-0.289028030011347,32.9756155641944,
47.9135803289705));
#17636=CARTESIAN_POINT('Ctrl Pts',(-0.290151105636925,32.9755968396661,
47.9135727242207));
#17637=CARTESIAN_POINT('Ctrl Pts',(-0.290645802456765,32.9755886843435,
47.9135695270925));
#17638=CARTESIAN_POINT('Ctrl Pts',(-0.291615609203089,32.9755728779986,
47.9135635586627));
#17639=CARTESIAN_POINT('Ctrl Pts',(-0.292090718753741,32.9755652197985,
47.9135607755125));
#17640=CARTESIAN_POINT('Ctrl Pts',(-0.29321670374883,32.9755472725322,47.9135545132575));
#17641=CARTESIAN_POINT('Ctrl Pts',(-0.293867580950652,32.9755370582652,
47.9135511575783));
#17642=CARTESIAN_POINT('Ctrl Pts',(-0.296001919607553,32.9755040891644,
47.9135410201668));
#17643=CARTESIAN_POINT('Ctrl Pts',(-0.297485395190452,32.975482005975,47.9135353466702));
#17644=CARTESIAN_POINT('Ctrl Pts',(-0.341549846483652,32.9748507718471,
47.9134075922713));
#17645=CARTESIAN_POINT('Ctrl Pts',(-0.384111613704642,32.974926563486,47.9144149636289));
#17646=CARTESIAN_POINT('Ctrl Pts',(-0.544428271512558,32.9777877959916,
47.9224575922029));
#17647=CARTESIAN_POINT('Ctrl Pts',(-0.66105958463499,32.9851160668402,47.9369611544333));
#17648=CARTESIAN_POINT('Ctrl Pts',(-0.959813185315758,33.0169388209901,
47.9956482259754));
#17649=CARTESIAN_POINT('Ctrl Pts',(-1.13654290761119,33.0487223152527,48.0517468025327));
#17650=CARTESIAN_POINT('Ctrl Pts',(-1.61889911237043,33.1675753501152,48.2580271501411));
#17651=CARTESIAN_POINT('Ctrl Pts',(-1.90056409522944,33.2774762837005,48.4455751910135));
#17652=CARTESIAN_POINT('Ctrl Pts',(-2.14849279754675,33.4030003256338,48.658920044375));
#17653=CARTESIAN_POINT('Ctrl Pts',(-46.,55.6250000136559,0.));
#17654=CARTESIAN_POINT('Ctrl Pts',(-46.,55.4166666803226,-12.3256628518316));
#17655=CARTESIAN_POINT('Ctrl Pts',(-39.8371685740842,55.2083333469893,-23.));
#17656=CARTESIAN_POINT('Ctrl Pts',(-33.6743371481684,55.0000000136559,-33.6743371481684));
#17657=CARTESIAN_POINT('Ctrl Pts',(-23.,54.7916666803226,-39.8371685740842));
#17658=CARTESIAN_POINT('Ctrl Pts',(-12.3256628518317,54.5833333469893,-46.));
#17659=CARTESIAN_POINT('Ctrl Pts',(-2.81668763803891E-15,54.3750000136559,
-46.));
#17660=CARTESIAN_POINT('Ctrl Pts',(12.3256628518316,54.1666666803226,-46.));
#17661=CARTESIAN_POINT('Ctrl Pts',(23.,53.9583333469893,-39.8371685740842));
#17662=CARTESIAN_POINT('Ctrl Pts',(33.6743371481683,53.7500000136559,-33.6743371481684));
#17663=CARTESIAN_POINT('Ctrl Pts',(39.8371685740842,53.5416666803226,-23.));
#17664=CARTESIAN_POINT('Ctrl Pts',(46.,53.3333333469893,-12.3256628518317));
#17665=CARTESIAN_POINT('Ctrl Pts',(46.,53.1250000136559,-5.63337527607782E-15));
#17666=CARTESIAN_POINT('Ctrl Pts',(46.,52.9166666803226,12.3256628518316));
#17667=CARTESIAN_POINT('Ctrl Pts',(39.8371685740842,52.7083333469893,23.));
#17668=CARTESIAN_POINT('Ctrl Pts',(33.6743371481684,52.5000000136559,33.6743371481683));
#17669=CARTESIAN_POINT('Ctrl Pts',(23.,52.2916666803226,39.8371685740842));
#17670=CARTESIAN_POINT('Ctrl Pts',(12.3256628518317,52.0833333469893,46.));
#17671=CARTESIAN_POINT('Ctrl Pts',(8.45006291411674E-15,51.8750000136559,
46.));
#17672=CARTESIAN_POINT('Ctrl Pts',(-12.3256628518316,51.6666666803226,46.));
#17673=CARTESIAN_POINT('Ctrl Pts',(-23.,51.4583333469893,39.8371685740842));
#17674=CARTESIAN_POINT('Ctrl Pts',(-33.6743371481683,51.2500000136559,33.6743371481684));
#17675=CARTESIAN_POINT('Ctrl Pts',(-39.8371685740842,51.0416666803226,23.));
#17676=CARTESIAN_POINT('Ctrl Pts',(-46.,50.8333333469893,12.3256628518317));
#17677=CARTESIAN_POINT('Ctrl Pts',(-46.,50.6250000136559,0.));
#17678=CARTESIAN_POINT('Ctrl Pts',(-46.,50.4166666803226,-12.3256628518316));
#17679=CARTESIAN_POINT('Ctrl Pts',(-39.8371685740842,50.2083333469893,-23.));
#17680=CARTESIAN_POINT('Ctrl Pts',(-33.6743371481684,50.0000000136559,-33.6743371481684));
#17681=CARTESIAN_POINT('Ctrl Pts',(-23.,49.7916666803226,-39.8371685740842));
#17682=CARTESIAN_POINT('Ctrl Pts',(-12.3256628518317,49.5833333469893,-46.));
#17683=CARTESIAN_POINT('Ctrl Pts',(-2.81668763803891E-15,49.3750000136559,
-46.));
#17684=CARTESIAN_POINT('Ctrl Pts',(12.3256628518316,49.1666666803226,-46.));
#17685=CARTESIAN_POINT('Ctrl Pts',(23.,48.9583333469893,-39.8371685740842));
#17686=CARTESIAN_POINT('Ctrl Pts',(33.6743371481683,48.7500000136559,-33.6743371481684));
#17687=CARTESIAN_POINT('Ctrl Pts',(39.8371685740842,48.5416666803226,-23.));
#17688=CARTESIAN_POINT('Ctrl Pts',(46.,48.3333333469893,-12.3256628518317));
#17689=CARTESIAN_POINT('Ctrl Pts',(46.,48.1250000136559,-5.63337527607782E-15));
#17690=CARTESIAN_POINT('Ctrl Pts',(46.,47.9166666803226,12.3256628518316));
#17691=CARTESIAN_POINT('Ctrl Pts',(39.8371685740842,47.7083333469893,23.));
#17692=CARTESIAN_POINT('Ctrl Pts',(33.6743371481684,47.5000000136559,33.6743371481683));
#17693=CARTESIAN_POINT('Ctrl Pts',(23.,47.2916666803226,39.8371685740842));
#17694=CARTESIAN_POINT('Ctrl Pts',(12.3256628518317,47.0833333469893,46.));
#17695=CARTESIAN_POINT('Ctrl Pts',(8.45006291411674E-15,46.8750000136559,
46.));
#17696=CARTESIAN_POINT('Ctrl Pts',(-12.3256628518316,46.6666666803226,46.));
#17697=CARTESIAN_POINT('Ctrl Pts',(-23.,46.4583333469893,39.8371685740842));
#17698=CARTESIAN_POINT('Ctrl Pts',(-33.6743371481683,46.2500000136559,33.6743371481684));
#17699=CARTESIAN_POINT('Ctrl Pts',(-39.8371685740842,46.0416666803226,23.));
#17700=CARTESIAN_POINT('Ctrl Pts',(-46.,45.8333333469892,12.3256628518317));
#17701=CARTESIAN_POINT('Ctrl Pts',(-46.,45.6250000136559,0.));
#17702=CARTESIAN_POINT('Ctrl Pts',(-46.,45.4166666803226,-12.3256628518316));
#17703=CARTESIAN_POINT('Ctrl Pts',(-39.8371685740842,45.2083333469893,-23.));
#17704=CARTESIAN_POINT('Ctrl Pts',(-33.6743371481684,45.0000000136559,-33.6743371481684));
#17705=CARTESIAN_POINT('Ctrl Pts',(-23.,44.7916666803226,-39.8371685740842));
#17706=CARTESIAN_POINT('Ctrl Pts',(-12.3256628518317,44.5833333469893,-46.));
#17707=CARTESIAN_POINT('Ctrl Pts',(-2.81668763803891E-15,44.3750000136559,
-46.));
#17708=CARTESIAN_POINT('Ctrl Pts',(12.3256628518316,44.1666666803226,-46.));
#17709=CARTESIAN_POINT('Ctrl Pts',(23.,43.9583333469893,-39.8371685740842));
#17710=CARTESIAN_POINT('Ctrl Pts',(33.6743371481683,43.7500000136559,-33.6743371481684));
#17711=CARTESIAN_POINT('Ctrl Pts',(39.8371685740842,43.5416666803226,-23.));
#17712=CARTESIAN_POINT('Ctrl Pts',(46.,43.3333333469893,-12.3256628518317));
#17713=CARTESIAN_POINT('Ctrl Pts',(46.,43.1250000136559,-5.63337527607782E-15));
#17714=CARTESIAN_POINT('Ctrl Pts',(46.,42.9166666803226,12.3256628518316));
#17715=CARTESIAN_POINT('Ctrl Pts',(39.8371685740842,42.7083333469893,23.));
#17716=CARTESIAN_POINT('Ctrl Pts',(33.6743371481684,42.5000000136559,33.6743371481683));
#17717=CARTESIAN_POINT('Ctrl Pts',(23.,42.2916666803226,39.8371685740842));
#17718=CARTESIAN_POINT('Ctrl Pts',(12.3256628518317,42.0833333469893,46.));
#17719=CARTESIAN_POINT('Ctrl Pts',(8.45006291411674E-15,41.8750000136559,
46.));
#17720=CARTESIAN_POINT('Ctrl Pts',(-12.3256628518316,41.6666666803226,46.));
#17721=CARTESIAN_POINT('Ctrl Pts',(-23.,41.4583333469893,39.8371685740842));
#17722=CARTESIAN_POINT('Ctrl Pts',(-33.6743371481683,41.2500000136559,33.6743371481684));
#17723=CARTESIAN_POINT('Ctrl Pts',(-39.8371685740842,41.0416666803226,23.));
#17724=CARTESIAN_POINT('Ctrl Pts',(-46.,40.8333333469893,12.3256628518317));
#17725=CARTESIAN_POINT('Ctrl Pts',(-46.,40.6250000136559,0.));
#17726=CARTESIAN_POINT('Ctrl Pts',(-46.,40.4166666803226,-12.3256628518316));
#17727=CARTESIAN_POINT('Ctrl Pts',(-39.8371685740842,40.2083333469893,-23.));
#17728=CARTESIAN_POINT('Ctrl Pts',(-33.6743371481684,40.0000000136559,-33.6743371481684));
#17729=CARTESIAN_POINT('Ctrl Pts',(-23.,39.7916666803226,-39.8371685740842));
#17730=CARTESIAN_POINT('Ctrl Pts',(-12.3256628518317,39.5833333469893,-46.));
#17731=CARTESIAN_POINT('Ctrl Pts',(-2.81668763803891E-15,39.3750000136559,
-46.));
#17732=CARTESIAN_POINT('Ctrl Pts',(12.3256628518316,39.1666666803226,-46.));
#17733=CARTESIAN_POINT('Ctrl Pts',(23.,38.9583333469893,-39.8371685740842));
#17734=CARTESIAN_POINT('Ctrl Pts',(33.6743371481683,38.7500000136559,-33.6743371481684));
#17735=CARTESIAN_POINT('Ctrl Pts',(39.8371685740842,38.5416666803226,-23.));
#17736=CARTESIAN_POINT('Ctrl Pts',(46.,38.3333333469893,-12.3256628518317));
#17737=CARTESIAN_POINT('Ctrl Pts',(46.,38.1250000136559,-5.63337527607782E-15));
#17738=CARTESIAN_POINT('Ctrl Pts',(46.,37.9166666803226,12.3256628518316));
#17739=CARTESIAN_POINT('Ctrl Pts',(39.8371685740842,37.7083333469893,23.));
#17740=CARTESIAN_POINT('Ctrl Pts',(33.6743371481684,37.5000000136559,33.6743371481683));
#17741=CARTESIAN_POINT('Ctrl Pts',(23.,37.2916666803226,39.8371685740842));
#17742=CARTESIAN_POINT('Ctrl Pts',(12.3256628518317,37.0833333469893,46.));
#17743=CARTESIAN_POINT('Ctrl Pts',(8.45006291411674E-15,36.8750000136559,
46.));
#17744=CARTESIAN_POINT('Ctrl Pts',(-12.3256628518316,36.6666666803226,46.));
#17745=CARTESIAN_POINT('Ctrl Pts',(-23.,36.4583333469893,39.8371685740842));
#17746=CARTESIAN_POINT('Ctrl Pts',(-33.6743371481683,36.2500000136559,33.6743371481684));
#17747=CARTESIAN_POINT('Ctrl Pts',(-39.8371685740842,36.0416666803226,23.));
#17748=CARTESIAN_POINT('Ctrl Pts',(-46.,35.8333333469893,12.3256628518317));
#17749=CARTESIAN_POINT('Ctrl Pts',(-46.,35.6250000136559,0.));
#17750=CARTESIAN_POINT('Ctrl Pts',(-46.,35.4166666803226,-12.3256628518316));
#17751=CARTESIAN_POINT('Ctrl Pts',(-39.8371685740842,35.2083333469893,-23.));
#17752=CARTESIAN_POINT('Ctrl Pts',(-33.6743371481684,35.0000000136559,-33.6743371481684));
#17753=CARTESIAN_POINT('Ctrl Pts',(-23.,34.7916666803226,-39.8371685740842));
#17754=CARTESIAN_POINT('Ctrl Pts',(-12.3256628518317,34.5833333469893,-46.));
#17755=CARTESIAN_POINT('Ctrl Pts',(-2.81668763803891E-15,34.3750000136559,
-46.));
#17756=CARTESIAN_POINT('Ctrl Pts',(12.3256628518316,34.1666666803226,-46.));
#17757=CARTESIAN_POINT('Ctrl Pts',(23.,33.9583333469893,-39.8371685740842));
#17758=CARTESIAN_POINT('Ctrl Pts',(33.6743371481683,33.7500000136559,-33.6743371481684));
#17759=CARTESIAN_POINT('Ctrl Pts',(39.8371685740842,33.5416666803226,-23.));
#17760=CARTESIAN_POINT('Ctrl Pts',(46.,33.3333333469893,-12.3256628518317));
#17761=CARTESIAN_POINT('Ctrl Pts',(46.,33.1250000136559,-5.63337527607782E-15));
#17762=CARTESIAN_POINT('Ctrl Pts',(46.,32.9166666803226,12.3256628518316));
#17763=CARTESIAN_POINT('Ctrl Pts',(39.8371685740842,32.7083333469893,23.));
#17764=CARTESIAN_POINT('Ctrl Pts',(33.6743371481684,32.5000000136559,33.6743371481683));
#17765=CARTESIAN_POINT('Ctrl Pts',(23.,32.2916666803226,39.8371685740842));
#17766=CARTESIAN_POINT('Ctrl Pts',(12.3256628518317,32.0833333469893,46.));
#17767=CARTESIAN_POINT('Ctrl Pts',(8.45006291411674E-15,31.8750000136559,
46.));
#17768=CARTESIAN_POINT('Ctrl Pts',(-12.3256628518316,31.6666666803226,46.));
#17769=CARTESIAN_POINT('Ctrl Pts',(-23.,31.4583333469893,39.8371685740842));
#17770=CARTESIAN_POINT('Ctrl Pts',(-33.6743371481683,31.2500000136559,33.6743371481684));
#17771=CARTESIAN_POINT('Ctrl Pts',(-39.8371685740842,31.0416666803226,23.));
#17772=CARTESIAN_POINT('Ctrl Pts',(-46.,30.8333333469893,12.3256628518317));
#17773=CARTESIAN_POINT('Ctrl Pts',(-46.,30.6250000136559,0.));
#17774=CARTESIAN_POINT('Ctrl Pts',(-46.,30.4166666803226,-12.3256628518316));
#17775=CARTESIAN_POINT('Ctrl Pts',(-39.8371685740842,30.2083333469893,-23.));
#17776=CARTESIAN_POINT('Ctrl Pts',(-33.6743371481684,30.0000000136559,-33.6743371481684));
#17777=CARTESIAN_POINT('Ctrl Pts',(-23.,29.7916666803226,-39.8371685740842));
#17778=CARTESIAN_POINT('Ctrl Pts',(-12.3256628518317,29.5833333469893,-46.));
#17779=CARTESIAN_POINT('Ctrl Pts',(-2.81668763803891E-15,29.3750000136559,
-46.));
#17780=CARTESIAN_POINT('Ctrl Pts',(12.3256628518316,29.1666666803226,-46.));
#17781=CARTESIAN_POINT('Ctrl Pts',(23.,28.9583333469893,-39.8371685740842));
#17782=CARTESIAN_POINT('Ctrl Pts',(33.6743371481683,28.7500000136559,-33.6743371481684));
#17783=CARTESIAN_POINT('Ctrl Pts',(39.8371685740842,28.5416666803226,-23.));
#17784=CARTESIAN_POINT('Ctrl Pts',(46.,28.3333333469893,-12.3256628518317));
#17785=CARTESIAN_POINT('Ctrl Pts',(46.,28.1250000136559,-5.63337527607782E-15));
#17786=CARTESIAN_POINT('Ctrl Pts',(46.,27.9166666803226,12.3256628518316));
#17787=CARTESIAN_POINT('Ctrl Pts',(39.8371685740842,27.7083333469893,23.));
#17788=CARTESIAN_POINT('Ctrl Pts',(33.6743371481684,27.5000000136559,33.6743371481683));
#17789=CARTESIAN_POINT('Ctrl Pts',(23.,27.2916666803226,39.8371685740842));
#17790=CARTESIAN_POINT('Ctrl Pts',(12.3256628518317,27.0833333469893,46.));
#17791=CARTESIAN_POINT('Ctrl Pts',(8.45006291411674E-15,26.8750000136559,
46.));
#17792=CARTESIAN_POINT('Ctrl Pts',(-12.3256628518316,26.6666666803226,46.));
#17793=CARTESIAN_POINT('Ctrl Pts',(-23.,26.4583333469893,39.8371685740842));
#17794=CARTESIAN_POINT('Ctrl Pts',(-33.6743371481683,26.2500000136559,33.6743371481684));
#17795=CARTESIAN_POINT('Ctrl Pts',(-39.8371685740842,26.0416666803226,23.));
#17796=CARTESIAN_POINT('Ctrl Pts',(-46.,25.8333333469893,12.3256628518317));
#17797=CARTESIAN_POINT('Ctrl Pts',(-46.,25.6250000136559,0.));
#17798=CARTESIAN_POINT('Ctrl Pts',(-48.706329375,57.187500006828,-1.8898197019151E-14));
#17799=CARTESIAN_POINT('Ctrl Pts',(-48.706329375,56.9791666734946,-13.0508216223155));
#17800=CARTESIAN_POINT('Ctrl Pts',(-42.1809185638422,56.7708333401613,-24.3531646875));
#17801=CARTESIAN_POINT('Ctrl Pts',(-35.6555077526845,56.562500006828,-35.6555077526845));
#17802=CARTESIAN_POINT('Ctrl Pts',(-24.3531646875,56.3541666734946,-42.1809185638423));
#17803=CARTESIAN_POINT('Ctrl Pts',(-13.0508216223155,56.1458333401613,-48.706329375));
#17804=CARTESIAN_POINT('Ctrl Pts',(1.59157945007855E-14,55.937500006828,
-48.706329375));
#17805=CARTESIAN_POINT('Ctrl Pts',(13.0508216223155,55.7291666734946,-48.706329375));
#17806=CARTESIAN_POINT('Ctrl Pts',(24.3531646875,55.5208333401613,-42.1809185638422));
#17807=CARTESIAN_POINT('Ctrl Pts',(35.6555077526845,55.312500006828,-35.6555077526845));
#17808=CARTESIAN_POINT('Ctrl Pts',(42.1809185638422,55.1041666734946,-24.3531646875));
#17809=CARTESIAN_POINT('Ctrl Pts',(48.706329375,54.8958333401613,-13.0508216223155));
#17810=CARTESIAN_POINT('Ctrl Pts',(48.706329375,54.687500006828,1.293339198242E-14));
#17811=CARTESIAN_POINT('Ctrl Pts',(48.706329375,54.4791666734946,13.0508216223155));
#17812=CARTESIAN_POINT('Ctrl Pts',(42.1809185638422,54.2708333401613,24.3531646875));
#17813=CARTESIAN_POINT('Ctrl Pts',(35.6555077526845,54.062500006828,35.6555077526845));
#17814=CARTESIAN_POINT('Ctrl Pts',(24.3531646875,53.8541666734946,42.1809185638422));
#17815=CARTESIAN_POINT('Ctrl Pts',(13.0508216223155,53.6458333401613,48.706329375));
#17816=CARTESIAN_POINT('Ctrl Pts',(-9.95098946405443E-15,53.437500006828,
48.706329375));
#17817=CARTESIAN_POINT('Ctrl Pts',(-13.0508216223155,53.2291666734946,48.706329375));
#17818=CARTESIAN_POINT('Ctrl Pts',(-24.3531646875,53.0208333401613,42.1809185638423));
#17819=CARTESIAN_POINT('Ctrl Pts',(-35.6555077526845,52.812500006828,35.6555077526845));
#17820=CARTESIAN_POINT('Ctrl Pts',(-42.1809185638422,52.6041666734946,24.3531646875));
#17821=CARTESIAN_POINT('Ctrl Pts',(-48.706329375,52.3958333401613,13.0508216223155));
#17822=CARTESIAN_POINT('Ctrl Pts',(-48.706329375,52.187500006828,-1.8898197019151E-14));
#17823=CARTESIAN_POINT('Ctrl Pts',(-48.706329375,51.9791666734946,-13.0508216223155));
#17824=CARTESIAN_POINT('Ctrl Pts',(-42.1809185638422,51.7708333401613,-24.3531646875));
#17825=CARTESIAN_POINT('Ctrl Pts',(-35.6555077526845,51.562500006828,-35.6555077526845));
#17826=CARTESIAN_POINT('Ctrl Pts',(-24.3531646875,51.3541666734946,-42.1809185638423));
#17827=CARTESIAN_POINT('Ctrl Pts',(-13.0508216223155,51.1458333401613,-48.706329375));
#17828=CARTESIAN_POINT('Ctrl Pts',(1.59157945007855E-14,50.937500006828,
-48.706329375));
#17829=CARTESIAN_POINT('Ctrl Pts',(13.0508216223155,50.7291666734946,-48.706329375));
#17830=CARTESIAN_POINT('Ctrl Pts',(24.3531646875,50.5208333401613,-42.1809185638422));
#17831=CARTESIAN_POINT('Ctrl Pts',(35.6555077526845,50.312500006828,-35.6555077526845));
#17832=CARTESIAN_POINT('Ctrl Pts',(42.1809185638422,50.1041666734946,-24.3531646875));
#17833=CARTESIAN_POINT('Ctrl Pts',(48.706329375,49.8958333401613,-13.0508216223155));
#17834=CARTESIAN_POINT('Ctrl Pts',(48.706329375,49.687500006828,1.293339198242E-14));
#17835=CARTESIAN_POINT('Ctrl Pts',(48.706329375,49.4791666734946,13.0508216223155));
#17836=CARTESIAN_POINT('Ctrl Pts',(42.1809185638422,49.2708333401613,24.3531646875));
#17837=CARTESIAN_POINT('Ctrl Pts',(35.6555077526845,49.062500006828,35.6555077526845));
#17838=CARTESIAN_POINT('Ctrl Pts',(24.3531646875,48.8541666734946,42.1809185638422));
#17839=CARTESIAN_POINT('Ctrl Pts',(13.0508216223155,48.6458333401613,48.706329375));
#17840=CARTESIAN_POINT('Ctrl Pts',(-9.95098946405443E-15,48.437500006828,
48.706329375));
#17841=CARTESIAN_POINT('Ctrl Pts',(-13.0508216223155,48.2291666734946,48.706329375));
#17842=CARTESIAN_POINT('Ctrl Pts',(-24.3531646875,48.0208333401613,42.1809185638423));
#17843=CARTESIAN_POINT('Ctrl Pts',(-35.6555077526845,47.812500006828,35.6555077526845));
#17844=CARTESIAN_POINT('Ctrl Pts',(-42.1809185638422,47.6041666734946,24.3531646875));
#17845=CARTESIAN_POINT('Ctrl Pts',(-48.706329375,47.3958333401613,13.0508216223155));
#17846=CARTESIAN_POINT('Ctrl Pts',(-48.706329375,47.187500006828,-1.8898197019151E-14));
#17847=CARTESIAN_POINT('Ctrl Pts',(-48.706329375,46.9791666734946,-13.0508216223155));
#17848=CARTESIAN_POINT('Ctrl Pts',(-42.1809185638422,46.7708333401613,-24.3531646875));
#17849=CARTESIAN_POINT('Ctrl Pts',(-35.6555077526845,46.562500006828,-35.6555077526845));
#17850=CARTESIAN_POINT('Ctrl Pts',(-24.3531646875,46.3541666734946,-42.1809185638423));
#17851=CARTESIAN_POINT('Ctrl Pts',(-13.0508216223155,46.1458333401613,-48.706329375));
#17852=CARTESIAN_POINT('Ctrl Pts',(1.59157945007855E-14,45.937500006828,
-48.706329375));
#17853=CARTESIAN_POINT('Ctrl Pts',(13.0508216223155,45.7291666734946,-48.706329375));
#17854=CARTESIAN_POINT('Ctrl Pts',(24.3531646875,45.5208333401613,-42.1809185638422));
#17855=CARTESIAN_POINT('Ctrl Pts',(35.6555077526845,45.312500006828,-35.6555077526845));
#17856=CARTESIAN_POINT('Ctrl Pts',(42.1809185638422,45.1041666734946,-24.3531646875));
#17857=CARTESIAN_POINT('Ctrl Pts',(48.706329375,44.8958333401613,-13.0508216223155));
#17858=CARTESIAN_POINT('Ctrl Pts',(48.706329375,44.687500006828,1.293339198242E-14));
#17859=CARTESIAN_POINT('Ctrl Pts',(48.706329375,44.4791666734946,13.0508216223155));
#17860=CARTESIAN_POINT('Ctrl Pts',(42.1809185638422,44.2708333401613,24.3531646875));
#17861=CARTESIAN_POINT('Ctrl Pts',(35.6555077526845,44.062500006828,35.6555077526845));
#17862=CARTESIAN_POINT('Ctrl Pts',(24.3531646875,43.8541666734946,42.1809185638422));
#17863=CARTESIAN_POINT('Ctrl Pts',(13.0508216223155,43.6458333401613,48.706329375));
#17864=CARTESIAN_POINT('Ctrl Pts',(-9.95098946405443E-15,43.437500006828,
48.706329375));
#17865=CARTESIAN_POINT('Ctrl Pts',(-13.0508216223155,43.2291666734946,48.706329375));
#17866=CARTESIAN_POINT('Ctrl Pts',(-24.3531646875,43.0208333401613,42.1809185638423));
#17867=CARTESIAN_POINT('Ctrl Pts',(-35.6555077526845,42.812500006828,35.6555077526845));
#17868=CARTESIAN_POINT('Ctrl Pts',(-42.1809185638422,42.6041666734946,24.3531646875));
#17869=CARTESIAN_POINT('Ctrl Pts',(-48.706329375,42.3958333401613,13.0508216223155));
#17870=CARTESIAN_POINT('Ctrl Pts',(-48.706329375,42.187500006828,-1.8898197019151E-14));
#17871=CARTESIAN_POINT('Ctrl Pts',(-48.706329375,41.9791666734946,-13.0508216223155));
#17872=CARTESIAN_POINT('Ctrl Pts',(-42.1809185638422,41.7708333401613,-24.3531646875));
#17873=CARTESIAN_POINT('Ctrl Pts',(-35.6555077526845,41.562500006828,-35.6555077526845));
#17874=CARTESIAN_POINT('Ctrl Pts',(-24.3531646875,41.3541666734946,-42.1809185638423));
#17875=CARTESIAN_POINT('Ctrl Pts',(-13.0508216223155,41.1458333401613,-48.706329375));
#17876=CARTESIAN_POINT('Ctrl Pts',(1.59157945007855E-14,40.937500006828,
-48.706329375));
#17877=CARTESIAN_POINT('Ctrl Pts',(13.0508216223155,40.7291666734946,-48.706329375));
#17878=CARTESIAN_POINT('Ctrl Pts',(24.3531646875,40.5208333401613,-42.1809185638422));
#17879=CARTESIAN_POINT('Ctrl Pts',(35.6555077526845,40.312500006828,-35.6555077526845));
#17880=CARTESIAN_POINT('Ctrl Pts',(42.1809185638422,40.1041666734946,-24.3531646875));
#17881=CARTESIAN_POINT('Ctrl Pts',(48.706329375,39.8958333401613,-13.0508216223155));
#17882=CARTESIAN_POINT('Ctrl Pts',(48.706329375,39.687500006828,1.293339198242E-14));
#17883=CARTESIAN_POINT('Ctrl Pts',(48.706329375,39.4791666734946,13.0508216223155));
#17884=CARTESIAN_POINT('Ctrl Pts',(42.1809185638422,39.2708333401613,24.3531646875));
#17885=CARTESIAN_POINT('Ctrl Pts',(35.6555077526845,39.062500006828,35.6555077526845));
#17886=CARTESIAN_POINT('Ctrl Pts',(24.3531646875,38.8541666734946,42.1809185638422));
#17887=CARTESIAN_POINT('Ctrl Pts',(13.0508216223155,38.6458333401613,48.706329375));
#17888=CARTESIAN_POINT('Ctrl Pts',(-9.95098946405443E-15,38.437500006828,
48.706329375));
#17889=CARTESIAN_POINT('Ctrl Pts',(-13.0508216223155,38.2291666734946,48.706329375));
#17890=CARTESIAN_POINT('Ctrl Pts',(-24.3531646875,38.0208333401613,42.1809185638423));
#17891=CARTESIAN_POINT('Ctrl Pts',(-35.6555077526845,37.812500006828,35.6555077526845));
#17892=CARTESIAN_POINT('Ctrl Pts',(-42.1809185638422,37.6041666734946,24.3531646875));
#17893=CARTESIAN_POINT('Ctrl Pts',(-48.706329375,37.3958333401613,13.0508216223155));
#17894=CARTESIAN_POINT('Ctrl Pts',(-48.706329375,37.187500006828,-1.8898197019151E-14));
#17895=CARTESIAN_POINT('Ctrl Pts',(-48.706329375,36.9791666734946,-13.0508216223155));
#17896=CARTESIAN_POINT('Ctrl Pts',(-42.1809185638422,36.7708333401613,-24.3531646875));
#17897=CARTESIAN_POINT('Ctrl Pts',(-35.6555077526845,36.562500006828,-35.6555077526845));
#17898=CARTESIAN_POINT('Ctrl Pts',(-24.3531646875,36.3541666734946,-42.1809185638423));
#17899=CARTESIAN_POINT('Ctrl Pts',(-13.0508216223155,36.1458333401613,-48.706329375));
#17900=CARTESIAN_POINT('Ctrl Pts',(1.59157945007855E-14,35.937500006828,
-48.706329375));
#17901=CARTESIAN_POINT('Ctrl Pts',(13.0508216223155,35.7291666734946,-48.706329375));
#17902=CARTESIAN_POINT('Ctrl Pts',(24.3531646875,35.5208333401613,-42.1809185638422));
#17903=CARTESIAN_POINT('Ctrl Pts',(35.6555077526845,35.312500006828,-35.6555077526845));
#17904=CARTESIAN_POINT('Ctrl Pts',(42.1809185638422,35.1041666734946,-24.3531646875));
#17905=CARTESIAN_POINT('Ctrl Pts',(48.706329375,34.8958333401613,-13.0508216223155));
#17906=CARTESIAN_POINT('Ctrl Pts',(48.706329375,34.687500006828,1.293339198242E-14));
#17907=CARTESIAN_POINT('Ctrl Pts',(48.706329375,34.4791666734946,13.0508216223155));
#17908=CARTESIAN_POINT('Ctrl Pts',(42.1809185638422,34.2708333401613,24.3531646875));
#17909=CARTESIAN_POINT('Ctrl Pts',(35.6555077526845,34.062500006828,35.6555077526845));
#17910=CARTESIAN_POINT('Ctrl Pts',(24.3531646875,33.8541666734946,42.1809185638422));
#17911=CARTESIAN_POINT('Ctrl Pts',(13.0508216223155,33.6458333401613,48.706329375));
#17912=CARTESIAN_POINT('Ctrl Pts',(-9.95098946405443E-15,33.437500006828,
48.706329375));
#17913=CARTESIAN_POINT('Ctrl Pts',(-13.0508216223155,33.2291666734946,48.706329375));
#17914=CARTESIAN_POINT('Ctrl Pts',(-24.3531646875,33.0208333401613,42.1809185638423));
#17915=CARTESIAN_POINT('Ctrl Pts',(-35.6555077526845,32.812500006828,35.6555077526845));
#17916=CARTESIAN_POINT('Ctrl Pts',(-42.1809185638422,32.6041666734946,24.3531646875));
#17917=CARTESIAN_POINT('Ctrl Pts',(-48.706329375,32.3958333401613,13.0508216223155));
#17918=CARTESIAN_POINT('Ctrl Pts',(-48.706329375,32.187500006828,-1.8898197019151E-14));
#17919=CARTESIAN_POINT('Ctrl Pts',(-48.706329375,31.9791666734946,-13.0508216223155));
#17920=CARTESIAN_POINT('Ctrl Pts',(-42.1809185638422,31.7708333401613,-24.3531646875));
#17921=CARTESIAN_POINT('Ctrl Pts',(-35.6555077526845,31.562500006828,-35.6555077526845));
#17922=CARTESIAN_POINT('Ctrl Pts',(-24.3531646875,31.3541666734946,-42.1809185638423));
#17923=CARTESIAN_POINT('Ctrl Pts',(-13.0508216223155,31.1458333401613,-48.706329375));
#17924=CARTESIAN_POINT('Ctrl Pts',(1.59157945007855E-14,30.937500006828,
-48.706329375));
#17925=CARTESIAN_POINT('Ctrl Pts',(13.0508216223155,30.7291666734946,-48.706329375));
#17926=CARTESIAN_POINT('Ctrl Pts',(24.3531646875,30.5208333401613,-42.1809185638422));
#17927=CARTESIAN_POINT('Ctrl Pts',(35.6555077526845,30.312500006828,-35.6555077526845));
#17928=CARTESIAN_POINT('Ctrl Pts',(42.1809185638422,30.1041666734946,-24.3531646875));
#17929=CARTESIAN_POINT('Ctrl Pts',(48.706329375,29.8958333401613,-13.0508216223155));
#17930=CARTESIAN_POINT('Ctrl Pts',(48.706329375,29.687500006828,1.293339198242E-14));
#17931=CARTESIAN_POINT('Ctrl Pts',(48.706329375,29.4791666734946,13.0508216223155));
#17932=CARTESIAN_POINT('Ctrl Pts',(42.1809185638422,29.2708333401613,24.3531646875));
#17933=CARTESIAN_POINT('Ctrl Pts',(35.6555077526845,29.062500006828,35.6555077526845));
#17934=CARTESIAN_POINT('Ctrl Pts',(24.3531646875,28.8541666734946,42.1809185638422));
#17935=CARTESIAN_POINT('Ctrl Pts',(13.0508216223155,28.6458333401613,48.706329375));
#17936=CARTESIAN_POINT('Ctrl Pts',(-9.95098946405443E-15,28.437500006828,
48.706329375));
#17937=CARTESIAN_POINT('Ctrl Pts',(-13.0508216223155,28.2291666734946,48.706329375));
#17938=CARTESIAN_POINT('Ctrl Pts',(-24.3531646875,28.0208333401613,42.1809185638423));
#17939=CARTESIAN_POINT('Ctrl Pts',(-35.6555077526845,27.812500006828,35.6555077526845));
#17940=CARTESIAN_POINT('Ctrl Pts',(-42.1809185638422,27.6041666734946,24.3531646875));
#17941=CARTESIAN_POINT('Ctrl Pts',(-48.706329375,27.3958333401613,13.0508216223155));
#17942=CARTESIAN_POINT('Ctrl Pts',(-48.706329375,27.187500006828,-1.8898197019151E-14));
#17943=CARTESIAN_POINT('',(-48.5134353784345,32.1175463684955,-4.33048599679665));
#17944=CARTESIAN_POINT('',(48.5134353784344,29.7574536451604,-4.33048599679682));
#17945=CARTESIAN_POINT('Ctrl Pts',(-48.5134353784345,32.1175463684955,-4.33048599679665));
#17946=CARTESIAN_POINT('Ctrl Pts',(-47.5573898704235,31.9424850907232,-15.040843219065));
#17947=CARTESIAN_POINT('Ctrl Pts',(-42.1809185638422,31.7708333401613,-24.3531646875));
#17948=CARTESIAN_POINT('Ctrl Pts',(-35.6555077526845,31.562500006828,-35.6555077526845));
#17949=CARTESIAN_POINT('Ctrl Pts',(-24.3531646875,31.3541666734946,-42.1809185638423));
#17950=CARTESIAN_POINT('Ctrl Pts',(-13.0508216223155,31.1458333401613,-48.706329375));
#17951=CARTESIAN_POINT('Ctrl Pts',(1.59157945007855E-14,30.937500006828,
-48.706329375));
#17952=CARTESIAN_POINT('Ctrl Pts',(13.0508216223155,30.7291666734946,-48.706329375));
#17953=CARTESIAN_POINT('Ctrl Pts',(24.3531646875,30.5208333401613,-42.1809185638422));
#17954=CARTESIAN_POINT('Ctrl Pts',(35.6555077526845,30.312500006828,-35.6555077526845));
#17955=CARTESIAN_POINT('Ctrl Pts',(42.1809185638422,30.1041666734946,-24.3531646875));
#17956=CARTESIAN_POINT('Ctrl Pts',(47.5573898704235,29.9325149229327,-15.0408432190651));
#17957=CARTESIAN_POINT('Ctrl Pts',(48.5134353784344,29.7574536451604,-4.33048599679682));
#17958=CARTESIAN_POINT('',(48.235295107789,29.597913825102,-4.33048599679673));
#17959=CARTESIAN_POINT('',(48.5134353784344,29.7574536451604,-4.33048599679682));
#17960=CARTESIAN_POINT('Ctrl Pts',(48.2352951077952,29.5979138250913,-4.33048599679673));
#17961=CARTESIAN_POINT('Ctrl Pts',(47.829636183139,29.3652387164921,-4.33048599679611));
#17962=CARTESIAN_POINT('Ctrl Pts',(47.4228292493871,29.1305469649764,-4.3100254215245));
#17963=CARTESIAN_POINT('Ctrl Pts',(46.6173892826498,28.6628669666112,-4.22607365724017));
#17964=CARTESIAN_POINT('Ctrl Pts',(46.214789133894,28.4275716411426,-4.16216527479196));
#17965=CARTESIAN_POINT('Ctrl Pts',(45.8192253759654,28.1946814357457,-4.07413622090531));
#17966=CARTESIAN_POINT('Ctrl Pts',(-45.7957082162897,30.5508791552084,-4.33048599679682));
#17967=CARTESIAN_POINT('Ctrl Pts',(-46.027322302781,30.6843839384496,-4.33048599679682));
#17968=CARTESIAN_POINT('Ctrl Pts',(-46.4905476657728,30.9513983799647,-4.33048599679661));
#17969=CARTESIAN_POINT('Ctrl Pts',(-46.9537676533565,31.2184221466352,-4.33048599679666));
#17970=CARTESIAN_POINT('Ctrl Pts',(-47.6280672732222,31.6071316973962,-4.33048599679666));
#17971=CARTESIAN_POINT('Ctrl Pts',(-48.0707534890442,31.8623352807796,-4.33048599679665));
#17972=CARTESIAN_POINT('Ctrl Pts',(-48.5134353784345,32.1175463684955,-4.33048599679665));
#17973=CARTESIAN_POINT('Ctrl Pts',(-46.,55.6250000136559,0.));
#17974=CARTESIAN_POINT('Ctrl Pts',(-46.,55.4166666803226,-12.3256628518316));
#17975=CARTESIAN_POINT('Ctrl Pts',(-39.8371685740842,55.2083333469893,-23.));
#17976=CARTESIAN_POINT('Ctrl Pts',(-33.6743371481684,55.0000000136559,-33.6743371481684));
#17977=CARTESIAN_POINT('Ctrl Pts',(-23.,54.7916666803226,-39.8371685740842));
#17978=CARTESIAN_POINT('Ctrl Pts',(-12.3256628518317,54.5833333469893,-46.));
#17979=CARTESIAN_POINT('Ctrl Pts',(-2.81668763803891E-15,54.3750000136559,
-46.));
#17980=CARTESIAN_POINT('Ctrl Pts',(12.3256628518316,54.1666666803226,-46.));
#17981=CARTESIAN_POINT('Ctrl Pts',(23.,53.9583333469893,-39.8371685740842));
#17982=CARTESIAN_POINT('Ctrl Pts',(33.6743371481683,53.7500000136559,-33.6743371481684));
#17983=CARTESIAN_POINT('Ctrl Pts',(39.8371685740842,53.5416666803226,-23.));
#17984=CARTESIAN_POINT('Ctrl Pts',(46.,53.3333333469893,-12.3256628518317));
#17985=CARTESIAN_POINT('Ctrl Pts',(46.,53.1250000136559,-5.63337527607782E-15));
#17986=CARTESIAN_POINT('Ctrl Pts',(46.,52.9166666803226,12.3256628518316));
#17987=CARTESIAN_POINT('Ctrl Pts',(39.8371685740842,52.7083333469893,23.));
#17988=CARTESIAN_POINT('Ctrl Pts',(33.6743371481684,52.5000000136559,33.6743371481683));
#17989=CARTESIAN_POINT('Ctrl Pts',(23.,52.2916666803226,39.8371685740842));
#17990=CARTESIAN_POINT('Ctrl Pts',(12.3256628518317,52.0833333469893,46.));
#17991=CARTESIAN_POINT('Ctrl Pts',(8.45006291411674E-15,51.8750000136559,
46.));
#17992=CARTESIAN_POINT('Ctrl Pts',(-12.3256628518316,51.6666666803226,46.));
#17993=CARTESIAN_POINT('Ctrl Pts',(-23.,51.4583333469893,39.8371685740842));
#17994=CARTESIAN_POINT('Ctrl Pts',(-33.6743371481683,51.2500000136559,33.6743371481684));
#17995=CARTESIAN_POINT('Ctrl Pts',(-39.8371685740842,51.0416666803226,23.));
#17996=CARTESIAN_POINT('Ctrl Pts',(-46.,50.8333333469893,12.3256628518317));
#17997=CARTESIAN_POINT('Ctrl Pts',(-46.,50.6250000136559,0.));
#17998=CARTESIAN_POINT('Ctrl Pts',(-46.,50.4166666803226,-12.3256628518316));
#17999=CARTESIAN_POINT('Ctrl Pts',(-39.8371685740842,50.2083333469893,-23.));
#18000=CARTESIAN_POINT('Ctrl Pts',(-33.6743371481684,50.0000000136559,-33.6743371481684));
#18001=CARTESIAN_POINT('Ctrl Pts',(-23.,49.7916666803226,-39.8371685740842));
#18002=CARTESIAN_POINT('Ctrl Pts',(-12.3256628518317,49.5833333469893,-46.));
#18003=CARTESIAN_POINT('Ctrl Pts',(-2.81668763803891E-15,49.3750000136559,
-46.));
#18004=CARTESIAN_POINT('Ctrl Pts',(12.3256628518316,49.1666666803226,-46.));
#18005=CARTESIAN_POINT('Ctrl Pts',(23.,48.9583333469893,-39.8371685740842));
#18006=CARTESIAN_POINT('Ctrl Pts',(33.6743371481683,48.7500000136559,-33.6743371481684));
#18007=CARTESIAN_POINT('Ctrl Pts',(39.8371685740842,48.5416666803226,-23.));
#18008=CARTESIAN_POINT('Ctrl Pts',(46.,48.3333333469893,-12.3256628518317));
#18009=CARTESIAN_POINT('Ctrl Pts',(46.,48.1250000136559,-5.63337527607782E-15));
#18010=CARTESIAN_POINT('Ctrl Pts',(46.,47.9166666803226,12.3256628518316));
#18011=CARTESIAN_POINT('Ctrl Pts',(39.8371685740842,47.7083333469893,23.));
#18012=CARTESIAN_POINT('Ctrl Pts',(33.6743371481684,47.5000000136559,33.6743371481683));
#18013=CARTESIAN_POINT('Ctrl Pts',(23.,47.2916666803226,39.8371685740842));
#18014=CARTESIAN_POINT('Ctrl Pts',(12.3256628518317,47.0833333469893,46.));
#18015=CARTESIAN_POINT('Ctrl Pts',(8.45006291411674E-15,46.8750000136559,
46.));
#18016=CARTESIAN_POINT('Ctrl Pts',(-12.3256628518316,46.6666666803226,46.));
#18017=CARTESIAN_POINT('Ctrl Pts',(-23.,46.4583333469893,39.8371685740842));
#18018=CARTESIAN_POINT('Ctrl Pts',(-33.6743371481683,46.2500000136559,33.6743371481684));
#18019=CARTESIAN_POINT('Ctrl Pts',(-39.8371685740842,46.0416666803226,23.));
#18020=CARTESIAN_POINT('Ctrl Pts',(-46.,45.8333333469892,12.3256628518317));
#18021=CARTESIAN_POINT('Ctrl Pts',(-46.,45.6250000136559,0.));
#18022=CARTESIAN_POINT('Ctrl Pts',(-46.,45.4166666803226,-12.3256628518316));
#18023=CARTESIAN_POINT('Ctrl Pts',(-39.8371685740842,45.2083333469893,-23.));
#18024=CARTESIAN_POINT('Ctrl Pts',(-33.6743371481684,45.0000000136559,-33.6743371481684));
#18025=CARTESIAN_POINT('Ctrl Pts',(-23.,44.7916666803226,-39.8371685740842));
#18026=CARTESIAN_POINT('Ctrl Pts',(-12.3256628518317,44.5833333469893,-46.));
#18027=CARTESIAN_POINT('Ctrl Pts',(-2.81668763803891E-15,44.3750000136559,
-46.));
#18028=CARTESIAN_POINT('Ctrl Pts',(12.3256628518316,44.1666666803226,-46.));
#18029=CARTESIAN_POINT('Ctrl Pts',(23.,43.9583333469893,-39.8371685740842));
#18030=CARTESIAN_POINT('Ctrl Pts',(33.6743371481683,43.7500000136559,-33.6743371481684));
#18031=CARTESIAN_POINT('Ctrl Pts',(39.8371685740842,43.5416666803226,-23.));
#18032=CARTESIAN_POINT('Ctrl Pts',(46.,43.3333333469893,-12.3256628518317));
#18033=CARTESIAN_POINT('Ctrl Pts',(46.,43.1250000136559,-5.63337527607782E-15));
#18034=CARTESIAN_POINT('Ctrl Pts',(46.,42.9166666803226,12.3256628518316));
#18035=CARTESIAN_POINT('Ctrl Pts',(39.8371685740842,42.7083333469893,23.));
#18036=CARTESIAN_POINT('Ctrl Pts',(33.6743371481684,42.5000000136559,33.6743371481683));
#18037=CARTESIAN_POINT('Ctrl Pts',(23.,42.2916666803226,39.8371685740842));
#18038=CARTESIAN_POINT('Ctrl Pts',(12.3256628518317,42.0833333469893,46.));
#18039=CARTESIAN_POINT('Ctrl Pts',(8.45006291411674E-15,41.8750000136559,
46.));
#18040=CARTESIAN_POINT('Ctrl Pts',(-12.3256628518316,41.6666666803226,46.));
#18041=CARTESIAN_POINT('Ctrl Pts',(-23.,41.4583333469893,39.8371685740842));
#18042=CARTESIAN_POINT('Ctrl Pts',(-33.6743371481683,41.2500000136559,33.6743371481684));
#18043=CARTESIAN_POINT('Ctrl Pts',(-39.8371685740842,41.0416666803226,23.));
#18044=CARTESIAN_POINT('Ctrl Pts',(-46.,40.8333333469893,12.3256628518317));
#18045=CARTESIAN_POINT('Ctrl Pts',(-46.,40.6250000136559,0.));
#18046=CARTESIAN_POINT('Ctrl Pts',(-46.,40.4166666803226,-12.3256628518316));
#18047=CARTESIAN_POINT('Ctrl Pts',(-39.8371685740842,40.2083333469893,-23.));
#18048=CARTESIAN_POINT('Ctrl Pts',(-33.6743371481684,40.0000000136559,-33.6743371481684));
#18049=CARTESIAN_POINT('Ctrl Pts',(-23.,39.7916666803226,-39.8371685740842));
#18050=CARTESIAN_POINT('Ctrl Pts',(-12.3256628518317,39.5833333469893,-46.));
#18051=CARTESIAN_POINT('Ctrl Pts',(-2.81668763803891E-15,39.3750000136559,
-46.));
#18052=CARTESIAN_POINT('Ctrl Pts',(12.3256628518316,39.1666666803226,-46.));
#18053=CARTESIAN_POINT('Ctrl Pts',(23.,38.9583333469893,-39.8371685740842));
#18054=CARTESIAN_POINT('Ctrl Pts',(33.6743371481683,38.7500000136559,-33.6743371481684));
#18055=CARTESIAN_POINT('Ctrl Pts',(39.8371685740842,38.5416666803226,-23.));
#18056=CARTESIAN_POINT('Ctrl Pts',(46.,38.3333333469893,-12.3256628518317));
#18057=CARTESIAN_POINT('Ctrl Pts',(46.,38.1250000136559,-5.63337527607782E-15));
#18058=CARTESIAN_POINT('Ctrl Pts',(46.,37.9166666803226,12.3256628518316));
#18059=CARTESIAN_POINT('Ctrl Pts',(39.8371685740842,37.7083333469893,23.));
#18060=CARTESIAN_POINT('Ctrl Pts',(33.6743371481684,37.5000000136559,33.6743371481683));
#18061=CARTESIAN_POINT('Ctrl Pts',(23.,37.2916666803226,39.8371685740842));
#18062=CARTESIAN_POINT('Ctrl Pts',(12.3256628518317,37.0833333469893,46.));
#18063=CARTESIAN_POINT('Ctrl Pts',(8.45006291411674E-15,36.8750000136559,
46.));
#18064=CARTESIAN_POINT('Ctrl Pts',(-12.3256628518316,36.6666666803226,46.));
#18065=CARTESIAN_POINT('Ctrl Pts',(-23.,36.4583333469893,39.8371685740842));
#18066=CARTESIAN_POINT('Ctrl Pts',(-33.6743371481683,36.2500000136559,33.6743371481684));
#18067=CARTESIAN_POINT('Ctrl Pts',(-39.8371685740842,36.0416666803226,23.));
#18068=CARTESIAN_POINT('Ctrl Pts',(-46.,35.8333333469893,12.3256628518317));
#18069=CARTESIAN_POINT('Ctrl Pts',(-46.,35.6250000136559,0.));
#18070=CARTESIAN_POINT('Ctrl Pts',(-46.,35.4166666803226,-12.3256628518316));
#18071=CARTESIAN_POINT('Ctrl Pts',(-39.8371685740842,35.2083333469893,-23.));
#18072=CARTESIAN_POINT('Ctrl Pts',(-33.6743371481684,35.0000000136559,-33.6743371481684));
#18073=CARTESIAN_POINT('Ctrl Pts',(-23.,34.7916666803226,-39.8371685740842));
#18074=CARTESIAN_POINT('Ctrl Pts',(-12.3256628518317,34.5833333469893,-46.));
#18075=CARTESIAN_POINT('Ctrl Pts',(-2.81668763803891E-15,34.3750000136559,
-46.));
#18076=CARTESIAN_POINT('Ctrl Pts',(12.3256628518316,34.1666666803226,-46.));
#18077=CARTESIAN_POINT('Ctrl Pts',(23.,33.9583333469893,-39.8371685740842));
#18078=CARTESIAN_POINT('Ctrl Pts',(33.6743371481683,33.7500000136559,-33.6743371481684));
#18079=CARTESIAN_POINT('Ctrl Pts',(39.8371685740842,33.5416666803226,-23.));
#18080=CARTESIAN_POINT('Ctrl Pts',(46.,33.3333333469893,-12.3256628518317));
#18081=CARTESIAN_POINT('Ctrl Pts',(46.,33.1250000136559,-5.63337527607782E-15));
#18082=CARTESIAN_POINT('Ctrl Pts',(46.,32.9166666803226,12.3256628518316));
#18083=CARTESIAN_POINT('Ctrl Pts',(39.8371685740842,32.7083333469893,23.));
#18084=CARTESIAN_POINT('Ctrl Pts',(33.6743371481684,32.5000000136559,33.6743371481683));
#18085=CARTESIAN_POINT('Ctrl Pts',(23.,32.2916666803226,39.8371685740842));
#18086=CARTESIAN_POINT('Ctrl Pts',(12.3256628518317,32.0833333469893,46.));
#18087=CARTESIAN_POINT('Ctrl Pts',(8.45006291411674E-15,31.8750000136559,
46.));
#18088=CARTESIAN_POINT('Ctrl Pts',(-12.3256628518316,31.6666666803226,46.));
#18089=CARTESIAN_POINT('Ctrl Pts',(-23.,31.4583333469893,39.8371685740842));
#18090=CARTESIAN_POINT('Ctrl Pts',(-33.6743371481683,31.2500000136559,33.6743371481684));
#18091=CARTESIAN_POINT('Ctrl Pts',(-39.8371685740842,31.0416666803226,23.));
#18092=CARTESIAN_POINT('Ctrl Pts',(-46.,30.8333333469893,12.3256628518317));
#18093=CARTESIAN_POINT('Ctrl Pts',(-46.,30.6250000136559,0.));
#18094=CARTESIAN_POINT('Ctrl Pts',(-46.,30.4166666803226,-12.3256628518316));
#18095=CARTESIAN_POINT('Ctrl Pts',(-39.8371685740842,30.2083333469893,-23.));
#18096=CARTESIAN_POINT('Ctrl Pts',(-33.6743371481684,30.0000000136559,-33.6743371481684));
#18097=CARTESIAN_POINT('Ctrl Pts',(-23.,29.7916666803226,-39.8371685740842));
#18098=CARTESIAN_POINT('Ctrl Pts',(-12.3256628518317,29.5833333469893,-46.));
#18099=CARTESIAN_POINT('Ctrl Pts',(-2.81668763803891E-15,29.3750000136559,
-46.));
#18100=CARTESIAN_POINT('Ctrl Pts',(12.3256628518316,29.1666666803226,-46.));
#18101=CARTESIAN_POINT('Ctrl Pts',(23.,28.9583333469893,-39.8371685740842));
#18102=CARTESIAN_POINT('Ctrl Pts',(33.6743371481683,28.7500000136559,-33.6743371481684));
#18103=CARTESIAN_POINT('Ctrl Pts',(39.8371685740842,28.5416666803226,-23.));
#18104=CARTESIAN_POINT('Ctrl Pts',(46.,28.3333333469893,-12.3256628518317));
#18105=CARTESIAN_POINT('Ctrl Pts',(46.,28.1250000136559,-5.63337527607782E-15));
#18106=CARTESIAN_POINT('Ctrl Pts',(46.,27.9166666803226,12.3256628518316));
#18107=CARTESIAN_POINT('Ctrl Pts',(39.8371685740842,27.7083333469893,23.));
#18108=CARTESIAN_POINT('Ctrl Pts',(33.6743371481684,27.5000000136559,33.6743371481683));
#18109=CARTESIAN_POINT('Ctrl Pts',(23.,27.2916666803226,39.8371685740842));
#18110=CARTESIAN_POINT('Ctrl Pts',(12.3256628518317,27.0833333469893,46.));
#18111=CARTESIAN_POINT('Ctrl Pts',(8.45006291411674E-15,26.8750000136559,
46.));
#18112=CARTESIAN_POINT('Ctrl Pts',(-12.3256628518316,26.6666666803226,46.));
#18113=CARTESIAN_POINT('Ctrl Pts',(-23.,26.4583333469893,39.8371685740842));
#18114=CARTESIAN_POINT('Ctrl Pts',(-33.6743371481683,26.2500000136559,33.6743371481684));
#18115=CARTESIAN_POINT('Ctrl Pts',(-39.8371685740842,26.0416666803226,23.));
#18116=CARTESIAN_POINT('Ctrl Pts',(-46.,25.8333333469893,12.3256628518317));
#18117=CARTESIAN_POINT('Ctrl Pts',(-46.,25.6250000136559,0.));
#18118=CARTESIAN_POINT('Ctrl Pts',(-48.706329375,57.187500006828,-1.8898197019151E-14));
#18119=CARTESIAN_POINT('Ctrl Pts',(-48.706329375,56.9791666734946,-13.0508216223155));
#18120=CARTESIAN_POINT('Ctrl Pts',(-42.1809185638422,56.7708333401613,-24.3531646875));
#18121=CARTESIAN_POINT('Ctrl Pts',(-35.6555077526845,56.562500006828,-35.6555077526845));
#18122=CARTESIAN_POINT('Ctrl Pts',(-24.3531646875,56.3541666734946,-42.1809185638423));
#18123=CARTESIAN_POINT('Ctrl Pts',(-13.0508216223155,56.1458333401613,-48.706329375));
#18124=CARTESIAN_POINT('Ctrl Pts',(1.59157945007855E-14,55.937500006828,
-48.706329375));
#18125=CARTESIAN_POINT('Ctrl Pts',(13.0508216223155,55.7291666734946,-48.706329375));
#18126=CARTESIAN_POINT('Ctrl Pts',(24.3531646875,55.5208333401613,-42.1809185638422));
#18127=CARTESIAN_POINT('Ctrl Pts',(35.6555077526845,55.312500006828,-35.6555077526845));
#18128=CARTESIAN_POINT('Ctrl Pts',(42.1809185638422,55.1041666734946,-24.3531646875));
#18129=CARTESIAN_POINT('Ctrl Pts',(48.706329375,54.8958333401613,-13.0508216223155));
#18130=CARTESIAN_POINT('Ctrl Pts',(48.706329375,54.687500006828,1.293339198242E-14));
#18131=CARTESIAN_POINT('Ctrl Pts',(48.706329375,54.4791666734946,13.0508216223155));
#18132=CARTESIAN_POINT('Ctrl Pts',(42.1809185638422,54.2708333401613,24.3531646875));
#18133=CARTESIAN_POINT('Ctrl Pts',(35.6555077526845,54.062500006828,35.6555077526845));
#18134=CARTESIAN_POINT('Ctrl Pts',(24.3531646875,53.8541666734946,42.1809185638422));
#18135=CARTESIAN_POINT('Ctrl Pts',(13.0508216223155,53.6458333401613,48.706329375));
#18136=CARTESIAN_POINT('Ctrl Pts',(-9.95098946405443E-15,53.437500006828,
48.706329375));
#18137=CARTESIAN_POINT('Ctrl Pts',(-13.0508216223155,53.2291666734946,48.706329375));
#18138=CARTESIAN_POINT('Ctrl Pts',(-24.3531646875,53.0208333401613,42.1809185638423));
#18139=CARTESIAN_POINT('Ctrl Pts',(-35.6555077526845,52.812500006828,35.6555077526845));
#18140=CARTESIAN_POINT('Ctrl Pts',(-42.1809185638422,52.6041666734946,24.3531646875));
#18141=CARTESIAN_POINT('Ctrl Pts',(-48.706329375,52.3958333401613,13.0508216223155));
#18142=CARTESIAN_POINT('Ctrl Pts',(-48.706329375,52.187500006828,-1.8898197019151E-14));
#18143=CARTESIAN_POINT('Ctrl Pts',(-48.706329375,51.9791666734946,-13.0508216223155));
#18144=CARTESIAN_POINT('Ctrl Pts',(-42.1809185638422,51.7708333401613,-24.3531646875));
#18145=CARTESIAN_POINT('Ctrl Pts',(-35.6555077526845,51.562500006828,-35.6555077526845));
#18146=CARTESIAN_POINT('Ctrl Pts',(-24.3531646875,51.3541666734946,-42.1809185638423));
#18147=CARTESIAN_POINT('Ctrl Pts',(-13.0508216223155,51.1458333401613,-48.706329375));
#18148=CARTESIAN_POINT('Ctrl Pts',(1.59157945007855E-14,50.937500006828,
-48.706329375));
#18149=CARTESIAN_POINT('Ctrl Pts',(13.0508216223155,50.7291666734946,-48.706329375));
#18150=CARTESIAN_POINT('Ctrl Pts',(24.3531646875,50.5208333401613,-42.1809185638422));
#18151=CARTESIAN_POINT('Ctrl Pts',(35.6555077526845,50.312500006828,-35.6555077526845));
#18152=CARTESIAN_POINT('Ctrl Pts',(42.1809185638422,50.1041666734946,-24.3531646875));
#18153=CARTESIAN_POINT('Ctrl Pts',(48.706329375,49.8958333401613,-13.0508216223155));
#18154=CARTESIAN_POINT('Ctrl Pts',(48.706329375,49.687500006828,1.293339198242E-14));
#18155=CARTESIAN_POINT('Ctrl Pts',(48.706329375,49.4791666734946,13.0508216223155));
#18156=CARTESIAN_POINT('Ctrl Pts',(42.1809185638422,49.2708333401613,24.3531646875));
#18157=CARTESIAN_POINT('Ctrl Pts',(35.6555077526845,49.062500006828,35.6555077526845));
#18158=CARTESIAN_POINT('Ctrl Pts',(24.3531646875,48.8541666734946,42.1809185638422));
#18159=CARTESIAN_POINT('Ctrl Pts',(13.0508216223155,48.6458333401613,48.706329375));
#18160=CARTESIAN_POINT('Ctrl Pts',(-9.95098946405443E-15,48.437500006828,
48.706329375));
#18161=CARTESIAN_POINT('Ctrl Pts',(-13.0508216223155,48.2291666734946,48.706329375));
#18162=CARTESIAN_POINT('Ctrl Pts',(-24.3531646875,48.0208333401613,42.1809185638423));
#18163=CARTESIAN_POINT('Ctrl Pts',(-35.6555077526845,47.812500006828,35.6555077526845));
#18164=CARTESIAN_POINT('Ctrl Pts',(-42.1809185638422,47.6041666734946,24.3531646875));
#18165=CARTESIAN_POINT('Ctrl Pts',(-48.706329375,47.3958333401613,13.0508216223155));
#18166=CARTESIAN_POINT('Ctrl Pts',(-48.706329375,47.187500006828,-1.8898197019151E-14));
#18167=CARTESIAN_POINT('Ctrl Pts',(-48.706329375,46.9791666734946,-13.0508216223155));
#18168=CARTESIAN_POINT('Ctrl Pts',(-42.1809185638422,46.7708333401613,-24.3531646875));
#18169=CARTESIAN_POINT('Ctrl Pts',(-35.6555077526845,46.562500006828,-35.6555077526845));
#18170=CARTESIAN_POINT('Ctrl Pts',(-24.3531646875,46.3541666734946,-42.1809185638423));
#18171=CARTESIAN_POINT('Ctrl Pts',(-13.0508216223155,46.1458333401613,-48.706329375));
#18172=CARTESIAN_POINT('Ctrl Pts',(1.59157945007855E-14,45.937500006828,
-48.706329375));
#18173=CARTESIAN_POINT('Ctrl Pts',(13.0508216223155,45.7291666734946,-48.706329375));
#18174=CARTESIAN_POINT('Ctrl Pts',(24.3531646875,45.5208333401613,-42.1809185638422));
#18175=CARTESIAN_POINT('Ctrl Pts',(35.6555077526845,45.312500006828,-35.6555077526845));
#18176=CARTESIAN_POINT('Ctrl Pts',(42.1809185638422,45.1041666734946,-24.3531646875));
#18177=CARTESIAN_POINT('Ctrl Pts',(48.706329375,44.8958333401613,-13.0508216223155));
#18178=CARTESIAN_POINT('Ctrl Pts',(48.706329375,44.687500006828,1.293339198242E-14));
#18179=CARTESIAN_POINT('Ctrl Pts',(48.706329375,44.4791666734946,13.0508216223155));
#18180=CARTESIAN_POINT('Ctrl Pts',(42.1809185638422,44.2708333401613,24.3531646875));
#18181=CARTESIAN_POINT('Ctrl Pts',(35.6555077526845,44.062500006828,35.6555077526845));
#18182=CARTESIAN_POINT('Ctrl Pts',(24.3531646875,43.8541666734946,42.1809185638422));
#18183=CARTESIAN_POINT('Ctrl Pts',(13.0508216223155,43.6458333401613,48.706329375));
#18184=CARTESIAN_POINT('Ctrl Pts',(-9.95098946405443E-15,43.437500006828,
48.706329375));
#18185=CARTESIAN_POINT('Ctrl Pts',(-13.0508216223155,43.2291666734946,48.706329375));
#18186=CARTESIAN_POINT('Ctrl Pts',(-24.3531646875,43.0208333401613,42.1809185638423));
#18187=CARTESIAN_POINT('Ctrl Pts',(-35.6555077526845,42.812500006828,35.6555077526845));
#18188=CARTESIAN_POINT('Ctrl Pts',(-42.1809185638422,42.6041666734946,24.3531646875));
#18189=CARTESIAN_POINT('Ctrl Pts',(-48.706329375,42.3958333401613,13.0508216223155));
#18190=CARTESIAN_POINT('Ctrl Pts',(-48.706329375,42.187500006828,-1.8898197019151E-14));
#18191=CARTESIAN_POINT('Ctrl Pts',(-48.706329375,41.9791666734946,-13.0508216223155));
#18192=CARTESIAN_POINT('Ctrl Pts',(-42.1809185638422,41.7708333401613,-24.3531646875));
#18193=CARTESIAN_POINT('Ctrl Pts',(-35.6555077526845,41.562500006828,-35.6555077526845));
#18194=CARTESIAN_POINT('Ctrl Pts',(-24.3531646875,41.3541666734946,-42.1809185638423));
#18195=CARTESIAN_POINT('Ctrl Pts',(-13.0508216223155,41.1458333401613,-48.706329375));
#18196=CARTESIAN_POINT('Ctrl Pts',(1.59157945007855E-14,40.937500006828,
-48.706329375));
#18197=CARTESIAN_POINT('Ctrl Pts',(13.0508216223155,40.7291666734946,-48.706329375));
#18198=CARTESIAN_POINT('Ctrl Pts',(24.3531646875,40.5208333401613,-42.1809185638422));
#18199=CARTESIAN_POINT('Ctrl Pts',(35.6555077526845,40.312500006828,-35.6555077526845));
#18200=CARTESIAN_POINT('Ctrl Pts',(42.1809185638422,40.1041666734946,-24.3531646875));
#18201=CARTESIAN_POINT('Ctrl Pts',(48.706329375,39.8958333401613,-13.0508216223155));
#18202=CARTESIAN_POINT('Ctrl Pts',(48.706329375,39.687500006828,1.293339198242E-14));
#18203=CARTESIAN_POINT('Ctrl Pts',(48.706329375,39.4791666734946,13.0508216223155));
#18204=CARTESIAN_POINT('Ctrl Pts',(42.1809185638422,39.2708333401613,24.3531646875));
#18205=CARTESIAN_POINT('Ctrl Pts',(35.6555077526845,39.062500006828,35.6555077526845));
#18206=CARTESIAN_POINT('Ctrl Pts',(24.3531646875,38.8541666734946,42.1809185638422));
#18207=CARTESIAN_POINT('Ctrl Pts',(13.0508216223155,38.6458333401613,48.706329375));
#18208=CARTESIAN_POINT('Ctrl Pts',(-9.95098946405443E-15,38.437500006828,
48.706329375));
#18209=CARTESIAN_POINT('Ctrl Pts',(-13.0508216223155,38.2291666734946,48.706329375));
#18210=CARTESIAN_POINT('Ctrl Pts',(-24.3531646875,38.0208333401613,42.1809185638423));
#18211=CARTESIAN_POINT('Ctrl Pts',(-35.6555077526845,37.812500006828,35.6555077526845));
#18212=CARTESIAN_POINT('Ctrl Pts',(-42.1809185638422,37.6041666734946,24.3531646875));
#18213=CARTESIAN_POINT('Ctrl Pts',(-48.706329375,37.3958333401613,13.0508216223155));
#18214=CARTESIAN_POINT('Ctrl Pts',(-48.706329375,37.187500006828,-1.8898197019151E-14));
#18215=CARTESIAN_POINT('Ctrl Pts',(-48.706329375,36.9791666734946,-13.0508216223155));
#18216=CARTESIAN_POINT('Ctrl Pts',(-42.1809185638422,36.7708333401613,-24.3531646875));
#18217=CARTESIAN_POINT('Ctrl Pts',(-35.6555077526845,36.562500006828,-35.6555077526845));
#18218=CARTESIAN_POINT('Ctrl Pts',(-24.3531646875,36.3541666734946,-42.1809185638423));
#18219=CARTESIAN_POINT('Ctrl Pts',(-13.0508216223155,36.1458333401613,-48.706329375));
#18220=CARTESIAN_POINT('Ctrl Pts',(1.59157945007855E-14,35.937500006828,
-48.706329375));
#18221=CARTESIAN_POINT('Ctrl Pts',(13.0508216223155,35.7291666734946,-48.706329375));
#18222=CARTESIAN_POINT('Ctrl Pts',(24.3531646875,35.5208333401613,-42.1809185638422));
#18223=CARTESIAN_POINT('Ctrl Pts',(35.6555077526845,35.312500006828,-35.6555077526845));
#18224=CARTESIAN_POINT('Ctrl Pts',(42.1809185638422,35.1041666734946,-24.3531646875));
#18225=CARTESIAN_POINT('Ctrl Pts',(48.706329375,34.8958333401613,-13.0508216223155));
#18226=CARTESIAN_POINT('Ctrl Pts',(48.706329375,34.687500006828,1.293339198242E-14));
#18227=CARTESIAN_POINT('Ctrl Pts',(48.706329375,34.4791666734946,13.0508216223155));
#18228=CARTESIAN_POINT('Ctrl Pts',(42.1809185638422,34.2708333401613,24.3531646875));
#18229=CARTESIAN_POINT('Ctrl Pts',(35.6555077526845,34.062500006828,35.6555077526845));
#18230=CARTESIAN_POINT('Ctrl Pts',(24.3531646875,33.8541666734946,42.1809185638422));
#18231=CARTESIAN_POINT('Ctrl Pts',(13.0508216223155,33.6458333401613,48.706329375));
#18232=CARTESIAN_POINT('Ctrl Pts',(-9.95098946405443E-15,33.437500006828,
48.706329375));
#18233=CARTESIAN_POINT('Ctrl Pts',(-13.0508216223155,33.2291666734946,48.706329375));
#18234=CARTESIAN_POINT('Ctrl Pts',(-24.3531646875,33.0208333401613,42.1809185638423));
#18235=CARTESIAN_POINT('Ctrl Pts',(-35.6555077526845,32.812500006828,35.6555077526845));
#18236=CARTESIAN_POINT('Ctrl Pts',(-42.1809185638422,32.6041666734946,24.3531646875));
#18237=CARTESIAN_POINT('Ctrl Pts',(-48.706329375,32.3958333401613,13.0508216223155));
#18238=CARTESIAN_POINT('Ctrl Pts',(-48.706329375,32.187500006828,-1.8898197019151E-14));
#18239=CARTESIAN_POINT('Ctrl Pts',(-48.706329375,31.9791666734946,-13.0508216223155));
#18240=CARTESIAN_POINT('Ctrl Pts',(-42.1809185638422,31.7708333401613,-24.3531646875));
#18241=CARTESIAN_POINT('Ctrl Pts',(-35.6555077526845,31.562500006828,-35.6555077526845));
#18242=CARTESIAN_POINT('Ctrl Pts',(-24.3531646875,31.3541666734946,-42.1809185638423));
#18243=CARTESIAN_POINT('Ctrl Pts',(-13.0508216223155,31.1458333401613,-48.706329375));
#18244=CARTESIAN_POINT('Ctrl Pts',(1.59157945007855E-14,30.937500006828,
-48.706329375));
#18245=CARTESIAN_POINT('Ctrl Pts',(13.0508216223155,30.7291666734946,-48.706329375));
#18246=CARTESIAN_POINT('Ctrl Pts',(24.3531646875,30.5208333401613,-42.1809185638422));
#18247=CARTESIAN_POINT('Ctrl Pts',(35.6555077526845,30.312500006828,-35.6555077526845));
#18248=CARTESIAN_POINT('Ctrl Pts',(42.1809185638422,30.1041666734946,-24.3531646875));
#18249=CARTESIAN_POINT('Ctrl Pts',(48.706329375,29.8958333401613,-13.0508216223155));
#18250=CARTESIAN_POINT('Ctrl Pts',(48.706329375,29.687500006828,1.293339198242E-14));
#18251=CARTESIAN_POINT('Ctrl Pts',(48.706329375,29.4791666734946,13.0508216223155));
#18252=CARTESIAN_POINT('Ctrl Pts',(42.1809185638422,29.2708333401613,24.3531646875));
#18253=CARTESIAN_POINT('Ctrl Pts',(35.6555077526845,29.062500006828,35.6555077526845));
#18254=CARTESIAN_POINT('Ctrl Pts',(24.3531646875,28.8541666734946,42.1809185638422));
#18255=CARTESIAN_POINT('Ctrl Pts',(13.0508216223155,28.6458333401613,48.706329375));
#18256=CARTESIAN_POINT('Ctrl Pts',(-9.95098946405443E-15,28.437500006828,
48.706329375));
#18257=CARTESIAN_POINT('Ctrl Pts',(-13.0508216223155,28.2291666734946,48.706329375));
#18258=CARTESIAN_POINT('Ctrl Pts',(-24.3531646875,28.0208333401613,42.1809185638423));
#18259=CARTESIAN_POINT('Ctrl Pts',(-35.6555077526845,27.812500006828,35.6555077526845));
#18260=CARTESIAN_POINT('Ctrl Pts',(-42.1809185638422,27.6041666734946,24.3531646875));
#18261=CARTESIAN_POINT('Ctrl Pts',(-48.706329375,27.3958333401613,13.0508216223155));
#18262=CARTESIAN_POINT('Ctrl Pts',(-48.706329375,27.187500006828,-1.8898197019151E-14));
#18263=CARTESIAN_POINT('',(45.8814375100776,28.0686756582683,3.30055934787433));
#18264=CARTESIAN_POINT('',(48.5181022360497,29.5979138251126,3.60701400320334));
#18265=CARTESIAN_POINT('Ctrl Pts',(45.8814375100777,28.0686756582683,3.30055934787429));
#18266=CARTESIAN_POINT('Ctrl Pts',(46.3128558578264,28.3201957499304,3.40558477255907));
#18267=CARTESIAN_POINT('Ctrl Pts',(46.7525547486081,28.5759183229237,3.48196024335446));
#18268=CARTESIAN_POINT('Ctrl Pts',(47.6315848511997,29.085761698813,3.5823978354635));
#18269=CARTESIAN_POINT('Ctrl Pts',(48.0757758296302,29.3427063296139,3.60701400320394));
#18270=CARTESIAN_POINT('Ctrl Pts',(48.5181022360497,29.5979138251126,3.60701400320325));
#18271=CARTESIAN_POINT('',(48.5725845633798,29.6293483229262,3.60701400320327));
#18272=CARTESIAN_POINT('',(48.5181022360497,29.5979138251126,3.60701400320334));
#18273=CARTESIAN_POINT('',(-25.470688436697,28.,41.5156663411139));
#18274=CARTESIAN_POINT('Ctrl Pts',(48.5725845633798,29.6293483229262,3.60701400320327));
#18275=CARTESIAN_POINT('Ctrl Pts',(47.7480251419552,29.4485714020251,14.7106532430575));
#18276=CARTESIAN_POINT('Ctrl Pts',(42.1809185638422,29.2708333401613,24.3531646875));
#18277=CARTESIAN_POINT('Ctrl Pts',(35.6555077526845,29.062500006828,35.6555077526845));
#18278=CARTESIAN_POINT('Ctrl Pts',(24.3531646875,28.8541666734946,42.1809185638422));
#18279=CARTESIAN_POINT('Ctrl Pts',(13.0508216223155,28.6458333401613,48.706329375));
#18280=CARTESIAN_POINT('Ctrl Pts',(-9.95098946405443E-15,28.437500006828,
48.706329375));
#18281=CARTESIAN_POINT('Ctrl Pts',(-13.0508216223155,28.2291666734946,48.706329375));
#18282=CARTESIAN_POINT('Ctrl Pts',(-24.3531646875,28.0208333401613,42.1809185638423));
#18283=CARTESIAN_POINT('Ctrl Pts',(-24.9163678135483,28.0104519542914,41.8557530874098));
#18284=CARTESIAN_POINT('Ctrl Pts',(-25.470688436697,28.,41.5156663411139));
#18285=CARTESIAN_POINT('',(45.4263991839739,28.,7.24170264359533));
#18286=CARTESIAN_POINT('Ctrl Pts',(-25.470688436697,28.,41.5156663411139));
#18287=CARTESIAN_POINT('Ctrl Pts',(-23.6703350842583,28.,42.5523965045972));
#18288=CARTESIAN_POINT('Ctrl Pts',(-21.81189807311,28.0000000000232,43.4701513578078));
#18289=CARTESIAN_POINT('Ctrl Pts',(-18.0206934377531,28.0000000000232,45.0463202583268));
#18290=CARTESIAN_POINT('Ctrl Pts',(-16.1003577817121,28.,45.7062614770701));
#18291=CARTESIAN_POINT('Ctrl Pts',(-10.2442149716332,28.,47.3145402613375));
#18292=CARTESIAN_POINT('Ctrl Pts',(-6.22509096152426,28.,47.8914048604989));
#18293=CARTESIAN_POINT('Ctrl Pts',(-1.01023763277435,28.,47.9805573793013));
#18294=CARTESIAN_POINT('Ctrl Pts',(0.168261352715039,28.,47.9580910618091));
#18295=CARTESIAN_POINT('Ctrl Pts',(7.53171066766197,28.,47.5428134300488));
#18296=CARTESIAN_POINT('Ctrl Pts',(13.5927405733154,28.,45.9875890675615));
#18297=CARTESIAN_POINT('Ctrl Pts',(21.9842976922167,28.,41.975061721578));
#18298=CARTESIAN_POINT('Ctrl Pts',(24.6631550733832,28.,40.3575666553121));
#18299=CARTESIAN_POINT('Ctrl Pts',(31.9704924411577,28.,34.8747898052096));
#18300=CARTESIAN_POINT('Ctrl Pts',(36.0419398812146,28.,30.37145046818));
#18301=CARTESIAN_POINT('Ctrl Pts',(39.9915074797196,28.,23.8278896741577));
#18302=CARTESIAN_POINT('Ctrl Pts',(40.7638953703109,28.,22.3840580410818));
#18303=CARTESIAN_POINT('Ctrl Pts',(43.4788432880031,28.,16.5807834518621));
#18304=CARTESIAN_POINT('Ctrl Pts',(44.8177402925238,28.,11.9727439180169));
#18305=CARTESIAN_POINT('Ctrl Pts',(45.4263991839739,28.,7.24170264359532));
#18306=CARTESIAN_POINT('Origin',(-0.013153225928777,27.9166674358441,-0.0035690946937661));
#18307=CARTESIAN_POINT('Origin',(-7.99360577730113E-14,57.8125000068276,
4.34631818602828E-14));
#18308=CARTESIAN_POINT('',(-3.58014543786854,34.6297857346188,48.5745723586909));
#18309=CARTESIAN_POINT('',(-48.5725845633798,33.4956516907297,3.60701400320325));
#18310=CARTESIAN_POINT('Ctrl Pts',(-3.58014543786854,34.6297857346188,48.5745723586909));
#18311=CARTESIAN_POINT('Ctrl Pts',(-14.6983765927309,34.4487976945266,47.755113069326));
#18312=CARTESIAN_POINT('Ctrl Pts',(-24.3531646875,34.2708333401613,42.1809185638423));
#18313=CARTESIAN_POINT('Ctrl Pts',(-35.6555077526845,34.062500006828,35.6555077526845));
#18314=CARTESIAN_POINT('Ctrl Pts',(-42.1809185638422,33.8541666734946,24.3531646875));
#18315=CARTESIAN_POINT('Ctrl Pts',(-47.7480251419552,33.6764286116308,14.7106532430575));
#18316=CARTESIAN_POINT('Ctrl Pts',(-48.5725845633798,33.4956516907297,3.60701400320325));
#18317=CARTESIAN_POINT('',(-48.5725845633798,33.4956516907297,3.60701400320325));
#18318=CARTESIAN_POINT('Ctrl Pts',(-2.14849279754675,33.4030003256338,48.658920044375));
#18319=CARTESIAN_POINT('Ctrl Pts',(-2.53041200358172,33.5963625381787,48.6420567300503));
#18320=CARTESIAN_POINT('Ctrl Pts',(-2.8769017960051,33.8521925418285,48.6221324989406));
#18321=CARTESIAN_POINT('Ctrl Pts',(-3.31108160489208,34.2864277377636,48.5938831734733));
#18322=CARTESIAN_POINT('Ctrl Pts',(-3.45216898319886,34.4514646385294,48.584004748892));
#18323=CARTESIAN_POINT('Ctrl Pts',(-3.58014543786852,34.6297857346188,48.5745723586909));
#18324=CARTESIAN_POINT('Origin',(-7.99360577730113E-14,57.8125000068276,
4.34631818602828E-14));
#18325=CARTESIAN_POINT('',(-48.5134353784345,33.3675463684955,-4.33048599679665));
#18326=CARTESIAN_POINT('',(48.5134353784344,31.0074536451604,-4.33048599679682));
#18327=CARTESIAN_POINT('Ctrl Pts',(-48.5134353784345,33.3675463684955,-4.33048599679665));
#18328=CARTESIAN_POINT('Ctrl Pts',(-47.5573898704235,33.1924850907233,-15.040843219065));
#18329=CARTESIAN_POINT('Ctrl Pts',(-42.1809185638422,33.0208333401613,-24.3531646875));
#18330=CARTESIAN_POINT('Ctrl Pts',(-35.6555077526845,32.812500006828,-35.6555077526845));
#18331=CARTESIAN_POINT('Ctrl Pts',(-24.3531646875,32.6041666734946,-42.1809185638422));
#18332=CARTESIAN_POINT('Ctrl Pts',(-13.0508216223155,32.3958333401613,-48.706329375));
#18333=CARTESIAN_POINT('Ctrl Pts',(1.59157945007855E-14,32.187500006828,
-48.706329375));
#18334=CARTESIAN_POINT('Ctrl Pts',(13.0508216223155,31.9791666734946,-48.706329375));
#18335=CARTESIAN_POINT('Ctrl Pts',(24.3531646875,31.7708333401613,-42.1809185638422));
#18336=CARTESIAN_POINT('Ctrl Pts',(35.6555077526845,31.562500006828,-35.6555077526845));
#18337=CARTESIAN_POINT('Ctrl Pts',(42.1809185638422,31.3541666734946,-24.3531646875));
#18338=CARTESIAN_POINT('Ctrl Pts',(47.5573898704234,31.1825149229327,-15.0408432190651));
#18339=CARTESIAN_POINT('Ctrl Pts',(48.5134353784344,31.0074536451604,-4.33048599679682));
#18340=CARTESIAN_POINT('',(48.5134353784344,31.0074536451604,-4.33048599679682));
#18341=CARTESIAN_POINT('',(-48.5134353784345,32.1175463684955,-4.33048599679665));
#18342=CARTESIAN_POINT('Origin',(-7.99360577730113E-14,57.8125000068276,
4.34631818602828E-14));
#18343=CARTESIAN_POINT('',(48.5725845633798,30.8793483229262,3.60701400320327));
#18344=CARTESIAN_POINT('',(48.5725845633798,29.6293483229262,3.60701400320327));
#18345=CARTESIAN_POINT('',(-48.5839797682363,28.4930986521586,3.45013493440411));
#18346=CARTESIAN_POINT('Ctrl Pts',(48.5725845633798,30.8793483229262,3.60701400320327));
#18347=CARTESIAN_POINT('Ctrl Pts',(47.7480251419552,30.6985714020251,14.7106532430575));
#18348=CARTESIAN_POINT('Ctrl Pts',(42.1809185638422,30.5208333401613,24.3531646875));
#18349=CARTESIAN_POINT('Ctrl Pts',(35.6555077526845,30.312500006828,35.6555077526845));
#18350=CARTESIAN_POINT('Ctrl Pts',(24.3531646875,30.1041666734946,42.1809185638422));
#18351=CARTESIAN_POINT('Ctrl Pts',(13.0508216223155,29.8958333401613,48.706329375));
#18352=CARTESIAN_POINT('Ctrl Pts',(-9.95098946405443E-15,29.687500006828,
48.706329375));
#18353=CARTESIAN_POINT('Ctrl Pts',(-13.0508216223155,29.4791666734946,48.706329375));
#18354=CARTESIAN_POINT('Ctrl Pts',(-24.3531646875,29.2708333401613,42.1809185638423));
#18355=CARTESIAN_POINT('Ctrl Pts',(-35.6555077526845,29.062500006828,35.6555077526845));
#18356=CARTESIAN_POINT('Ctrl Pts',(-42.1809185638422,28.8541666734946,24.3531646875));
#18357=CARTESIAN_POINT('Ctrl Pts',(-47.7894184949761,28.6751070679821,14.6389578525296));
#18358=CARTESIAN_POINT('Ctrl Pts',(-48.5839797682363,28.4930986521586,3.45013493440411));
#18359=CARTESIAN_POINT('',(-48.5963608758988,28.,3.27112072623103));
#18360=CARTESIAN_POINT('Ctrl Pts',(-48.5839797682365,28.4930986521586,3.45013493440413));
#18361=CARTESIAN_POINT('Ctrl Pts',(-48.5868672036625,28.352811517686,3.40947475531321));
#18362=CARTESIAN_POINT('Ctrl Pts',(-48.5902683144096,28.2142234168628,3.36087918405085));
#18363=CARTESIAN_POINT('Ctrl Pts',(-48.5948275946602,28.0524147745889,3.2938385397297));
#18364=CARTESIAN_POINT('Ctrl Pts',(-48.5955868421039,28.0261433967151,3.28261991219711));
#18365=CARTESIAN_POINT('Ctrl Pts',(-48.5963608758972,28.,3.27112072623101));
#18366=CARTESIAN_POINT('Origin',(7.105427357601E-14,28.0000000000001,-4.66293670342566E-14));
#18367=CARTESIAN_POINT('Ctrl Pts',(-48.706329375,58.437500006828,-1.8898197019151E-14));
#18368=CARTESIAN_POINT('Ctrl Pts',(-48.706329375,58.2291666734946,-13.0508216223155));
#18369=CARTESIAN_POINT('Ctrl Pts',(-42.1809185638422,58.0208333401613,-24.3531646875));
#18370=CARTESIAN_POINT('Ctrl Pts',(-35.6555077526845,57.812500006828,-35.6555077526845));
#18371=CARTESIAN_POINT('Ctrl Pts',(-24.3531646875,57.6041666734946,-42.1809185638422));
#18372=CARTESIAN_POINT('Ctrl Pts',(-13.0508216223155,57.3958333401613,-48.706329375));
#18373=CARTESIAN_POINT('Ctrl Pts',(1.59157945007855E-14,57.187500006828,
-48.706329375));
#18374=CARTESIAN_POINT('Ctrl Pts',(13.0508216223155,56.9791666734946,-48.706329375));
#18375=CARTESIAN_POINT('Ctrl Pts',(24.3531646875,56.7708333401613,-42.1809185638422));
#18376=CARTESIAN_POINT('Ctrl Pts',(35.6555077526845,56.562500006828,-35.6555077526845));
#18377=CARTESIAN_POINT('Ctrl Pts',(42.1809185638422,56.3541666734946,-24.3531646875));
#18378=CARTESIAN_POINT('Ctrl Pts',(48.706329375,56.1458333401613,-13.0508216223155));
#18379=CARTESIAN_POINT('Ctrl Pts',(48.706329375,55.937500006828,1.293339198242E-14));
#18380=CARTESIAN_POINT('Ctrl Pts',(48.706329375,55.7291666734946,13.0508216223155));
#18381=CARTESIAN_POINT('Ctrl Pts',(42.1809185638422,55.5208333401613,24.3531646875));
#18382=CARTESIAN_POINT('Ctrl Pts',(35.6555077526845,55.312500006828,35.6555077526845));
#18383=CARTESIAN_POINT('Ctrl Pts',(24.3531646875,55.1041666734946,42.1809185638422));
#18384=CARTESIAN_POINT('Ctrl Pts',(13.0508216223155,54.8958333401613,48.706329375));
#18385=CARTESIAN_POINT('Ctrl Pts',(-9.95098946405443E-15,54.687500006828,
48.706329375));
#18386=CARTESIAN_POINT('Ctrl Pts',(-13.0508216223155,54.4791666734946,48.706329375));
#18387=CARTESIAN_POINT('Ctrl Pts',(-24.3531646875,54.2708333401613,42.1809185638423));
#18388=CARTESIAN_POINT('Ctrl Pts',(-35.6555077526845,54.062500006828,35.6555077526845));
#18389=CARTESIAN_POINT('Ctrl Pts',(-42.1809185638422,53.8541666734946,24.3531646875));
#18390=CARTESIAN_POINT('Ctrl Pts',(-48.706329375,53.6458333401613,13.0508216223155));
#18391=CARTESIAN_POINT('Ctrl Pts',(-48.706329375,53.437500006828,-1.8898197019151E-14));
#18392=CARTESIAN_POINT('Ctrl Pts',(-48.706329375,53.2291666734946,-13.0508216223155));
#18393=CARTESIAN_POINT('Ctrl Pts',(-42.1809185638422,53.0208333401613,-24.3531646875));
#18394=CARTESIAN_POINT('Ctrl Pts',(-35.6555077526845,52.812500006828,-35.6555077526845));
#18395=CARTESIAN_POINT('Ctrl Pts',(-24.3531646875,52.6041666734946,-42.1809185638422));
#18396=CARTESIAN_POINT('Ctrl Pts',(-13.0508216223155,52.3958333401613,-48.706329375));
#18397=CARTESIAN_POINT('Ctrl Pts',(1.59157945007855E-14,52.187500006828,
-48.706329375));
#18398=CARTESIAN_POINT('Ctrl Pts',(13.0508216223155,51.9791666734946,-48.706329375));
#18399=CARTESIAN_POINT('Ctrl Pts',(24.3531646875,51.7708333401613,-42.1809185638422));
#18400=CARTESIAN_POINT('Ctrl Pts',(35.6555077526845,51.562500006828,-35.6555077526845));
#18401=CARTESIAN_POINT('Ctrl Pts',(42.1809185638422,51.3541666734946,-24.3531646875));
#18402=CARTESIAN_POINT('Ctrl Pts',(48.706329375,51.1458333401613,-13.0508216223155));
#18403=CARTESIAN_POINT('Ctrl Pts',(48.706329375,50.937500006828,1.293339198242E-14));
#18404=CARTESIAN_POINT('Ctrl Pts',(48.706329375,50.7291666734946,13.0508216223155));
#18405=CARTESIAN_POINT('Ctrl Pts',(42.1809185638422,50.5208333401613,24.3531646875));
#18406=CARTESIAN_POINT('Ctrl Pts',(35.6555077526845,50.312500006828,35.6555077526845));
#18407=CARTESIAN_POINT('Ctrl Pts',(24.3531646875,50.1041666734946,42.1809185638422));
#18408=CARTESIAN_POINT('Ctrl Pts',(13.0508216223155,49.8958333401613,48.706329375));
#18409=CARTESIAN_POINT('Ctrl Pts',(-9.95098946405443E-15,49.687500006828,
48.706329375));
#18410=CARTESIAN_POINT('Ctrl Pts',(-13.0508216223155,49.4791666734946,48.706329375));
#18411=CARTESIAN_POINT('Ctrl Pts',(-24.3531646875,49.2708333401613,42.1809185638423));
#18412=CARTESIAN_POINT('Ctrl Pts',(-35.6555077526845,49.062500006828,35.6555077526845));
#18413=CARTESIAN_POINT('Ctrl Pts',(-42.1809185638422,48.8541666734946,24.3531646875));
#18414=CARTESIAN_POINT('Ctrl Pts',(-48.706329375,48.6458333401613,13.0508216223155));
#18415=CARTESIAN_POINT('Ctrl Pts',(-48.706329375,48.437500006828,-1.8898197019151E-14));
#18416=CARTESIAN_POINT('Ctrl Pts',(-48.706329375,48.2291666734946,-13.0508216223155));
#18417=CARTESIAN_POINT('Ctrl Pts',(-42.1809185638422,48.0208333401613,-24.3531646875));
#18418=CARTESIAN_POINT('Ctrl Pts',(-35.6555077526845,47.812500006828,-35.6555077526845));
#18419=CARTESIAN_POINT('Ctrl Pts',(-24.3531646875,47.6041666734946,-42.1809185638422));
#18420=CARTESIAN_POINT('Ctrl Pts',(-13.0508216223155,47.3958333401613,-48.706329375));
#18421=CARTESIAN_POINT('Ctrl Pts',(1.59157945007855E-14,47.187500006828,
-48.706329375));
#18422=CARTESIAN_POINT('Ctrl Pts',(13.0508216223155,46.9791666734946,-48.706329375));
#18423=CARTESIAN_POINT('Ctrl Pts',(24.3531646875,46.7708333401613,-42.1809185638422));
#18424=CARTESIAN_POINT('Ctrl Pts',(35.6555077526845,46.562500006828,-35.6555077526845));
#18425=CARTESIAN_POINT('Ctrl Pts',(42.1809185638422,46.3541666734946,-24.3531646875));
#18426=CARTESIAN_POINT('Ctrl Pts',(48.706329375,46.1458333401613,-13.0508216223155));
#18427=CARTESIAN_POINT('Ctrl Pts',(48.706329375,45.937500006828,1.293339198242E-14));
#18428=CARTESIAN_POINT('Ctrl Pts',(48.706329375,45.7291666734946,13.0508216223155));
#18429=CARTESIAN_POINT('Ctrl Pts',(42.1809185638422,45.5208333401613,24.3531646875));
#18430=CARTESIAN_POINT('Ctrl Pts',(35.6555077526845,45.312500006828,35.6555077526845));
#18431=CARTESIAN_POINT('Ctrl Pts',(24.3531646875,45.1041666734946,42.1809185638422));
#18432=CARTESIAN_POINT('Ctrl Pts',(13.0508216223155,44.8958333401613,48.706329375));
#18433=CARTESIAN_POINT('Ctrl Pts',(-9.95098946405443E-15,44.687500006828,
48.706329375));
#18434=CARTESIAN_POINT('Ctrl Pts',(-13.0508216223155,44.4791666734946,48.706329375));
#18435=CARTESIAN_POINT('Ctrl Pts',(-24.3531646875,44.2708333401613,42.1809185638423));
#18436=CARTESIAN_POINT('Ctrl Pts',(-35.6555077526845,44.062500006828,35.6555077526845));
#18437=CARTESIAN_POINT('Ctrl Pts',(-42.1809185638422,43.8541666734946,24.3531646875));
#18438=CARTESIAN_POINT('Ctrl Pts',(-48.706329375,43.6458333401613,13.0508216223155));
#18439=CARTESIAN_POINT('Ctrl Pts',(-48.706329375,43.437500006828,-1.8898197019151E-14));
#18440=CARTESIAN_POINT('Ctrl Pts',(-48.706329375,43.2291666734946,-13.0508216223155));
#18441=CARTESIAN_POINT('Ctrl Pts',(-42.1809185638422,43.0208333401613,-24.3531646875));
#18442=CARTESIAN_POINT('Ctrl Pts',(-35.6555077526845,42.812500006828,-35.6555077526845));
#18443=CARTESIAN_POINT('Ctrl Pts',(-24.3531646875,42.6041666734946,-42.1809185638422));
#18444=CARTESIAN_POINT('Ctrl Pts',(-13.0508216223155,42.3958333401613,-48.706329375));
#18445=CARTESIAN_POINT('Ctrl Pts',(1.59157945007855E-14,42.187500006828,
-48.706329375));
#18446=CARTESIAN_POINT('Ctrl Pts',(13.0508216223155,41.9791666734946,-48.706329375));
#18447=CARTESIAN_POINT('Ctrl Pts',(24.3531646875,41.7708333401613,-42.1809185638422));
#18448=CARTESIAN_POINT('Ctrl Pts',(35.6555077526845,41.562500006828,-35.6555077526845));
#18449=CARTESIAN_POINT('Ctrl Pts',(42.1809185638422,41.3541666734946,-24.3531646875));
#18450=CARTESIAN_POINT('Ctrl Pts',(48.706329375,41.1458333401613,-13.0508216223155));
#18451=CARTESIAN_POINT('Ctrl Pts',(48.706329375,40.937500006828,1.293339198242E-14));
#18452=CARTESIAN_POINT('Ctrl Pts',(48.706329375,40.7291666734946,13.0508216223155));
#18453=CARTESIAN_POINT('Ctrl Pts',(42.1809185638422,40.5208333401613,24.3531646875));
#18454=CARTESIAN_POINT('Ctrl Pts',(35.6555077526845,40.312500006828,35.6555077526845));
#18455=CARTESIAN_POINT('Ctrl Pts',(24.3531646875,40.1041666734946,42.1809185638422));
#18456=CARTESIAN_POINT('Ctrl Pts',(13.0508216223155,39.8958333401613,48.706329375));
#18457=CARTESIAN_POINT('Ctrl Pts',(-9.95098946405443E-15,39.687500006828,
48.706329375));
#18458=CARTESIAN_POINT('Ctrl Pts',(-13.0508216223155,39.4791666734946,48.706329375));
#18459=CARTESIAN_POINT('Ctrl Pts',(-24.3531646875,39.2708333401613,42.1809185638423));
#18460=CARTESIAN_POINT('Ctrl Pts',(-35.6555077526845,39.062500006828,35.6555077526845));
#18461=CARTESIAN_POINT('Ctrl Pts',(-42.1809185638422,38.8541666734946,24.3531646875));
#18462=CARTESIAN_POINT('Ctrl Pts',(-48.706329375,38.6458333401613,13.0508216223155));
#18463=CARTESIAN_POINT('Ctrl Pts',(-48.706329375,38.437500006828,-1.8898197019151E-14));
#18464=CARTESIAN_POINT('Ctrl Pts',(-48.706329375,38.2291666734946,-13.0508216223155));
#18465=CARTESIAN_POINT('Ctrl Pts',(-42.1809185638422,38.0208333401613,-24.3531646875));
#18466=CARTESIAN_POINT('Ctrl Pts',(-35.6555077526845,37.812500006828,-35.6555077526845));
#18467=CARTESIAN_POINT('Ctrl Pts',(-24.3531646875,37.6041666734946,-42.1809185638422));
#18468=CARTESIAN_POINT('Ctrl Pts',(-13.0508216223155,37.3958333401613,-48.706329375));
#18469=CARTESIAN_POINT('Ctrl Pts',(1.59157945007855E-14,37.187500006828,
-48.706329375));
#18470=CARTESIAN_POINT('Ctrl Pts',(13.0508216223155,36.9791666734946,-48.706329375));
#18471=CARTESIAN_POINT('Ctrl Pts',(24.3531646875,36.7708333401613,-42.1809185638422));
#18472=CARTESIAN_POINT('Ctrl Pts',(35.6555077526845,36.562500006828,-35.6555077526845));
#18473=CARTESIAN_POINT('Ctrl Pts',(42.1809185638422,36.3541666734946,-24.3531646875));
#18474=CARTESIAN_POINT('Ctrl Pts',(48.706329375,36.1458333401613,-13.0508216223155));
#18475=CARTESIAN_POINT('Ctrl Pts',(48.706329375,35.937500006828,1.293339198242E-14));
#18476=CARTESIAN_POINT('Ctrl Pts',(48.706329375,35.7291666734946,13.0508216223155));
#18477=CARTESIAN_POINT('Ctrl Pts',(42.1809185638422,35.5208333401613,24.3531646875));
#18478=CARTESIAN_POINT('Ctrl Pts',(35.6555077526845,35.312500006828,35.6555077526845));
#18479=CARTESIAN_POINT('Ctrl Pts',(24.3531646875,35.1041666734946,42.1809185638422));
#18480=CARTESIAN_POINT('Ctrl Pts',(13.0508216223155,34.8958333401613,48.706329375));
#18481=CARTESIAN_POINT('Ctrl Pts',(-9.95098946405443E-15,34.687500006828,
48.706329375));
#18482=CARTESIAN_POINT('Ctrl Pts',(-13.0508216223155,34.4791666734946,48.706329375));
#18483=CARTESIAN_POINT('Ctrl Pts',(-24.3531646875,34.2708333401613,42.1809185638423));
#18484=CARTESIAN_POINT('Ctrl Pts',(-35.6555077526845,34.062500006828,35.6555077526845));
#18485=CARTESIAN_POINT('Ctrl Pts',(-42.1809185638422,33.8541666734946,24.3531646875));
#18486=CARTESIAN_POINT('Ctrl Pts',(-48.706329375,33.6458333401613,13.0508216223155));
#18487=CARTESIAN_POINT('Ctrl Pts',(-48.706329375,33.437500006828,-1.8898197019151E-14));
#18488=CARTESIAN_POINT('Ctrl Pts',(-48.706329375,33.2291666734946,-13.0508216223155));
#18489=CARTESIAN_POINT('Ctrl Pts',(-42.1809185638422,33.0208333401613,-24.3531646875));
#18490=CARTESIAN_POINT('Ctrl Pts',(-35.6555077526845,32.812500006828,-35.6555077526845));
#18491=CARTESIAN_POINT('Ctrl Pts',(-24.3531646875,32.6041666734946,-42.1809185638422));
#18492=CARTESIAN_POINT('Ctrl Pts',(-13.0508216223155,32.3958333401613,-48.706329375));
#18493=CARTESIAN_POINT('Ctrl Pts',(1.59157945007855E-14,32.187500006828,
-48.706329375));
#18494=CARTESIAN_POINT('Ctrl Pts',(13.0508216223155,31.9791666734946,-48.706329375));
#18495=CARTESIAN_POINT('Ctrl Pts',(24.3531646875,31.7708333401613,-42.1809185638422));
#18496=CARTESIAN_POINT('Ctrl Pts',(35.6555077526845,31.562500006828,-35.6555077526845));
#18497=CARTESIAN_POINT('Ctrl Pts',(42.1809185638422,31.3541666734946,-24.3531646875));
#18498=CARTESIAN_POINT('Ctrl Pts',(48.706329375,31.1458333401613,-13.0508216223155));
#18499=CARTESIAN_POINT('Ctrl Pts',(48.706329375,30.937500006828,1.293339198242E-14));
#18500=CARTESIAN_POINT('Ctrl Pts',(48.706329375,30.7291666734946,13.0508216223155));
#18501=CARTESIAN_POINT('Ctrl Pts',(42.1809185638422,30.5208333401613,24.3531646875));
#18502=CARTESIAN_POINT('Ctrl Pts',(35.6555077526845,30.312500006828,35.6555077526845));
#18503=CARTESIAN_POINT('Ctrl Pts',(24.3531646875,30.1041666734946,42.1809185638422));
#18504=CARTESIAN_POINT('Ctrl Pts',(13.0508216223155,29.8958333401613,48.706329375));
#18505=CARTESIAN_POINT('Ctrl Pts',(-9.95098946405443E-15,29.687500006828,
48.706329375));
#18506=CARTESIAN_POINT('Ctrl Pts',(-13.0508216223155,29.4791666734946,48.706329375));
#18507=CARTESIAN_POINT('Ctrl Pts',(-24.3531646875,29.2708333401613,42.1809185638423));
#18508=CARTESIAN_POINT('Ctrl Pts',(-35.6555077526845,29.062500006828,35.6555077526845));
#18509=CARTESIAN_POINT('Ctrl Pts',(-42.1809185638422,28.8541666734946,24.3531646875));
#18510=CARTESIAN_POINT('Ctrl Pts',(-48.706329375,28.6458333401613,13.0508216223155));
#18511=CARTESIAN_POINT('Ctrl Pts',(-48.706329375,28.437500006828,-1.8898197019151E-14));
#18512=CARTESIAN_POINT('Ctrl Pts',(-45.9999999733281,60.000000015399,1.86248708600067E-22));
#18513=CARTESIAN_POINT('Ctrl Pts',(-45.9999999733281,59.7916666820657,-12.3256628446849));
#18514=CARTESIAN_POINT('Ctrl Pts',(-39.8371685509857,59.5833333487323,-22.9999999866641));
#18515=CARTESIAN_POINT('Ctrl Pts',(-33.6743371286432,59.375000015399,-33.6743371286432));
#18516=CARTESIAN_POINT('Ctrl Pts',(-22.9999999866641,59.1666666820657,-39.8371685509857));
#18517=CARTESIAN_POINT('Ctrl Pts',(-12.3256628446849,58.9583333487323,-45.9999999733281));
#18518=CARTESIAN_POINT('Ctrl Pts',(-2.81668782265444E-15,58.750000015399,
-45.9999999733281));
#18519=CARTESIAN_POINT('Ctrl Pts',(12.3256628446849,58.5416666820657,-45.9999999733281));
#18520=CARTESIAN_POINT('Ctrl Pts',(22.9999999866641,58.3333333487324,-39.8371685509857));
#18521=CARTESIAN_POINT('Ctrl Pts',(33.6743371286432,58.125000015399,-33.6743371286432));
#18522=CARTESIAN_POINT('Ctrl Pts',(39.8371685509856,57.9166666820657,-22.9999999866641));
#18523=CARTESIAN_POINT('Ctrl Pts',(45.9999999733281,57.7083333487323,-12.3256628446849));
#18524=CARTESIAN_POINT('Ctrl Pts',(45.9999999733281,57.500000015399,-5.63337545906017E-15));
#18525=CARTESIAN_POINT('Ctrl Pts',(45.9999999733281,57.2916666820657,12.3256628446849));
#18526=CARTESIAN_POINT('Ctrl Pts',(39.8371685509857,57.0833333487324,22.999999986664));
#18527=CARTESIAN_POINT('Ctrl Pts',(33.6743371286432,56.875000015399,33.6743371286432));
#18528=CARTESIAN_POINT('Ctrl Pts',(22.9999999866641,56.6666666820657,39.8371685509856));
#18529=CARTESIAN_POINT('Ctrl Pts',(12.325662844685,56.4583333487323,45.9999999733281));
#18530=CARTESIAN_POINT('Ctrl Pts',(8.4500630954659E-15,56.250000015399,
45.9999999733281));
#18531=CARTESIAN_POINT('Ctrl Pts',(-12.3256628446849,56.0416666820657,45.9999999733281));
#18532=CARTESIAN_POINT('Ctrl Pts',(-22.999999986664,55.8333333487323,39.8371685509857));
#18533=CARTESIAN_POINT('Ctrl Pts',(-33.6743371286432,55.625000015399,33.6743371286432));
#18534=CARTESIAN_POINT('Ctrl Pts',(-39.8371685509856,55.4166666820657,22.9999999866641));
#18535=CARTESIAN_POINT('Ctrl Pts',(-45.9999999733281,55.2083333487323,12.325662844685));
#18536=CARTESIAN_POINT('Ctrl Pts',(-45.9999999733281,55.000000015399,1.86248708600067E-22));
#18537=CARTESIAN_POINT('Ctrl Pts',(-45.9999999733281,54.7916666820657,-12.3256628446849));
#18538=CARTESIAN_POINT('Ctrl Pts',(-39.8371685509857,54.5833333487323,-22.9999999866641));
#18539=CARTESIAN_POINT('Ctrl Pts',(-33.6743371286432,54.375000015399,-33.6743371286432));
#18540=CARTESIAN_POINT('Ctrl Pts',(-22.9999999866641,54.1666666820657,-39.8371685509857));
#18541=CARTESIAN_POINT('Ctrl Pts',(-12.3256628446849,53.9583333487323,-45.9999999733281));
#18542=CARTESIAN_POINT('Ctrl Pts',(-2.81668782265444E-15,53.750000015399,
-45.9999999733281));
#18543=CARTESIAN_POINT('Ctrl Pts',(12.3256628446849,53.5416666820657,-45.9999999733281));
#18544=CARTESIAN_POINT('Ctrl Pts',(22.9999999866641,53.3333333487323,-39.8371685509857));
#18545=CARTESIAN_POINT('Ctrl Pts',(33.6743371286432,53.125000015399,-33.6743371286432));
#18546=CARTESIAN_POINT('Ctrl Pts',(39.8371685509856,52.9166666820657,-22.9999999866641));
#18547=CARTESIAN_POINT('Ctrl Pts',(45.9999999733281,52.7083333487324,-12.3256628446849));
#18548=CARTESIAN_POINT('Ctrl Pts',(45.9999999733281,52.500000015399,-5.63337545906017E-15));
#18549=CARTESIAN_POINT('Ctrl Pts',(45.9999999733281,52.2916666820657,12.3256628446849));
#18550=CARTESIAN_POINT('Ctrl Pts',(39.8371685509857,52.0833333487323,22.999999986664));
#18551=CARTESIAN_POINT('Ctrl Pts',(33.6743371286432,51.875000015399,33.6743371286432));
#18552=CARTESIAN_POINT('Ctrl Pts',(22.9999999866641,51.6666666820657,39.8371685509856));
#18553=CARTESIAN_POINT('Ctrl Pts',(12.325662844685,51.4583333487323,45.9999999733281));
#18554=CARTESIAN_POINT('Ctrl Pts',(8.4500630954659E-15,51.250000015399,
45.9999999733281));
#18555=CARTESIAN_POINT('Ctrl Pts',(-12.3256628446849,51.0416666820657,45.9999999733281));
#18556=CARTESIAN_POINT('Ctrl Pts',(-22.999999986664,50.8333333487323,39.8371685509857));
#18557=CARTESIAN_POINT('Ctrl Pts',(-33.6743371286432,50.625000015399,33.6743371286432));
#18558=CARTESIAN_POINT('Ctrl Pts',(-39.8371685509856,50.4166666820657,22.9999999866641));
#18559=CARTESIAN_POINT('Ctrl Pts',(-45.9999999733281,50.2083333487323,12.325662844685));
#18560=CARTESIAN_POINT('Ctrl Pts',(-45.9999999733281,50.000000015399,1.86248708600067E-22));
#18561=CARTESIAN_POINT('Ctrl Pts',(-45.9999999733281,49.7916666820657,-12.3256628446849));
#18562=CARTESIAN_POINT('Ctrl Pts',(-39.8371685509857,49.5833333487323,-22.9999999866641));
#18563=CARTESIAN_POINT('Ctrl Pts',(-33.6743371286432,49.375000015399,-33.6743371286432));
#18564=CARTESIAN_POINT('Ctrl Pts',(-22.9999999866641,49.1666666820657,-39.8371685509857));
#18565=CARTESIAN_POINT('Ctrl Pts',(-12.3256628446849,48.9583333487323,-45.9999999733281));
#18566=CARTESIAN_POINT('Ctrl Pts',(-2.81668782265444E-15,48.750000015399,
-45.9999999733281));
#18567=CARTESIAN_POINT('Ctrl Pts',(12.3256628446849,48.5416666820657,-45.9999999733281));
#18568=CARTESIAN_POINT('Ctrl Pts',(22.9999999866641,48.3333333487324,-39.8371685509857));
#18569=CARTESIAN_POINT('Ctrl Pts',(33.6743371286432,48.125000015399,-33.6743371286432));
#18570=CARTESIAN_POINT('Ctrl Pts',(39.8371685509856,47.9166666820657,-22.9999999866641));
#18571=CARTESIAN_POINT('Ctrl Pts',(45.9999999733281,47.7083333487324,-12.3256628446849));
#18572=CARTESIAN_POINT('Ctrl Pts',(45.9999999733281,47.500000015399,-5.63337545906017E-15));
#18573=CARTESIAN_POINT('Ctrl Pts',(45.9999999733281,47.2916666820657,12.3256628446849));
#18574=CARTESIAN_POINT('Ctrl Pts',(39.8371685509857,47.0833333487323,22.999999986664));
#18575=CARTESIAN_POINT('Ctrl Pts',(33.6743371286432,46.875000015399,33.6743371286432));
#18576=CARTESIAN_POINT('Ctrl Pts',(22.9999999866641,46.6666666820657,39.8371685509856));
#18577=CARTESIAN_POINT('Ctrl Pts',(12.325662844685,46.4583333487324,45.9999999733281));
#18578=CARTESIAN_POINT('Ctrl Pts',(8.4500630954659E-15,46.250000015399,
45.9999999733281));
#18579=CARTESIAN_POINT('Ctrl Pts',(-12.3256628446849,46.0416666820657,45.9999999733281));
#18580=CARTESIAN_POINT('Ctrl Pts',(-22.999999986664,45.8333333487323,39.8371685509857));
#18581=CARTESIAN_POINT('Ctrl Pts',(-33.6743371286432,45.625000015399,33.6743371286432));
#18582=CARTESIAN_POINT('Ctrl Pts',(-39.8371685509856,45.4166666820657,22.9999999866641));
#18583=CARTESIAN_POINT('Ctrl Pts',(-45.9999999733281,45.2083333487323,12.325662844685));
#18584=CARTESIAN_POINT('Ctrl Pts',(-45.9999999733281,45.000000015399,1.86248708600067E-22));
#18585=CARTESIAN_POINT('Ctrl Pts',(-45.9999999733281,44.7916666820657,-12.3256628446849));
#18586=CARTESIAN_POINT('Ctrl Pts',(-39.8371685509857,44.5833333487323,-22.9999999866641));
#18587=CARTESIAN_POINT('Ctrl Pts',(-33.6743371286432,44.375000015399,-33.6743371286432));
#18588=CARTESIAN_POINT('Ctrl Pts',(-22.9999999866641,44.1666666820657,-39.8371685509857));
#18589=CARTESIAN_POINT('Ctrl Pts',(-12.3256628446849,43.9583333487323,-45.9999999733281));
#18590=CARTESIAN_POINT('Ctrl Pts',(-2.81668782265444E-15,43.750000015399,
-45.9999999733281));
#18591=CARTESIAN_POINT('Ctrl Pts',(12.3256628446849,43.5416666820657,-45.9999999733281));
#18592=CARTESIAN_POINT('Ctrl Pts',(22.9999999866641,43.3333333487324,-39.8371685509857));
#18593=CARTESIAN_POINT('Ctrl Pts',(33.6743371286432,43.125000015399,-33.6743371286432));
#18594=CARTESIAN_POINT('Ctrl Pts',(39.8371685509856,42.9166666820657,-22.9999999866641));
#18595=CARTESIAN_POINT('Ctrl Pts',(45.9999999733281,42.7083333487324,-12.3256628446849));
#18596=CARTESIAN_POINT('Ctrl Pts',(45.9999999733281,42.500000015399,-5.63337545906017E-15));
#18597=CARTESIAN_POINT('Ctrl Pts',(45.9999999733281,42.2916666820657,12.3256628446849));
#18598=CARTESIAN_POINT('Ctrl Pts',(39.8371685509857,42.0833333487324,22.999999986664));
#18599=CARTESIAN_POINT('Ctrl Pts',(33.6743371286432,41.875000015399,33.6743371286432));
#18600=CARTESIAN_POINT('Ctrl Pts',(22.9999999866641,41.6666666820657,39.8371685509856));
#18601=CARTESIAN_POINT('Ctrl Pts',(12.325662844685,41.4583333487323,45.9999999733281));
#18602=CARTESIAN_POINT('Ctrl Pts',(8.4500630954659E-15,41.250000015399,
45.9999999733281));
#18603=CARTESIAN_POINT('Ctrl Pts',(-12.3256628446849,41.0416666820657,45.9999999733281));
#18604=CARTESIAN_POINT('Ctrl Pts',(-22.999999986664,40.8333333487324,39.8371685509857));
#18605=CARTESIAN_POINT('Ctrl Pts',(-33.6743371286432,40.625000015399,33.6743371286432));
#18606=CARTESIAN_POINT('Ctrl Pts',(-39.8371685509856,40.4166666820657,22.9999999866641));
#18607=CARTESIAN_POINT('Ctrl Pts',(-45.9999999733281,40.2083333487324,12.325662844685));
#18608=CARTESIAN_POINT('Ctrl Pts',(-45.9999999733281,40.000000015399,1.86248708600067E-22));
#18609=CARTESIAN_POINT('Ctrl Pts',(-45.9999999733281,39.7916666820657,-12.3256628446849));
#18610=CARTESIAN_POINT('Ctrl Pts',(-39.8371685509857,39.5833333487323,-22.9999999866641));
#18611=CARTESIAN_POINT('Ctrl Pts',(-33.6743371286432,39.375000015399,-33.6743371286432));
#18612=CARTESIAN_POINT('Ctrl Pts',(-22.9999999866641,39.1666666820657,-39.8371685509857));
#18613=CARTESIAN_POINT('Ctrl Pts',(-12.3256628446849,38.9583333487323,-45.9999999733281));
#18614=CARTESIAN_POINT('Ctrl Pts',(-2.81668782265444E-15,38.750000015399,
-45.9999999733281));
#18615=CARTESIAN_POINT('Ctrl Pts',(12.3256628446849,38.5416666820657,-45.9999999733281));
#18616=CARTESIAN_POINT('Ctrl Pts',(22.9999999866641,38.3333333487323,-39.8371685509857));
#18617=CARTESIAN_POINT('Ctrl Pts',(33.6743371286432,38.125000015399,-33.6743371286432));
#18618=CARTESIAN_POINT('Ctrl Pts',(39.8371685509856,37.9166666820657,-22.9999999866641));
#18619=CARTESIAN_POINT('Ctrl Pts',(45.9999999733281,37.7083333487323,-12.3256628446849));
#18620=CARTESIAN_POINT('Ctrl Pts',(45.9999999733281,37.500000015399,-5.63337545906017E-15));
#18621=CARTESIAN_POINT('Ctrl Pts',(45.9999999733281,37.2916666820657,12.3256628446849));
#18622=CARTESIAN_POINT('Ctrl Pts',(39.8371685509857,37.0833333487323,22.999999986664));
#18623=CARTESIAN_POINT('Ctrl Pts',(33.6743371286432,36.875000015399,33.6743371286432));
#18624=CARTESIAN_POINT('Ctrl Pts',(22.9999999866641,36.6666666820657,39.8371685509856));
#18625=CARTESIAN_POINT('Ctrl Pts',(12.325662844685,36.4583333487323,45.9999999733281));
#18626=CARTESIAN_POINT('Ctrl Pts',(8.4500630954659E-15,36.250000015399,
45.9999999733281));
#18627=CARTESIAN_POINT('Ctrl Pts',(-12.3256628446849,36.0416666820657,45.9999999733281));
#18628=CARTESIAN_POINT('Ctrl Pts',(-22.999999986664,35.8333333487323,39.8371685509857));
#18629=CARTESIAN_POINT('Ctrl Pts',(-33.6743371286432,35.625000015399,33.6743371286432));
#18630=CARTESIAN_POINT('Ctrl Pts',(-39.8371685509856,35.4166666820657,22.9999999866641));
#18631=CARTESIAN_POINT('Ctrl Pts',(-45.9999999733281,35.2083333487323,12.325662844685));
#18632=CARTESIAN_POINT('Ctrl Pts',(-45.9999999733281,35.000000015399,1.86248708600067E-22));
#18633=CARTESIAN_POINT('Ctrl Pts',(-45.9999999733281,34.7916666820657,-12.3256628446849));
#18634=CARTESIAN_POINT('Ctrl Pts',(-39.8371685509857,34.5833333487323,-22.9999999866641));
#18635=CARTESIAN_POINT('Ctrl Pts',(-33.6743371286432,34.375000015399,-33.6743371286432));
#18636=CARTESIAN_POINT('Ctrl Pts',(-22.9999999866641,34.1666666820657,-39.8371685509857));
#18637=CARTESIAN_POINT('Ctrl Pts',(-12.3256628446849,33.9583333487323,-45.9999999733281));
#18638=CARTESIAN_POINT('Ctrl Pts',(-2.81668782265444E-15,33.750000015399,
-45.9999999733281));
#18639=CARTESIAN_POINT('Ctrl Pts',(12.3256628446849,33.5416666820657,-45.9999999733281));
#18640=CARTESIAN_POINT('Ctrl Pts',(22.9999999866641,33.3333333487323,-39.8371685509857));
#18641=CARTESIAN_POINT('Ctrl Pts',(33.6743371286432,33.125000015399,-33.6743371286432));
#18642=CARTESIAN_POINT('Ctrl Pts',(39.8371685509856,32.9166666820657,-22.9999999866641));
#18643=CARTESIAN_POINT('Ctrl Pts',(45.9999999733281,32.7083333487323,-12.3256628446849));
#18644=CARTESIAN_POINT('Ctrl Pts',(45.9999999733281,32.500000015399,-5.63337545906017E-15));
#18645=CARTESIAN_POINT('Ctrl Pts',(45.9999999733281,32.2916666820657,12.3256628446849));
#18646=CARTESIAN_POINT('Ctrl Pts',(39.8371685509857,32.0833333487323,22.999999986664));
#18647=CARTESIAN_POINT('Ctrl Pts',(33.6743371286432,31.875000015399,33.6743371286432));
#18648=CARTESIAN_POINT('Ctrl Pts',(22.9999999866641,31.6666666820657,39.8371685509856));
#18649=CARTESIAN_POINT('Ctrl Pts',(12.325662844685,31.4583333487323,45.9999999733281));
#18650=CARTESIAN_POINT('Ctrl Pts',(8.4500630954659E-15,31.250000015399,
45.9999999733281));
#18651=CARTESIAN_POINT('Ctrl Pts',(-12.3256628446849,31.0416666820657,45.9999999733281));
#18652=CARTESIAN_POINT('Ctrl Pts',(-22.999999986664,30.8333333487323,39.8371685509857));
#18653=CARTESIAN_POINT('Ctrl Pts',(-33.6743371286432,30.625000015399,33.6743371286432));
#18654=CARTESIAN_POINT('Ctrl Pts',(-39.8371685509856,30.4166666820657,22.9999999866641));
#18655=CARTESIAN_POINT('Ctrl Pts',(-45.9999999733281,30.2083333487323,12.325662844685));
#18656=CARTESIAN_POINT('Ctrl Pts',(-45.9999999733281,30.000000015399,1.86248708600067E-22));
#18657=CARTESIAN_POINT('Ctrl Pts',(45.7957082162897,32.5741208584476,-4.33048599679664));
#18658=CARTESIAN_POINT('Ctrl Pts',(46.027322302781,32.4406160752063,-4.33048599679664));
#18659=CARTESIAN_POINT('Ctrl Pts',(46.4905476657728,32.1736016336912,-4.33048599679679));
#18660=CARTESIAN_POINT('Ctrl Pts',(46.9537676533565,31.9065778670208,-4.33048599679665));
#18661=CARTESIAN_POINT('Ctrl Pts',(47.6280672732222,31.5178683162597,-4.33048599679665));
#18662=CARTESIAN_POINT('Ctrl Pts',(48.0707534890442,31.2626647328764,-4.33048599679682));
#18663=CARTESIAN_POINT('Ctrl Pts',(48.5134353784344,31.0074536451604,-4.33048599679682));
#18664=CARTESIAN_POINT('Origin',(4513.80899750787,-7920.15854999024,-4.33048586364984));
#18665=CARTESIAN_POINT('Ctrl Pts',(-2.77456427460704,33.7972761197826,-45.9162475937012));
#18666=CARTESIAN_POINT('Ctrl Pts',(-2.63312591332868,33.6885519019789,-46.1089077818654));
#18667=CARTESIAN_POINT('Ctrl Pts',(-2.47630178223139,33.5831756620264,-46.2955459160921));
#18668=CARTESIAN_POINT('Ctrl Pts',(-2.09992691815342,33.371173761156,-46.6702834188207));
#18669=CARTESIAN_POINT('Ctrl Pts',(-1.86960700461488,33.2651451031817,-46.8571879502895));
#18670=CARTESIAN_POINT('Ctrl Pts',(-1.44126400733626,33.1220740404168,-47.1072221114464));
#18671=CARTESIAN_POINT('Ctrl Pts',(-1.25731789418526,33.0737193247225,-47.1910001179499));
#18672=CARTESIAN_POINT('Ctrl Pts',(-0.930990574714349,33.0146873105689,
-47.291192418918));
#18673=CARTESIAN_POINT('Ctrl Pts',(-0.79608853305349,32.9971216590757,-47.3202305438409));
#18674=CARTESIAN_POINT('Ctrl Pts',(-0.593494556430455,32.9816476890939,
-47.3440578144643));
#18675=CARTESIAN_POINT('Ctrl Pts',(-0.528604008161592,32.9782810542056,
-47.3488063321149));
#18676=CARTESIAN_POINT('Ctrl Pts',(-0.455514956847433,32.9762981123005,
-47.3508718861098));
#18677=CARTESIAN_POINT('Ctrl Pts',(-0.447577390437119,32.9761065917277,
-47.3510529648804));
#18678=CARTESIAN_POINT('Ctrl Pts',(-0.43531402020566,32.9758475255699,-47.3512658915012));
#18679=CARTESIAN_POINT('Ctrl Pts',(-0.430989393289628,32.9757632392308,
-47.3513281446522));
#18680=CARTESIAN_POINT('Ctrl Pts',(-0.425732734692202,32.9756693851213,
-47.3513882117866));
#18681=CARTESIAN_POINT('Ctrl Pts',(-0.424801004760669,32.9756530779659,
-47.3513982628154));
#18682=CARTESIAN_POINT('Ctrl Pts',(-0.423270430619263,32.9756268290707,
-47.3514137952413));
#18683=CARTESIAN_POINT('Ctrl Pts',(-0.42267159374665,32.9756166947886,-47.3514196262221));
#18684=CARTESIAN_POINT('Ctrl Pts',(-0.421601003469021,32.9755988193071,
-47.3514296108102));
#18685=CARTESIAN_POINT('Ctrl Pts',(-0.421129251994336,32.9755910266925,
-47.3514338577676));
#18686=CARTESIAN_POINT('Ctrl Pts',(-0.420123704778293,32.9755745959494,
-47.3514425847247));
#18687=CARTESIAN_POINT('Ctrl Pts',(-0.419589908379852,32.9755659813974,
-47.3514470219234));
#18688=CARTESIAN_POINT('Ctrl Pts',(-0.418167541624201,32.9755433139297,
-47.3514583243956));
#18689=CARTESIAN_POINT('Ctrl Pts',(-0.417278965930535,32.9755294517199,
-47.351464843457));
#18690=CARTESIAN_POINT('Ctrl Pts',(-0.4131415843562,32.9754662965793,-47.3514926748277));
#18691=CARTESIAN_POINT('Ctrl Pts',(-0.409892694872467,32.9754206944094,
-47.3515072872273));
#18692=CARTESIAN_POINT('Ctrl Pts',(-0.386060814153076,32.9751154571127,
-47.3515613489623));
#18693=CARTESIAN_POINT('Ctrl Pts',(-0.365479633441874,32.9750120157055,
-47.3513173638308));
#18694=CARTESIAN_POINT('Ctrl Pts',(-0.26272690047942,32.9752945949283,-47.3486490070669));
#18695=CARTESIAN_POINT('Ctrl Pts',(-0.180951746939931,32.9780716383461,
-47.3418930110935));
#18696=CARTESIAN_POINT('Ctrl Pts',(0.0529660757825567,32.9931992298982,
-47.309526490652));
#18697=CARTESIAN_POINT('Ctrl Pts',(0.201533978643987,33.0116665859949,-47.2728828889392));
#18698=CARTESIAN_POINT('Ctrl Pts',(0.553021373295282,33.0747615694622,-47.1509572093954));
#18699=CARTESIAN_POINT('Ctrl Pts',(0.747612808578448,33.1267664634886,-47.0524625034721));
#18700=CARTESIAN_POINT('Ctrl Pts',(1.29390814642398,33.3135276394169,-46.7021675926803));
#18701=CARTESIAN_POINT('Ctrl Pts',(1.63924643152126,33.4911286721254,-46.3728987766334));
#18702=CARTESIAN_POINT('Ctrl Pts',(1.95443836226863,33.716777165276,-45.958461361191));
#18703=CARTESIAN_POINT('Ctrl Pts',(-48.706329375,58.437500006828,-1.8898197019151E-14));
#18704=CARTESIAN_POINT('Ctrl Pts',(-48.706329375,58.2291666734946,-13.0508216223155));
#18705=CARTESIAN_POINT('Ctrl Pts',(-42.1809185638422,58.0208333401613,-24.3531646875));
#18706=CARTESIAN_POINT('Ctrl Pts',(-35.6555077526845,57.812500006828,-35.6555077526845));
#18707=CARTESIAN_POINT('Ctrl Pts',(-24.3531646875,57.6041666734946,-42.1809185638422));
#18708=CARTESIAN_POINT('Ctrl Pts',(-13.0508216223155,57.3958333401613,-48.706329375));
#18709=CARTESIAN_POINT('Ctrl Pts',(1.59157945007855E-14,57.187500006828,
-48.706329375));
#18710=CARTESIAN_POINT('Ctrl Pts',(13.0508216223155,56.9791666734946,-48.706329375));
#18711=CARTESIAN_POINT('Ctrl Pts',(24.3531646875,56.7708333401613,-42.1809185638422));
#18712=CARTESIAN_POINT('Ctrl Pts',(35.6555077526845,56.562500006828,-35.6555077526845));
#18713=CARTESIAN_POINT('Ctrl Pts',(42.1809185638422,56.3541666734946,-24.3531646875));
#18714=CARTESIAN_POINT('Ctrl Pts',(48.706329375,56.1458333401613,-13.0508216223155));
#18715=CARTESIAN_POINT('Ctrl Pts',(48.706329375,55.937500006828,1.293339198242E-14));
#18716=CARTESIAN_POINT('Ctrl Pts',(48.706329375,55.7291666734946,13.0508216223155));
#18717=CARTESIAN_POINT('Ctrl Pts',(42.1809185638422,55.5208333401613,24.3531646875));
#18718=CARTESIAN_POINT('Ctrl Pts',(35.6555077526845,55.312500006828,35.6555077526845));
#18719=CARTESIAN_POINT('Ctrl Pts',(24.3531646875,55.1041666734946,42.1809185638422));
#18720=CARTESIAN_POINT('Ctrl Pts',(13.0508216223155,54.8958333401613,48.706329375));
#18721=CARTESIAN_POINT('Ctrl Pts',(-9.95098946405443E-15,54.687500006828,
48.706329375));
#18722=CARTESIAN_POINT('Ctrl Pts',(-13.0508216223155,54.4791666734946,48.706329375));
#18723=CARTESIAN_POINT('Ctrl Pts',(-24.3531646875,54.2708333401613,42.1809185638423));
#18724=CARTESIAN_POINT('Ctrl Pts',(-35.6555077526845,54.062500006828,35.6555077526845));
#18725=CARTESIAN_POINT('Ctrl Pts',(-42.1809185638422,53.8541666734946,24.3531646875));
#18726=CARTESIAN_POINT('Ctrl Pts',(-48.706329375,53.6458333401613,13.0508216223155));
#18727=CARTESIAN_POINT('Ctrl Pts',(-48.706329375,53.437500006828,-1.8898197019151E-14));
#18728=CARTESIAN_POINT('Ctrl Pts',(-48.706329375,53.2291666734946,-13.0508216223155));
#18729=CARTESIAN_POINT('Ctrl Pts',(-42.1809185638422,53.0208333401613,-24.3531646875));
#18730=CARTESIAN_POINT('Ctrl Pts',(-35.6555077526845,52.812500006828,-35.6555077526845));
#18731=CARTESIAN_POINT('Ctrl Pts',(-24.3531646875,52.6041666734946,-42.1809185638422));
#18732=CARTESIAN_POINT('Ctrl Pts',(-13.0508216223155,52.3958333401613,-48.706329375));
#18733=CARTESIAN_POINT('Ctrl Pts',(1.59157945007855E-14,52.187500006828,
-48.706329375));
#18734=CARTESIAN_POINT('Ctrl Pts',(13.0508216223155,51.9791666734946,-48.706329375));
#18735=CARTESIAN_POINT('Ctrl Pts',(24.3531646875,51.7708333401613,-42.1809185638422));
#18736=CARTESIAN_POINT('Ctrl Pts',(35.6555077526845,51.562500006828,-35.6555077526845));
#18737=CARTESIAN_POINT('Ctrl Pts',(42.1809185638422,51.3541666734946,-24.3531646875));
#18738=CARTESIAN_POINT('Ctrl Pts',(48.706329375,51.1458333401613,-13.0508216223155));
#18739=CARTESIAN_POINT('Ctrl Pts',(48.706329375,50.937500006828,1.293339198242E-14));
#18740=CARTESIAN_POINT('Ctrl Pts',(48.706329375,50.7291666734946,13.0508216223155));
#18741=CARTESIAN_POINT('Ctrl Pts',(42.1809185638422,50.5208333401613,24.3531646875));
#18742=CARTESIAN_POINT('Ctrl Pts',(35.6555077526845,50.312500006828,35.6555077526845));
#18743=CARTESIAN_POINT('Ctrl Pts',(24.3531646875,50.1041666734946,42.1809185638422));
#18744=CARTESIAN_POINT('Ctrl Pts',(13.0508216223155,49.8958333401613,48.706329375));
#18745=CARTESIAN_POINT('Ctrl Pts',(-9.95098946405443E-15,49.687500006828,
48.706329375));
#18746=CARTESIAN_POINT('Ctrl Pts',(-13.0508216223155,49.4791666734946,48.706329375));
#18747=CARTESIAN_POINT('Ctrl Pts',(-24.3531646875,49.2708333401613,42.1809185638423));
#18748=CARTESIAN_POINT('Ctrl Pts',(-35.6555077526845,49.062500006828,35.6555077526845));
#18749=CARTESIAN_POINT('Ctrl Pts',(-42.1809185638422,48.8541666734946,24.3531646875));
#18750=CARTESIAN_POINT('Ctrl Pts',(-48.706329375,48.6458333401613,13.0508216223155));
#18751=CARTESIAN_POINT('Ctrl Pts',(-48.706329375,48.437500006828,-1.8898197019151E-14));
#18752=CARTESIAN_POINT('Ctrl Pts',(-48.706329375,48.2291666734946,-13.0508216223155));
#18753=CARTESIAN_POINT('Ctrl Pts',(-42.1809185638422,48.0208333401613,-24.3531646875));
#18754=CARTESIAN_POINT('Ctrl Pts',(-35.6555077526845,47.812500006828,-35.6555077526845));
#18755=CARTESIAN_POINT('Ctrl Pts',(-24.3531646875,47.6041666734946,-42.1809185638422));
#18756=CARTESIAN_POINT('Ctrl Pts',(-13.0508216223155,47.3958333401613,-48.706329375));
#18757=CARTESIAN_POINT('Ctrl Pts',(1.59157945007855E-14,47.187500006828,
-48.706329375));
#18758=CARTESIAN_POINT('Ctrl Pts',(13.0508216223155,46.9791666734946,-48.706329375));
#18759=CARTESIAN_POINT('Ctrl Pts',(24.3531646875,46.7708333401613,-42.1809185638422));
#18760=CARTESIAN_POINT('Ctrl Pts',(35.6555077526845,46.562500006828,-35.6555077526845));
#18761=CARTESIAN_POINT('Ctrl Pts',(42.1809185638422,46.3541666734946,-24.3531646875));
#18762=CARTESIAN_POINT('Ctrl Pts',(48.706329375,46.1458333401613,-13.0508216223155));
#18763=CARTESIAN_POINT('Ctrl Pts',(48.706329375,45.937500006828,1.293339198242E-14));
#18764=CARTESIAN_POINT('Ctrl Pts',(48.706329375,45.7291666734946,13.0508216223155));
#18765=CARTESIAN_POINT('Ctrl Pts',(42.1809185638422,45.5208333401613,24.3531646875));
#18766=CARTESIAN_POINT('Ctrl Pts',(35.6555077526845,45.312500006828,35.6555077526845));
#18767=CARTESIAN_POINT('Ctrl Pts',(24.3531646875,45.1041666734946,42.1809185638422));
#18768=CARTESIAN_POINT('Ctrl Pts',(13.0508216223155,44.8958333401613,48.706329375));
#18769=CARTESIAN_POINT('Ctrl Pts',(-9.95098946405443E-15,44.687500006828,
48.706329375));
#18770=CARTESIAN_POINT('Ctrl Pts',(-13.0508216223155,44.4791666734946,48.706329375));
#18771=CARTESIAN_POINT('Ctrl Pts',(-24.3531646875,44.2708333401613,42.1809185638423));
#18772=CARTESIAN_POINT('Ctrl Pts',(-35.6555077526845,44.062500006828,35.6555077526845));
#18773=CARTESIAN_POINT('Ctrl Pts',(-42.1809185638422,43.8541666734946,24.3531646875));
#18774=CARTESIAN_POINT('Ctrl Pts',(-48.706329375,43.6458333401613,13.0508216223155));
#18775=CARTESIAN_POINT('Ctrl Pts',(-48.706329375,43.437500006828,-1.8898197019151E-14));
#18776=CARTESIAN_POINT('Ctrl Pts',(-48.706329375,43.2291666734946,-13.0508216223155));
#18777=CARTESIAN_POINT('Ctrl Pts',(-42.1809185638422,43.0208333401613,-24.3531646875));
#18778=CARTESIAN_POINT('Ctrl Pts',(-35.6555077526845,42.812500006828,-35.6555077526845));
#18779=CARTESIAN_POINT('Ctrl Pts',(-24.3531646875,42.6041666734946,-42.1809185638422));
#18780=CARTESIAN_POINT('Ctrl Pts',(-13.0508216223155,42.3958333401613,-48.706329375));
#18781=CARTESIAN_POINT('Ctrl Pts',(1.59157945007855E-14,42.187500006828,
-48.706329375));
#18782=CARTESIAN_POINT('Ctrl Pts',(13.0508216223155,41.9791666734946,-48.706329375));
#18783=CARTESIAN_POINT('Ctrl Pts',(24.3531646875,41.7708333401613,-42.1809185638422));
#18784=CARTESIAN_POINT('Ctrl Pts',(35.6555077526845,41.562500006828,-35.6555077526845));
#18785=CARTESIAN_POINT('Ctrl Pts',(42.1809185638422,41.3541666734946,-24.3531646875));
#18786=CARTESIAN_POINT('Ctrl Pts',(48.706329375,41.1458333401613,-13.0508216223155));
#18787=CARTESIAN_POINT('Ctrl Pts',(48.706329375,40.937500006828,1.293339198242E-14));
#18788=CARTESIAN_POINT('Ctrl Pts',(48.706329375,40.7291666734946,13.0508216223155));
#18789=CARTESIAN_POINT('Ctrl Pts',(42.1809185638422,40.5208333401613,24.3531646875));
#18790=CARTESIAN_POINT('Ctrl Pts',(35.6555077526845,40.312500006828,35.6555077526845));
#18791=CARTESIAN_POINT('Ctrl Pts',(24.3531646875,40.1041666734946,42.1809185638422));
#18792=CARTESIAN_POINT('Ctrl Pts',(13.0508216223155,39.8958333401613,48.706329375));
#18793=CARTESIAN_POINT('Ctrl Pts',(-9.95098946405443E-15,39.687500006828,
48.706329375));
#18794=CARTESIAN_POINT('Ctrl Pts',(-13.0508216223155,39.4791666734946,48.706329375));
#18795=CARTESIAN_POINT('Ctrl Pts',(-24.3531646875,39.2708333401613,42.1809185638423));
#18796=CARTESIAN_POINT('Ctrl Pts',(-35.6555077526845,39.062500006828,35.6555077526845));
#18797=CARTESIAN_POINT('Ctrl Pts',(-42.1809185638422,38.8541666734946,24.3531646875));
#18798=CARTESIAN_POINT('Ctrl Pts',(-48.706329375,38.6458333401613,13.0508216223155));
#18799=CARTESIAN_POINT('Ctrl Pts',(-48.706329375,38.437500006828,-1.8898197019151E-14));
#18800=CARTESIAN_POINT('Ctrl Pts',(-48.706329375,38.2291666734946,-13.0508216223155));
#18801=CARTESIAN_POINT('Ctrl Pts',(-42.1809185638422,38.0208333401613,-24.3531646875));
#18802=CARTESIAN_POINT('Ctrl Pts',(-35.6555077526845,37.812500006828,-35.6555077526845));
#18803=CARTESIAN_POINT('Ctrl Pts',(-24.3531646875,37.6041666734946,-42.1809185638422));
#18804=CARTESIAN_POINT('Ctrl Pts',(-13.0508216223155,37.3958333401613,-48.706329375));
#18805=CARTESIAN_POINT('Ctrl Pts',(1.59157945007855E-14,37.187500006828,
-48.706329375));
#18806=CARTESIAN_POINT('Ctrl Pts',(13.0508216223155,36.9791666734946,-48.706329375));
#18807=CARTESIAN_POINT('Ctrl Pts',(24.3531646875,36.7708333401613,-42.1809185638422));
#18808=CARTESIAN_POINT('Ctrl Pts',(35.6555077526845,36.562500006828,-35.6555077526845));
#18809=CARTESIAN_POINT('Ctrl Pts',(42.1809185638422,36.3541666734946,-24.3531646875));
#18810=CARTESIAN_POINT('Ctrl Pts',(48.706329375,36.1458333401613,-13.0508216223155));
#18811=CARTESIAN_POINT('Ctrl Pts',(48.706329375,35.937500006828,1.293339198242E-14));
#18812=CARTESIAN_POINT('Ctrl Pts',(48.706329375,35.7291666734946,13.0508216223155));
#18813=CARTESIAN_POINT('Ctrl Pts',(42.1809185638422,35.5208333401613,24.3531646875));
#18814=CARTESIAN_POINT('Ctrl Pts',(35.6555077526845,35.312500006828,35.6555077526845));
#18815=CARTESIAN_POINT('Ctrl Pts',(24.3531646875,35.1041666734946,42.1809185638422));
#18816=CARTESIAN_POINT('Ctrl Pts',(13.0508216223155,34.8958333401613,48.706329375));
#18817=CARTESIAN_POINT('Ctrl Pts',(-9.95098946405443E-15,34.687500006828,
48.706329375));
#18818=CARTESIAN_POINT('Ctrl Pts',(-13.0508216223155,34.4791666734946,48.706329375));
#18819=CARTESIAN_POINT('Ctrl Pts',(-24.3531646875,34.2708333401613,42.1809185638423));
#18820=CARTESIAN_POINT('Ctrl Pts',(-35.6555077526845,34.062500006828,35.6555077526845));
#18821=CARTESIAN_POINT('Ctrl Pts',(-42.1809185638422,33.8541666734946,24.3531646875));
#18822=CARTESIAN_POINT('Ctrl Pts',(-48.706329375,33.6458333401613,13.0508216223155));
#18823=CARTESIAN_POINT('Ctrl Pts',(-48.706329375,33.437500006828,-1.8898197019151E-14));
#18824=CARTESIAN_POINT('Ctrl Pts',(-48.706329375,33.2291666734946,-13.0508216223155));
#18825=CARTESIAN_POINT('Ctrl Pts',(-42.1809185638422,33.0208333401613,-24.3531646875));
#18826=CARTESIAN_POINT('Ctrl Pts',(-35.6555077526845,32.812500006828,-35.6555077526845));
#18827=CARTESIAN_POINT('Ctrl Pts',(-24.3531646875,32.6041666734946,-42.1809185638422));
#18828=CARTESIAN_POINT('Ctrl Pts',(-13.0508216223155,32.3958333401613,-48.706329375));
#18829=CARTESIAN_POINT('Ctrl Pts',(1.59157945007855E-14,32.187500006828,
-48.706329375));
#18830=CARTESIAN_POINT('Ctrl Pts',(13.0508216223155,31.9791666734946,-48.706329375));
#18831=CARTESIAN_POINT('Ctrl Pts',(24.3531646875,31.7708333401613,-42.1809185638422));
#18832=CARTESIAN_POINT('Ctrl Pts',(35.6555077526845,31.562500006828,-35.6555077526845));
#18833=CARTESIAN_POINT('Ctrl Pts',(42.1809185638422,31.3541666734946,-24.3531646875));
#18834=CARTESIAN_POINT('Ctrl Pts',(48.706329375,31.1458333401613,-13.0508216223155));
#18835=CARTESIAN_POINT('Ctrl Pts',(48.706329375,30.937500006828,1.293339198242E-14));
#18836=CARTESIAN_POINT('Ctrl Pts',(48.706329375,30.7291666734946,13.0508216223155));
#18837=CARTESIAN_POINT('Ctrl Pts',(42.1809185638422,30.5208333401613,24.3531646875));
#18838=CARTESIAN_POINT('Ctrl Pts',(35.6555077526845,30.312500006828,35.6555077526845));
#18839=CARTESIAN_POINT('Ctrl Pts',(24.3531646875,30.1041666734946,42.1809185638422));
#18840=CARTESIAN_POINT('Ctrl Pts',(13.0508216223155,29.8958333401613,48.706329375));
#18841=CARTESIAN_POINT('Ctrl Pts',(-9.95098946405443E-15,29.687500006828,
48.706329375));
#18842=CARTESIAN_POINT('Ctrl Pts',(-13.0508216223155,29.4791666734946,48.706329375));
#18843=CARTESIAN_POINT('Ctrl Pts',(-24.3531646875,29.2708333401613,42.1809185638423));
#18844=CARTESIAN_POINT('Ctrl Pts',(-35.6555077526845,29.062500006828,35.6555077526845));
#18845=CARTESIAN_POINT('Ctrl Pts',(-42.1809185638422,28.8541666734946,24.3531646875));
#18846=CARTESIAN_POINT('Ctrl Pts',(-48.706329375,28.6458333401613,13.0508216223155));
#18847=CARTESIAN_POINT('Ctrl Pts',(-48.706329375,28.437500006828,-1.8898197019151E-14));
#18848=CARTESIAN_POINT('Ctrl Pts',(-46.,60.,0.));
#18849=CARTESIAN_POINT('Ctrl Pts',(-46.,59.7916666666667,-12.3256628518316));
#18850=CARTESIAN_POINT('Ctrl Pts',(-39.8371685740842,59.5833333333333,-23.));
#18851=CARTESIAN_POINT('Ctrl Pts',(-33.6743371481684,59.375,-33.6743371481684));
#18852=CARTESIAN_POINT('Ctrl Pts',(-23.,59.1666666666667,-39.8371685740842));
#18853=CARTESIAN_POINT('Ctrl Pts',(-12.3256628518317,58.9583333333333,-46.));
#18854=CARTESIAN_POINT('Ctrl Pts',(-2.81668763803891E-15,58.75,-46.));
#18855=CARTESIAN_POINT('Ctrl Pts',(12.3256628518316,58.5416666666667,-46.));
#18856=CARTESIAN_POINT('Ctrl Pts',(23.,58.3333333333333,-39.8371685740842));
#18857=CARTESIAN_POINT('Ctrl Pts',(33.6743371481683,58.125,-33.6743371481684));
#18858=CARTESIAN_POINT('Ctrl Pts',(39.8371685740842,57.9166666666667,-23.));
#18859=CARTESIAN_POINT('Ctrl Pts',(46.,57.7083333333333,-12.3256628518317));
#18860=CARTESIAN_POINT('Ctrl Pts',(46.,57.5,-5.63337527607782E-15));
#18861=CARTESIAN_POINT('Ctrl Pts',(46.,57.2916666666667,12.3256628518316));
#18862=CARTESIAN_POINT('Ctrl Pts',(39.8371685740842,57.0833333333333,23.));
#18863=CARTESIAN_POINT('Ctrl Pts',(33.6743371481684,56.875,33.6743371481683));
#18864=CARTESIAN_POINT('Ctrl Pts',(23.,56.6666666666667,39.8371685740842));
#18865=CARTESIAN_POINT('Ctrl Pts',(12.3256628518317,56.4583333333333,46.));
#18866=CARTESIAN_POINT('Ctrl Pts',(8.45006291411674E-15,56.25,46.));
#18867=CARTESIAN_POINT('Ctrl Pts',(-12.3256628518316,56.0416666666667,46.));
#18868=CARTESIAN_POINT('Ctrl Pts',(-23.,55.8333333333333,39.8371685740842));
#18869=CARTESIAN_POINT('Ctrl Pts',(-33.6743371481683,55.625,33.6743371481684));
#18870=CARTESIAN_POINT('Ctrl Pts',(-39.8371685740842,55.4166666666667,23.));
#18871=CARTESIAN_POINT('Ctrl Pts',(-46.,55.2083333333333,12.3256628518317));
#18872=CARTESIAN_POINT('Ctrl Pts',(-46.,55.,0.));
#18873=CARTESIAN_POINT('Ctrl Pts',(-46.,54.7916666666667,-12.3256628518316));
#18874=CARTESIAN_POINT('Ctrl Pts',(-39.8371685740842,54.5833333333333,-23.));
#18875=CARTESIAN_POINT('Ctrl Pts',(-33.6743371481684,54.375,-33.6743371481684));
#18876=CARTESIAN_POINT('Ctrl Pts',(-23.,54.1666666666667,-39.8371685740842));
#18877=CARTESIAN_POINT('Ctrl Pts',(-12.3256628518317,53.9583333333333,-46.));
#18878=CARTESIAN_POINT('Ctrl Pts',(-2.81668763803891E-15,53.75,-46.));
#18879=CARTESIAN_POINT('Ctrl Pts',(12.3256628518316,53.5416666666667,-46.));
#18880=CARTESIAN_POINT('Ctrl Pts',(23.,53.3333333333333,-39.8371685740842));
#18881=CARTESIAN_POINT('Ctrl Pts',(33.6743371481683,53.125,-33.6743371481684));
#18882=CARTESIAN_POINT('Ctrl Pts',(39.8371685740842,52.9166666666667,-23.));
#18883=CARTESIAN_POINT('Ctrl Pts',(46.,52.7083333333333,-12.3256628518317));
#18884=CARTESIAN_POINT('Ctrl Pts',(46.,52.5,-5.63337527607782E-15));
#18885=CARTESIAN_POINT('Ctrl Pts',(46.,52.2916666666667,12.3256628518316));
#18886=CARTESIAN_POINT('Ctrl Pts',(39.8371685740842,52.0833333333333,23.));
#18887=CARTESIAN_POINT('Ctrl Pts',(33.6743371481684,51.875,33.6743371481683));
#18888=CARTESIAN_POINT('Ctrl Pts',(23.,51.6666666666667,39.8371685740842));
#18889=CARTESIAN_POINT('Ctrl Pts',(12.3256628518317,51.4583333333333,46.));
#18890=CARTESIAN_POINT('Ctrl Pts',(8.45006291411674E-15,51.25,46.));
#18891=CARTESIAN_POINT('Ctrl Pts',(-12.3256628518316,51.0416666666667,46.));
#18892=CARTESIAN_POINT('Ctrl Pts',(-23.,50.8333333333333,39.8371685740842));
#18893=CARTESIAN_POINT('Ctrl Pts',(-33.6743371481683,50.625,33.6743371481684));
#18894=CARTESIAN_POINT('Ctrl Pts',(-39.8371685740842,50.4166666666667,23.));
#18895=CARTESIAN_POINT('Ctrl Pts',(-46.,50.2083333333333,12.3256628518317));
#18896=CARTESIAN_POINT('Ctrl Pts',(-46.,50.,0.));
#18897=CARTESIAN_POINT('Ctrl Pts',(-46.,49.7916666666667,-12.3256628518316));
#18898=CARTESIAN_POINT('Ctrl Pts',(-39.8371685740842,49.5833333333333,-23.));
#18899=CARTESIAN_POINT('Ctrl Pts',(-33.6743371481684,49.375,-33.6743371481684));
#18900=CARTESIAN_POINT('Ctrl Pts',(-23.,49.1666666666667,-39.8371685740842));
#18901=CARTESIAN_POINT('Ctrl Pts',(-12.3256628518317,48.9583333333333,-46.));
#18902=CARTESIAN_POINT('Ctrl Pts',(-2.81668763803891E-15,48.75,-46.));
#18903=CARTESIAN_POINT('Ctrl Pts',(12.3256628518316,48.5416666666667,-46.));
#18904=CARTESIAN_POINT('Ctrl Pts',(23.,48.3333333333333,-39.8371685740842));
#18905=CARTESIAN_POINT('Ctrl Pts',(33.6743371481683,48.125,-33.6743371481684));
#18906=CARTESIAN_POINT('Ctrl Pts',(39.8371685740842,47.9166666666667,-23.));
#18907=CARTESIAN_POINT('Ctrl Pts',(46.,47.7083333333333,-12.3256628518317));
#18908=CARTESIAN_POINT('Ctrl Pts',(46.,47.5,-5.63337527607782E-15));
#18909=CARTESIAN_POINT('Ctrl Pts',(46.,47.2916666666667,12.3256628518316));
#18910=CARTESIAN_POINT('Ctrl Pts',(39.8371685740842,47.0833333333333,23.));
#18911=CARTESIAN_POINT('Ctrl Pts',(33.6743371481684,46.875,33.6743371481683));
#18912=CARTESIAN_POINT('Ctrl Pts',(23.,46.6666666666667,39.8371685740842));
#18913=CARTESIAN_POINT('Ctrl Pts',(12.3256628518317,46.4583333333333,46.));
#18914=CARTESIAN_POINT('Ctrl Pts',(8.45006291411674E-15,46.25,46.));
#18915=CARTESIAN_POINT('Ctrl Pts',(-12.3256628518316,46.0416666666667,46.));
#18916=CARTESIAN_POINT('Ctrl Pts',(-23.,45.8333333333333,39.8371685740842));
#18917=CARTESIAN_POINT('Ctrl Pts',(-33.6743371481683,45.625,33.6743371481684));
#18918=CARTESIAN_POINT('Ctrl Pts',(-39.8371685740842,45.4166666666667,23.));
#18919=CARTESIAN_POINT('Ctrl Pts',(-46.,45.2083333333333,12.3256628518317));
#18920=CARTESIAN_POINT('Ctrl Pts',(-46.,45.,0.));
#18921=CARTESIAN_POINT('Ctrl Pts',(-46.,44.7916666666667,-12.3256628518316));
#18922=CARTESIAN_POINT('Ctrl Pts',(-39.8371685740842,44.5833333333333,-23.));
#18923=CARTESIAN_POINT('Ctrl Pts',(-33.6743371481684,44.375,-33.6743371481684));
#18924=CARTESIAN_POINT('Ctrl Pts',(-23.,44.1666666666667,-39.8371685740842));
#18925=CARTESIAN_POINT('Ctrl Pts',(-12.3256628518317,43.9583333333333,-46.));
#18926=CARTESIAN_POINT('Ctrl Pts',(-2.81668763803891E-15,43.75,-46.));
#18927=CARTESIAN_POINT('Ctrl Pts',(12.3256628518316,43.5416666666667,-46.));
#18928=CARTESIAN_POINT('Ctrl Pts',(23.,43.3333333333333,-39.8371685740842));
#18929=CARTESIAN_POINT('Ctrl Pts',(33.6743371481683,43.125,-33.6743371481684));
#18930=CARTESIAN_POINT('Ctrl Pts',(39.8371685740842,42.9166666666667,-23.));
#18931=CARTESIAN_POINT('Ctrl Pts',(46.,42.7083333333333,-12.3256628518317));
#18932=CARTESIAN_POINT('Ctrl Pts',(46.,42.5,-5.63337527607782E-15));
#18933=CARTESIAN_POINT('Ctrl Pts',(46.,42.2916666666667,12.3256628518316));
#18934=CARTESIAN_POINT('Ctrl Pts',(39.8371685740842,42.0833333333333,23.));
#18935=CARTESIAN_POINT('Ctrl Pts',(33.6743371481684,41.875,33.6743371481683));
#18936=CARTESIAN_POINT('Ctrl Pts',(23.,41.6666666666667,39.8371685740842));
#18937=CARTESIAN_POINT('Ctrl Pts',(12.3256628518317,41.4583333333333,46.));
#18938=CARTESIAN_POINT('Ctrl Pts',(8.45006291411674E-15,41.25,46.));
#18939=CARTESIAN_POINT('Ctrl Pts',(-12.3256628518316,41.0416666666667,46.));
#18940=CARTESIAN_POINT('Ctrl Pts',(-23.,40.8333333333333,39.8371685740842));
#18941=CARTESIAN_POINT('Ctrl Pts',(-33.6743371481683,40.625,33.6743371481684));
#18942=CARTESIAN_POINT('Ctrl Pts',(-39.8371685740842,40.4166666666667,23.));
#18943=CARTESIAN_POINT('Ctrl Pts',(-46.,40.2083333333333,12.3256628518317));
#18944=CARTESIAN_POINT('Ctrl Pts',(-46.,40.,0.));
#18945=CARTESIAN_POINT('Ctrl Pts',(-46.,39.7916666666667,-12.3256628518316));
#18946=CARTESIAN_POINT('Ctrl Pts',(-39.8371685740842,39.5833333333333,-23.));
#18947=CARTESIAN_POINT('Ctrl Pts',(-33.6743371481684,39.375,-33.6743371481684));
#18948=CARTESIAN_POINT('Ctrl Pts',(-23.,39.1666666666667,-39.8371685740842));
#18949=CARTESIAN_POINT('Ctrl Pts',(-12.3256628518317,38.9583333333333,-46.));
#18950=CARTESIAN_POINT('Ctrl Pts',(-2.81668763803891E-15,38.75,-46.));
#18951=CARTESIAN_POINT('Ctrl Pts',(12.3256628518316,38.5416666666667,-46.));
#18952=CARTESIAN_POINT('Ctrl Pts',(23.,38.3333333333333,-39.8371685740842));
#18953=CARTESIAN_POINT('Ctrl Pts',(33.6743371481683,38.125,-33.6743371481684));
#18954=CARTESIAN_POINT('Ctrl Pts',(39.8371685740842,37.9166666666667,-23.));
#18955=CARTESIAN_POINT('Ctrl Pts',(46.,37.7083333333333,-12.3256628518317));
#18956=CARTESIAN_POINT('Ctrl Pts',(46.,37.5,-5.63337527607782E-15));
#18957=CARTESIAN_POINT('Ctrl Pts',(46.,37.2916666666667,12.3256628518316));
#18958=CARTESIAN_POINT('Ctrl Pts',(39.8371685740842,37.0833333333333,23.));
#18959=CARTESIAN_POINT('Ctrl Pts',(33.6743371481684,36.875,33.6743371481683));
#18960=CARTESIAN_POINT('Ctrl Pts',(23.,36.6666666666667,39.8371685740842));
#18961=CARTESIAN_POINT('Ctrl Pts',(12.3256628518317,36.4583333333333,46.));
#18962=CARTESIAN_POINT('Ctrl Pts',(8.45006291411674E-15,36.25,46.));
#18963=CARTESIAN_POINT('Ctrl Pts',(-12.3256628518316,36.0416666666667,46.));
#18964=CARTESIAN_POINT('Ctrl Pts',(-23.,35.8333333333333,39.8371685740842));
#18965=CARTESIAN_POINT('Ctrl Pts',(-33.6743371481683,35.625,33.6743371481684));
#18966=CARTESIAN_POINT('Ctrl Pts',(-39.8371685740842,35.4166666666667,23.));
#18967=CARTESIAN_POINT('Ctrl Pts',(-46.,35.2083333333333,12.3256628518317));
#18968=CARTESIAN_POINT('Ctrl Pts',(-46.,35.,0.));
#18969=CARTESIAN_POINT('Ctrl Pts',(-46.,34.7916666666667,-12.3256628518316));
#18970=CARTESIAN_POINT('Ctrl Pts',(-39.8371685740842,34.5833333333333,-23.));
#18971=CARTESIAN_POINT('Ctrl Pts',(-33.6743371481684,34.375,-33.6743371481684));
#18972=CARTESIAN_POINT('Ctrl Pts',(-23.,34.1666666666667,-39.8371685740842));
#18973=CARTESIAN_POINT('Ctrl Pts',(-12.3256628518317,33.9583333333333,-46.));
#18974=CARTESIAN_POINT('Ctrl Pts',(-2.81668763803891E-15,33.75,-46.));
#18975=CARTESIAN_POINT('Ctrl Pts',(12.3256628518316,33.5416666666667,-46.));
#18976=CARTESIAN_POINT('Ctrl Pts',(23.,33.3333333333333,-39.8371685740842));
#18977=CARTESIAN_POINT('Ctrl Pts',(33.6743371481683,33.125,-33.6743371481684));
#18978=CARTESIAN_POINT('Ctrl Pts',(39.8371685740842,32.9166666666667,-23.));
#18979=CARTESIAN_POINT('Ctrl Pts',(46.,32.7083333333333,-12.3256628518317));
#18980=CARTESIAN_POINT('Ctrl Pts',(46.,32.5,-5.63337527607782E-15));
#18981=CARTESIAN_POINT('Ctrl Pts',(46.,32.2916666666667,12.3256628518316));
#18982=CARTESIAN_POINT('Ctrl Pts',(39.8371685740842,32.0833333333333,23.));
#18983=CARTESIAN_POINT('Ctrl Pts',(33.6743371481684,31.875,33.6743371481683));
#18984=CARTESIAN_POINT('Ctrl Pts',(23.,31.6666666666667,39.8371685740842));
#18985=CARTESIAN_POINT('Ctrl Pts',(12.3256628518317,31.4583333333333,46.));
#18986=CARTESIAN_POINT('Ctrl Pts',(8.45006291411674E-15,31.25,46.));
#18987=CARTESIAN_POINT('Ctrl Pts',(-12.3256628518316,31.0416666666667,46.));
#18988=CARTESIAN_POINT('Ctrl Pts',(-23.,30.8333333333333,39.8371685740842));
#18989=CARTESIAN_POINT('Ctrl Pts',(-33.6743371481683,30.625,33.6743371481684));
#18990=CARTESIAN_POINT('Ctrl Pts',(-39.8371685740842,30.4166666666667,23.));
#18991=CARTESIAN_POINT('Ctrl Pts',(-46.,30.2083333333333,12.3256628518317));
#18992=CARTESIAN_POINT('Ctrl Pts',(-46.,30.,0.));
#18993=CARTESIAN_POINT('Ctrl Pts',(-45.858362923034,35.061608680256,3.60701400320325));
#18994=CARTESIAN_POINT('Ctrl Pts',(-46.089925771934,34.9280150456296,3.60701400320325));
#18995=CARTESIAN_POINT('Ctrl Pts',(-46.5530501979845,34.6608255719955,3.60701400320344));
#18996=CARTESIAN_POINT('Ctrl Pts',(-47.0161721905706,34.3936318804496,3.60701400320332));
#18997=CARTESIAN_POINT('Ctrl Pts',(-47.6893519862319,34.0052434879083,3.60701400320332));
#18998=CARTESIAN_POINT('Ctrl Pts',(-48.1309692507095,33.7504492807381,3.60701400320324));
#18999=CARTESIAN_POINT('Ctrl Pts',(-48.5725845633798,33.4956516907297,3.60701400320325));
#19000=CARTESIAN_POINT('Ctrl Pts',(-3.5801454378685,34.6297857346188,48.5745723586909));
#19001=CARTESIAN_POINT('Ctrl Pts',(-3.75675791161119,34.8758757672123,48.1282675842178));
#19002=CARTESIAN_POINT('Ctrl Pts',(-3.89802648524866,35.1321260590805,47.6664043022228));
#19003=CARTESIAN_POINT('Ctrl Pts',(-4.11753371733878,35.6479820980819,46.7424335165373));
#19004=CARTESIAN_POINT('Ctrl Pts',(-4.19766087013856,35.9122067971139,46.2720484535312));
#19005=CARTESIAN_POINT('Ctrl Pts',(-4.24983907177926,36.1772764823076,45.8032626333974));
#19006=CARTESIAN_POINT('Ctrl Pts',(-48.706329375,58.437500006828,-1.8898197019151E-14));
#19007=CARTESIAN_POINT('Ctrl Pts',(-48.706329375,58.2291666734946,-13.0508216223155));
#19008=CARTESIAN_POINT('Ctrl Pts',(-42.1809185638422,58.0208333401613,-24.3531646875));
#19009=CARTESIAN_POINT('Ctrl Pts',(-35.6555077526845,57.812500006828,-35.6555077526845));
#19010=CARTESIAN_POINT('Ctrl Pts',(-24.3531646875,57.6041666734946,-42.1809185638422));
#19011=CARTESIAN_POINT('Ctrl Pts',(-13.0508216223155,57.3958333401613,-48.706329375));
#19012=CARTESIAN_POINT('Ctrl Pts',(1.59157945007855E-14,57.187500006828,
-48.706329375));
#19013=CARTESIAN_POINT('Ctrl Pts',(13.0508216223155,56.9791666734946,-48.706329375));
#19014=CARTESIAN_POINT('Ctrl Pts',(24.3531646875,56.7708333401613,-42.1809185638422));
#19015=CARTESIAN_POINT('Ctrl Pts',(35.6555077526845,56.562500006828,-35.6555077526845));
#19016=CARTESIAN_POINT('Ctrl Pts',(42.1809185638422,56.3541666734946,-24.3531646875));
#19017=CARTESIAN_POINT('Ctrl Pts',(48.706329375,56.1458333401613,-13.0508216223155));
#19018=CARTESIAN_POINT('Ctrl Pts',(48.706329375,55.937500006828,1.293339198242E-14));
#19019=CARTESIAN_POINT('Ctrl Pts',(48.706329375,55.7291666734946,13.0508216223155));
#19020=CARTESIAN_POINT('Ctrl Pts',(42.1809185638422,55.5208333401613,24.3531646875));
#19021=CARTESIAN_POINT('Ctrl Pts',(35.6555077526845,55.312500006828,35.6555077526845));
#19022=CARTESIAN_POINT('Ctrl Pts',(24.3531646875,55.1041666734946,42.1809185638422));
#19023=CARTESIAN_POINT('Ctrl Pts',(13.0508216223155,54.8958333401613,48.706329375));
#19024=CARTESIAN_POINT('Ctrl Pts',(-9.95098946405443E-15,54.687500006828,
48.706329375));
#19025=CARTESIAN_POINT('Ctrl Pts',(-13.0508216223155,54.4791666734946,48.706329375));
#19026=CARTESIAN_POINT('Ctrl Pts',(-24.3531646875,54.2708333401613,42.1809185638423));
#19027=CARTESIAN_POINT('Ctrl Pts',(-35.6555077526845,54.062500006828,35.6555077526845));
#19028=CARTESIAN_POINT('Ctrl Pts',(-42.1809185638422,53.8541666734946,24.3531646875));
#19029=CARTESIAN_POINT('Ctrl Pts',(-48.706329375,53.6458333401613,13.0508216223155));
#19030=CARTESIAN_POINT('Ctrl Pts',(-48.706329375,53.437500006828,-1.8898197019151E-14));
#19031=CARTESIAN_POINT('Ctrl Pts',(-48.706329375,53.2291666734946,-13.0508216223155));
#19032=CARTESIAN_POINT('Ctrl Pts',(-42.1809185638422,53.0208333401613,-24.3531646875));
#19033=CARTESIAN_POINT('Ctrl Pts',(-35.6555077526845,52.812500006828,-35.6555077526845));
#19034=CARTESIAN_POINT('Ctrl Pts',(-24.3531646875,52.6041666734946,-42.1809185638422));
#19035=CARTESIAN_POINT('Ctrl Pts',(-13.0508216223155,52.3958333401613,-48.706329375));
#19036=CARTESIAN_POINT('Ctrl Pts',(1.59157945007855E-14,52.187500006828,
-48.706329375));
#19037=CARTESIAN_POINT('Ctrl Pts',(13.0508216223155,51.9791666734946,-48.706329375));
#19038=CARTESIAN_POINT('Ctrl Pts',(24.3531646875,51.7708333401613,-42.1809185638422));
#19039=CARTESIAN_POINT('Ctrl Pts',(35.6555077526845,51.562500006828,-35.6555077526845));
#19040=CARTESIAN_POINT('Ctrl Pts',(42.1809185638422,51.3541666734946,-24.3531646875));
#19041=CARTESIAN_POINT('Ctrl Pts',(48.706329375,51.1458333401613,-13.0508216223155));
#19042=CARTESIAN_POINT('Ctrl Pts',(48.706329375,50.937500006828,1.293339198242E-14));
#19043=CARTESIAN_POINT('Ctrl Pts',(48.706329375,50.7291666734946,13.0508216223155));
#19044=CARTESIAN_POINT('Ctrl Pts',(42.1809185638422,50.5208333401613,24.3531646875));
#19045=CARTESIAN_POINT('Ctrl Pts',(35.6555077526845,50.312500006828,35.6555077526845));
#19046=CARTESIAN_POINT('Ctrl Pts',(24.3531646875,50.1041666734946,42.1809185638422));
#19047=CARTESIAN_POINT('Ctrl Pts',(13.0508216223155,49.8958333401613,48.706329375));
#19048=CARTESIAN_POINT('Ctrl Pts',(-9.95098946405443E-15,49.687500006828,
48.706329375));
#19049=CARTESIAN_POINT('Ctrl Pts',(-13.0508216223155,49.4791666734946,48.706329375));
#19050=CARTESIAN_POINT('Ctrl Pts',(-24.3531646875,49.2708333401613,42.1809185638423));
#19051=CARTESIAN_POINT('Ctrl Pts',(-35.6555077526845,49.062500006828,35.6555077526845));
#19052=CARTESIAN_POINT('Ctrl Pts',(-42.1809185638422,48.8541666734946,24.3531646875));
#19053=CARTESIAN_POINT('Ctrl Pts',(-48.706329375,48.6458333401613,13.0508216223155));
#19054=CARTESIAN_POINT('Ctrl Pts',(-48.706329375,48.437500006828,-1.8898197019151E-14));
#19055=CARTESIAN_POINT('Ctrl Pts',(-48.706329375,48.2291666734946,-13.0508216223155));
#19056=CARTESIAN_POINT('Ctrl Pts',(-42.1809185638422,48.0208333401613,-24.3531646875));
#19057=CARTESIAN_POINT('Ctrl Pts',(-35.6555077526845,47.812500006828,-35.6555077526845));
#19058=CARTESIAN_POINT('Ctrl Pts',(-24.3531646875,47.6041666734946,-42.1809185638422));
#19059=CARTESIAN_POINT('Ctrl Pts',(-13.0508216223155,47.3958333401613,-48.706329375));
#19060=CARTESIAN_POINT('Ctrl Pts',(1.59157945007855E-14,47.187500006828,
-48.706329375));
#19061=CARTESIAN_POINT('Ctrl Pts',(13.0508216223155,46.9791666734946,-48.706329375));
#19062=CARTESIAN_POINT('Ctrl Pts',(24.3531646875,46.7708333401613,-42.1809185638422));
#19063=CARTESIAN_POINT('Ctrl Pts',(35.6555077526845,46.562500006828,-35.6555077526845));
#19064=CARTESIAN_POINT('Ctrl Pts',(42.1809185638422,46.3541666734946,-24.3531646875));
#19065=CARTESIAN_POINT('Ctrl Pts',(48.706329375,46.1458333401613,-13.0508216223155));
#19066=CARTESIAN_POINT('Ctrl Pts',(48.706329375,45.937500006828,1.293339198242E-14));
#19067=CARTESIAN_POINT('Ctrl Pts',(48.706329375,45.7291666734946,13.0508216223155));
#19068=CARTESIAN_POINT('Ctrl Pts',(42.1809185638422,45.5208333401613,24.3531646875));
#19069=CARTESIAN_POINT('Ctrl Pts',(35.6555077526845,45.312500006828,35.6555077526845));
#19070=CARTESIAN_POINT('Ctrl Pts',(24.3531646875,45.1041666734946,42.1809185638422));
#19071=CARTESIAN_POINT('Ctrl Pts',(13.0508216223155,44.8958333401613,48.706329375));
#19072=CARTESIAN_POINT('Ctrl Pts',(-9.95098946405443E-15,44.687500006828,
48.706329375));
#19073=CARTESIAN_POINT('Ctrl Pts',(-13.0508216223155,44.4791666734946,48.706329375));
#19074=CARTESIAN_POINT('Ctrl Pts',(-24.3531646875,44.2708333401613,42.1809185638423));
#19075=CARTESIAN_POINT('Ctrl Pts',(-35.6555077526845,44.062500006828,35.6555077526845));
#19076=CARTESIAN_POINT('Ctrl Pts',(-42.1809185638422,43.8541666734946,24.3531646875));
#19077=CARTESIAN_POINT('Ctrl Pts',(-48.706329375,43.6458333401613,13.0508216223155));
#19078=CARTESIAN_POINT('Ctrl Pts',(-48.706329375,43.437500006828,-1.8898197019151E-14));
#19079=CARTESIAN_POINT('Ctrl Pts',(-48.706329375,43.2291666734946,-13.0508216223155));
#19080=CARTESIAN_POINT('Ctrl Pts',(-42.1809185638422,43.0208333401613,-24.3531646875));
#19081=CARTESIAN_POINT('Ctrl Pts',(-35.6555077526845,42.812500006828,-35.6555077526845));
#19082=CARTESIAN_POINT('Ctrl Pts',(-24.3531646875,42.6041666734946,-42.1809185638422));
#19083=CARTESIAN_POINT('Ctrl Pts',(-13.0508216223155,42.3958333401613,-48.706329375));
#19084=CARTESIAN_POINT('Ctrl Pts',(1.59157945007855E-14,42.187500006828,
-48.706329375));
#19085=CARTESIAN_POINT('Ctrl Pts',(13.0508216223155,41.9791666734946,-48.706329375));
#19086=CARTESIAN_POINT('Ctrl Pts',(24.3531646875,41.7708333401613,-42.1809185638422));
#19087=CARTESIAN_POINT('Ctrl Pts',(35.6555077526845,41.562500006828,-35.6555077526845));
#19088=CARTESIAN_POINT('Ctrl Pts',(42.1809185638422,41.3541666734946,-24.3531646875));
#19089=CARTESIAN_POINT('Ctrl Pts',(48.706329375,41.1458333401613,-13.0508216223155));
#19090=CARTESIAN_POINT('Ctrl Pts',(48.706329375,40.937500006828,1.293339198242E-14));
#19091=CARTESIAN_POINT('Ctrl Pts',(48.706329375,40.7291666734946,13.0508216223155));
#19092=CARTESIAN_POINT('Ctrl Pts',(42.1809185638422,40.5208333401613,24.3531646875));
#19093=CARTESIAN_POINT('Ctrl Pts',(35.6555077526845,40.312500006828,35.6555077526845));
#19094=CARTESIAN_POINT('Ctrl Pts',(24.3531646875,40.1041666734946,42.1809185638422));
#19095=CARTESIAN_POINT('Ctrl Pts',(13.0508216223155,39.8958333401613,48.706329375));
#19096=CARTESIAN_POINT('Ctrl Pts',(-9.95098946405443E-15,39.687500006828,
48.706329375));
#19097=CARTESIAN_POINT('Ctrl Pts',(-13.0508216223155,39.4791666734946,48.706329375));
#19098=CARTESIAN_POINT('Ctrl Pts',(-24.3531646875,39.2708333401613,42.1809185638423));
#19099=CARTESIAN_POINT('Ctrl Pts',(-35.6555077526845,39.062500006828,35.6555077526845));
#19100=CARTESIAN_POINT('Ctrl Pts',(-42.1809185638422,38.8541666734946,24.3531646875));
#19101=CARTESIAN_POINT('Ctrl Pts',(-48.706329375,38.6458333401613,13.0508216223155));
#19102=CARTESIAN_POINT('Ctrl Pts',(-48.706329375,38.437500006828,-1.8898197019151E-14));
#19103=CARTESIAN_POINT('Ctrl Pts',(-48.706329375,38.2291666734946,-13.0508216223155));
#19104=CARTESIAN_POINT('Ctrl Pts',(-42.1809185638422,38.0208333401613,-24.3531646875));
#19105=CARTESIAN_POINT('Ctrl Pts',(-35.6555077526845,37.812500006828,-35.6555077526845));
#19106=CARTESIAN_POINT('Ctrl Pts',(-24.3531646875,37.6041666734946,-42.1809185638422));
#19107=CARTESIAN_POINT('Ctrl Pts',(-13.0508216223155,37.3958333401613,-48.706329375));
#19108=CARTESIAN_POINT('Ctrl Pts',(1.59157945007855E-14,37.187500006828,
-48.706329375));
#19109=CARTESIAN_POINT('Ctrl Pts',(13.0508216223155,36.9791666734946,-48.706329375));
#19110=CARTESIAN_POINT('Ctrl Pts',(24.3531646875,36.7708333401613,-42.1809185638422));
#19111=CARTESIAN_POINT('Ctrl Pts',(35.6555077526845,36.562500006828,-35.6555077526845));
#19112=CARTESIAN_POINT('Ctrl Pts',(42.1809185638422,36.3541666734946,-24.3531646875));
#19113=CARTESIAN_POINT('Ctrl Pts',(48.706329375,36.1458333401613,-13.0508216223155));
#19114=CARTESIAN_POINT('Ctrl Pts',(48.706329375,35.937500006828,1.293339198242E-14));
#19115=CARTESIAN_POINT('Ctrl Pts',(48.706329375,35.7291666734946,13.0508216223155));
#19116=CARTESIAN_POINT('Ctrl Pts',(42.1809185638422,35.5208333401613,24.3531646875));
#19117=CARTESIAN_POINT('Ctrl Pts',(35.6555077526845,35.312500006828,35.6555077526845));
#19118=CARTESIAN_POINT('Ctrl Pts',(24.3531646875,35.1041666734946,42.1809185638422));
#19119=CARTESIAN_POINT('Ctrl Pts',(13.0508216223155,34.8958333401613,48.706329375));
#19120=CARTESIAN_POINT('Ctrl Pts',(-9.95098946405443E-15,34.687500006828,
48.706329375));
#19121=CARTESIAN_POINT('Ctrl Pts',(-13.0508216223155,34.4791666734946,48.706329375));
#19122=CARTESIAN_POINT('Ctrl Pts',(-24.3531646875,34.2708333401613,42.1809185638423));
#19123=CARTESIAN_POINT('Ctrl Pts',(-35.6555077526845,34.062500006828,35.6555077526845));
#19124=CARTESIAN_POINT('Ctrl Pts',(-42.1809185638422,33.8541666734946,24.3531646875));
#19125=CARTESIAN_POINT('Ctrl Pts',(-48.706329375,33.6458333401613,13.0508216223155));
#19126=CARTESIAN_POINT('Ctrl Pts',(-48.706329375,33.437500006828,-1.8898197019151E-14));
#19127=CARTESIAN_POINT('Ctrl Pts',(-48.706329375,33.2291666734946,-13.0508216223155));
#19128=CARTESIAN_POINT('Ctrl Pts',(-42.1809185638422,33.0208333401613,-24.3531646875));
#19129=CARTESIAN_POINT('Ctrl Pts',(-35.6555077526845,32.812500006828,-35.6555077526845));
#19130=CARTESIAN_POINT('Ctrl Pts',(-24.3531646875,32.6041666734946,-42.1809185638422));
#19131=CARTESIAN_POINT('Ctrl Pts',(-13.0508216223155,32.3958333401613,-48.706329375));
#19132=CARTESIAN_POINT('Ctrl Pts',(1.59157945007855E-14,32.187500006828,
-48.706329375));
#19133=CARTESIAN_POINT('Ctrl Pts',(13.0508216223155,31.9791666734946,-48.706329375));
#19134=CARTESIAN_POINT('Ctrl Pts',(24.3531646875,31.7708333401613,-42.1809185638422));
#19135=CARTESIAN_POINT('Ctrl Pts',(35.6555077526845,31.562500006828,-35.6555077526845));
#19136=CARTESIAN_POINT('Ctrl Pts',(42.1809185638422,31.3541666734946,-24.3531646875));
#19137=CARTESIAN_POINT('Ctrl Pts',(48.706329375,31.1458333401613,-13.0508216223155));
#19138=CARTESIAN_POINT('Ctrl Pts',(48.706329375,30.937500006828,1.293339198242E-14));
#19139=CARTESIAN_POINT('Ctrl Pts',(48.706329375,30.7291666734946,13.0508216223155));
#19140=CARTESIAN_POINT('Ctrl Pts',(42.1809185638422,30.5208333401613,24.3531646875));
#19141=CARTESIAN_POINT('Ctrl Pts',(35.6555077526845,30.312500006828,35.6555077526845));
#19142=CARTESIAN_POINT('Ctrl Pts',(24.3531646875,30.1041666734946,42.1809185638422));
#19143=CARTESIAN_POINT('Ctrl Pts',(13.0508216223155,29.8958333401613,48.706329375));
#19144=CARTESIAN_POINT('Ctrl Pts',(-9.95098946405443E-15,29.687500006828,
48.706329375));
#19145=CARTESIAN_POINT('Ctrl Pts',(-13.0508216223155,29.4791666734946,48.706329375));
#19146=CARTESIAN_POINT('Ctrl Pts',(-24.3531646875,29.2708333401613,42.1809185638423));
#19147=CARTESIAN_POINT('Ctrl Pts',(-35.6555077526845,29.062500006828,35.6555077526845));
#19148=CARTESIAN_POINT('Ctrl Pts',(-42.1809185638422,28.8541666734946,24.3531646875));
#19149=CARTESIAN_POINT('Ctrl Pts',(-48.706329375,28.6458333401613,13.0508216223155));
#19150=CARTESIAN_POINT('Ctrl Pts',(-48.706329375,28.437500006828,-1.8898197019151E-14));
#19151=CARTESIAN_POINT('Ctrl Pts',(-46.,60.,0.));
#19152=CARTESIAN_POINT('Ctrl Pts',(-46.,59.7916666666667,-12.3256628518316));
#19153=CARTESIAN_POINT('Ctrl Pts',(-39.8371685740842,59.5833333333333,-23.));
#19154=CARTESIAN_POINT('Ctrl Pts',(-33.6743371481684,59.375,-33.6743371481684));
#19155=CARTESIAN_POINT('Ctrl Pts',(-23.,59.1666666666667,-39.8371685740842));
#19156=CARTESIAN_POINT('Ctrl Pts',(-12.3256628518317,58.9583333333333,-46.));
#19157=CARTESIAN_POINT('Ctrl Pts',(-2.81668763803891E-15,58.75,-46.));
#19158=CARTESIAN_POINT('Ctrl Pts',(12.3256628518316,58.5416666666667,-46.));
#19159=CARTESIAN_POINT('Ctrl Pts',(23.,58.3333333333333,-39.8371685740842));
#19160=CARTESIAN_POINT('Ctrl Pts',(33.6743371481683,58.125,-33.6743371481684));
#19161=CARTESIAN_POINT('Ctrl Pts',(39.8371685740842,57.9166666666667,-23.));
#19162=CARTESIAN_POINT('Ctrl Pts',(46.,57.7083333333333,-12.3256628518317));
#19163=CARTESIAN_POINT('Ctrl Pts',(46.,57.5,-5.63337527607782E-15));
#19164=CARTESIAN_POINT('Ctrl Pts',(46.,57.2916666666667,12.3256628518316));
#19165=CARTESIAN_POINT('Ctrl Pts',(39.8371685740842,57.0833333333333,23.));
#19166=CARTESIAN_POINT('Ctrl Pts',(33.6743371481684,56.875,33.6743371481683));
#19167=CARTESIAN_POINT('Ctrl Pts',(23.,56.6666666666667,39.8371685740842));
#19168=CARTESIAN_POINT('Ctrl Pts',(12.3256628518317,56.4583333333333,46.));
#19169=CARTESIAN_POINT('Ctrl Pts',(8.45006291411674E-15,56.25,46.));
#19170=CARTESIAN_POINT('Ctrl Pts',(-12.3256628518316,56.0416666666667,46.));
#19171=CARTESIAN_POINT('Ctrl Pts',(-23.,55.8333333333333,39.8371685740842));
#19172=CARTESIAN_POINT('Ctrl Pts',(-33.6743371481683,55.625,33.6743371481684));
#19173=CARTESIAN_POINT('Ctrl Pts',(-39.8371685740842,55.4166666666667,23.));
#19174=CARTESIAN_POINT('Ctrl Pts',(-46.,55.2083333333333,12.3256628518317));
#19175=CARTESIAN_POINT('Ctrl Pts',(-46.,55.,0.));
#19176=CARTESIAN_POINT('Ctrl Pts',(-46.,54.7916666666667,-12.3256628518316));
#19177=CARTESIAN_POINT('Ctrl Pts',(-39.8371685740842,54.5833333333333,-23.));
#19178=CARTESIAN_POINT('Ctrl Pts',(-33.6743371481684,54.375,-33.6743371481684));
#19179=CARTESIAN_POINT('Ctrl Pts',(-23.,54.1666666666667,-39.8371685740842));
#19180=CARTESIAN_POINT('Ctrl Pts',(-12.3256628518317,53.9583333333333,-46.));
#19181=CARTESIAN_POINT('Ctrl Pts',(-2.81668763803891E-15,53.75,-46.));
#19182=CARTESIAN_POINT('Ctrl Pts',(12.3256628518316,53.5416666666667,-46.));
#19183=CARTESIAN_POINT('Ctrl Pts',(23.,53.3333333333333,-39.8371685740842));
#19184=CARTESIAN_POINT('Ctrl Pts',(33.6743371481683,53.125,-33.6743371481684));
#19185=CARTESIAN_POINT('Ctrl Pts',(39.8371685740842,52.9166666666667,-23.));
#19186=CARTESIAN_POINT('Ctrl Pts',(46.,52.7083333333333,-12.3256628518317));
#19187=CARTESIAN_POINT('Ctrl Pts',(46.,52.5,-5.63337527607782E-15));
#19188=CARTESIAN_POINT('Ctrl Pts',(46.,52.2916666666667,12.3256628518316));
#19189=CARTESIAN_POINT('Ctrl Pts',(39.8371685740842,52.0833333333333,23.));
#19190=CARTESIAN_POINT('Ctrl Pts',(33.6743371481684,51.875,33.6743371481683));
#19191=CARTESIAN_POINT('Ctrl Pts',(23.,51.6666666666667,39.8371685740842));
#19192=CARTESIAN_POINT('Ctrl Pts',(12.3256628518317,51.4583333333333,46.));
#19193=CARTESIAN_POINT('Ctrl Pts',(8.45006291411674E-15,51.25,46.));
#19194=CARTESIAN_POINT('Ctrl Pts',(-12.3256628518316,51.0416666666667,46.));
#19195=CARTESIAN_POINT('Ctrl Pts',(-23.,50.8333333333333,39.8371685740842));
#19196=CARTESIAN_POINT('Ctrl Pts',(-33.6743371481683,50.625,33.6743371481684));
#19197=CARTESIAN_POINT('Ctrl Pts',(-39.8371685740842,50.4166666666667,23.));
#19198=CARTESIAN_POINT('Ctrl Pts',(-46.,50.2083333333333,12.3256628518317));
#19199=CARTESIAN_POINT('Ctrl Pts',(-46.,50.,0.));
#19200=CARTESIAN_POINT('Ctrl Pts',(-46.,49.7916666666667,-12.3256628518316));
#19201=CARTESIAN_POINT('Ctrl Pts',(-39.8371685740842,49.5833333333333,-23.));
#19202=CARTESIAN_POINT('Ctrl Pts',(-33.6743371481684,49.375,-33.6743371481684));
#19203=CARTESIAN_POINT('Ctrl Pts',(-23.,49.1666666666667,-39.8371685740842));
#19204=CARTESIAN_POINT('Ctrl Pts',(-12.3256628518317,48.9583333333333,-46.));
#19205=CARTESIAN_POINT('Ctrl Pts',(-2.81668763803891E-15,48.75,-46.));
#19206=CARTESIAN_POINT('Ctrl Pts',(12.3256628518316,48.5416666666667,-46.));
#19207=CARTESIAN_POINT('Ctrl Pts',(23.,48.3333333333333,-39.8371685740842));
#19208=CARTESIAN_POINT('Ctrl Pts',(33.6743371481683,48.125,-33.6743371481684));
#19209=CARTESIAN_POINT('Ctrl Pts',(39.8371685740842,47.9166666666667,-23.));
#19210=CARTESIAN_POINT('Ctrl Pts',(46.,47.7083333333333,-12.3256628518317));
#19211=CARTESIAN_POINT('Ctrl Pts',(46.,47.5,-5.63337527607782E-15));
#19212=CARTESIAN_POINT('Ctrl Pts',(46.,47.2916666666667,12.3256628518316));
#19213=CARTESIAN_POINT('Ctrl Pts',(39.8371685740842,47.0833333333333,23.));
#19214=CARTESIAN_POINT('Ctrl Pts',(33.6743371481684,46.875,33.6743371481683));
#19215=CARTESIAN_POINT('Ctrl Pts',(23.,46.6666666666667,39.8371685740842));
#19216=CARTESIAN_POINT('Ctrl Pts',(12.3256628518317,46.4583333333333,46.));
#19217=CARTESIAN_POINT('Ctrl Pts',(8.45006291411674E-15,46.25,46.));
#19218=CARTESIAN_POINT('Ctrl Pts',(-12.3256628518316,46.0416666666667,46.));
#19219=CARTESIAN_POINT('Ctrl Pts',(-23.,45.8333333333333,39.8371685740842));
#19220=CARTESIAN_POINT('Ctrl Pts',(-33.6743371481683,45.625,33.6743371481684));
#19221=CARTESIAN_POINT('Ctrl Pts',(-39.8371685740842,45.4166666666667,23.));
#19222=CARTESIAN_POINT('Ctrl Pts',(-46.,45.2083333333333,12.3256628518317));
#19223=CARTESIAN_POINT('Ctrl Pts',(-46.,45.,0.));
#19224=CARTESIAN_POINT('Ctrl Pts',(-46.,44.7916666666667,-12.3256628518316));
#19225=CARTESIAN_POINT('Ctrl Pts',(-39.8371685740842,44.5833333333333,-23.));
#19226=CARTESIAN_POINT('Ctrl Pts',(-33.6743371481684,44.375,-33.6743371481684));
#19227=CARTESIAN_POINT('Ctrl Pts',(-23.,44.1666666666667,-39.8371685740842));
#19228=CARTESIAN_POINT('Ctrl Pts',(-12.3256628518317,43.9583333333333,-46.));
#19229=CARTESIAN_POINT('Ctrl Pts',(-2.81668763803891E-15,43.75,-46.));
#19230=CARTESIAN_POINT('Ctrl Pts',(12.3256628518316,43.5416666666667,-46.));
#19231=CARTESIAN_POINT('Ctrl Pts',(23.,43.3333333333333,-39.8371685740842));
#19232=CARTESIAN_POINT('Ctrl Pts',(33.6743371481683,43.125,-33.6743371481684));
#19233=CARTESIAN_POINT('Ctrl Pts',(39.8371685740842,42.9166666666667,-23.));
#19234=CARTESIAN_POINT('Ctrl Pts',(46.,42.7083333333333,-12.3256628518317));
#19235=CARTESIAN_POINT('Ctrl Pts',(46.,42.5,-5.63337527607782E-15));
#19236=CARTESIAN_POINT('Ctrl Pts',(46.,42.2916666666667,12.3256628518316));
#19237=CARTESIAN_POINT('Ctrl Pts',(39.8371685740842,42.0833333333333,23.));
#19238=CARTESIAN_POINT('Ctrl Pts',(33.6743371481684,41.875,33.6743371481683));
#19239=CARTESIAN_POINT('Ctrl Pts',(23.,41.6666666666667,39.8371685740842));
#19240=CARTESIAN_POINT('Ctrl Pts',(12.3256628518317,41.4583333333333,46.));
#19241=CARTESIAN_POINT('Ctrl Pts',(8.45006291411674E-15,41.25,46.));
#19242=CARTESIAN_POINT('Ctrl Pts',(-12.3256628518316,41.0416666666667,46.));
#19243=CARTESIAN_POINT('Ctrl Pts',(-23.,40.8333333333333,39.8371685740842));
#19244=CARTESIAN_POINT('Ctrl Pts',(-33.6743371481683,40.625,33.6743371481684));
#19245=CARTESIAN_POINT('Ctrl Pts',(-39.8371685740842,40.4166666666667,23.));
#19246=CARTESIAN_POINT('Ctrl Pts',(-46.,40.2083333333333,12.3256628518317));
#19247=CARTESIAN_POINT('Ctrl Pts',(-46.,40.,0.));
#19248=CARTESIAN_POINT('Ctrl Pts',(-46.,39.7916666666667,-12.3256628518316));
#19249=CARTESIAN_POINT('Ctrl Pts',(-39.8371685740842,39.5833333333333,-23.));
#19250=CARTESIAN_POINT('Ctrl Pts',(-33.6743371481684,39.375,-33.6743371481684));
#19251=CARTESIAN_POINT('Ctrl Pts',(-23.,39.1666666666667,-39.8371685740842));
#19252=CARTESIAN_POINT('Ctrl Pts',(-12.3256628518317,38.9583333333333,-46.));
#19253=CARTESIAN_POINT('Ctrl Pts',(-2.81668763803891E-15,38.75,-46.));
#19254=CARTESIAN_POINT('Ctrl Pts',(12.3256628518316,38.5416666666667,-46.));
#19255=CARTESIAN_POINT('Ctrl Pts',(23.,38.3333333333333,-39.8371685740842));
#19256=CARTESIAN_POINT('Ctrl Pts',(33.6743371481683,38.125,-33.6743371481684));
#19257=CARTESIAN_POINT('Ctrl Pts',(39.8371685740842,37.9166666666667,-23.));
#19258=CARTESIAN_POINT('Ctrl Pts',(46.,37.7083333333333,-12.3256628518317));
#19259=CARTESIAN_POINT('Ctrl Pts',(46.,37.5,-5.63337527607782E-15));
#19260=CARTESIAN_POINT('Ctrl Pts',(46.,37.2916666666667,12.3256628518316));
#19261=CARTESIAN_POINT('Ctrl Pts',(39.8371685740842,37.0833333333333,23.));
#19262=CARTESIAN_POINT('Ctrl Pts',(33.6743371481684,36.875,33.6743371481683));
#19263=CARTESIAN_POINT('Ctrl Pts',(23.,36.6666666666667,39.8371685740842));
#19264=CARTESIAN_POINT('Ctrl Pts',(12.3256628518317,36.4583333333333,46.));
#19265=CARTESIAN_POINT('Ctrl Pts',(8.45006291411674E-15,36.25,46.));
#19266=CARTESIAN_POINT('Ctrl Pts',(-12.3256628518316,36.0416666666667,46.));
#19267=CARTESIAN_POINT('Ctrl Pts',(-23.,35.8333333333333,39.8371685740842));
#19268=CARTESIAN_POINT('Ctrl Pts',(-33.6743371481683,35.625,33.6743371481684));
#19269=CARTESIAN_POINT('Ctrl Pts',(-39.8371685740842,35.4166666666667,23.));
#19270=CARTESIAN_POINT('Ctrl Pts',(-46.,35.2083333333333,12.3256628518317));
#19271=CARTESIAN_POINT('Ctrl Pts',(-46.,35.,0.));
#19272=CARTESIAN_POINT('Ctrl Pts',(-46.,34.7916666666667,-12.3256628518316));
#19273=CARTESIAN_POINT('Ctrl Pts',(-39.8371685740842,34.5833333333333,-23.));
#19274=CARTESIAN_POINT('Ctrl Pts',(-33.6743371481684,34.375,-33.6743371481684));
#19275=CARTESIAN_POINT('Ctrl Pts',(-23.,34.1666666666667,-39.8371685740842));
#19276=CARTESIAN_POINT('Ctrl Pts',(-12.3256628518317,33.9583333333333,-46.));
#19277=CARTESIAN_POINT('Ctrl Pts',(-2.81668763803891E-15,33.75,-46.));
#19278=CARTESIAN_POINT('Ctrl Pts',(12.3256628518316,33.5416666666667,-46.));
#19279=CARTESIAN_POINT('Ctrl Pts',(23.,33.3333333333333,-39.8371685740842));
#19280=CARTESIAN_POINT('Ctrl Pts',(33.6743371481683,33.125,-33.6743371481684));
#19281=CARTESIAN_POINT('Ctrl Pts',(39.8371685740842,32.9166666666667,-23.));
#19282=CARTESIAN_POINT('Ctrl Pts',(46.,32.7083333333333,-12.3256628518317));
#19283=CARTESIAN_POINT('Ctrl Pts',(46.,32.5,-5.63337527607782E-15));
#19284=CARTESIAN_POINT('Ctrl Pts',(46.,32.2916666666667,12.3256628518316));
#19285=CARTESIAN_POINT('Ctrl Pts',(39.8371685740842,32.0833333333333,23.));
#19286=CARTESIAN_POINT('Ctrl Pts',(33.6743371481684,31.875,33.6743371481683));
#19287=CARTESIAN_POINT('Ctrl Pts',(23.,31.6666666666667,39.8371685740842));
#19288=CARTESIAN_POINT('Ctrl Pts',(12.3256628518317,31.4583333333333,46.));
#19289=CARTESIAN_POINT('Ctrl Pts',(8.45006291411674E-15,31.25,46.));
#19290=CARTESIAN_POINT('Ctrl Pts',(-12.3256628518316,31.0416666666667,46.));
#19291=CARTESIAN_POINT('Ctrl Pts',(-23.,30.8333333333333,39.8371685740842));
#19292=CARTESIAN_POINT('Ctrl Pts',(-33.6743371481683,30.625,33.6743371481684));
#19293=CARTESIAN_POINT('Ctrl Pts',(-39.8371685740842,30.4166666666667,23.));
#19294=CARTESIAN_POINT('Ctrl Pts',(-46.,30.2083333333333,12.3256628518317));
#19295=CARTESIAN_POINT('Ctrl Pts',(-46.,30.,0.));
#19296=CARTESIAN_POINT('',(-46.6620925223333,29.597913825102,3.60701400320327));
#19297=CARTESIAN_POINT('',(-45.858362923034,30.061608680256,3.60701400320318));
#19298=CARTESIAN_POINT('Ctrl Pts',(-46.6620925223333,29.597913825102,3.60701400320326));
#19299=CARTESIAN_POINT('Ctrl Pts',(-46.9829117922315,29.4128216316687,3.60701400320326));
#19300=CARTESIAN_POINT('Ctrl Pts',(-47.3046963748559,29.2275305610077,3.5940657325934));
#19301=CARTESIAN_POINT('Ctrl Pts',(-47.9453311027174,28.8592841960704,3.54210581887907));
#19302=CARTESIAN_POINT('Ctrl Pts',(-48.2659302181934,28.6753237953703,3.50295023343856));
#19303=CARTESIAN_POINT('Ctrl Pts',(-48.5839797682363,28.4930986521586,3.45013493440412));
#19304=CARTESIAN_POINT('Ctrl Pts',(48.5725845633798,30.8793483229262,3.60701400320327));
#19305=CARTESIAN_POINT('Ctrl Pts',(48.3407853679392,31.0125314497137,3.60701400320327));
#19306=CARTESIAN_POINT('Ctrl Pts',(48.1089821836664,31.1457076343818,3.60701400320325));
#19307=CARTESIAN_POINT('Ctrl Pts',(47.6453674864979,31.4120455056142,3.60701400320325));
#19308=CARTESIAN_POINT('Ctrl Pts',(47.4135559734253,31.5452071923974,3.60701400320323));
#19309=CARTESIAN_POINT('Ctrl Pts',(47.1817401099609,31.6783613050641,3.60701400320323));
#19310=CARTESIAN_POINT('Ctrl Pts',(46.7406305897488,31.9317328641751,3.60701400320323));
#19311=CARTESIAN_POINT('Ctrl Pts',(46.2995053259033,32.1850770165972,3.60701400320323));
#19312=CARTESIAN_POINT('Ctrl Pts',(45.858362923034,32.438391319744,3.60701400320325));
#19313=CARTESIAN_POINT('Origin',(107.751358612144,29.597913825102,-0.361735996796731));
#19314=CARTESIAN_POINT('',(65.,29.597913825102,-4.33048599679673));
#19315=CARTESIAN_POINT('',(107.751358612144,28.,-3.99459271982449));
#19316=CARTESIAN_POINT('',(107.751358612144,28.,3.27112072623103));
#19317=CARTESIAN_POINT('',(65.,29.597913825102,3.60701400320327));
#19318=CARTESIAN_POINT('Origin',(107.751358612144,29.597913825102,-0.361735996796731));
#19319=CARTESIAN_POINT('',(107.751358612144,29.597913825102,-4.33048599679673));
#19320=CARTESIAN_POINT('',(107.751358612144,29.597913825102,3.60701400320327));
#19321=CARTESIAN_POINT('',(45.8835457347666,28.,3.27112072623103));
#19322=CARTESIAN_POINT('Origin',(46.089894195239,29.5885902225026,-0.356468963009084));
#19323=CARTESIAN_POINT('',(107.751358612144,28.,3.27112072623103));
#19324=CARTESIAN_POINT('',(107.751358612144,28.,-3.99459271982449));
#19325=CARTESIAN_POINT('Origin',(0.,60.,0.));
#19326=CARTESIAN_POINT('',(3.61292728433799,60.,45.8578974271399));
#19327=CARTESIAN_POINT('Origin',(0.,57.,0.));
#19328=CARTESIAN_POINT('',(3.61292728433799,57.,-48.4459777332189));
#19329=CARTESIAN_POINT('Origin',(-0.355816377580837,36.9438035983105,109.846845895932));
#19330=CARTESIAN_POINT('',(-4.32456320853981,36.9438035983105,109.846845895932));
#19331=CARTESIAN_POINT('',(3.61293045337858,36.9438035983105,109.846845895932));
#19332=CARTESIAN_POINT('Origin',(0.,60.,0.));
#19333=CARTESIAN_POINT('Origin',(0.,28.,0.));
#19334=CARTESIAN_POINT('Origin',(0.,28.,0.));
#19335=CARTESIAN_POINT('Origin',(0.,28.,0.));
#19336=CARTESIAN_POINT('Origin',(0.,0.,0.));
#19337=CARTESIAN_POINT('Origin',(0.,20.,0.));
#19338=CARTESIAN_POINT('Origin',(-0.355816377580837,36.9438035983105,109.846845895932));
#19339=CARTESIAN_POINT('',(-4.32456320853981,36.9438035983105,109.846845895932));
#19340=CARTESIAN_POINT('',(3.61293045337858,36.9438035983105,109.846845895932));
#19341=CARTESIAN_POINT('Origin',(-4.32456003949879,64.1203831012736,71.));
#19342=CARTESIAN_POINT('Origin',(3.61292728433799,36.9367107508029,71.));
#19343=CARTESIAN_POINT('Origin',(-4.32456003949879,64.1203831012736,71.));
#19344=CARTESIAN_POINT('Origin',(3.61292728433799,36.9367107508029,71.));
#19345=CARTESIAN_POINT('Origin',(65.,29.597913825102,3.60701400320327));
#19346=CARTESIAN_POINT('Origin',(65.,60.4726068567958,-4.33048599679673));
#19347=CARTESIAN_POINT('Origin',(65.,29.597913825102,3.60701400320327));
#19348=CARTESIAN_POINT('Origin',(65.,60.4726068567958,-4.33048599679673));
#19349=CARTESIAN_POINT('Origin',(65.,60.4726068567958,-4.33048599679673));
#19350=CARTESIAN_POINT('Origin',(0.,3.42,0.));
#20635=UNCERTAINTY_MEASURE_WITH_UNIT(LENGTH_MEASURE(0.01),#20659,
'DISTANCE_ACCURACY_VALUE',
'Maximum model space distance between geometric entities at asserted c
onnectivities');
#20644=UNCERTAINTY_MEASURE_WITH_UNIT(LENGTH_MEASURE(0.01),#20659,
'DISTANCE_ACCURACY_VALUE',
'Maximum model space distance between geometric entities at asserted c
onnectivities');
#20649=(
GEOMETRIC_REPRESENTATION_CONTEXT(3)
GLOBAL_UNCERTAINTY_ASSIGNED_CONTEXT((#20635))
GLOBAL_UNIT_ASSIGNED_CONTEXT((#20659,#20661,#20662))
REPRESENTATION_CONTEXT('','3D')
);
#20658=(
GEOMETRIC_REPRESENTATION_CONTEXT(3)
GLOBAL_UNCERTAINTY_ASSIGNED_CONTEXT((#20644))
GLOBAL_UNIT_ASSIGNED_CONTEXT((#20659,#20661,#20662))
REPRESENTATION_CONTEXT('','3D')
);
#20659=(
LENGTH_UNIT()
NAMED_UNIT(*)
SI_UNIT(.MILLI.,.METRE.)
);
#20661=(
NAMED_UNIT(*)
PLANE_ANGLE_UNIT()
SI_UNIT($,.RADIAN.)
);
#20662=(
NAMED_UNIT(*)
SI_UNIT($,.STERADIAN.)
SOLID_ANGLE_UNIT()
);
#20667=SHAPE_DEFINITION_REPRESENTATION(#20680,#20719);
#20680=PRODUCT_DEFINITION_SHAPE('',$,#20733);
#20719=SHAPE_REPRESENTATION('',(#3813),#20649);
#20728=PRODUCT_DEFINITION_CONTEXT('part definition',#20769,'design');
#20733=PRODUCT_DEFINITION('Rotating Hub','Rotating Hub',#20746,#20728);
#20746=PRODUCT_DEFINITION_FORMATION('',$,#20775);
#20769=APPLICATION_CONTEXT(
'Core Data for Automotive Mechanical Design Process');
#20770=PRODUCT_CONTEXT('part definition',#20769,'mechanical');
#20775=PRODUCT('Rotating Hub','Rotating Hub',$,(#20770));
#20786=PRESENTATION_STYLE_ASSIGNMENT((#20791));
#20791=SURFACE_STYLE_USAGE(.BOTH.,#20796);
#20796=SURFACE_SIDE_STYLE('',(#20801));
#20801=SURFACE_STYLE_FILL_AREA(#20806);
#20806=FILL_AREA_STYLE('Opaque(61,176,222)',(#20811));
#20811=FILL_AREA_STYLE_COLOUR('Opaque(61,176,222)',#20816);
#20816=COLOUR_RGB('Opaque(61,176,222)',0.23921568627451,0.690196078431373,
0.870588235294118);
ENDSEC;
END-ISO-10303-21;
